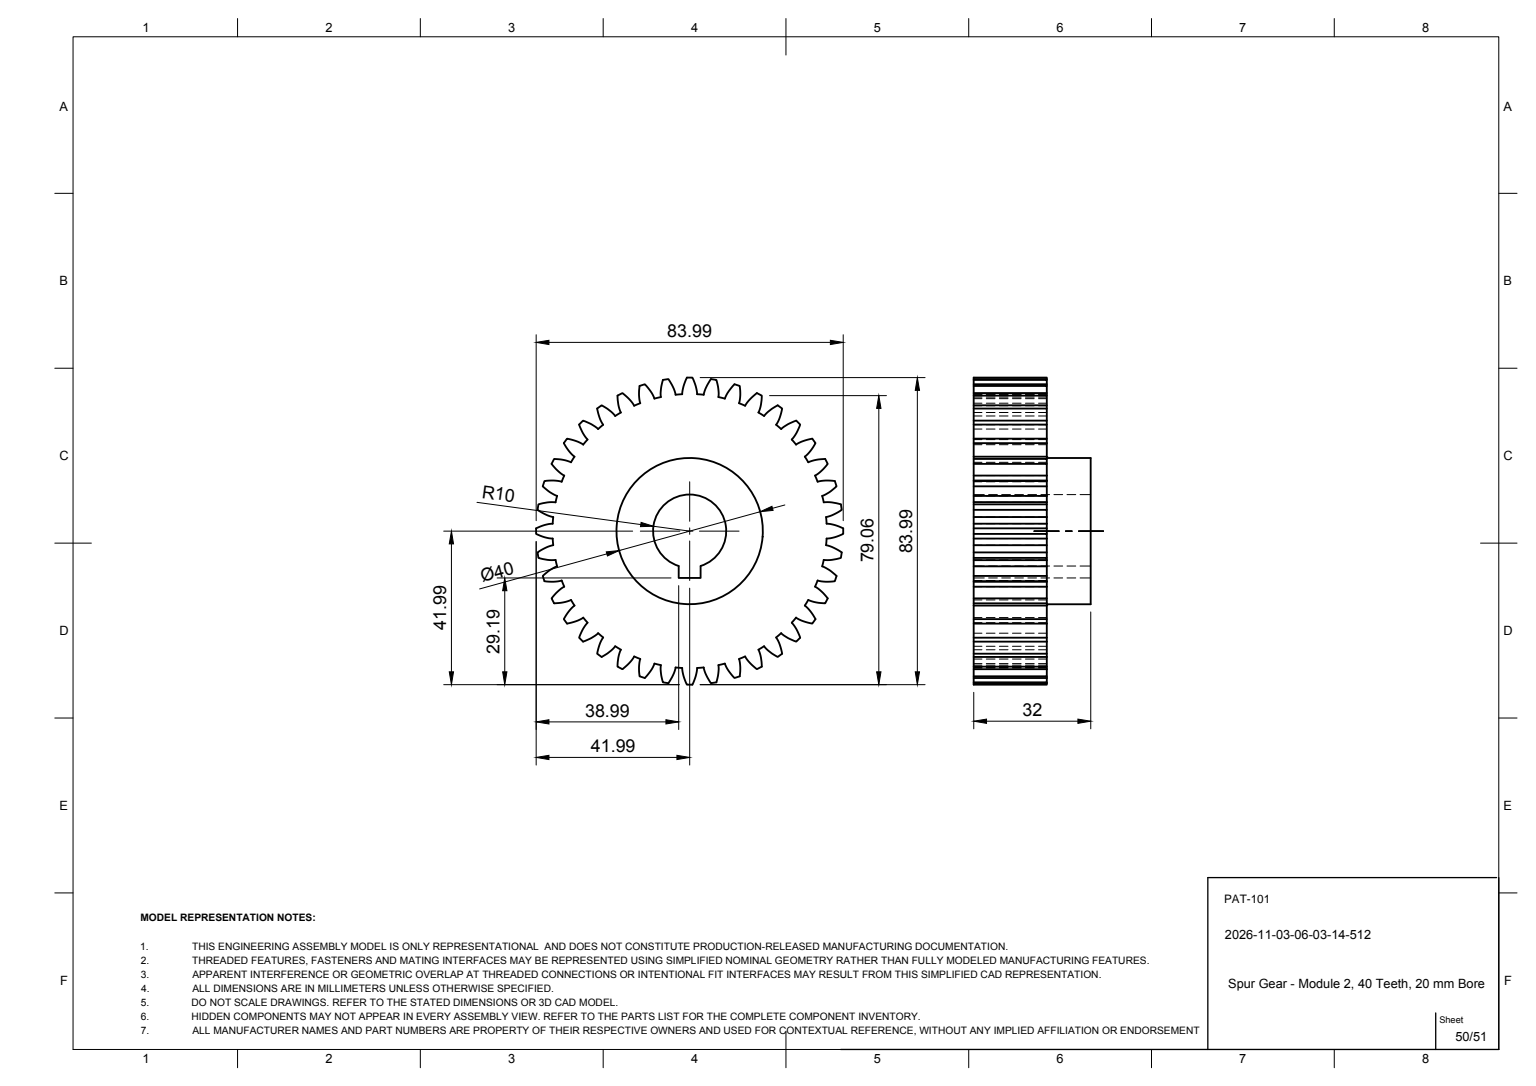
ISO-10303-21;
HEADER;
/* Generated by software containing ST-Developer
 * from STEP Tools, Inc. (www.steptools.com) 
 */

FILE_DESCRIPTION(
/* description */ ('Spur gear reduction stage 2-1 on bearing plates'),
/* implementation_level */ '2;1');

FILE_NAME(
/* name */ 'Spur Gear - Module 2, 40 Teeth, 20 mm Bore.step',
/* time_stamp */ '2026-10-28T03:22:07-07:00',
/* author */ (''),
/* organization */ (''),
/* preprocessor_version */ 'ST-DEVELOPER v20.2',
/* originating_system */ 'Autodesk Translation Framework v15.17.0.0',
/* authorisation */ '');

FILE_SCHEMA (('AUTOMOTIVE_DESIGN { 1 0 10303 214 3 1 1 }'));
ENDSEC;

DATA;
#10=MECHANICAL_DESIGN_GEOMETRIC_PRESENTATION_REPRESENTATION('',(#1002),#53909);
#51=(
BOUNDED_SURFACE()
B_SPLINE_SURFACE(5,1,((#35999,#36000),(#36001,#36002),(#36003,#36004),(#36005,
#36006),(#36007,#36008),(#36009,#36010),(#36011,#36012),(#36013,#36014),
(#36015,#36016),(#36017,#36018),(#36019,#36020),(#36021,#36022),(#36023,
#36024),(#36025,#36026),(#36027,#36028),(#36029,#36030),(#36031,#36032),
(#36033,#36034),(#36035,#36036),(#36037,#36038),(#36039,#36040),(#36041,
#36042),(#36043,#36044),(#36045,#36046),(#36047,#36048),(#36049,#36050),
(#36051,#36052),(#36053,#36054),(#36055,#36056),(#36057,#36058),(#36059,
#36060),(#36061,#36062),(#36063,#36064),(#36065,#36066),(#36067,#36068),
(#36069,#36070),(#36071,#36072),(#36073,#36074),(#36075,#36076),(#36077,
#36078),(#36079,#36080),(#36081,#36082),(#36083,#36084),(#36085,#36086),
(#36087,#36088),(#36089,#36090),(#36091,#36092),(#36093,#36094),(#36095,
#36096),(#36097,#36098),(#36099,#36100),(#36101,#36102),(#36103,#36104),
(#36105,#36106),(#36107,#36108),(#36109,#36110),(#36111,#36112),(#36113,
#36114),(#36115,#36116),(#36117,#36118),(#36119,#36120),(#36121,#36122),
(#36123,#36124),(#36125,#36126),(#36127,#36128),(#36129,#36130),(#36131,
#36132),(#36133,#36134),(#36135,#36136),(#36137,#36138)),.UNSPECIFIED.,
 .F.,.F.,.F.)
B_SPLINE_SURFACE_WITH_KNOTS((6,1,1,1,1,1,1,1,1,1,1,1,1,1,1,1,1,1,1,1,1,
1,1,1,1,1,1,1,1,1,1,1,1,1,1,1,1,1,1,1,1,1,1,1,1,1,1,1,1,1,1,1,1,1,1,1,1,
1,1,1,1,1,1,1,1,6),(2,2),(-1.,-0.984615384615383,-0.969230769230768,-0.953846153846152,
-0.938461538461537,-0.923076923076922,-0.907692307692306,-0.892307692307691,
-0.876923076923076,-0.86153846153846,-0.846153846153845,-0.83076923076923,
-0.815384615384614,-0.799999999999999,-0.784615384615384,-0.769230769230768,
-0.753846153846153,-0.738461538461538,-0.723076923076922,-0.707692307692307,
-0.692307692307692,-0.676923076923076,-0.661538461538461,-0.646153846153846,
-0.63076923076923,-0.615384615384615,-0.6,-0.584615384615384,-0.569230769230769,
-0.553846153846154,-0.538461538461538,-0.523076923076923,-0.507692307692308,
-0.492307692307692,-0.476923076923077,-0.461538461538462,-0.446153846153846,
-0.430769230769231,-0.415384615384615,-0.4,-0.384615384615385,-0.369230769230769,
-0.353846153846154,-0.338461538461538,-0.323076923076923,-0.307692307692308,
-0.292307692307692,-0.276923076923077,-0.261538461538462,-0.246153846153846,
-0.230769230769231,-0.215384615384615,-0.2,-0.184615384615385,-0.169230769230769,
-0.153846153846154,-0.138461538461538,-0.123076923076923,-0.107692307692308,
-0.0923076923076923,-0.0769230769230769,-0.0615384615384615,-0.0461538461538462,
-0.0307692307692308,-0.0153846153846154,0.),(-1.,1.),.UNSPECIFIED.)
GEOMETRIC_REPRESENTATION_ITEM()
RATIONAL_B_SPLINE_SURFACE(((1.,1.),(1.,1.),(1.,1.),(1.,1.),(1.,1.),(1.,
1.),(1.,1.),(1.,1.),(1.,1.),(1.,1.),(1.,1.),(1.,1.),(1.,1.),(1.,1.),(1.,
1.),(1.,1.),(1.,1.),(1.,1.),(1.,1.),(1.,1.),(1.,1.),(1.,1.),(1.,1.),(1.,
1.),(1.,1.),(1.,1.),(1.,1.),(1.,1.),(1.,1.),(1.,1.),(1.,1.),(1.,1.),(1.,
1.),(1.,1.),(1.,1.),(1.,1.),(1.,1.),(1.,1.),(1.,1.),(1.,1.),(1.,1.),(1.,
1.),(1.,1.),(1.,1.),(1.,1.),(1.,1.),(1.,1.),(1.,1.),(1.,1.),(1.,1.),(1.,
1.),(1.,1.),(1.,1.),(1.,1.),(1.,1.),(1.,1.),(1.,1.),(1.,1.),(1.,1.),(1.,
1.),(1.,1.),(1.,1.),(1.,1.),(1.,1.),(1.,1.),(1.,1.),(1.,1.),(1.,1.),(1.,
1.),(1.,1.)))
REPRESENTATION_ITEM('')
SURFACE()
);
#52=(
BOUNDED_SURFACE()
B_SPLINE_SURFACE(5,1,((#36218,#36219),(#36220,#36221),(#36222,#36223),(#36224,
#36225),(#36226,#36227),(#36228,#36229),(#36230,#36231),(#36232,#36233),
(#36234,#36235),(#36236,#36237),(#36238,#36239),(#36240,#36241),(#36242,
#36243),(#36244,#36245),(#36246,#36247),(#36248,#36249),(#36250,#36251),
(#36252,#36253),(#36254,#36255),(#36256,#36257),(#36258,#36259),(#36260,
#36261),(#36262,#36263),(#36264,#36265),(#36266,#36267),(#36268,#36269),
(#36270,#36271),(#36272,#36273),(#36274,#36275),(#36276,#36277),(#36278,
#36279),(#36280,#36281),(#36282,#36283),(#36284,#36285),(#36286,#36287),
(#36288,#36289),(#36290,#36291),(#36292,#36293),(#36294,#36295),(#36296,
#36297),(#36298,#36299),(#36300,#36301),(#36302,#36303),(#36304,#36305),
(#36306,#36307),(#36308,#36309),(#36310,#36311),(#36312,#36313),(#36314,
#36315),(#36316,#36317),(#36318,#36319),(#36320,#36321),(#36322,#36323),
(#36324,#36325),(#36326,#36327),(#36328,#36329),(#36330,#36331),(#36332,
#36333),(#36334,#36335),(#36336,#36337),(#36338,#36339),(#36340,#36341),
(#36342,#36343),(#36344,#36345),(#36346,#36347),(#36348,#36349),(#36350,
#36351),(#36352,#36353),(#36354,#36355),(#36356,#36357)),.UNSPECIFIED.,
 .F.,.F.,.F.)
B_SPLINE_SURFACE_WITH_KNOTS((6,1,1,1,1,1,1,1,1,1,1,1,1,1,1,1,1,1,1,1,1,
1,1,1,1,1,1,1,1,1,1,1,1,1,1,1,1,1,1,1,1,1,1,1,1,1,1,1,1,1,1,1,1,1,1,1,1,
1,1,1,1,1,1,1,1,6),(2,2),(-1.,-0.984615384615383,-0.969230769230768,-0.953846153846152,
-0.938461538461537,-0.923076923076922,-0.907692307692306,-0.892307692307691,
-0.876923076923076,-0.86153846153846,-0.846153846153845,-0.83076923076923,
-0.815384615384614,-0.799999999999999,-0.784615384615384,-0.769230769230768,
-0.753846153846153,-0.738461538461538,-0.723076923076922,-0.707692307692307,
-0.692307692307692,-0.676923076923076,-0.661538461538461,-0.646153846153846,
-0.63076923076923,-0.615384615384615,-0.6,-0.584615384615384,-0.569230769230769,
-0.553846153846154,-0.538461538461538,-0.523076923076923,-0.507692307692308,
-0.492307692307692,-0.476923076923077,-0.461538461538462,-0.446153846153846,
-0.430769230769231,-0.415384615384615,-0.4,-0.384615384615385,-0.369230769230769,
-0.353846153846154,-0.338461538461538,-0.323076923076923,-0.307692307692308,
-0.292307692307692,-0.276923076923077,-0.261538461538462,-0.246153846153846,
-0.230769230769231,-0.215384615384615,-0.2,-0.184615384615385,-0.169230769230769,
-0.153846153846154,-0.138461538461538,-0.123076923076923,-0.107692307692308,
-0.0923076923076923,-0.0769230769230769,-0.0615384615384615,-0.0461538461538462,
-0.0307692307692308,-0.0153846153846154,0.),(-1.,1.),.UNSPECIFIED.)
GEOMETRIC_REPRESENTATION_ITEM()
RATIONAL_B_SPLINE_SURFACE(((1.,1.),(1.,1.),(1.,1.),(1.,1.),(1.,1.),(1.,
1.),(1.,1.),(1.,1.),(1.,1.),(1.,1.),(1.,1.),(1.,1.),(1.,1.),(1.,1.),(1.,
1.),(1.,1.),(1.,1.),(1.,1.),(1.,1.),(1.,1.),(1.,1.),(1.,1.),(1.,1.),(1.,
1.),(1.,1.),(1.,1.),(1.,1.),(1.,1.),(1.,1.),(1.,1.),(1.,1.),(1.,1.),(1.,
1.),(1.,1.),(1.,1.),(1.,1.),(1.,1.),(1.,1.),(1.,1.),(1.,1.),(1.,1.),(1.,
1.),(1.,1.),(1.,1.),(1.,1.),(1.,1.),(1.,1.),(1.,1.),(1.,1.),(1.,1.),(1.,
1.),(1.,1.),(1.,1.),(1.,1.),(1.,1.),(1.,1.),(1.,1.),(1.,1.),(1.,1.),(1.,
1.),(1.,1.),(1.,1.),(1.,1.),(1.,1.),(1.,1.),(1.,1.),(1.,1.),(1.,1.),(1.,
1.),(1.,1.)))
REPRESENTATION_ITEM('')
SURFACE()
);
#53=(
BOUNDED_SURFACE()
B_SPLINE_SURFACE(5,1,((#36448,#36449),(#36450,#36451),(#36452,#36453),(#36454,
#36455),(#36456,#36457),(#36458,#36459),(#36460,#36461),(#36462,#36463),
(#36464,#36465),(#36466,#36467),(#36468,#36469),(#36470,#36471),(#36472,
#36473),(#36474,#36475),(#36476,#36477),(#36478,#36479),(#36480,#36481),
(#36482,#36483),(#36484,#36485),(#36486,#36487),(#36488,#36489),(#36490,
#36491),(#36492,#36493),(#36494,#36495),(#36496,#36497),(#36498,#36499),
(#36500,#36501),(#36502,#36503),(#36504,#36505),(#36506,#36507),(#36508,
#36509),(#36510,#36511),(#36512,#36513),(#36514,#36515),(#36516,#36517),
(#36518,#36519),(#36520,#36521),(#36522,#36523),(#36524,#36525),(#36526,
#36527),(#36528,#36529),(#36530,#36531),(#36532,#36533),(#36534,#36535),
(#36536,#36537),(#36538,#36539),(#36540,#36541),(#36542,#36543),(#36544,
#36545),(#36546,#36547),(#36548,#36549),(#36550,#36551),(#36552,#36553),
(#36554,#36555),(#36556,#36557),(#36558,#36559),(#36560,#36561),(#36562,
#36563),(#36564,#36565),(#36566,#36567),(#36568,#36569),(#36570,#36571),
(#36572,#36573),(#36574,#36575),(#36576,#36577),(#36578,#36579),(#36580,
#36581),(#36582,#36583),(#36584,#36585),(#36586,#36587)),.UNSPECIFIED.,
 .F.,.F.,.F.)
B_SPLINE_SURFACE_WITH_KNOTS((6,1,1,1,1,1,1,1,1,1,1,1,1,1,1,1,1,1,1,1,1,
1,1,1,1,1,1,1,1,1,1,1,1,1,1,1,1,1,1,1,1,1,1,1,1,1,1,1,1,1,1,1,1,1,1,1,1,
1,1,1,1,1,1,1,1,6),(2,2),(-1.,-0.984615384615383,-0.969230769230768,-0.953846153846152,
-0.938461538461537,-0.923076923076922,-0.907692307692306,-0.892307692307691,
-0.876923076923076,-0.86153846153846,-0.846153846153845,-0.83076923076923,
-0.815384615384614,-0.799999999999999,-0.784615384615384,-0.769230769230768,
-0.753846153846153,-0.738461538461538,-0.723076923076922,-0.707692307692307,
-0.692307692307692,-0.676923076923076,-0.661538461538461,-0.646153846153846,
-0.63076923076923,-0.615384615384615,-0.6,-0.584615384615384,-0.569230769230769,
-0.553846153846154,-0.538461538461538,-0.523076923076923,-0.507692307692308,
-0.492307692307692,-0.476923076923077,-0.461538461538462,-0.446153846153846,
-0.430769230769231,-0.415384615384615,-0.4,-0.384615384615385,-0.369230769230769,
-0.353846153846154,-0.338461538461538,-0.323076923076923,-0.307692307692308,
-0.292307692307692,-0.276923076923077,-0.261538461538462,-0.246153846153846,
-0.230769230769231,-0.215384615384615,-0.2,-0.184615384615385,-0.169230769230769,
-0.153846153846154,-0.138461538461538,-0.123076923076923,-0.107692307692308,
-0.0923076923076923,-0.0769230769230769,-0.0615384615384615,-0.0461538461538462,
-0.0307692307692308,-0.0153846153846154,0.),(-1.,1.),.UNSPECIFIED.)
GEOMETRIC_REPRESENTATION_ITEM()
RATIONAL_B_SPLINE_SURFACE(((1.,1.),(1.,1.),(1.,1.),(1.,1.),(1.,1.),(1.,
1.),(1.,1.),(1.,1.),(1.,1.),(1.,1.),(1.,1.),(1.,1.),(1.,1.),(1.,1.),(1.,
1.),(1.,1.),(1.,1.),(1.,1.),(1.,1.),(1.,1.),(1.,1.),(1.,1.),(1.,1.),(1.,
1.),(1.,1.),(1.,1.),(1.,1.),(1.,1.),(1.,1.),(1.,1.),(1.,1.),(1.,1.),(1.,
1.),(1.,1.),(1.,1.),(1.,1.),(1.,1.),(1.,1.),(1.,1.),(1.,1.),(1.,1.),(1.,
1.),(1.,1.),(1.,1.),(1.,1.),(1.,1.),(1.,1.),(1.,1.),(1.,1.),(1.,1.),(1.,
1.),(1.,1.),(1.,1.),(1.,1.),(1.,1.),(1.,1.),(1.,1.),(1.,1.),(1.,1.),(1.,
1.),(1.,1.),(1.,1.),(1.,1.),(1.,1.),(1.,1.),(1.,1.),(1.,1.),(1.,1.),(1.,
1.),(1.,1.)))
REPRESENTATION_ITEM('')
SURFACE()
);
#54=(
BOUNDED_SURFACE()
B_SPLINE_SURFACE(5,1,((#36660,#36661),(#36662,#36663),(#36664,#36665),(#36666,
#36667),(#36668,#36669),(#36670,#36671),(#36672,#36673),(#36674,#36675),
(#36676,#36677),(#36678,#36679),(#36680,#36681),(#36682,#36683),(#36684,
#36685),(#36686,#36687),(#36688,#36689),(#36690,#36691),(#36692,#36693),
(#36694,#36695),(#36696,#36697),(#36698,#36699),(#36700,#36701),(#36702,
#36703),(#36704,#36705),(#36706,#36707),(#36708,#36709),(#36710,#36711),
(#36712,#36713),(#36714,#36715),(#36716,#36717),(#36718,#36719),(#36720,
#36721),(#36722,#36723),(#36724,#36725),(#36726,#36727),(#36728,#36729),
(#36730,#36731),(#36732,#36733),(#36734,#36735),(#36736,#36737),(#36738,
#36739),(#36740,#36741),(#36742,#36743),(#36744,#36745),(#36746,#36747),
(#36748,#36749),(#36750,#36751),(#36752,#36753),(#36754,#36755),(#36756,
#36757),(#36758,#36759),(#36760,#36761),(#36762,#36763),(#36764,#36765),
(#36766,#36767),(#36768,#36769),(#36770,#36771),(#36772,#36773),(#36774,
#36775),(#36776,#36777),(#36778,#36779),(#36780,#36781),(#36782,#36783),
(#36784,#36785),(#36786,#36787),(#36788,#36789),(#36790,#36791),(#36792,
#36793),(#36794,#36795),(#36796,#36797),(#36798,#36799)),.UNSPECIFIED.,
 .F.,.F.,.F.)
B_SPLINE_SURFACE_WITH_KNOTS((6,1,1,1,1,1,1,1,1,1,1,1,1,1,1,1,1,1,1,1,1,
1,1,1,1,1,1,1,1,1,1,1,1,1,1,1,1,1,1,1,1,1,1,1,1,1,1,1,1,1,1,1,1,1,1,1,1,
1,1,1,1,1,1,1,1,6),(2,2),(-1.,-0.984615384615383,-0.969230769230768,-0.953846153846152,
-0.938461538461537,-0.923076923076922,-0.907692307692306,-0.892307692307691,
-0.876923076923076,-0.86153846153846,-0.846153846153845,-0.83076923076923,
-0.815384615384614,-0.799999999999999,-0.784615384615384,-0.769230769230768,
-0.753846153846153,-0.738461538461538,-0.723076923076922,-0.707692307692307,
-0.692307692307692,-0.676923076923076,-0.661538461538461,-0.646153846153846,
-0.63076923076923,-0.615384615384615,-0.6,-0.584615384615384,-0.569230769230769,
-0.553846153846154,-0.538461538461538,-0.523076923076923,-0.507692307692308,
-0.492307692307692,-0.476923076923077,-0.461538461538462,-0.446153846153846,
-0.430769230769231,-0.415384615384615,-0.4,-0.384615384615385,-0.369230769230769,
-0.353846153846154,-0.338461538461538,-0.323076923076923,-0.307692307692308,
-0.292307692307692,-0.276923076923077,-0.261538461538462,-0.246153846153846,
-0.230769230769231,-0.215384615384615,-0.2,-0.184615384615385,-0.169230769230769,
-0.153846153846154,-0.138461538461538,-0.123076923076923,-0.107692307692308,
-0.0923076923076923,-0.0769230769230769,-0.0615384615384615,-0.0461538461538462,
-0.0307692307692308,-0.0153846153846154,0.),(-1.,1.),.UNSPECIFIED.)
GEOMETRIC_REPRESENTATION_ITEM()
RATIONAL_B_SPLINE_SURFACE(((1.,1.),(1.,1.),(1.,1.),(1.,1.),(1.,1.),(1.,
1.),(1.,1.),(1.,1.),(1.,1.),(1.,1.),(1.,1.),(1.,1.),(1.,1.),(1.,1.),(1.,
1.),(1.,1.),(1.,1.),(1.,1.),(1.,1.),(1.,1.),(1.,1.),(1.,1.),(1.,1.),(1.,
1.),(1.,1.),(1.,1.),(1.,1.),(1.,1.),(1.,1.),(1.,1.),(1.,1.),(1.,1.),(1.,
1.),(1.,1.),(1.,1.),(1.,1.),(1.,1.),(1.,1.),(1.,1.),(1.,1.),(1.,1.),(1.,
1.),(1.,1.),(1.,1.),(1.,1.),(1.,1.),(1.,1.),(1.,1.),(1.,1.),(1.,1.),(1.,
1.),(1.,1.),(1.,1.),(1.,1.),(1.,1.),(1.,1.),(1.,1.),(1.,1.),(1.,1.),(1.,
1.),(1.,1.),(1.,1.),(1.,1.),(1.,1.),(1.,1.),(1.,1.),(1.,1.),(1.,1.),(1.,
1.),(1.,1.)))
REPRESENTATION_ITEM('')
SURFACE()
);
#55=(
BOUNDED_SURFACE()
B_SPLINE_SURFACE(5,1,((#36890,#36891),(#36892,#36893),(#36894,#36895),(#36896,
#36897),(#36898,#36899),(#36900,#36901),(#36902,#36903),(#36904,#36905),
(#36906,#36907),(#36908,#36909),(#36910,#36911),(#36912,#36913),(#36914,
#36915),(#36916,#36917),(#36918,#36919),(#36920,#36921),(#36922,#36923),
(#36924,#36925),(#36926,#36927),(#36928,#36929),(#36930,#36931),(#36932,
#36933),(#36934,#36935),(#36936,#36937),(#36938,#36939),(#36940,#36941),
(#36942,#36943),(#36944,#36945),(#36946,#36947),(#36948,#36949),(#36950,
#36951),(#36952,#36953),(#36954,#36955),(#36956,#36957),(#36958,#36959),
(#36960,#36961),(#36962,#36963),(#36964,#36965),(#36966,#36967),(#36968,
#36969),(#36970,#36971),(#36972,#36973),(#36974,#36975),(#36976,#36977),
(#36978,#36979),(#36980,#36981),(#36982,#36983),(#36984,#36985),(#36986,
#36987),(#36988,#36989),(#36990,#36991),(#36992,#36993),(#36994,#36995),
(#36996,#36997),(#36998,#36999),(#37000,#37001),(#37002,#37003),(#37004,
#37005),(#37006,#37007),(#37008,#37009),(#37010,#37011),(#37012,#37013),
(#37014,#37015),(#37016,#37017),(#37018,#37019),(#37020,#37021),(#37022,
#37023),(#37024,#37025),(#37026,#37027),(#37028,#37029)),.UNSPECIFIED.,
 .F.,.F.,.F.)
B_SPLINE_SURFACE_WITH_KNOTS((6,1,1,1,1,1,1,1,1,1,1,1,1,1,1,1,1,1,1,1,1,
1,1,1,1,1,1,1,1,1,1,1,1,1,1,1,1,1,1,1,1,1,1,1,1,1,1,1,1,1,1,1,1,1,1,1,1,
1,1,1,1,1,1,1,1,6),(2,2),(-1.,-0.984615384615383,-0.969230769230768,-0.953846153846152,
-0.938461538461537,-0.923076923076922,-0.907692307692306,-0.892307692307691,
-0.876923076923076,-0.86153846153846,-0.846153846153845,-0.83076923076923,
-0.815384615384614,-0.799999999999999,-0.784615384615384,-0.769230769230768,
-0.753846153846153,-0.738461538461538,-0.723076923076922,-0.707692307692307,
-0.692307692307692,-0.676923076923076,-0.661538461538461,-0.646153846153846,
-0.63076923076923,-0.615384615384615,-0.6,-0.584615384615384,-0.569230769230769,
-0.553846153846154,-0.538461538461538,-0.523076923076923,-0.507692307692308,
-0.492307692307692,-0.476923076923077,-0.461538461538462,-0.446153846153846,
-0.430769230769231,-0.415384615384615,-0.4,-0.384615384615385,-0.369230769230769,
-0.353846153846154,-0.338461538461538,-0.323076923076923,-0.307692307692308,
-0.292307692307692,-0.276923076923077,-0.261538461538462,-0.246153846153846,
-0.230769230769231,-0.215384615384615,-0.2,-0.184615384615385,-0.169230769230769,
-0.153846153846154,-0.138461538461538,-0.123076923076923,-0.107692307692308,
-0.0923076923076923,-0.0769230769230769,-0.0615384615384615,-0.0461538461538462,
-0.0307692307692308,-0.0153846153846154,0.),(-1.,1.),.UNSPECIFIED.)
GEOMETRIC_REPRESENTATION_ITEM()
RATIONAL_B_SPLINE_SURFACE(((1.,1.),(1.,1.),(1.,1.),(1.,1.),(1.,1.),(1.,
1.),(1.,1.),(1.,1.),(1.,1.),(1.,1.),(1.,1.),(1.,1.),(1.,1.),(1.,1.),(1.,
1.),(1.,1.),(1.,1.),(1.,1.),(1.,1.),(1.,1.),(1.,1.),(1.,1.),(1.,1.),(1.,
1.),(1.,1.),(1.,1.),(1.,1.),(1.,1.),(1.,1.),(1.,1.),(1.,1.),(1.,1.),(1.,
1.),(1.,1.),(1.,1.),(1.,1.),(1.,1.),(1.,1.),(1.,1.),(1.,1.),(1.,1.),(1.,
1.),(1.,1.),(1.,1.),(1.,1.),(1.,1.),(1.,1.),(1.,1.),(1.,1.),(1.,1.),(1.,
1.),(1.,1.),(1.,1.),(1.,1.),(1.,1.),(1.,1.),(1.,1.),(1.,1.),(1.,1.),(1.,
1.),(1.,1.),(1.,1.),(1.,1.),(1.,1.),(1.,1.),(1.,1.),(1.,1.),(1.,1.),(1.,
1.),(1.,1.)))
REPRESENTATION_ITEM('')
SURFACE()
);
#56=(
BOUNDED_SURFACE()
B_SPLINE_SURFACE(5,1,((#37102,#37103),(#37104,#37105),(#37106,#37107),(#37108,
#37109),(#37110,#37111),(#37112,#37113),(#37114,#37115),(#37116,#37117),
(#37118,#37119),(#37120,#37121),(#37122,#37123),(#37124,#37125),(#37126,
#37127),(#37128,#37129),(#37130,#37131),(#37132,#37133),(#37134,#37135),
(#37136,#37137),(#37138,#37139),(#37140,#37141),(#37142,#37143),(#37144,
#37145),(#37146,#37147),(#37148,#37149),(#37150,#37151),(#37152,#37153),
(#37154,#37155),(#37156,#37157),(#37158,#37159),(#37160,#37161),(#37162,
#37163),(#37164,#37165),(#37166,#37167),(#37168,#37169),(#37170,#37171),
(#37172,#37173),(#37174,#37175),(#37176,#37177),(#37178,#37179),(#37180,
#37181),(#37182,#37183),(#37184,#37185),(#37186,#37187),(#37188,#37189),
(#37190,#37191),(#37192,#37193),(#37194,#37195),(#37196,#37197),(#37198,
#37199),(#37200,#37201),(#37202,#37203),(#37204,#37205),(#37206,#37207),
(#37208,#37209),(#37210,#37211),(#37212,#37213),(#37214,#37215),(#37216,
#37217),(#37218,#37219),(#37220,#37221),(#37222,#37223),(#37224,#37225),
(#37226,#37227),(#37228,#37229),(#37230,#37231),(#37232,#37233),(#37234,
#37235),(#37236,#37237),(#37238,#37239),(#37240,#37241)),.UNSPECIFIED.,
 .F.,.F.,.F.)
B_SPLINE_SURFACE_WITH_KNOTS((6,1,1,1,1,1,1,1,1,1,1,1,1,1,1,1,1,1,1,1,1,
1,1,1,1,1,1,1,1,1,1,1,1,1,1,1,1,1,1,1,1,1,1,1,1,1,1,1,1,1,1,1,1,1,1,1,1,
1,1,1,1,1,1,1,1,6),(2,2),(-1.,-0.984615384615383,-0.969230769230768,-0.953846153846152,
-0.938461538461537,-0.923076923076922,-0.907692307692306,-0.892307692307691,
-0.876923076923076,-0.86153846153846,-0.846153846153845,-0.83076923076923,
-0.815384615384614,-0.799999999999999,-0.784615384615384,-0.769230769230768,
-0.753846153846153,-0.738461538461538,-0.723076923076922,-0.707692307692307,
-0.692307692307692,-0.676923076923076,-0.661538461538461,-0.646153846153846,
-0.63076923076923,-0.615384615384615,-0.6,-0.584615384615384,-0.569230769230769,
-0.553846153846154,-0.538461538461538,-0.523076923076923,-0.507692307692308,
-0.492307692307692,-0.476923076923077,-0.461538461538462,-0.446153846153846,
-0.430769230769231,-0.415384615384615,-0.4,-0.384615384615385,-0.369230769230769,
-0.353846153846154,-0.338461538461538,-0.323076923076923,-0.307692307692308,
-0.292307692307692,-0.276923076923077,-0.261538461538462,-0.246153846153846,
-0.230769230769231,-0.215384615384615,-0.2,-0.184615384615385,-0.169230769230769,
-0.153846153846154,-0.138461538461538,-0.123076923076923,-0.107692307692308,
-0.0923076923076923,-0.0769230769230769,-0.0615384615384615,-0.0461538461538462,
-0.0307692307692308,-0.0153846153846154,0.),(-1.,1.),.UNSPECIFIED.)
GEOMETRIC_REPRESENTATION_ITEM()
RATIONAL_B_SPLINE_SURFACE(((1.,1.),(1.,1.),(1.,1.),(1.,1.),(1.,1.),(1.,
1.),(1.,1.),(1.,1.),(1.,1.),(1.,1.),(1.,1.),(1.,1.),(1.,1.),(1.,1.),(1.,
1.),(1.,1.),(1.,1.),(1.,1.),(1.,1.),(1.,1.),(1.,1.),(1.,1.),(1.,1.),(1.,
1.),(1.,1.),(1.,1.),(1.,1.),(1.,1.),(1.,1.),(1.,1.),(1.,1.),(1.,1.),(1.,
1.),(1.,1.),(1.,1.),(1.,1.),(1.,1.),(1.,1.),(1.,1.),(1.,1.),(1.,1.),(1.,
1.),(1.,1.),(1.,1.),(1.,1.),(1.,1.),(1.,1.),(1.,1.),(1.,1.),(1.,1.),(1.,
1.),(1.,1.),(1.,1.),(1.,1.),(1.,1.),(1.,1.),(1.,1.),(1.,1.),(1.,1.),(1.,
1.),(1.,1.),(1.,1.),(1.,1.),(1.,1.),(1.,1.),(1.,1.),(1.,1.),(1.,1.),(1.,
1.),(1.,1.)))
REPRESENTATION_ITEM('')
SURFACE()
);
#57=(
BOUNDED_SURFACE()
B_SPLINE_SURFACE(5,1,((#37332,#37333),(#37334,#37335),(#37336,#37337),(#37338,
#37339),(#37340,#37341),(#37342,#37343),(#37344,#37345),(#37346,#37347),
(#37348,#37349),(#37350,#37351),(#37352,#37353),(#37354,#37355),(#37356,
#37357),(#37358,#37359),(#37360,#37361),(#37362,#37363),(#37364,#37365),
(#37366,#37367),(#37368,#37369),(#37370,#37371),(#37372,#37373),(#37374,
#37375),(#37376,#37377),(#37378,#37379),(#37380,#37381),(#37382,#37383),
(#37384,#37385),(#37386,#37387),(#37388,#37389),(#37390,#37391),(#37392,
#37393),(#37394,#37395),(#37396,#37397),(#37398,#37399),(#37400,#37401),
(#37402,#37403),(#37404,#37405),(#37406,#37407),(#37408,#37409),(#37410,
#37411),(#37412,#37413),(#37414,#37415),(#37416,#37417),(#37418,#37419),
(#37420,#37421),(#37422,#37423),(#37424,#37425),(#37426,#37427),(#37428,
#37429),(#37430,#37431),(#37432,#37433),(#37434,#37435),(#37436,#37437),
(#37438,#37439),(#37440,#37441),(#37442,#37443),(#37444,#37445),(#37446,
#37447),(#37448,#37449),(#37450,#37451),(#37452,#37453),(#37454,#37455),
(#37456,#37457),(#37458,#37459),(#37460,#37461),(#37462,#37463),(#37464,
#37465),(#37466,#37467),(#37468,#37469),(#37470,#37471)),.UNSPECIFIED.,
 .F.,.F.,.F.)
B_SPLINE_SURFACE_WITH_KNOTS((6,1,1,1,1,1,1,1,1,1,1,1,1,1,1,1,1,1,1,1,1,
1,1,1,1,1,1,1,1,1,1,1,1,1,1,1,1,1,1,1,1,1,1,1,1,1,1,1,1,1,1,1,1,1,1,1,1,
1,1,1,1,1,1,1,1,6),(2,2),(-1.,-0.984615384615383,-0.969230769230768,-0.953846153846152,
-0.938461538461537,-0.923076923076922,-0.907692307692306,-0.892307692307691,
-0.876923076923076,-0.86153846153846,-0.846153846153845,-0.83076923076923,
-0.815384615384614,-0.799999999999999,-0.784615384615384,-0.769230769230768,
-0.753846153846153,-0.738461538461538,-0.723076923076922,-0.707692307692307,
-0.692307692307692,-0.676923076923076,-0.661538461538461,-0.646153846153846,
-0.63076923076923,-0.615384615384615,-0.6,-0.584615384615384,-0.569230769230769,
-0.553846153846154,-0.538461538461538,-0.523076923076923,-0.507692307692308,
-0.492307692307692,-0.476923076923077,-0.461538461538462,-0.446153846153846,
-0.430769230769231,-0.415384615384615,-0.4,-0.384615384615385,-0.369230769230769,
-0.353846153846154,-0.338461538461538,-0.323076923076923,-0.307692307692308,
-0.292307692307692,-0.276923076923077,-0.261538461538462,-0.246153846153846,
-0.230769230769231,-0.215384615384615,-0.2,-0.184615384615385,-0.169230769230769,
-0.153846153846154,-0.138461538461538,-0.123076923076923,-0.107692307692308,
-0.0923076923076923,-0.0769230769230769,-0.0615384615384615,-0.0461538461538462,
-0.0307692307692308,-0.0153846153846154,0.),(-1.,1.),.UNSPECIFIED.)
GEOMETRIC_REPRESENTATION_ITEM()
RATIONAL_B_SPLINE_SURFACE(((1.,1.),(1.,1.),(1.,1.),(1.,1.),(1.,1.),(1.,
1.),(1.,1.),(1.,1.),(1.,1.),(1.,1.),(1.,1.),(1.,1.),(1.,1.),(1.,1.),(1.,
1.),(1.,1.),(1.,1.),(1.,1.),(1.,1.),(1.,1.),(1.,1.),(1.,1.),(1.,1.),(1.,
1.),(1.,1.),(1.,1.),(1.,1.),(1.,1.),(1.,1.),(1.,1.),(1.,1.),(1.,1.),(1.,
1.),(1.,1.),(1.,1.),(1.,1.),(1.,1.),(1.,1.),(1.,1.),(1.,1.),(1.,1.),(1.,
1.),(1.,1.),(1.,1.),(1.,1.),(1.,1.),(1.,1.),(1.,1.),(1.,1.),(1.,1.),(1.,
1.),(1.,1.),(1.,1.),(1.,1.),(1.,1.),(1.,1.),(1.,1.),(1.,1.),(1.,1.),(1.,
1.),(1.,1.),(1.,1.),(1.,1.),(1.,1.),(1.,1.),(1.,1.),(1.,1.),(1.,1.),(1.,
1.),(1.,1.)))
REPRESENTATION_ITEM('')
SURFACE()
);
#58=(
BOUNDED_SURFACE()
B_SPLINE_SURFACE(5,1,((#37544,#37545),(#37546,#37547),(#37548,#37549),(#37550,
#37551),(#37552,#37553),(#37554,#37555),(#37556,#37557),(#37558,#37559),
(#37560,#37561),(#37562,#37563),(#37564,#37565),(#37566,#37567),(#37568,
#37569),(#37570,#37571),(#37572,#37573),(#37574,#37575),(#37576,#37577),
(#37578,#37579),(#37580,#37581),(#37582,#37583),(#37584,#37585),(#37586,
#37587),(#37588,#37589),(#37590,#37591),(#37592,#37593),(#37594,#37595),
(#37596,#37597),(#37598,#37599),(#37600,#37601),(#37602,#37603),(#37604,
#37605),(#37606,#37607),(#37608,#37609),(#37610,#37611),(#37612,#37613),
(#37614,#37615),(#37616,#37617),(#37618,#37619),(#37620,#37621),(#37622,
#37623),(#37624,#37625),(#37626,#37627),(#37628,#37629),(#37630,#37631),
(#37632,#37633),(#37634,#37635),(#37636,#37637),(#37638,#37639),(#37640,
#37641),(#37642,#37643),(#37644,#37645),(#37646,#37647),(#37648,#37649),
(#37650,#37651),(#37652,#37653),(#37654,#37655),(#37656,#37657),(#37658,
#37659),(#37660,#37661),(#37662,#37663),(#37664,#37665),(#37666,#37667),
(#37668,#37669),(#37670,#37671),(#37672,#37673),(#37674,#37675),(#37676,
#37677),(#37678,#37679),(#37680,#37681),(#37682,#37683)),.UNSPECIFIED.,
 .F.,.F.,.F.)
B_SPLINE_SURFACE_WITH_KNOTS((6,1,1,1,1,1,1,1,1,1,1,1,1,1,1,1,1,1,1,1,1,
1,1,1,1,1,1,1,1,1,1,1,1,1,1,1,1,1,1,1,1,1,1,1,1,1,1,1,1,1,1,1,1,1,1,1,1,
1,1,1,1,1,1,1,1,6),(2,2),(-1.,-0.984615384615383,-0.969230769230768,-0.953846153846152,
-0.938461538461537,-0.923076923076922,-0.907692307692306,-0.892307692307691,
-0.876923076923076,-0.86153846153846,-0.846153846153845,-0.83076923076923,
-0.815384615384614,-0.799999999999999,-0.784615384615384,-0.769230769230768,
-0.753846153846153,-0.738461538461538,-0.723076923076922,-0.707692307692307,
-0.692307692307692,-0.676923076923076,-0.661538461538461,-0.646153846153846,
-0.63076923076923,-0.615384615384615,-0.6,-0.584615384615384,-0.569230769230769,
-0.553846153846154,-0.538461538461538,-0.523076923076923,-0.507692307692308,
-0.492307692307692,-0.476923076923077,-0.461538461538462,-0.446153846153846,
-0.430769230769231,-0.415384615384615,-0.4,-0.384615384615385,-0.369230769230769,
-0.353846153846154,-0.338461538461538,-0.323076923076923,-0.307692307692308,
-0.292307692307692,-0.276923076923077,-0.261538461538462,-0.246153846153846,
-0.230769230769231,-0.215384615384615,-0.2,-0.184615384615385,-0.169230769230769,
-0.153846153846154,-0.138461538461538,-0.123076923076923,-0.107692307692308,
-0.0923076923076923,-0.0769230769230769,-0.0615384615384615,-0.0461538461538462,
-0.0307692307692308,-0.0153846153846154,0.),(-1.,1.),.UNSPECIFIED.)
GEOMETRIC_REPRESENTATION_ITEM()
RATIONAL_B_SPLINE_SURFACE(((1.,1.),(1.,1.),(1.,1.),(1.,1.),(1.,1.),(1.,
1.),(1.,1.),(1.,1.),(1.,1.),(1.,1.),(1.,1.),(1.,1.),(1.,1.),(1.,1.),(1.,
1.),(1.,1.),(1.,1.),(1.,1.),(1.,1.),(1.,1.),(1.,1.),(1.,1.),(1.,1.),(1.,
1.),(1.,1.),(1.,1.),(1.,1.),(1.,1.),(1.,1.),(1.,1.),(1.,1.),(1.,1.),(1.,
1.),(1.,1.),(1.,1.),(1.,1.),(1.,1.),(1.,1.),(1.,1.),(1.,1.),(1.,1.),(1.,
1.),(1.,1.),(1.,1.),(1.,1.),(1.,1.),(1.,1.),(1.,1.),(1.,1.),(1.,1.),(1.,
1.),(1.,1.),(1.,1.),(1.,1.),(1.,1.),(1.,1.),(1.,1.),(1.,1.),(1.,1.),(1.,
1.),(1.,1.),(1.,1.),(1.,1.),(1.,1.),(1.,1.),(1.,1.),(1.,1.),(1.,1.),(1.,
1.),(1.,1.)))
REPRESENTATION_ITEM('')
SURFACE()
);
#59=(
BOUNDED_SURFACE()
B_SPLINE_SURFACE(5,1,((#37774,#37775),(#37776,#37777),(#37778,#37779),(#37780,
#37781),(#37782,#37783),(#37784,#37785),(#37786,#37787),(#37788,#37789),
(#37790,#37791),(#37792,#37793),(#37794,#37795),(#37796,#37797),(#37798,
#37799),(#37800,#37801),(#37802,#37803),(#37804,#37805),(#37806,#37807),
(#37808,#37809),(#37810,#37811),(#37812,#37813),(#37814,#37815),(#37816,
#37817),(#37818,#37819),(#37820,#37821),(#37822,#37823),(#37824,#37825),
(#37826,#37827),(#37828,#37829),(#37830,#37831),(#37832,#37833),(#37834,
#37835),(#37836,#37837),(#37838,#37839),(#37840,#37841),(#37842,#37843),
(#37844,#37845),(#37846,#37847),(#37848,#37849),(#37850,#37851),(#37852,
#37853),(#37854,#37855),(#37856,#37857),(#37858,#37859),(#37860,#37861),
(#37862,#37863),(#37864,#37865),(#37866,#37867),(#37868,#37869),(#37870,
#37871),(#37872,#37873),(#37874,#37875),(#37876,#37877),(#37878,#37879),
(#37880,#37881),(#37882,#37883),(#37884,#37885),(#37886,#37887),(#37888,
#37889),(#37890,#37891),(#37892,#37893),(#37894,#37895),(#37896,#37897),
(#37898,#37899),(#37900,#37901),(#37902,#37903),(#37904,#37905),(#37906,
#37907),(#37908,#37909),(#37910,#37911),(#37912,#37913)),.UNSPECIFIED.,
 .F.,.F.,.F.)
B_SPLINE_SURFACE_WITH_KNOTS((6,1,1,1,1,1,1,1,1,1,1,1,1,1,1,1,1,1,1,1,1,
1,1,1,1,1,1,1,1,1,1,1,1,1,1,1,1,1,1,1,1,1,1,1,1,1,1,1,1,1,1,1,1,1,1,1,1,
1,1,1,1,1,1,1,1,6),(2,2),(-1.,-0.984615384615383,-0.969230769230768,-0.953846153846152,
-0.938461538461537,-0.923076923076922,-0.907692307692306,-0.892307692307691,
-0.876923076923076,-0.86153846153846,-0.846153846153845,-0.83076923076923,
-0.815384615384614,-0.799999999999999,-0.784615384615384,-0.769230769230768,
-0.753846153846153,-0.738461538461538,-0.723076923076922,-0.707692307692307,
-0.692307692307692,-0.676923076923076,-0.661538461538461,-0.646153846153846,
-0.63076923076923,-0.615384615384615,-0.6,-0.584615384615384,-0.569230769230769,
-0.553846153846154,-0.538461538461538,-0.523076923076923,-0.507692307692308,
-0.492307692307692,-0.476923076923077,-0.461538461538462,-0.446153846153846,
-0.430769230769231,-0.415384615384615,-0.4,-0.384615384615385,-0.369230769230769,
-0.353846153846154,-0.338461538461538,-0.323076923076923,-0.307692307692308,
-0.292307692307692,-0.276923076923077,-0.261538461538462,-0.246153846153846,
-0.230769230769231,-0.215384615384615,-0.2,-0.184615384615385,-0.169230769230769,
-0.153846153846154,-0.138461538461538,-0.123076923076923,-0.107692307692308,
-0.0923076923076923,-0.0769230769230769,-0.0615384615384615,-0.0461538461538462,
-0.0307692307692308,-0.0153846153846154,0.),(-1.,1.),.UNSPECIFIED.)
GEOMETRIC_REPRESENTATION_ITEM()
RATIONAL_B_SPLINE_SURFACE(((1.,1.),(1.,1.),(1.,1.),(1.,1.),(1.,1.),(1.,
1.),(1.,1.),(1.,1.),(1.,1.),(1.,1.),(1.,1.),(1.,1.),(1.,1.),(1.,1.),(1.,
1.),(1.,1.),(1.,1.),(1.,1.),(1.,1.),(1.,1.),(1.,1.),(1.,1.),(1.,1.),(1.,
1.),(1.,1.),(1.,1.),(1.,1.),(1.,1.),(1.,1.),(1.,1.),(1.,1.),(1.,1.),(1.,
1.),(1.,1.),(1.,1.),(1.,1.),(1.,1.),(1.,1.),(1.,1.),(1.,1.),(1.,1.),(1.,
1.),(1.,1.),(1.,1.),(1.,1.),(1.,1.),(1.,1.),(1.,1.),(1.,1.),(1.,1.),(1.,
1.),(1.,1.),(1.,1.),(1.,1.),(1.,1.),(1.,1.),(1.,1.),(1.,1.),(1.,1.),(1.,
1.),(1.,1.),(1.,1.),(1.,1.),(1.,1.),(1.,1.),(1.,1.),(1.,1.),(1.,1.),(1.,
1.),(1.,1.)))
REPRESENTATION_ITEM('')
SURFACE()
);
#60=(
BOUNDED_SURFACE()
B_SPLINE_SURFACE(5,1,((#37986,#37987),(#37988,#37989),(#37990,#37991),(#37992,
#37993),(#37994,#37995),(#37996,#37997),(#37998,#37999),(#38000,#38001),
(#38002,#38003),(#38004,#38005),(#38006,#38007),(#38008,#38009),(#38010,
#38011),(#38012,#38013),(#38014,#38015),(#38016,#38017),(#38018,#38019),
(#38020,#38021),(#38022,#38023),(#38024,#38025),(#38026,#38027),(#38028,
#38029),(#38030,#38031),(#38032,#38033),(#38034,#38035),(#38036,#38037),
(#38038,#38039),(#38040,#38041),(#38042,#38043),(#38044,#38045),(#38046,
#38047),(#38048,#38049),(#38050,#38051),(#38052,#38053),(#38054,#38055),
(#38056,#38057),(#38058,#38059),(#38060,#38061),(#38062,#38063),(#38064,
#38065),(#38066,#38067),(#38068,#38069),(#38070,#38071),(#38072,#38073),
(#38074,#38075),(#38076,#38077),(#38078,#38079),(#38080,#38081),(#38082,
#38083),(#38084,#38085),(#38086,#38087),(#38088,#38089),(#38090,#38091),
(#38092,#38093),(#38094,#38095),(#38096,#38097),(#38098,#38099),(#38100,
#38101),(#38102,#38103),(#38104,#38105),(#38106,#38107),(#38108,#38109),
(#38110,#38111),(#38112,#38113),(#38114,#38115),(#38116,#38117),(#38118,
#38119),(#38120,#38121),(#38122,#38123),(#38124,#38125)),.UNSPECIFIED.,
 .F.,.F.,.F.)
B_SPLINE_SURFACE_WITH_KNOTS((6,1,1,1,1,1,1,1,1,1,1,1,1,1,1,1,1,1,1,1,1,
1,1,1,1,1,1,1,1,1,1,1,1,1,1,1,1,1,1,1,1,1,1,1,1,1,1,1,1,1,1,1,1,1,1,1,1,
1,1,1,1,1,1,1,1,6),(2,2),(-1.,-0.984615384615383,-0.969230769230768,-0.953846153846152,
-0.938461538461537,-0.923076923076922,-0.907692307692306,-0.892307692307691,
-0.876923076923076,-0.86153846153846,-0.846153846153845,-0.83076923076923,
-0.815384615384614,-0.799999999999999,-0.784615384615384,-0.769230769230768,
-0.753846153846153,-0.738461538461538,-0.723076923076922,-0.707692307692307,
-0.692307692307692,-0.676923076923076,-0.661538461538461,-0.646153846153846,
-0.63076923076923,-0.615384615384615,-0.6,-0.584615384615384,-0.569230769230769,
-0.553846153846154,-0.538461538461538,-0.523076923076923,-0.507692307692308,
-0.492307692307692,-0.476923076923077,-0.461538461538462,-0.446153846153846,
-0.430769230769231,-0.415384615384615,-0.4,-0.384615384615385,-0.369230769230769,
-0.353846153846154,-0.338461538461538,-0.323076923076923,-0.307692307692308,
-0.292307692307692,-0.276923076923077,-0.261538461538462,-0.246153846153846,
-0.230769230769231,-0.215384615384615,-0.2,-0.184615384615385,-0.169230769230769,
-0.153846153846154,-0.138461538461538,-0.123076923076923,-0.107692307692308,
-0.0923076923076923,-0.0769230769230769,-0.0615384615384615,-0.0461538461538462,
-0.0307692307692308,-0.0153846153846154,0.),(-1.,1.),.UNSPECIFIED.)
GEOMETRIC_REPRESENTATION_ITEM()
RATIONAL_B_SPLINE_SURFACE(((1.,1.),(1.,1.),(1.,1.),(1.,1.),(1.,1.),(1.,
1.),(1.,1.),(1.,1.),(1.,1.),(1.,1.),(1.,1.),(1.,1.),(1.,1.),(1.,1.),(1.,
1.),(1.,1.),(1.,1.),(1.,1.),(1.,1.),(1.,1.),(1.,1.),(1.,1.),(1.,1.),(1.,
1.),(1.,1.),(1.,1.),(1.,1.),(1.,1.),(1.,1.),(1.,1.),(1.,1.),(1.,1.),(1.,
1.),(1.,1.),(1.,1.),(1.,1.),(1.,1.),(1.,1.),(1.,1.),(1.,1.),(1.,1.),(1.,
1.),(1.,1.),(1.,1.),(1.,1.),(1.,1.),(1.,1.),(1.,1.),(1.,1.),(1.,1.),(1.,
1.),(1.,1.),(1.,1.),(1.,1.),(1.,1.),(1.,1.),(1.,1.),(1.,1.),(1.,1.),(1.,
1.),(1.,1.),(1.,1.),(1.,1.),(1.,1.),(1.,1.),(1.,1.),(1.,1.),(1.,1.),(1.,
1.),(1.,1.)))
REPRESENTATION_ITEM('')
SURFACE()
);
#61=(
BOUNDED_SURFACE()
B_SPLINE_SURFACE(5,1,((#38216,#38217),(#38218,#38219),(#38220,#38221),(#38222,
#38223),(#38224,#38225),(#38226,#38227),(#38228,#38229),(#38230,#38231),
(#38232,#38233),(#38234,#38235),(#38236,#38237),(#38238,#38239),(#38240,
#38241),(#38242,#38243),(#38244,#38245),(#38246,#38247),(#38248,#38249),
(#38250,#38251),(#38252,#38253),(#38254,#38255),(#38256,#38257),(#38258,
#38259),(#38260,#38261),(#38262,#38263),(#38264,#38265),(#38266,#38267),
(#38268,#38269),(#38270,#38271),(#38272,#38273),(#38274,#38275),(#38276,
#38277),(#38278,#38279),(#38280,#38281),(#38282,#38283),(#38284,#38285),
(#38286,#38287),(#38288,#38289),(#38290,#38291),(#38292,#38293),(#38294,
#38295),(#38296,#38297),(#38298,#38299),(#38300,#38301),(#38302,#38303),
(#38304,#38305),(#38306,#38307),(#38308,#38309),(#38310,#38311),(#38312,
#38313),(#38314,#38315),(#38316,#38317),(#38318,#38319),(#38320,#38321),
(#38322,#38323),(#38324,#38325),(#38326,#38327),(#38328,#38329),(#38330,
#38331),(#38332,#38333),(#38334,#38335),(#38336,#38337),(#38338,#38339),
(#38340,#38341),(#38342,#38343),(#38344,#38345),(#38346,#38347),(#38348,
#38349),(#38350,#38351),(#38352,#38353),(#38354,#38355)),.UNSPECIFIED.,
 .F.,.F.,.F.)
B_SPLINE_SURFACE_WITH_KNOTS((6,1,1,1,1,1,1,1,1,1,1,1,1,1,1,1,1,1,1,1,1,
1,1,1,1,1,1,1,1,1,1,1,1,1,1,1,1,1,1,1,1,1,1,1,1,1,1,1,1,1,1,1,1,1,1,1,1,
1,1,1,1,1,1,1,1,6),(2,2),(-1.,-0.984615384615383,-0.969230769230768,-0.953846153846152,
-0.938461538461537,-0.923076923076922,-0.907692307692306,-0.892307692307691,
-0.876923076923076,-0.86153846153846,-0.846153846153845,-0.83076923076923,
-0.815384615384614,-0.799999999999999,-0.784615384615384,-0.769230769230768,
-0.753846153846153,-0.738461538461538,-0.723076923076922,-0.707692307692307,
-0.692307692307692,-0.676923076923076,-0.661538461538461,-0.646153846153846,
-0.63076923076923,-0.615384615384615,-0.6,-0.584615384615384,-0.569230769230769,
-0.553846153846154,-0.538461538461538,-0.523076923076923,-0.507692307692308,
-0.492307692307692,-0.476923076923077,-0.461538461538462,-0.446153846153846,
-0.430769230769231,-0.415384615384615,-0.4,-0.384615384615385,-0.369230769230769,
-0.353846153846154,-0.338461538461538,-0.323076923076923,-0.307692307692308,
-0.292307692307692,-0.276923076923077,-0.261538461538462,-0.246153846153846,
-0.230769230769231,-0.215384615384615,-0.2,-0.184615384615385,-0.169230769230769,
-0.153846153846154,-0.138461538461538,-0.123076923076923,-0.107692307692308,
-0.0923076923076923,-0.0769230769230769,-0.0615384615384615,-0.0461538461538462,
-0.0307692307692308,-0.0153846153846154,0.),(-1.,1.),.UNSPECIFIED.)
GEOMETRIC_REPRESENTATION_ITEM()
RATIONAL_B_SPLINE_SURFACE(((1.,1.),(1.,1.),(1.,1.),(1.,1.),(1.,1.),(1.,
1.),(1.,1.),(1.,1.),(1.,1.),(1.,1.),(1.,1.),(1.,1.),(1.,1.),(1.,1.),(1.,
1.),(1.,1.),(1.,1.),(1.,1.),(1.,1.),(1.,1.),(1.,1.),(1.,1.),(1.,1.),(1.,
1.),(1.,1.),(1.,1.),(1.,1.),(1.,1.),(1.,1.),(1.,1.),(1.,1.),(1.,1.),(1.,
1.),(1.,1.),(1.,1.),(1.,1.),(1.,1.),(1.,1.),(1.,1.),(1.,1.),(1.,1.),(1.,
1.),(1.,1.),(1.,1.),(1.,1.),(1.,1.),(1.,1.),(1.,1.),(1.,1.),(1.,1.),(1.,
1.),(1.,1.),(1.,1.),(1.,1.),(1.,1.),(1.,1.),(1.,1.),(1.,1.),(1.,1.),(1.,
1.),(1.,1.),(1.,1.),(1.,1.),(1.,1.),(1.,1.),(1.,1.),(1.,1.),(1.,1.),(1.,
1.),(1.,1.)))
REPRESENTATION_ITEM('')
SURFACE()
);
#62=(
BOUNDED_SURFACE()
B_SPLINE_SURFACE(5,1,((#38428,#38429),(#38430,#38431),(#38432,#38433),(#38434,
#38435),(#38436,#38437),(#38438,#38439),(#38440,#38441),(#38442,#38443),
(#38444,#38445),(#38446,#38447),(#38448,#38449),(#38450,#38451),(#38452,
#38453),(#38454,#38455),(#38456,#38457),(#38458,#38459),(#38460,#38461),
(#38462,#38463),(#38464,#38465),(#38466,#38467),(#38468,#38469),(#38470,
#38471),(#38472,#38473),(#38474,#38475),(#38476,#38477),(#38478,#38479),
(#38480,#38481),(#38482,#38483),(#38484,#38485),(#38486,#38487),(#38488,
#38489),(#38490,#38491),(#38492,#38493),(#38494,#38495),(#38496,#38497),
(#38498,#38499),(#38500,#38501),(#38502,#38503),(#38504,#38505),(#38506,
#38507),(#38508,#38509),(#38510,#38511),(#38512,#38513),(#38514,#38515),
(#38516,#38517),(#38518,#38519),(#38520,#38521),(#38522,#38523),(#38524,
#38525),(#38526,#38527),(#38528,#38529),(#38530,#38531),(#38532,#38533),
(#38534,#38535),(#38536,#38537),(#38538,#38539),(#38540,#38541),(#38542,
#38543),(#38544,#38545),(#38546,#38547),(#38548,#38549),(#38550,#38551),
(#38552,#38553),(#38554,#38555),(#38556,#38557),(#38558,#38559),(#38560,
#38561),(#38562,#38563),(#38564,#38565),(#38566,#38567)),.UNSPECIFIED.,
 .F.,.F.,.F.)
B_SPLINE_SURFACE_WITH_KNOTS((6,1,1,1,1,1,1,1,1,1,1,1,1,1,1,1,1,1,1,1,1,
1,1,1,1,1,1,1,1,1,1,1,1,1,1,1,1,1,1,1,1,1,1,1,1,1,1,1,1,1,1,1,1,1,1,1,1,
1,1,1,1,1,1,1,1,6),(2,2),(-1.,-0.984615384615383,-0.969230769230768,-0.953846153846152,
-0.938461538461537,-0.923076923076922,-0.907692307692306,-0.892307692307691,
-0.876923076923076,-0.86153846153846,-0.846153846153845,-0.83076923076923,
-0.815384615384614,-0.799999999999999,-0.784615384615384,-0.769230769230768,
-0.753846153846153,-0.738461538461538,-0.723076923076922,-0.707692307692307,
-0.692307692307692,-0.676923076923076,-0.661538461538461,-0.646153846153846,
-0.63076923076923,-0.615384615384615,-0.6,-0.584615384615384,-0.569230769230769,
-0.553846153846154,-0.538461538461538,-0.523076923076923,-0.507692307692308,
-0.492307692307692,-0.476923076923077,-0.461538461538462,-0.446153846153846,
-0.430769230769231,-0.415384615384615,-0.4,-0.384615384615385,-0.369230769230769,
-0.353846153846154,-0.338461538461538,-0.323076923076923,-0.307692307692308,
-0.292307692307692,-0.276923076923077,-0.261538461538462,-0.246153846153846,
-0.230769230769231,-0.215384615384615,-0.2,-0.184615384615385,-0.169230769230769,
-0.153846153846154,-0.138461538461538,-0.123076923076923,-0.107692307692308,
-0.0923076923076923,-0.0769230769230769,-0.0615384615384615,-0.0461538461538462,
-0.0307692307692308,-0.0153846153846154,0.),(-1.,1.),.UNSPECIFIED.)
GEOMETRIC_REPRESENTATION_ITEM()
RATIONAL_B_SPLINE_SURFACE(((1.,1.),(1.,1.),(1.,1.),(1.,1.),(1.,1.),(1.,
1.),(1.,1.),(1.,1.),(1.,1.),(1.,1.),(1.,1.),(1.,1.),(1.,1.),(1.,1.),(1.,
1.),(1.,1.),(1.,1.),(1.,1.),(1.,1.),(1.,1.),(1.,1.),(1.,1.),(1.,1.),(1.,
1.),(1.,1.),(1.,1.),(1.,1.),(1.,1.),(1.,1.),(1.,1.),(1.,1.),(1.,1.),(1.,
1.),(1.,1.),(1.,1.),(1.,1.),(1.,1.),(1.,1.),(1.,1.),(1.,1.),(1.,1.),(1.,
1.),(1.,1.),(1.,1.),(1.,1.),(1.,1.),(1.,1.),(1.,1.),(1.,1.),(1.,1.),(1.,
1.),(1.,1.),(1.,1.),(1.,1.),(1.,1.),(1.,1.),(1.,1.),(1.,1.),(1.,1.),(1.,
1.),(1.,1.),(1.,1.),(1.,1.),(1.,1.),(1.,1.),(1.,1.),(1.,1.),(1.,1.),(1.,
1.),(1.,1.)))
REPRESENTATION_ITEM('')
SURFACE()
);
#63=(
BOUNDED_SURFACE()
B_SPLINE_SURFACE(5,1,((#38658,#38659),(#38660,#38661),(#38662,#38663),(#38664,
#38665),(#38666,#38667),(#38668,#38669),(#38670,#38671),(#38672,#38673),
(#38674,#38675),(#38676,#38677),(#38678,#38679),(#38680,#38681),(#38682,
#38683),(#38684,#38685),(#38686,#38687),(#38688,#38689),(#38690,#38691),
(#38692,#38693),(#38694,#38695),(#38696,#38697),(#38698,#38699),(#38700,
#38701),(#38702,#38703),(#38704,#38705),(#38706,#38707),(#38708,#38709),
(#38710,#38711),(#38712,#38713),(#38714,#38715),(#38716,#38717),(#38718,
#38719),(#38720,#38721),(#38722,#38723),(#38724,#38725),(#38726,#38727),
(#38728,#38729),(#38730,#38731),(#38732,#38733),(#38734,#38735),(#38736,
#38737),(#38738,#38739),(#38740,#38741),(#38742,#38743),(#38744,#38745),
(#38746,#38747),(#38748,#38749),(#38750,#38751),(#38752,#38753),(#38754,
#38755),(#38756,#38757),(#38758,#38759),(#38760,#38761),(#38762,#38763),
(#38764,#38765),(#38766,#38767),(#38768,#38769),(#38770,#38771),(#38772,
#38773),(#38774,#38775),(#38776,#38777),(#38778,#38779),(#38780,#38781),
(#38782,#38783),(#38784,#38785),(#38786,#38787),(#38788,#38789),(#38790,
#38791),(#38792,#38793),(#38794,#38795),(#38796,#38797)),.UNSPECIFIED.,
 .F.,.F.,.F.)
B_SPLINE_SURFACE_WITH_KNOTS((6,1,1,1,1,1,1,1,1,1,1,1,1,1,1,1,1,1,1,1,1,
1,1,1,1,1,1,1,1,1,1,1,1,1,1,1,1,1,1,1,1,1,1,1,1,1,1,1,1,1,1,1,1,1,1,1,1,
1,1,1,1,1,1,1,1,6),(2,2),(-1.,-0.984615384615383,-0.969230769230768,-0.953846153846152,
-0.938461538461537,-0.923076923076922,-0.907692307692306,-0.892307692307691,
-0.876923076923076,-0.86153846153846,-0.846153846153845,-0.83076923076923,
-0.815384615384614,-0.799999999999999,-0.784615384615384,-0.769230769230768,
-0.753846153846153,-0.738461538461538,-0.723076923076922,-0.707692307692307,
-0.692307692307692,-0.676923076923076,-0.661538461538461,-0.646153846153846,
-0.63076923076923,-0.615384615384615,-0.6,-0.584615384615384,-0.569230769230769,
-0.553846153846154,-0.538461538461538,-0.523076923076923,-0.507692307692308,
-0.492307692307692,-0.476923076923077,-0.461538461538462,-0.446153846153846,
-0.430769230769231,-0.415384615384615,-0.4,-0.384615384615385,-0.369230769230769,
-0.353846153846154,-0.338461538461538,-0.323076923076923,-0.307692307692308,
-0.292307692307692,-0.276923076923077,-0.261538461538462,-0.246153846153846,
-0.230769230769231,-0.215384615384615,-0.2,-0.184615384615385,-0.169230769230769,
-0.153846153846154,-0.138461538461538,-0.123076923076923,-0.107692307692308,
-0.0923076923076923,-0.0769230769230769,-0.0615384615384615,-0.0461538461538462,
-0.0307692307692308,-0.0153846153846154,0.),(-1.,1.),.UNSPECIFIED.)
GEOMETRIC_REPRESENTATION_ITEM()
RATIONAL_B_SPLINE_SURFACE(((1.,1.),(1.,1.),(1.,1.),(1.,1.),(1.,1.),(1.,
1.),(1.,1.),(1.,1.),(1.,1.),(1.,1.),(1.,1.),(1.,1.),(1.,1.),(1.,1.),(1.,
1.),(1.,1.),(1.,1.),(1.,1.),(1.,1.),(1.,1.),(1.,1.),(1.,1.),(1.,1.),(1.,
1.),(1.,1.),(1.,1.),(1.,1.),(1.,1.),(1.,1.),(1.,1.),(1.,1.),(1.,1.),(1.,
1.),(1.,1.),(1.,1.),(1.,1.),(1.,1.),(1.,1.),(1.,1.),(1.,1.),(1.,1.),(1.,
1.),(1.,1.),(1.,1.),(1.,1.),(1.,1.),(1.,1.),(1.,1.),(1.,1.),(1.,1.),(1.,
1.),(1.,1.),(1.,1.),(1.,1.),(1.,1.),(1.,1.),(1.,1.),(1.,1.),(1.,1.),(1.,
1.),(1.,1.),(1.,1.),(1.,1.),(1.,1.),(1.,1.),(1.,1.),(1.,1.),(1.,1.),(1.,
1.),(1.,1.)))
REPRESENTATION_ITEM('')
SURFACE()
);
#64=(
BOUNDED_SURFACE()
B_SPLINE_SURFACE(5,1,((#38870,#38871),(#38872,#38873),(#38874,#38875),(#38876,
#38877),(#38878,#38879),(#38880,#38881),(#38882,#38883),(#38884,#38885),
(#38886,#38887),(#38888,#38889),(#38890,#38891),(#38892,#38893),(#38894,
#38895),(#38896,#38897),(#38898,#38899),(#38900,#38901),(#38902,#38903),
(#38904,#38905),(#38906,#38907),(#38908,#38909),(#38910,#38911),(#38912,
#38913),(#38914,#38915),(#38916,#38917),(#38918,#38919),(#38920,#38921),
(#38922,#38923),(#38924,#38925),(#38926,#38927),(#38928,#38929),(#38930,
#38931),(#38932,#38933),(#38934,#38935),(#38936,#38937),(#38938,#38939),
(#38940,#38941),(#38942,#38943),(#38944,#38945),(#38946,#38947),(#38948,
#38949),(#38950,#38951),(#38952,#38953),(#38954,#38955),(#38956,#38957),
(#38958,#38959),(#38960,#38961),(#38962,#38963),(#38964,#38965),(#38966,
#38967),(#38968,#38969),(#38970,#38971),(#38972,#38973),(#38974,#38975),
(#38976,#38977),(#38978,#38979),(#38980,#38981),(#38982,#38983),(#38984,
#38985),(#38986,#38987),(#38988,#38989),(#38990,#38991),(#38992,#38993),
(#38994,#38995),(#38996,#38997),(#38998,#38999),(#39000,#39001),(#39002,
#39003),(#39004,#39005),(#39006,#39007),(#39008,#39009)),.UNSPECIFIED.,
 .F.,.F.,.F.)
B_SPLINE_SURFACE_WITH_KNOTS((6,1,1,1,1,1,1,1,1,1,1,1,1,1,1,1,1,1,1,1,1,
1,1,1,1,1,1,1,1,1,1,1,1,1,1,1,1,1,1,1,1,1,1,1,1,1,1,1,1,1,1,1,1,1,1,1,1,
1,1,1,1,1,1,1,1,6),(2,2),(-1.,-0.984615384615383,-0.969230769230768,-0.953846153846152,
-0.938461538461537,-0.923076923076922,-0.907692307692306,-0.892307692307691,
-0.876923076923076,-0.86153846153846,-0.846153846153845,-0.83076923076923,
-0.815384615384614,-0.799999999999999,-0.784615384615384,-0.769230769230768,
-0.753846153846153,-0.738461538461538,-0.723076923076922,-0.707692307692307,
-0.692307692307692,-0.676923076923076,-0.661538461538461,-0.646153846153846,
-0.63076923076923,-0.615384615384615,-0.6,-0.584615384615384,-0.569230769230769,
-0.553846153846154,-0.538461538461538,-0.523076923076923,-0.507692307692308,
-0.492307692307692,-0.476923076923077,-0.461538461538462,-0.446153846153846,
-0.430769230769231,-0.415384615384615,-0.4,-0.384615384615385,-0.369230769230769,
-0.353846153846154,-0.338461538461538,-0.323076923076923,-0.307692307692308,
-0.292307692307692,-0.276923076923077,-0.261538461538462,-0.246153846153846,
-0.230769230769231,-0.215384615384615,-0.2,-0.184615384615385,-0.169230769230769,
-0.153846153846154,-0.138461538461538,-0.123076923076923,-0.107692307692308,
-0.0923076923076923,-0.0769230769230769,-0.0615384615384615,-0.0461538461538462,
-0.0307692307692308,-0.0153846153846154,0.),(-1.,1.),.UNSPECIFIED.)
GEOMETRIC_REPRESENTATION_ITEM()
RATIONAL_B_SPLINE_SURFACE(((1.,1.),(1.,1.),(1.,1.),(1.,1.),(1.,1.),(1.,
1.),(1.,1.),(1.,1.),(1.,1.),(1.,1.),(1.,1.),(1.,1.),(1.,1.),(1.,1.),(1.,
1.),(1.,1.),(1.,1.),(1.,1.),(1.,1.),(1.,1.),(1.,1.),(1.,1.),(1.,1.),(1.,
1.),(1.,1.),(1.,1.),(1.,1.),(1.,1.),(1.,1.),(1.,1.),(1.,1.),(1.,1.),(1.,
1.),(1.,1.),(1.,1.),(1.,1.),(1.,1.),(1.,1.),(1.,1.),(1.,1.),(1.,1.),(1.,
1.),(1.,1.),(1.,1.),(1.,1.),(1.,1.),(1.,1.),(1.,1.),(1.,1.),(1.,1.),(1.,
1.),(1.,1.),(1.,1.),(1.,1.),(1.,1.),(1.,1.),(1.,1.),(1.,1.),(1.,1.),(1.,
1.),(1.,1.),(1.,1.),(1.,1.),(1.,1.),(1.,1.),(1.,1.),(1.,1.),(1.,1.),(1.,
1.),(1.,1.)))
REPRESENTATION_ITEM('')
SURFACE()
);
#65=(
BOUNDED_SURFACE()
B_SPLINE_SURFACE(5,1,((#39100,#39101),(#39102,#39103),(#39104,#39105),(#39106,
#39107),(#39108,#39109),(#39110,#39111),(#39112,#39113),(#39114,#39115),
(#39116,#39117),(#39118,#39119),(#39120,#39121),(#39122,#39123),(#39124,
#39125),(#39126,#39127),(#39128,#39129),(#39130,#39131),(#39132,#39133),
(#39134,#39135),(#39136,#39137),(#39138,#39139),(#39140,#39141),(#39142,
#39143),(#39144,#39145),(#39146,#39147),(#39148,#39149),(#39150,#39151),
(#39152,#39153),(#39154,#39155),(#39156,#39157),(#39158,#39159),(#39160,
#39161),(#39162,#39163),(#39164,#39165),(#39166,#39167),(#39168,#39169),
(#39170,#39171),(#39172,#39173),(#39174,#39175),(#39176,#39177),(#39178,
#39179),(#39180,#39181),(#39182,#39183),(#39184,#39185),(#39186,#39187),
(#39188,#39189),(#39190,#39191),(#39192,#39193),(#39194,#39195),(#39196,
#39197),(#39198,#39199),(#39200,#39201),(#39202,#39203),(#39204,#39205),
(#39206,#39207),(#39208,#39209),(#39210,#39211),(#39212,#39213),(#39214,
#39215),(#39216,#39217),(#39218,#39219),(#39220,#39221),(#39222,#39223),
(#39224,#39225),(#39226,#39227),(#39228,#39229),(#39230,#39231),(#39232,
#39233),(#39234,#39235),(#39236,#39237),(#39238,#39239)),.UNSPECIFIED.,
 .F.,.F.,.F.)
B_SPLINE_SURFACE_WITH_KNOTS((6,1,1,1,1,1,1,1,1,1,1,1,1,1,1,1,1,1,1,1,1,
1,1,1,1,1,1,1,1,1,1,1,1,1,1,1,1,1,1,1,1,1,1,1,1,1,1,1,1,1,1,1,1,1,1,1,1,
1,1,1,1,1,1,1,1,6),(2,2),(-1.,-0.984615384615383,-0.969230769230768,-0.953846153846152,
-0.938461538461537,-0.923076923076922,-0.907692307692306,-0.892307692307691,
-0.876923076923076,-0.86153846153846,-0.846153846153845,-0.83076923076923,
-0.815384615384614,-0.799999999999999,-0.784615384615384,-0.769230769230768,
-0.753846153846153,-0.738461538461538,-0.723076923076922,-0.707692307692307,
-0.692307692307692,-0.676923076923076,-0.661538461538461,-0.646153846153846,
-0.63076923076923,-0.615384615384615,-0.6,-0.584615384615384,-0.569230769230769,
-0.553846153846154,-0.538461538461538,-0.523076923076923,-0.507692307692308,
-0.492307692307692,-0.476923076923077,-0.461538461538462,-0.446153846153846,
-0.430769230769231,-0.415384615384615,-0.4,-0.384615384615385,-0.369230769230769,
-0.353846153846154,-0.338461538461538,-0.323076923076923,-0.307692307692308,
-0.292307692307692,-0.276923076923077,-0.261538461538462,-0.246153846153846,
-0.230769230769231,-0.215384615384615,-0.2,-0.184615384615385,-0.169230769230769,
-0.153846153846154,-0.138461538461538,-0.123076923076923,-0.107692307692308,
-0.0923076923076923,-0.0769230769230769,-0.0615384615384615,-0.0461538461538462,
-0.0307692307692308,-0.0153846153846154,0.),(-1.,1.),.UNSPECIFIED.)
GEOMETRIC_REPRESENTATION_ITEM()
RATIONAL_B_SPLINE_SURFACE(((1.,1.),(1.,1.),(1.,1.),(1.,1.),(1.,1.),(1.,
1.),(1.,1.),(1.,1.),(1.,1.),(1.,1.),(1.,1.),(1.,1.),(1.,1.),(1.,1.),(1.,
1.),(1.,1.),(1.,1.),(1.,1.),(1.,1.),(1.,1.),(1.,1.),(1.,1.),(1.,1.),(1.,
1.),(1.,1.),(1.,1.),(1.,1.),(1.,1.),(1.,1.),(1.,1.),(1.,1.),(1.,1.),(1.,
1.),(1.,1.),(1.,1.),(1.,1.),(1.,1.),(1.,1.),(1.,1.),(1.,1.),(1.,1.),(1.,
1.),(1.,1.),(1.,1.),(1.,1.),(1.,1.),(1.,1.),(1.,1.),(1.,1.),(1.,1.),(1.,
1.),(1.,1.),(1.,1.),(1.,1.),(1.,1.),(1.,1.),(1.,1.),(1.,1.),(1.,1.),(1.,
1.),(1.,1.),(1.,1.),(1.,1.),(1.,1.),(1.,1.),(1.,1.),(1.,1.),(1.,1.),(1.,
1.),(1.,1.)))
REPRESENTATION_ITEM('')
SURFACE()
);
#66=(
BOUNDED_SURFACE()
B_SPLINE_SURFACE(5,1,((#39312,#39313),(#39314,#39315),(#39316,#39317),(#39318,
#39319),(#39320,#39321),(#39322,#39323),(#39324,#39325),(#39326,#39327),
(#39328,#39329),(#39330,#39331),(#39332,#39333),(#39334,#39335),(#39336,
#39337),(#39338,#39339),(#39340,#39341),(#39342,#39343),(#39344,#39345),
(#39346,#39347),(#39348,#39349),(#39350,#39351),(#39352,#39353),(#39354,
#39355),(#39356,#39357),(#39358,#39359),(#39360,#39361),(#39362,#39363),
(#39364,#39365),(#39366,#39367),(#39368,#39369),(#39370,#39371),(#39372,
#39373),(#39374,#39375),(#39376,#39377),(#39378,#39379),(#39380,#39381),
(#39382,#39383),(#39384,#39385),(#39386,#39387),(#39388,#39389),(#39390,
#39391),(#39392,#39393),(#39394,#39395),(#39396,#39397),(#39398,#39399),
(#39400,#39401),(#39402,#39403),(#39404,#39405),(#39406,#39407),(#39408,
#39409),(#39410,#39411),(#39412,#39413),(#39414,#39415),(#39416,#39417),
(#39418,#39419),(#39420,#39421),(#39422,#39423),(#39424,#39425),(#39426,
#39427),(#39428,#39429),(#39430,#39431),(#39432,#39433),(#39434,#39435),
(#39436,#39437),(#39438,#39439),(#39440,#39441),(#39442,#39443),(#39444,
#39445),(#39446,#39447),(#39448,#39449),(#39450,#39451)),.UNSPECIFIED.,
 .F.,.F.,.F.)
B_SPLINE_SURFACE_WITH_KNOTS((6,1,1,1,1,1,1,1,1,1,1,1,1,1,1,1,1,1,1,1,1,
1,1,1,1,1,1,1,1,1,1,1,1,1,1,1,1,1,1,1,1,1,1,1,1,1,1,1,1,1,1,1,1,1,1,1,1,
1,1,1,1,1,1,1,1,6),(2,2),(-1.,-0.984615384615383,-0.969230769230768,-0.953846153846152,
-0.938461538461537,-0.923076923076922,-0.907692307692306,-0.892307692307691,
-0.876923076923076,-0.86153846153846,-0.846153846153845,-0.83076923076923,
-0.815384615384614,-0.799999999999999,-0.784615384615384,-0.769230769230768,
-0.753846153846153,-0.738461538461538,-0.723076923076922,-0.707692307692307,
-0.692307692307692,-0.676923076923076,-0.661538461538461,-0.646153846153846,
-0.63076923076923,-0.615384615384615,-0.6,-0.584615384615384,-0.569230769230769,
-0.553846153846154,-0.538461538461538,-0.523076923076923,-0.507692307692308,
-0.492307692307692,-0.476923076923077,-0.461538461538462,-0.446153846153846,
-0.430769230769231,-0.415384615384615,-0.4,-0.384615384615385,-0.369230769230769,
-0.353846153846154,-0.338461538461538,-0.323076923076923,-0.307692307692308,
-0.292307692307692,-0.276923076923077,-0.261538461538462,-0.246153846153846,
-0.230769230769231,-0.215384615384615,-0.2,-0.184615384615385,-0.169230769230769,
-0.153846153846154,-0.138461538461538,-0.123076923076923,-0.107692307692308,
-0.0923076923076923,-0.0769230769230769,-0.0615384615384615,-0.0461538461538462,
-0.0307692307692308,-0.0153846153846154,0.),(-1.,1.),.UNSPECIFIED.)
GEOMETRIC_REPRESENTATION_ITEM()
RATIONAL_B_SPLINE_SURFACE(((1.,1.),(1.,1.),(1.,1.),(1.,1.),(1.,1.),(1.,
1.),(1.,1.),(1.,1.),(1.,1.),(1.,1.),(1.,1.),(1.,1.),(1.,1.),(1.,1.),(1.,
1.),(1.,1.),(1.,1.),(1.,1.),(1.,1.),(1.,1.),(1.,1.),(1.,1.),(1.,1.),(1.,
1.),(1.,1.),(1.,1.),(1.,1.),(1.,1.),(1.,1.),(1.,1.),(1.,1.),(1.,1.),(1.,
1.),(1.,1.),(1.,1.),(1.,1.),(1.,1.),(1.,1.),(1.,1.),(1.,1.),(1.,1.),(1.,
1.),(1.,1.),(1.,1.),(1.,1.),(1.,1.),(1.,1.),(1.,1.),(1.,1.),(1.,1.),(1.,
1.),(1.,1.),(1.,1.),(1.,1.),(1.,1.),(1.,1.),(1.,1.),(1.,1.),(1.,1.),(1.,
1.),(1.,1.),(1.,1.),(1.,1.),(1.,1.),(1.,1.),(1.,1.),(1.,1.),(1.,1.),(1.,
1.),(1.,1.)))
REPRESENTATION_ITEM('')
SURFACE()
);
#67=(
BOUNDED_SURFACE()
B_SPLINE_SURFACE(5,1,((#39542,#39543),(#39544,#39545),(#39546,#39547),(#39548,
#39549),(#39550,#39551),(#39552,#39553),(#39554,#39555),(#39556,#39557),
(#39558,#39559),(#39560,#39561),(#39562,#39563),(#39564,#39565),(#39566,
#39567),(#39568,#39569),(#39570,#39571),(#39572,#39573),(#39574,#39575),
(#39576,#39577),(#39578,#39579),(#39580,#39581),(#39582,#39583),(#39584,
#39585),(#39586,#39587),(#39588,#39589),(#39590,#39591),(#39592,#39593),
(#39594,#39595),(#39596,#39597),(#39598,#39599),(#39600,#39601),(#39602,
#39603),(#39604,#39605),(#39606,#39607),(#39608,#39609),(#39610,#39611),
(#39612,#39613),(#39614,#39615),(#39616,#39617),(#39618,#39619),(#39620,
#39621),(#39622,#39623),(#39624,#39625),(#39626,#39627),(#39628,#39629),
(#39630,#39631),(#39632,#39633),(#39634,#39635),(#39636,#39637),(#39638,
#39639),(#39640,#39641),(#39642,#39643),(#39644,#39645),(#39646,#39647),
(#39648,#39649),(#39650,#39651),(#39652,#39653),(#39654,#39655),(#39656,
#39657),(#39658,#39659),(#39660,#39661),(#39662,#39663),(#39664,#39665),
(#39666,#39667),(#39668,#39669),(#39670,#39671),(#39672,#39673),(#39674,
#39675),(#39676,#39677),(#39678,#39679),(#39680,#39681)),.UNSPECIFIED.,
 .F.,.F.,.F.)
B_SPLINE_SURFACE_WITH_KNOTS((6,1,1,1,1,1,1,1,1,1,1,1,1,1,1,1,1,1,1,1,1,
1,1,1,1,1,1,1,1,1,1,1,1,1,1,1,1,1,1,1,1,1,1,1,1,1,1,1,1,1,1,1,1,1,1,1,1,
1,1,1,1,1,1,1,1,6),(2,2),(-1.,-0.984615384615383,-0.969230769230768,-0.953846153846152,
-0.938461538461537,-0.923076923076922,-0.907692307692306,-0.892307692307691,
-0.876923076923076,-0.86153846153846,-0.846153846153845,-0.83076923076923,
-0.815384615384614,-0.799999999999999,-0.784615384615384,-0.769230769230768,
-0.753846153846153,-0.738461538461538,-0.723076923076922,-0.707692307692307,
-0.692307692307692,-0.676923076923076,-0.661538461538461,-0.646153846153846,
-0.63076923076923,-0.615384615384615,-0.6,-0.584615384615384,-0.569230769230769,
-0.553846153846154,-0.538461538461538,-0.523076923076923,-0.507692307692308,
-0.492307692307692,-0.476923076923077,-0.461538461538462,-0.446153846153846,
-0.430769230769231,-0.415384615384615,-0.4,-0.384615384615385,-0.369230769230769,
-0.353846153846154,-0.338461538461538,-0.323076923076923,-0.307692307692308,
-0.292307692307692,-0.276923076923077,-0.261538461538462,-0.246153846153846,
-0.230769230769231,-0.215384615384615,-0.2,-0.184615384615385,-0.169230769230769,
-0.153846153846154,-0.138461538461538,-0.123076923076923,-0.107692307692308,
-0.0923076923076923,-0.0769230769230769,-0.0615384615384615,-0.0461538461538462,
-0.0307692307692308,-0.0153846153846154,0.),(-1.,1.),.UNSPECIFIED.)
GEOMETRIC_REPRESENTATION_ITEM()
RATIONAL_B_SPLINE_SURFACE(((1.,1.),(1.,1.),(1.,1.),(1.,1.),(1.,1.),(1.,
1.),(1.,1.),(1.,1.),(1.,1.),(1.,1.),(1.,1.),(1.,1.),(1.,1.),(1.,1.),(1.,
1.),(1.,1.),(1.,1.),(1.,1.),(1.,1.),(1.,1.),(1.,1.),(1.,1.),(1.,1.),(1.,
1.),(1.,1.),(1.,1.),(1.,1.),(1.,1.),(1.,1.),(1.,1.),(1.,1.),(1.,1.),(1.,
1.),(1.,1.),(1.,1.),(1.,1.),(1.,1.),(1.,1.),(1.,1.),(1.,1.),(1.,1.),(1.,
1.),(1.,1.),(1.,1.),(1.,1.),(1.,1.),(1.,1.),(1.,1.),(1.,1.),(1.,1.),(1.,
1.),(1.,1.),(1.,1.),(1.,1.),(1.,1.),(1.,1.),(1.,1.),(1.,1.),(1.,1.),(1.,
1.),(1.,1.),(1.,1.),(1.,1.),(1.,1.),(1.,1.),(1.,1.),(1.,1.),(1.,1.),(1.,
1.),(1.,1.)))
REPRESENTATION_ITEM('')
SURFACE()
);
#68=(
BOUNDED_SURFACE()
B_SPLINE_SURFACE(5,1,((#39754,#39755),(#39756,#39757),(#39758,#39759),(#39760,
#39761),(#39762,#39763),(#39764,#39765),(#39766,#39767),(#39768,#39769),
(#39770,#39771),(#39772,#39773),(#39774,#39775),(#39776,#39777),(#39778,
#39779),(#39780,#39781),(#39782,#39783),(#39784,#39785),(#39786,#39787),
(#39788,#39789),(#39790,#39791),(#39792,#39793),(#39794,#39795),(#39796,
#39797),(#39798,#39799),(#39800,#39801),(#39802,#39803),(#39804,#39805),
(#39806,#39807),(#39808,#39809),(#39810,#39811),(#39812,#39813),(#39814,
#39815),(#39816,#39817),(#39818,#39819),(#39820,#39821),(#39822,#39823),
(#39824,#39825),(#39826,#39827),(#39828,#39829),(#39830,#39831),(#39832,
#39833),(#39834,#39835),(#39836,#39837),(#39838,#39839),(#39840,#39841),
(#39842,#39843),(#39844,#39845),(#39846,#39847),(#39848,#39849),(#39850,
#39851),(#39852,#39853),(#39854,#39855),(#39856,#39857),(#39858,#39859),
(#39860,#39861),(#39862,#39863),(#39864,#39865),(#39866,#39867),(#39868,
#39869),(#39870,#39871),(#39872,#39873),(#39874,#39875),(#39876,#39877),
(#39878,#39879),(#39880,#39881),(#39882,#39883),(#39884,#39885),(#39886,
#39887),(#39888,#39889),(#39890,#39891),(#39892,#39893)),.UNSPECIFIED.,
 .F.,.F.,.F.)
B_SPLINE_SURFACE_WITH_KNOTS((6,1,1,1,1,1,1,1,1,1,1,1,1,1,1,1,1,1,1,1,1,
1,1,1,1,1,1,1,1,1,1,1,1,1,1,1,1,1,1,1,1,1,1,1,1,1,1,1,1,1,1,1,1,1,1,1,1,
1,1,1,1,1,1,1,1,6),(2,2),(-1.,-0.984615384615383,-0.969230769230768,-0.953846153846152,
-0.938461538461537,-0.923076923076922,-0.907692307692306,-0.892307692307691,
-0.876923076923076,-0.86153846153846,-0.846153846153845,-0.83076923076923,
-0.815384615384614,-0.799999999999999,-0.784615384615384,-0.769230769230768,
-0.753846153846153,-0.738461538461538,-0.723076923076922,-0.707692307692307,
-0.692307692307692,-0.676923076923076,-0.661538461538461,-0.646153846153846,
-0.63076923076923,-0.615384615384615,-0.6,-0.584615384615384,-0.569230769230769,
-0.553846153846154,-0.538461538461538,-0.523076923076923,-0.507692307692308,
-0.492307692307692,-0.476923076923077,-0.461538461538462,-0.446153846153846,
-0.430769230769231,-0.415384615384615,-0.4,-0.384615384615385,-0.369230769230769,
-0.353846153846154,-0.338461538461538,-0.323076923076923,-0.307692307692308,
-0.292307692307692,-0.276923076923077,-0.261538461538462,-0.246153846153846,
-0.230769230769231,-0.215384615384615,-0.2,-0.184615384615385,-0.169230769230769,
-0.153846153846154,-0.138461538461538,-0.123076923076923,-0.107692307692308,
-0.0923076923076923,-0.0769230769230769,-0.0615384615384615,-0.0461538461538462,
-0.0307692307692308,-0.0153846153846154,0.),(-1.,1.),.UNSPECIFIED.)
GEOMETRIC_REPRESENTATION_ITEM()
RATIONAL_B_SPLINE_SURFACE(((1.,1.),(1.,1.),(1.,1.),(1.,1.),(1.,1.),(1.,
1.),(1.,1.),(1.,1.),(1.,1.),(1.,1.),(1.,1.),(1.,1.),(1.,1.),(1.,1.),(1.,
1.),(1.,1.),(1.,1.),(1.,1.),(1.,1.),(1.,1.),(1.,1.),(1.,1.),(1.,1.),(1.,
1.),(1.,1.),(1.,1.),(1.,1.),(1.,1.),(1.,1.),(1.,1.),(1.,1.),(1.,1.),(1.,
1.),(1.,1.),(1.,1.),(1.,1.),(1.,1.),(1.,1.),(1.,1.),(1.,1.),(1.,1.),(1.,
1.),(1.,1.),(1.,1.),(1.,1.),(1.,1.),(1.,1.),(1.,1.),(1.,1.),(1.,1.),(1.,
1.),(1.,1.),(1.,1.),(1.,1.),(1.,1.),(1.,1.),(1.,1.),(1.,1.),(1.,1.),(1.,
1.),(1.,1.),(1.,1.),(1.,1.),(1.,1.),(1.,1.),(1.,1.),(1.,1.),(1.,1.),(1.,
1.),(1.,1.)))
REPRESENTATION_ITEM('')
SURFACE()
);
#69=(
BOUNDED_SURFACE()
B_SPLINE_SURFACE(5,1,((#39984,#39985),(#39986,#39987),(#39988,#39989),(#39990,
#39991),(#39992,#39993),(#39994,#39995),(#39996,#39997),(#39998,#39999),
(#40000,#40001),(#40002,#40003),(#40004,#40005),(#40006,#40007),(#40008,
#40009),(#40010,#40011),(#40012,#40013),(#40014,#40015),(#40016,#40017),
(#40018,#40019),(#40020,#40021),(#40022,#40023),(#40024,#40025),(#40026,
#40027),(#40028,#40029),(#40030,#40031),(#40032,#40033),(#40034,#40035),
(#40036,#40037),(#40038,#40039),(#40040,#40041),(#40042,#40043),(#40044,
#40045),(#40046,#40047),(#40048,#40049),(#40050,#40051),(#40052,#40053),
(#40054,#40055),(#40056,#40057),(#40058,#40059),(#40060,#40061),(#40062,
#40063),(#40064,#40065),(#40066,#40067),(#40068,#40069),(#40070,#40071),
(#40072,#40073),(#40074,#40075),(#40076,#40077),(#40078,#40079),(#40080,
#40081),(#40082,#40083),(#40084,#40085),(#40086,#40087),(#40088,#40089),
(#40090,#40091),(#40092,#40093),(#40094,#40095),(#40096,#40097),(#40098,
#40099),(#40100,#40101),(#40102,#40103),(#40104,#40105),(#40106,#40107),
(#40108,#40109),(#40110,#40111),(#40112,#40113),(#40114,#40115),(#40116,
#40117),(#40118,#40119),(#40120,#40121),(#40122,#40123)),.UNSPECIFIED.,
 .F.,.F.,.F.)
B_SPLINE_SURFACE_WITH_KNOTS((6,1,1,1,1,1,1,1,1,1,1,1,1,1,1,1,1,1,1,1,1,
1,1,1,1,1,1,1,1,1,1,1,1,1,1,1,1,1,1,1,1,1,1,1,1,1,1,1,1,1,1,1,1,1,1,1,1,
1,1,1,1,1,1,1,1,6),(2,2),(-1.,-0.984615384615383,-0.969230769230768,-0.953846153846152,
-0.938461538461537,-0.923076923076922,-0.907692307692306,-0.892307692307691,
-0.876923076923076,-0.86153846153846,-0.846153846153845,-0.83076923076923,
-0.815384615384614,-0.799999999999999,-0.784615384615384,-0.769230769230768,
-0.753846153846153,-0.738461538461538,-0.723076923076922,-0.707692307692307,
-0.692307692307692,-0.676923076923076,-0.661538461538461,-0.646153846153846,
-0.63076923076923,-0.615384615384615,-0.6,-0.584615384615384,-0.569230769230769,
-0.553846153846154,-0.538461538461538,-0.523076923076923,-0.507692307692308,
-0.492307692307692,-0.476923076923077,-0.461538461538462,-0.446153846153846,
-0.430769230769231,-0.415384615384615,-0.4,-0.384615384615385,-0.369230769230769,
-0.353846153846154,-0.338461538461538,-0.323076923076923,-0.307692307692308,
-0.292307692307692,-0.276923076923077,-0.261538461538462,-0.246153846153846,
-0.230769230769231,-0.215384615384615,-0.2,-0.184615384615385,-0.169230769230769,
-0.153846153846154,-0.138461538461538,-0.123076923076923,-0.107692307692308,
-0.0923076923076923,-0.0769230769230769,-0.0615384615384615,-0.0461538461538462,
-0.0307692307692308,-0.0153846153846154,0.),(-1.,1.),.UNSPECIFIED.)
GEOMETRIC_REPRESENTATION_ITEM()
RATIONAL_B_SPLINE_SURFACE(((1.,1.),(1.,1.),(1.,1.),(1.,1.),(1.,1.),(1.,
1.),(1.,1.),(1.,1.),(1.,1.),(1.,1.),(1.,1.),(1.,1.),(1.,1.),(1.,1.),(1.,
1.),(1.,1.),(1.,1.),(1.,1.),(1.,1.),(1.,1.),(1.,1.),(1.,1.),(1.,1.),(1.,
1.),(1.,1.),(1.,1.),(1.,1.),(1.,1.),(1.,1.),(1.,1.),(1.,1.),(1.,1.),(1.,
1.),(1.,1.),(1.,1.),(1.,1.),(1.,1.),(1.,1.),(1.,1.),(1.,1.),(1.,1.),(1.,
1.),(1.,1.),(1.,1.),(1.,1.),(1.,1.),(1.,1.),(1.,1.),(1.,1.),(1.,1.),(1.,
1.),(1.,1.),(1.,1.),(1.,1.),(1.,1.),(1.,1.),(1.,1.),(1.,1.),(1.,1.),(1.,
1.),(1.,1.),(1.,1.),(1.,1.),(1.,1.),(1.,1.),(1.,1.),(1.,1.),(1.,1.),(1.,
1.),(1.,1.)))
REPRESENTATION_ITEM('')
SURFACE()
);
#70=(
BOUNDED_SURFACE()
B_SPLINE_SURFACE(5,1,((#40196,#40197),(#40198,#40199),(#40200,#40201),(#40202,
#40203),(#40204,#40205),(#40206,#40207),(#40208,#40209),(#40210,#40211),
(#40212,#40213),(#40214,#40215),(#40216,#40217),(#40218,#40219),(#40220,
#40221),(#40222,#40223),(#40224,#40225),(#40226,#40227),(#40228,#40229),
(#40230,#40231),(#40232,#40233),(#40234,#40235),(#40236,#40237),(#40238,
#40239),(#40240,#40241),(#40242,#40243),(#40244,#40245),(#40246,#40247),
(#40248,#40249),(#40250,#40251),(#40252,#40253),(#40254,#40255),(#40256,
#40257),(#40258,#40259),(#40260,#40261),(#40262,#40263),(#40264,#40265),
(#40266,#40267),(#40268,#40269),(#40270,#40271),(#40272,#40273),(#40274,
#40275),(#40276,#40277),(#40278,#40279),(#40280,#40281),(#40282,#40283),
(#40284,#40285),(#40286,#40287),(#40288,#40289),(#40290,#40291),(#40292,
#40293),(#40294,#40295),(#40296,#40297),(#40298,#40299),(#40300,#40301),
(#40302,#40303),(#40304,#40305),(#40306,#40307),(#40308,#40309),(#40310,
#40311),(#40312,#40313),(#40314,#40315),(#40316,#40317),(#40318,#40319),
(#40320,#40321),(#40322,#40323),(#40324,#40325),(#40326,#40327),(#40328,
#40329),(#40330,#40331),(#40332,#40333),(#40334,#40335)),.UNSPECIFIED.,
 .F.,.F.,.F.)
B_SPLINE_SURFACE_WITH_KNOTS((6,1,1,1,1,1,1,1,1,1,1,1,1,1,1,1,1,1,1,1,1,
1,1,1,1,1,1,1,1,1,1,1,1,1,1,1,1,1,1,1,1,1,1,1,1,1,1,1,1,1,1,1,1,1,1,1,1,
1,1,1,1,1,1,1,1,6),(2,2),(-1.,-0.984615384615383,-0.969230769230768,-0.953846153846152,
-0.938461538461537,-0.923076923076922,-0.907692307692306,-0.892307692307691,
-0.876923076923076,-0.86153846153846,-0.846153846153845,-0.83076923076923,
-0.815384615384614,-0.799999999999999,-0.784615384615384,-0.769230769230768,
-0.753846153846153,-0.738461538461538,-0.723076923076922,-0.707692307692307,
-0.692307692307692,-0.676923076923076,-0.661538461538461,-0.646153846153846,
-0.63076923076923,-0.615384615384615,-0.6,-0.584615384615384,-0.569230769230769,
-0.553846153846154,-0.538461538461538,-0.523076923076923,-0.507692307692308,
-0.492307692307692,-0.476923076923077,-0.461538461538462,-0.446153846153846,
-0.430769230769231,-0.415384615384615,-0.4,-0.384615384615385,-0.369230769230769,
-0.353846153846154,-0.338461538461538,-0.323076923076923,-0.307692307692308,
-0.292307692307692,-0.276923076923077,-0.261538461538462,-0.246153846153846,
-0.230769230769231,-0.215384615384615,-0.2,-0.184615384615385,-0.169230769230769,
-0.153846153846154,-0.138461538461538,-0.123076923076923,-0.107692307692308,
-0.0923076923076923,-0.0769230769230769,-0.0615384615384615,-0.0461538461538462,
-0.0307692307692308,-0.0153846153846154,0.),(-1.,1.),.UNSPECIFIED.)
GEOMETRIC_REPRESENTATION_ITEM()
RATIONAL_B_SPLINE_SURFACE(((1.,1.),(1.,1.),(1.,1.),(1.,1.),(1.,1.),(1.,
1.),(1.,1.),(1.,1.),(1.,1.),(1.,1.),(1.,1.),(1.,1.),(1.,1.),(1.,1.),(1.,
1.),(1.,1.),(1.,1.),(1.,1.),(1.,1.),(1.,1.),(1.,1.),(1.,1.),(1.,1.),(1.,
1.),(1.,1.),(1.,1.),(1.,1.),(1.,1.),(1.,1.),(1.,1.),(1.,1.),(1.,1.),(1.,
1.),(1.,1.),(1.,1.),(1.,1.),(1.,1.),(1.,1.),(1.,1.),(1.,1.),(1.,1.),(1.,
1.),(1.,1.),(1.,1.),(1.,1.),(1.,1.),(1.,1.),(1.,1.),(1.,1.),(1.,1.),(1.,
1.),(1.,1.),(1.,1.),(1.,1.),(1.,1.),(1.,1.),(1.,1.),(1.,1.),(1.,1.),(1.,
1.),(1.,1.),(1.,1.),(1.,1.),(1.,1.),(1.,1.),(1.,1.),(1.,1.),(1.,1.),(1.,
1.),(1.,1.)))
REPRESENTATION_ITEM('')
SURFACE()
);
#71=(
BOUNDED_SURFACE()
B_SPLINE_SURFACE(5,1,((#40426,#40427),(#40428,#40429),(#40430,#40431),(#40432,
#40433),(#40434,#40435),(#40436,#40437),(#40438,#40439),(#40440,#40441),
(#40442,#40443),(#40444,#40445),(#40446,#40447),(#40448,#40449),(#40450,
#40451),(#40452,#40453),(#40454,#40455),(#40456,#40457),(#40458,#40459),
(#40460,#40461),(#40462,#40463),(#40464,#40465),(#40466,#40467),(#40468,
#40469),(#40470,#40471),(#40472,#40473),(#40474,#40475),(#40476,#40477),
(#40478,#40479),(#40480,#40481),(#40482,#40483),(#40484,#40485),(#40486,
#40487),(#40488,#40489),(#40490,#40491),(#40492,#40493),(#40494,#40495),
(#40496,#40497),(#40498,#40499),(#40500,#40501),(#40502,#40503),(#40504,
#40505),(#40506,#40507),(#40508,#40509),(#40510,#40511),(#40512,#40513),
(#40514,#40515),(#40516,#40517),(#40518,#40519),(#40520,#40521),(#40522,
#40523),(#40524,#40525),(#40526,#40527),(#40528,#40529),(#40530,#40531),
(#40532,#40533),(#40534,#40535),(#40536,#40537),(#40538,#40539),(#40540,
#40541),(#40542,#40543),(#40544,#40545),(#40546,#40547),(#40548,#40549),
(#40550,#40551),(#40552,#40553),(#40554,#40555),(#40556,#40557),(#40558,
#40559),(#40560,#40561),(#40562,#40563),(#40564,#40565)),.UNSPECIFIED.,
 .F.,.F.,.F.)
B_SPLINE_SURFACE_WITH_KNOTS((6,1,1,1,1,1,1,1,1,1,1,1,1,1,1,1,1,1,1,1,1,
1,1,1,1,1,1,1,1,1,1,1,1,1,1,1,1,1,1,1,1,1,1,1,1,1,1,1,1,1,1,1,1,1,1,1,1,
1,1,1,1,1,1,1,1,6),(2,2),(-1.,-0.984615384615383,-0.969230769230768,-0.953846153846152,
-0.938461538461537,-0.923076923076922,-0.907692307692306,-0.892307692307691,
-0.876923076923076,-0.86153846153846,-0.846153846153845,-0.83076923076923,
-0.815384615384614,-0.799999999999999,-0.784615384615384,-0.769230769230768,
-0.753846153846153,-0.738461538461538,-0.723076923076922,-0.707692307692307,
-0.692307692307692,-0.676923076923076,-0.661538461538461,-0.646153846153846,
-0.63076923076923,-0.615384615384615,-0.6,-0.584615384615384,-0.569230769230769,
-0.553846153846154,-0.538461538461538,-0.523076923076923,-0.507692307692308,
-0.492307692307692,-0.476923076923077,-0.461538461538462,-0.446153846153846,
-0.430769230769231,-0.415384615384615,-0.4,-0.384615384615385,-0.369230769230769,
-0.353846153846154,-0.338461538461538,-0.323076923076923,-0.307692307692308,
-0.292307692307692,-0.276923076923077,-0.261538461538462,-0.246153846153846,
-0.230769230769231,-0.215384615384615,-0.2,-0.184615384615385,-0.169230769230769,
-0.153846153846154,-0.138461538461538,-0.123076923076923,-0.107692307692308,
-0.0923076923076923,-0.0769230769230769,-0.0615384615384615,-0.0461538461538462,
-0.0307692307692308,-0.0153846153846154,0.),(-1.,1.),.UNSPECIFIED.)
GEOMETRIC_REPRESENTATION_ITEM()
RATIONAL_B_SPLINE_SURFACE(((1.,1.),(1.,1.),(1.,1.),(1.,1.),(1.,1.),(1.,
1.),(1.,1.),(1.,1.),(1.,1.),(1.,1.),(1.,1.),(1.,1.),(1.,1.),(1.,1.),(1.,
1.),(1.,1.),(1.,1.),(1.,1.),(1.,1.),(1.,1.),(1.,1.),(1.,1.),(1.,1.),(1.,
1.),(1.,1.),(1.,1.),(1.,1.),(1.,1.),(1.,1.),(1.,1.),(1.,1.),(1.,1.),(1.,
1.),(1.,1.),(1.,1.),(1.,1.),(1.,1.),(1.,1.),(1.,1.),(1.,1.),(1.,1.),(1.,
1.),(1.,1.),(1.,1.),(1.,1.),(1.,1.),(1.,1.),(1.,1.),(1.,1.),(1.,1.),(1.,
1.),(1.,1.),(1.,1.),(1.,1.),(1.,1.),(1.,1.),(1.,1.),(1.,1.),(1.,1.),(1.,
1.),(1.,1.),(1.,1.),(1.,1.),(1.,1.),(1.,1.),(1.,1.),(1.,1.),(1.,1.),(1.,
1.),(1.,1.)))
REPRESENTATION_ITEM('')
SURFACE()
);
#72=(
BOUNDED_SURFACE()
B_SPLINE_SURFACE(5,1,((#40638,#40639),(#40640,#40641),(#40642,#40643),(#40644,
#40645),(#40646,#40647),(#40648,#40649),(#40650,#40651),(#40652,#40653),
(#40654,#40655),(#40656,#40657),(#40658,#40659),(#40660,#40661),(#40662,
#40663),(#40664,#40665),(#40666,#40667),(#40668,#40669),(#40670,#40671),
(#40672,#40673),(#40674,#40675),(#40676,#40677),(#40678,#40679),(#40680,
#40681),(#40682,#40683),(#40684,#40685),(#40686,#40687),(#40688,#40689),
(#40690,#40691),(#40692,#40693),(#40694,#40695),(#40696,#40697),(#40698,
#40699),(#40700,#40701),(#40702,#40703),(#40704,#40705),(#40706,#40707),
(#40708,#40709),(#40710,#40711),(#40712,#40713),(#40714,#40715),(#40716,
#40717),(#40718,#40719),(#40720,#40721),(#40722,#40723),(#40724,#40725),
(#40726,#40727),(#40728,#40729),(#40730,#40731),(#40732,#40733),(#40734,
#40735),(#40736,#40737),(#40738,#40739),(#40740,#40741),(#40742,#40743),
(#40744,#40745),(#40746,#40747),(#40748,#40749),(#40750,#40751),(#40752,
#40753),(#40754,#40755),(#40756,#40757),(#40758,#40759),(#40760,#40761),
(#40762,#40763),(#40764,#40765),(#40766,#40767),(#40768,#40769),(#40770,
#40771),(#40772,#40773),(#40774,#40775),(#40776,#40777)),.UNSPECIFIED.,
 .F.,.F.,.F.)
B_SPLINE_SURFACE_WITH_KNOTS((6,1,1,1,1,1,1,1,1,1,1,1,1,1,1,1,1,1,1,1,1,
1,1,1,1,1,1,1,1,1,1,1,1,1,1,1,1,1,1,1,1,1,1,1,1,1,1,1,1,1,1,1,1,1,1,1,1,
1,1,1,1,1,1,1,1,6),(2,2),(-1.,-0.984615384615383,-0.969230769230768,-0.953846153846152,
-0.938461538461537,-0.923076923076922,-0.907692307692306,-0.892307692307691,
-0.876923076923076,-0.86153846153846,-0.846153846153845,-0.83076923076923,
-0.815384615384614,-0.799999999999999,-0.784615384615384,-0.769230769230768,
-0.753846153846153,-0.738461538461538,-0.723076923076922,-0.707692307692307,
-0.692307692307692,-0.676923076923076,-0.661538461538461,-0.646153846153846,
-0.63076923076923,-0.615384615384615,-0.6,-0.584615384615384,-0.569230769230769,
-0.553846153846154,-0.538461538461538,-0.523076923076923,-0.507692307692308,
-0.492307692307692,-0.476923076923077,-0.461538461538462,-0.446153846153846,
-0.430769230769231,-0.415384615384615,-0.4,-0.384615384615385,-0.369230769230769,
-0.353846153846154,-0.338461538461538,-0.323076923076923,-0.307692307692308,
-0.292307692307692,-0.276923076923077,-0.261538461538462,-0.246153846153846,
-0.230769230769231,-0.215384615384615,-0.2,-0.184615384615385,-0.169230769230769,
-0.153846153846154,-0.138461538461538,-0.123076923076923,-0.107692307692308,
-0.0923076923076923,-0.0769230769230769,-0.0615384615384615,-0.0461538461538462,
-0.0307692307692308,-0.0153846153846154,0.),(-1.,1.),.UNSPECIFIED.)
GEOMETRIC_REPRESENTATION_ITEM()
RATIONAL_B_SPLINE_SURFACE(((1.,1.),(1.,1.),(1.,1.),(1.,1.),(1.,1.),(1.,
1.),(1.,1.),(1.,1.),(1.,1.),(1.,1.),(1.,1.),(1.,1.),(1.,1.),(1.,1.),(1.,
1.),(1.,1.),(1.,1.),(1.,1.),(1.,1.),(1.,1.),(1.,1.),(1.,1.),(1.,1.),(1.,
1.),(1.,1.),(1.,1.),(1.,1.),(1.,1.),(1.,1.),(1.,1.),(1.,1.),(1.,1.),(1.,
1.),(1.,1.),(1.,1.),(1.,1.),(1.,1.),(1.,1.),(1.,1.),(1.,1.),(1.,1.),(1.,
1.),(1.,1.),(1.,1.),(1.,1.),(1.,1.),(1.,1.),(1.,1.),(1.,1.),(1.,1.),(1.,
1.),(1.,1.),(1.,1.),(1.,1.),(1.,1.),(1.,1.),(1.,1.),(1.,1.),(1.,1.),(1.,
1.),(1.,1.),(1.,1.),(1.,1.),(1.,1.),(1.,1.),(1.,1.),(1.,1.),(1.,1.),(1.,
1.),(1.,1.)))
REPRESENTATION_ITEM('')
SURFACE()
);
#73=(
BOUNDED_SURFACE()
B_SPLINE_SURFACE(5,1,((#40868,#40869),(#40870,#40871),(#40872,#40873),(#40874,
#40875),(#40876,#40877),(#40878,#40879),(#40880,#40881),(#40882,#40883),
(#40884,#40885),(#40886,#40887),(#40888,#40889),(#40890,#40891),(#40892,
#40893),(#40894,#40895),(#40896,#40897),(#40898,#40899),(#40900,#40901),
(#40902,#40903),(#40904,#40905),(#40906,#40907),(#40908,#40909),(#40910,
#40911),(#40912,#40913),(#40914,#40915),(#40916,#40917),(#40918,#40919),
(#40920,#40921),(#40922,#40923),(#40924,#40925),(#40926,#40927),(#40928,
#40929),(#40930,#40931),(#40932,#40933),(#40934,#40935),(#40936,#40937),
(#40938,#40939),(#40940,#40941),(#40942,#40943),(#40944,#40945),(#40946,
#40947),(#40948,#40949),(#40950,#40951),(#40952,#40953),(#40954,#40955),
(#40956,#40957),(#40958,#40959),(#40960,#40961),(#40962,#40963),(#40964,
#40965),(#40966,#40967),(#40968,#40969),(#40970,#40971),(#40972,#40973),
(#40974,#40975),(#40976,#40977),(#40978,#40979),(#40980,#40981),(#40982,
#40983),(#40984,#40985),(#40986,#40987),(#40988,#40989),(#40990,#40991),
(#40992,#40993),(#40994,#40995),(#40996,#40997),(#40998,#40999),(#41000,
#41001),(#41002,#41003),(#41004,#41005),(#41006,#41007)),.UNSPECIFIED.,
 .F.,.F.,.F.)
B_SPLINE_SURFACE_WITH_KNOTS((6,1,1,1,1,1,1,1,1,1,1,1,1,1,1,1,1,1,1,1,1,
1,1,1,1,1,1,1,1,1,1,1,1,1,1,1,1,1,1,1,1,1,1,1,1,1,1,1,1,1,1,1,1,1,1,1,1,
1,1,1,1,1,1,1,1,6),(2,2),(-1.,-0.984615384615383,-0.969230769230768,-0.953846153846152,
-0.938461538461537,-0.923076923076922,-0.907692307692306,-0.892307692307691,
-0.876923076923076,-0.86153846153846,-0.846153846153845,-0.83076923076923,
-0.815384615384614,-0.799999999999999,-0.784615384615384,-0.769230769230768,
-0.753846153846153,-0.738461538461538,-0.723076923076922,-0.707692307692307,
-0.692307692307692,-0.676923076923076,-0.661538461538461,-0.646153846153846,
-0.63076923076923,-0.615384615384615,-0.6,-0.584615384615384,-0.569230769230769,
-0.553846153846154,-0.538461538461538,-0.523076923076923,-0.507692307692308,
-0.492307692307692,-0.476923076923077,-0.461538461538462,-0.446153846153846,
-0.430769230769231,-0.415384615384615,-0.4,-0.384615384615385,-0.369230769230769,
-0.353846153846154,-0.338461538461538,-0.323076923076923,-0.307692307692308,
-0.292307692307692,-0.276923076923077,-0.261538461538462,-0.246153846153846,
-0.230769230769231,-0.215384615384615,-0.2,-0.184615384615385,-0.169230769230769,
-0.153846153846154,-0.138461538461538,-0.123076923076923,-0.107692307692308,
-0.0923076923076923,-0.0769230769230769,-0.0615384615384615,-0.0461538461538462,
-0.0307692307692308,-0.0153846153846154,0.),(-1.,1.),.UNSPECIFIED.)
GEOMETRIC_REPRESENTATION_ITEM()
RATIONAL_B_SPLINE_SURFACE(((1.,1.),(1.,1.),(1.,1.),(1.,1.),(1.,1.),(1.,
1.),(1.,1.),(1.,1.),(1.,1.),(1.,1.),(1.,1.),(1.,1.),(1.,1.),(1.,1.),(1.,
1.),(1.,1.),(1.,1.),(1.,1.),(1.,1.),(1.,1.),(1.,1.),(1.,1.),(1.,1.),(1.,
1.),(1.,1.),(1.,1.),(1.,1.),(1.,1.),(1.,1.),(1.,1.),(1.,1.),(1.,1.),(1.,
1.),(1.,1.),(1.,1.),(1.,1.),(1.,1.),(1.,1.),(1.,1.),(1.,1.),(1.,1.),(1.,
1.),(1.,1.),(1.,1.),(1.,1.),(1.,1.),(1.,1.),(1.,1.),(1.,1.),(1.,1.),(1.,
1.),(1.,1.),(1.,1.),(1.,1.),(1.,1.),(1.,1.),(1.,1.),(1.,1.),(1.,1.),(1.,
1.),(1.,1.),(1.,1.),(1.,1.),(1.,1.),(1.,1.),(1.,1.),(1.,1.),(1.,1.),(1.,
1.),(1.,1.)))
REPRESENTATION_ITEM('')
SURFACE()
);
#74=(
BOUNDED_SURFACE()
B_SPLINE_SURFACE(5,1,((#41080,#41081),(#41082,#41083),(#41084,#41085),(#41086,
#41087),(#41088,#41089),(#41090,#41091),(#41092,#41093),(#41094,#41095),
(#41096,#41097),(#41098,#41099),(#41100,#41101),(#41102,#41103),(#41104,
#41105),(#41106,#41107),(#41108,#41109),(#41110,#41111),(#41112,#41113),
(#41114,#41115),(#41116,#41117),(#41118,#41119),(#41120,#41121),(#41122,
#41123),(#41124,#41125),(#41126,#41127),(#41128,#41129),(#41130,#41131),
(#41132,#41133),(#41134,#41135),(#41136,#41137),(#41138,#41139),(#41140,
#41141),(#41142,#41143),(#41144,#41145),(#41146,#41147),(#41148,#41149),
(#41150,#41151),(#41152,#41153),(#41154,#41155),(#41156,#41157),(#41158,
#41159),(#41160,#41161),(#41162,#41163),(#41164,#41165),(#41166,#41167),
(#41168,#41169),(#41170,#41171),(#41172,#41173),(#41174,#41175),(#41176,
#41177),(#41178,#41179),(#41180,#41181),(#41182,#41183),(#41184,#41185),
(#41186,#41187),(#41188,#41189),(#41190,#41191),(#41192,#41193),(#41194,
#41195),(#41196,#41197),(#41198,#41199),(#41200,#41201),(#41202,#41203),
(#41204,#41205),(#41206,#41207),(#41208,#41209),(#41210,#41211),(#41212,
#41213),(#41214,#41215),(#41216,#41217),(#41218,#41219)),.UNSPECIFIED.,
 .F.,.F.,.F.)
B_SPLINE_SURFACE_WITH_KNOTS((6,1,1,1,1,1,1,1,1,1,1,1,1,1,1,1,1,1,1,1,1,
1,1,1,1,1,1,1,1,1,1,1,1,1,1,1,1,1,1,1,1,1,1,1,1,1,1,1,1,1,1,1,1,1,1,1,1,
1,1,1,1,1,1,1,1,6),(2,2),(-1.,-0.984615384615383,-0.969230769230768,-0.953846153846152,
-0.938461538461537,-0.923076923076922,-0.907692307692306,-0.892307692307691,
-0.876923076923076,-0.86153846153846,-0.846153846153845,-0.83076923076923,
-0.815384615384614,-0.799999999999999,-0.784615384615384,-0.769230769230768,
-0.753846153846153,-0.738461538461538,-0.723076923076922,-0.707692307692307,
-0.692307692307692,-0.676923076923076,-0.661538461538461,-0.646153846153846,
-0.63076923076923,-0.615384615384615,-0.6,-0.584615384615384,-0.569230769230769,
-0.553846153846154,-0.538461538461538,-0.523076923076923,-0.507692307692308,
-0.492307692307692,-0.476923076923077,-0.461538461538462,-0.446153846153846,
-0.430769230769231,-0.415384615384615,-0.4,-0.384615384615385,-0.369230769230769,
-0.353846153846154,-0.338461538461538,-0.323076923076923,-0.307692307692308,
-0.292307692307692,-0.276923076923077,-0.261538461538462,-0.246153846153846,
-0.230769230769231,-0.215384615384615,-0.2,-0.184615384615385,-0.169230769230769,
-0.153846153846154,-0.138461538461538,-0.123076923076923,-0.107692307692308,
-0.0923076923076923,-0.0769230769230769,-0.0615384615384615,-0.0461538461538462,
-0.0307692307692308,-0.0153846153846154,0.),(-1.,1.),.UNSPECIFIED.)
GEOMETRIC_REPRESENTATION_ITEM()
RATIONAL_B_SPLINE_SURFACE(((1.,1.),(1.,1.),(1.,1.),(1.,1.),(1.,1.),(1.,
1.),(1.,1.),(1.,1.),(1.,1.),(1.,1.),(1.,1.),(1.,1.),(1.,1.),(1.,1.),(1.,
1.),(1.,1.),(1.,1.),(1.,1.),(1.,1.),(1.,1.),(1.,1.),(1.,1.),(1.,1.),(1.,
1.),(1.,1.),(1.,1.),(1.,1.),(1.,1.),(1.,1.),(1.,1.),(1.,1.),(1.,1.),(1.,
1.),(1.,1.),(1.,1.),(1.,1.),(1.,1.),(1.,1.),(1.,1.),(1.,1.),(1.,1.),(1.,
1.),(1.,1.),(1.,1.),(1.,1.),(1.,1.),(1.,1.),(1.,1.),(1.,1.),(1.,1.),(1.,
1.),(1.,1.),(1.,1.),(1.,1.),(1.,1.),(1.,1.),(1.,1.),(1.,1.),(1.,1.),(1.,
1.),(1.,1.),(1.,1.),(1.,1.),(1.,1.),(1.,1.),(1.,1.),(1.,1.),(1.,1.),(1.,
1.),(1.,1.)))
REPRESENTATION_ITEM('')
SURFACE()
);
#75=(
BOUNDED_SURFACE()
B_SPLINE_SURFACE(5,1,((#41310,#41311),(#41312,#41313),(#41314,#41315),(#41316,
#41317),(#41318,#41319),(#41320,#41321),(#41322,#41323),(#41324,#41325),
(#41326,#41327),(#41328,#41329),(#41330,#41331),(#41332,#41333),(#41334,
#41335),(#41336,#41337),(#41338,#41339),(#41340,#41341),(#41342,#41343),
(#41344,#41345),(#41346,#41347),(#41348,#41349),(#41350,#41351),(#41352,
#41353),(#41354,#41355),(#41356,#41357),(#41358,#41359),(#41360,#41361),
(#41362,#41363),(#41364,#41365),(#41366,#41367),(#41368,#41369),(#41370,
#41371),(#41372,#41373),(#41374,#41375),(#41376,#41377),(#41378,#41379),
(#41380,#41381),(#41382,#41383),(#41384,#41385),(#41386,#41387),(#41388,
#41389),(#41390,#41391),(#41392,#41393),(#41394,#41395),(#41396,#41397),
(#41398,#41399),(#41400,#41401),(#41402,#41403),(#41404,#41405),(#41406,
#41407),(#41408,#41409),(#41410,#41411),(#41412,#41413),(#41414,#41415),
(#41416,#41417),(#41418,#41419),(#41420,#41421),(#41422,#41423),(#41424,
#41425),(#41426,#41427),(#41428,#41429),(#41430,#41431),(#41432,#41433),
(#41434,#41435),(#41436,#41437),(#41438,#41439),(#41440,#41441),(#41442,
#41443),(#41444,#41445),(#41446,#41447),(#41448,#41449)),.UNSPECIFIED.,
 .F.,.F.,.F.)
B_SPLINE_SURFACE_WITH_KNOTS((6,1,1,1,1,1,1,1,1,1,1,1,1,1,1,1,1,1,1,1,1,
1,1,1,1,1,1,1,1,1,1,1,1,1,1,1,1,1,1,1,1,1,1,1,1,1,1,1,1,1,1,1,1,1,1,1,1,
1,1,1,1,1,1,1,1,6),(2,2),(-1.,-0.984615384615383,-0.969230769230768,-0.953846153846152,
-0.938461538461537,-0.923076923076922,-0.907692307692306,-0.892307692307691,
-0.876923076923076,-0.86153846153846,-0.846153846153845,-0.83076923076923,
-0.815384615384614,-0.799999999999999,-0.784615384615384,-0.769230769230768,
-0.753846153846153,-0.738461538461538,-0.723076923076922,-0.707692307692307,
-0.692307692307692,-0.676923076923076,-0.661538461538461,-0.646153846153846,
-0.63076923076923,-0.615384615384615,-0.6,-0.584615384615384,-0.569230769230769,
-0.553846153846154,-0.538461538461538,-0.523076923076923,-0.507692307692308,
-0.492307692307692,-0.476923076923077,-0.461538461538462,-0.446153846153846,
-0.430769230769231,-0.415384615384615,-0.4,-0.384615384615385,-0.369230769230769,
-0.353846153846154,-0.338461538461538,-0.323076923076923,-0.307692307692308,
-0.292307692307692,-0.276923076923077,-0.261538461538462,-0.246153846153846,
-0.230769230769231,-0.215384615384615,-0.2,-0.184615384615385,-0.169230769230769,
-0.153846153846154,-0.138461538461538,-0.123076923076923,-0.107692307692308,
-0.0923076923076923,-0.0769230769230769,-0.0615384615384615,-0.0461538461538462,
-0.0307692307692308,-0.0153846153846154,0.),(-1.,1.),.UNSPECIFIED.)
GEOMETRIC_REPRESENTATION_ITEM()
RATIONAL_B_SPLINE_SURFACE(((1.,1.),(1.,1.),(1.,1.),(1.,1.),(1.,1.),(1.,
1.),(1.,1.),(1.,1.),(1.,1.),(1.,1.),(1.,1.),(1.,1.),(1.,1.),(1.,1.),(1.,
1.),(1.,1.),(1.,1.),(1.,1.),(1.,1.),(1.,1.),(1.,1.),(1.,1.),(1.,1.),(1.,
1.),(1.,1.),(1.,1.),(1.,1.),(1.,1.),(1.,1.),(1.,1.),(1.,1.),(1.,1.),(1.,
1.),(1.,1.),(1.,1.),(1.,1.),(1.,1.),(1.,1.),(1.,1.),(1.,1.),(1.,1.),(1.,
1.),(1.,1.),(1.,1.),(1.,1.),(1.,1.),(1.,1.),(1.,1.),(1.,1.),(1.,1.),(1.,
1.),(1.,1.),(1.,1.),(1.,1.),(1.,1.),(1.,1.),(1.,1.),(1.,1.),(1.,1.),(1.,
1.),(1.,1.),(1.,1.),(1.,1.),(1.,1.),(1.,1.),(1.,1.),(1.,1.),(1.,1.),(1.,
1.),(1.,1.)))
REPRESENTATION_ITEM('')
SURFACE()
);
#76=(
BOUNDED_SURFACE()
B_SPLINE_SURFACE(5,1,((#41522,#41523),(#41524,#41525),(#41526,#41527),(#41528,
#41529),(#41530,#41531),(#41532,#41533),(#41534,#41535),(#41536,#41537),
(#41538,#41539),(#41540,#41541),(#41542,#41543),(#41544,#41545),(#41546,
#41547),(#41548,#41549),(#41550,#41551),(#41552,#41553),(#41554,#41555),
(#41556,#41557),(#41558,#41559),(#41560,#41561),(#41562,#41563),(#41564,
#41565),(#41566,#41567),(#41568,#41569),(#41570,#41571),(#41572,#41573),
(#41574,#41575),(#41576,#41577),(#41578,#41579),(#41580,#41581),(#41582,
#41583),(#41584,#41585),(#41586,#41587),(#41588,#41589),(#41590,#41591),
(#41592,#41593),(#41594,#41595),(#41596,#41597),(#41598,#41599),(#41600,
#41601),(#41602,#41603),(#41604,#41605),(#41606,#41607),(#41608,#41609),
(#41610,#41611),(#41612,#41613),(#41614,#41615),(#41616,#41617),(#41618,
#41619),(#41620,#41621),(#41622,#41623),(#41624,#41625),(#41626,#41627),
(#41628,#41629),(#41630,#41631),(#41632,#41633),(#41634,#41635),(#41636,
#41637),(#41638,#41639),(#41640,#41641),(#41642,#41643),(#41644,#41645),
(#41646,#41647),(#41648,#41649),(#41650,#41651),(#41652,#41653),(#41654,
#41655),(#41656,#41657),(#41658,#41659),(#41660,#41661)),.UNSPECIFIED.,
 .F.,.F.,.F.)
B_SPLINE_SURFACE_WITH_KNOTS((6,1,1,1,1,1,1,1,1,1,1,1,1,1,1,1,1,1,1,1,1,
1,1,1,1,1,1,1,1,1,1,1,1,1,1,1,1,1,1,1,1,1,1,1,1,1,1,1,1,1,1,1,1,1,1,1,1,
1,1,1,1,1,1,1,1,6),(2,2),(-1.,-0.984615384615383,-0.969230769230768,-0.953846153846152,
-0.938461538461537,-0.923076923076922,-0.907692307692306,-0.892307692307691,
-0.876923076923076,-0.86153846153846,-0.846153846153845,-0.83076923076923,
-0.815384615384614,-0.799999999999999,-0.784615384615384,-0.769230769230768,
-0.753846153846153,-0.738461538461538,-0.723076923076922,-0.707692307692307,
-0.692307692307692,-0.676923076923076,-0.661538461538461,-0.646153846153846,
-0.63076923076923,-0.615384615384615,-0.6,-0.584615384615384,-0.569230769230769,
-0.553846153846154,-0.538461538461538,-0.523076923076923,-0.507692307692308,
-0.492307692307692,-0.476923076923077,-0.461538461538462,-0.446153846153846,
-0.430769230769231,-0.415384615384615,-0.4,-0.384615384615385,-0.369230769230769,
-0.353846153846154,-0.338461538461538,-0.323076923076923,-0.307692307692308,
-0.292307692307692,-0.276923076923077,-0.261538461538462,-0.246153846153846,
-0.230769230769231,-0.215384615384615,-0.2,-0.184615384615385,-0.169230769230769,
-0.153846153846154,-0.138461538461538,-0.123076923076923,-0.107692307692308,
-0.0923076923076923,-0.0769230769230769,-0.0615384615384615,-0.0461538461538462,
-0.0307692307692308,-0.0153846153846154,0.),(-1.,1.),.UNSPECIFIED.)
GEOMETRIC_REPRESENTATION_ITEM()
RATIONAL_B_SPLINE_SURFACE(((1.,1.),(1.,1.),(1.,1.),(1.,1.),(1.,1.),(1.,
1.),(1.,1.),(1.,1.),(1.,1.),(1.,1.),(1.,1.),(1.,1.),(1.,1.),(1.,1.),(1.,
1.),(1.,1.),(1.,1.),(1.,1.),(1.,1.),(1.,1.),(1.,1.),(1.,1.),(1.,1.),(1.,
1.),(1.,1.),(1.,1.),(1.,1.),(1.,1.),(1.,1.),(1.,1.),(1.,1.),(1.,1.),(1.,
1.),(1.,1.),(1.,1.),(1.,1.),(1.,1.),(1.,1.),(1.,1.),(1.,1.),(1.,1.),(1.,
1.),(1.,1.),(1.,1.),(1.,1.),(1.,1.),(1.,1.),(1.,1.),(1.,1.),(1.,1.),(1.,
1.),(1.,1.),(1.,1.),(1.,1.),(1.,1.),(1.,1.),(1.,1.),(1.,1.),(1.,1.),(1.,
1.),(1.,1.),(1.,1.),(1.,1.),(1.,1.),(1.,1.),(1.,1.),(1.,1.),(1.,1.),(1.,
1.),(1.,1.)))
REPRESENTATION_ITEM('')
SURFACE()
);
#77=(
BOUNDED_SURFACE()
B_SPLINE_SURFACE(5,1,((#41752,#41753),(#41754,#41755),(#41756,#41757),(#41758,
#41759),(#41760,#41761),(#41762,#41763),(#41764,#41765),(#41766,#41767),
(#41768,#41769),(#41770,#41771),(#41772,#41773),(#41774,#41775),(#41776,
#41777),(#41778,#41779),(#41780,#41781),(#41782,#41783),(#41784,#41785),
(#41786,#41787),(#41788,#41789),(#41790,#41791),(#41792,#41793),(#41794,
#41795),(#41796,#41797),(#41798,#41799),(#41800,#41801),(#41802,#41803),
(#41804,#41805),(#41806,#41807),(#41808,#41809),(#41810,#41811),(#41812,
#41813),(#41814,#41815),(#41816,#41817),(#41818,#41819),(#41820,#41821),
(#41822,#41823),(#41824,#41825),(#41826,#41827),(#41828,#41829),(#41830,
#41831),(#41832,#41833),(#41834,#41835),(#41836,#41837),(#41838,#41839),
(#41840,#41841),(#41842,#41843),(#41844,#41845),(#41846,#41847),(#41848,
#41849),(#41850,#41851),(#41852,#41853),(#41854,#41855),(#41856,#41857),
(#41858,#41859),(#41860,#41861),(#41862,#41863),(#41864,#41865),(#41866,
#41867),(#41868,#41869),(#41870,#41871),(#41872,#41873),(#41874,#41875),
(#41876,#41877),(#41878,#41879),(#41880,#41881),(#41882,#41883),(#41884,
#41885),(#41886,#41887),(#41888,#41889),(#41890,#41891)),.UNSPECIFIED.,
 .F.,.F.,.F.)
B_SPLINE_SURFACE_WITH_KNOTS((6,1,1,1,1,1,1,1,1,1,1,1,1,1,1,1,1,1,1,1,1,
1,1,1,1,1,1,1,1,1,1,1,1,1,1,1,1,1,1,1,1,1,1,1,1,1,1,1,1,1,1,1,1,1,1,1,1,
1,1,1,1,1,1,1,1,6),(2,2),(-1.,-0.984615384615383,-0.969230769230768,-0.953846153846152,
-0.938461538461537,-0.923076923076922,-0.907692307692306,-0.892307692307691,
-0.876923076923076,-0.86153846153846,-0.846153846153845,-0.83076923076923,
-0.815384615384614,-0.799999999999999,-0.784615384615384,-0.769230769230768,
-0.753846153846153,-0.738461538461538,-0.723076923076922,-0.707692307692307,
-0.692307692307692,-0.676923076923076,-0.661538461538461,-0.646153846153846,
-0.63076923076923,-0.615384615384615,-0.6,-0.584615384615384,-0.569230769230769,
-0.553846153846154,-0.538461538461538,-0.523076923076923,-0.507692307692308,
-0.492307692307692,-0.476923076923077,-0.461538461538462,-0.446153846153846,
-0.430769230769231,-0.415384615384615,-0.4,-0.384615384615385,-0.369230769230769,
-0.353846153846154,-0.338461538461538,-0.323076923076923,-0.307692307692308,
-0.292307692307692,-0.276923076923077,-0.261538461538462,-0.246153846153846,
-0.230769230769231,-0.215384615384615,-0.2,-0.184615384615385,-0.169230769230769,
-0.153846153846154,-0.138461538461538,-0.123076923076923,-0.107692307692308,
-0.0923076923076923,-0.0769230769230769,-0.0615384615384615,-0.0461538461538462,
-0.0307692307692308,-0.0153846153846154,0.),(-1.,1.),.UNSPECIFIED.)
GEOMETRIC_REPRESENTATION_ITEM()
RATIONAL_B_SPLINE_SURFACE(((1.,1.),(1.,1.),(1.,1.),(1.,1.),(1.,1.),(1.,
1.),(1.,1.),(1.,1.),(1.,1.),(1.,1.),(1.,1.),(1.,1.),(1.,1.),(1.,1.),(1.,
1.),(1.,1.),(1.,1.),(1.,1.),(1.,1.),(1.,1.),(1.,1.),(1.,1.),(1.,1.),(1.,
1.),(1.,1.),(1.,1.),(1.,1.),(1.,1.),(1.,1.),(1.,1.),(1.,1.),(1.,1.),(1.,
1.),(1.,1.),(1.,1.),(1.,1.),(1.,1.),(1.,1.),(1.,1.),(1.,1.),(1.,1.),(1.,
1.),(1.,1.),(1.,1.),(1.,1.),(1.,1.),(1.,1.),(1.,1.),(1.,1.),(1.,1.),(1.,
1.),(1.,1.),(1.,1.),(1.,1.),(1.,1.),(1.,1.),(1.,1.),(1.,1.),(1.,1.),(1.,
1.),(1.,1.),(1.,1.),(1.,1.),(1.,1.),(1.,1.),(1.,1.),(1.,1.),(1.,1.),(1.,
1.),(1.,1.)))
REPRESENTATION_ITEM('')
SURFACE()
);
#78=(
BOUNDED_SURFACE()
B_SPLINE_SURFACE(5,1,((#41964,#41965),(#41966,#41967),(#41968,#41969),(#41970,
#41971),(#41972,#41973),(#41974,#41975),(#41976,#41977),(#41978,#41979),
(#41980,#41981),(#41982,#41983),(#41984,#41985),(#41986,#41987),(#41988,
#41989),(#41990,#41991),(#41992,#41993),(#41994,#41995),(#41996,#41997),
(#41998,#41999),(#42000,#42001),(#42002,#42003),(#42004,#42005),(#42006,
#42007),(#42008,#42009),(#42010,#42011),(#42012,#42013),(#42014,#42015),
(#42016,#42017),(#42018,#42019),(#42020,#42021),(#42022,#42023),(#42024,
#42025),(#42026,#42027),(#42028,#42029),(#42030,#42031),(#42032,#42033),
(#42034,#42035),(#42036,#42037),(#42038,#42039),(#42040,#42041),(#42042,
#42043),(#42044,#42045),(#42046,#42047),(#42048,#42049),(#42050,#42051),
(#42052,#42053),(#42054,#42055),(#42056,#42057),(#42058,#42059),(#42060,
#42061),(#42062,#42063),(#42064,#42065),(#42066,#42067),(#42068,#42069),
(#42070,#42071),(#42072,#42073),(#42074,#42075),(#42076,#42077),(#42078,
#42079),(#42080,#42081),(#42082,#42083),(#42084,#42085),(#42086,#42087),
(#42088,#42089),(#42090,#42091),(#42092,#42093),(#42094,#42095),(#42096,
#42097),(#42098,#42099),(#42100,#42101),(#42102,#42103)),.UNSPECIFIED.,
 .F.,.F.,.F.)
B_SPLINE_SURFACE_WITH_KNOTS((6,1,1,1,1,1,1,1,1,1,1,1,1,1,1,1,1,1,1,1,1,
1,1,1,1,1,1,1,1,1,1,1,1,1,1,1,1,1,1,1,1,1,1,1,1,1,1,1,1,1,1,1,1,1,1,1,1,
1,1,1,1,1,1,1,1,6),(2,2),(-1.,-0.984615384615383,-0.969230769230768,-0.953846153846152,
-0.938461538461537,-0.923076923076922,-0.907692307692306,-0.892307692307691,
-0.876923076923076,-0.86153846153846,-0.846153846153845,-0.83076923076923,
-0.815384615384614,-0.799999999999999,-0.784615384615384,-0.769230769230768,
-0.753846153846153,-0.738461538461538,-0.723076923076922,-0.707692307692307,
-0.692307692307692,-0.676923076923076,-0.661538461538461,-0.646153846153846,
-0.63076923076923,-0.615384615384615,-0.6,-0.584615384615384,-0.569230769230769,
-0.553846153846154,-0.538461538461538,-0.523076923076923,-0.507692307692308,
-0.492307692307692,-0.476923076923077,-0.461538461538462,-0.446153846153846,
-0.430769230769231,-0.415384615384615,-0.4,-0.384615384615385,-0.369230769230769,
-0.353846153846154,-0.338461538461538,-0.323076923076923,-0.307692307692308,
-0.292307692307692,-0.276923076923077,-0.261538461538462,-0.246153846153846,
-0.230769230769231,-0.215384615384615,-0.2,-0.184615384615385,-0.169230769230769,
-0.153846153846154,-0.138461538461538,-0.123076923076923,-0.107692307692308,
-0.0923076923076923,-0.0769230769230769,-0.0615384615384615,-0.0461538461538462,
-0.0307692307692308,-0.0153846153846154,0.),(-1.,1.),.UNSPECIFIED.)
GEOMETRIC_REPRESENTATION_ITEM()
RATIONAL_B_SPLINE_SURFACE(((1.,1.),(1.,1.),(1.,1.),(1.,1.),(1.,1.),(1.,
1.),(1.,1.),(1.,1.),(1.,1.),(1.,1.),(1.,1.),(1.,1.),(1.,1.),(1.,1.),(1.,
1.),(1.,1.),(1.,1.),(1.,1.),(1.,1.),(1.,1.),(1.,1.),(1.,1.),(1.,1.),(1.,
1.),(1.,1.),(1.,1.),(1.,1.),(1.,1.),(1.,1.),(1.,1.),(1.,1.),(1.,1.),(1.,
1.),(1.,1.),(1.,1.),(1.,1.),(1.,1.),(1.,1.),(1.,1.),(1.,1.),(1.,1.),(1.,
1.),(1.,1.),(1.,1.),(1.,1.),(1.,1.),(1.,1.),(1.,1.),(1.,1.),(1.,1.),(1.,
1.),(1.,1.),(1.,1.),(1.,1.),(1.,1.),(1.,1.),(1.,1.),(1.,1.),(1.,1.),(1.,
1.),(1.,1.),(1.,1.),(1.,1.),(1.,1.),(1.,1.),(1.,1.),(1.,1.),(1.,1.),(1.,
1.),(1.,1.)))
REPRESENTATION_ITEM('')
SURFACE()
);
#79=(
BOUNDED_SURFACE()
B_SPLINE_SURFACE(5,1,((#42194,#42195),(#42196,#42197),(#42198,#42199),(#42200,
#42201),(#42202,#42203),(#42204,#42205),(#42206,#42207),(#42208,#42209),
(#42210,#42211),(#42212,#42213),(#42214,#42215),(#42216,#42217),(#42218,
#42219),(#42220,#42221),(#42222,#42223),(#42224,#42225),(#42226,#42227),
(#42228,#42229),(#42230,#42231),(#42232,#42233),(#42234,#42235),(#42236,
#42237),(#42238,#42239),(#42240,#42241),(#42242,#42243),(#42244,#42245),
(#42246,#42247),(#42248,#42249),(#42250,#42251),(#42252,#42253),(#42254,
#42255),(#42256,#42257),(#42258,#42259),(#42260,#42261),(#42262,#42263),
(#42264,#42265),(#42266,#42267),(#42268,#42269),(#42270,#42271),(#42272,
#42273),(#42274,#42275),(#42276,#42277),(#42278,#42279),(#42280,#42281),
(#42282,#42283),(#42284,#42285),(#42286,#42287),(#42288,#42289),(#42290,
#42291),(#42292,#42293),(#42294,#42295),(#42296,#42297),(#42298,#42299),
(#42300,#42301),(#42302,#42303),(#42304,#42305),(#42306,#42307),(#42308,
#42309),(#42310,#42311),(#42312,#42313),(#42314,#42315),(#42316,#42317),
(#42318,#42319),(#42320,#42321),(#42322,#42323),(#42324,#42325),(#42326,
#42327),(#42328,#42329),(#42330,#42331),(#42332,#42333)),.UNSPECIFIED.,
 .F.,.F.,.F.)
B_SPLINE_SURFACE_WITH_KNOTS((6,1,1,1,1,1,1,1,1,1,1,1,1,1,1,1,1,1,1,1,1,
1,1,1,1,1,1,1,1,1,1,1,1,1,1,1,1,1,1,1,1,1,1,1,1,1,1,1,1,1,1,1,1,1,1,1,1,
1,1,1,1,1,1,1,1,6),(2,2),(-1.,-0.984615384615383,-0.969230769230768,-0.953846153846152,
-0.938461538461537,-0.923076923076922,-0.907692307692306,-0.892307692307691,
-0.876923076923076,-0.86153846153846,-0.846153846153845,-0.83076923076923,
-0.815384615384614,-0.799999999999999,-0.784615384615384,-0.769230769230768,
-0.753846153846153,-0.738461538461538,-0.723076923076922,-0.707692307692307,
-0.692307692307692,-0.676923076923076,-0.661538461538461,-0.646153846153846,
-0.63076923076923,-0.615384615384615,-0.6,-0.584615384615384,-0.569230769230769,
-0.553846153846154,-0.538461538461538,-0.523076923076923,-0.507692307692308,
-0.492307692307692,-0.476923076923077,-0.461538461538462,-0.446153846153846,
-0.430769230769231,-0.415384615384615,-0.4,-0.384615384615385,-0.369230769230769,
-0.353846153846154,-0.338461538461538,-0.323076923076923,-0.307692307692308,
-0.292307692307692,-0.276923076923077,-0.261538461538462,-0.246153846153846,
-0.230769230769231,-0.215384615384615,-0.2,-0.184615384615385,-0.169230769230769,
-0.153846153846154,-0.138461538461538,-0.123076923076923,-0.107692307692308,
-0.0923076923076923,-0.0769230769230769,-0.0615384615384615,-0.0461538461538462,
-0.0307692307692308,-0.0153846153846154,0.),(-1.,1.),.UNSPECIFIED.)
GEOMETRIC_REPRESENTATION_ITEM()
RATIONAL_B_SPLINE_SURFACE(((1.,1.),(1.,1.),(1.,1.),(1.,1.),(1.,1.),(1.,
1.),(1.,1.),(1.,1.),(1.,1.),(1.,1.),(1.,1.),(1.,1.),(1.,1.),(1.,1.),(1.,
1.),(1.,1.),(1.,1.),(1.,1.),(1.,1.),(1.,1.),(1.,1.),(1.,1.),(1.,1.),(1.,
1.),(1.,1.),(1.,1.),(1.,1.),(1.,1.),(1.,1.),(1.,1.),(1.,1.),(1.,1.),(1.,
1.),(1.,1.),(1.,1.),(1.,1.),(1.,1.),(1.,1.),(1.,1.),(1.,1.),(1.,1.),(1.,
1.),(1.,1.),(1.,1.),(1.,1.),(1.,1.),(1.,1.),(1.,1.),(1.,1.),(1.,1.),(1.,
1.),(1.,1.),(1.,1.),(1.,1.),(1.,1.),(1.,1.),(1.,1.),(1.,1.),(1.,1.),(1.,
1.),(1.,1.),(1.,1.),(1.,1.),(1.,1.),(1.,1.),(1.,1.),(1.,1.),(1.,1.),(1.,
1.),(1.,1.)))
REPRESENTATION_ITEM('')
SURFACE()
);
#80=(
BOUNDED_SURFACE()
B_SPLINE_SURFACE(5,1,((#42406,#42407),(#42408,#42409),(#42410,#42411),(#42412,
#42413),(#42414,#42415),(#42416,#42417),(#42418,#42419),(#42420,#42421),
(#42422,#42423),(#42424,#42425),(#42426,#42427),(#42428,#42429),(#42430,
#42431),(#42432,#42433),(#42434,#42435),(#42436,#42437),(#42438,#42439),
(#42440,#42441),(#42442,#42443),(#42444,#42445),(#42446,#42447),(#42448,
#42449),(#42450,#42451),(#42452,#42453),(#42454,#42455),(#42456,#42457),
(#42458,#42459),(#42460,#42461),(#42462,#42463),(#42464,#42465),(#42466,
#42467),(#42468,#42469),(#42470,#42471),(#42472,#42473),(#42474,#42475),
(#42476,#42477),(#42478,#42479),(#42480,#42481),(#42482,#42483),(#42484,
#42485),(#42486,#42487),(#42488,#42489),(#42490,#42491),(#42492,#42493),
(#42494,#42495),(#42496,#42497),(#42498,#42499),(#42500,#42501),(#42502,
#42503),(#42504,#42505),(#42506,#42507),(#42508,#42509),(#42510,#42511),
(#42512,#42513),(#42514,#42515),(#42516,#42517),(#42518,#42519),(#42520,
#42521),(#42522,#42523),(#42524,#42525),(#42526,#42527),(#42528,#42529),
(#42530,#42531),(#42532,#42533),(#42534,#42535),(#42536,#42537),(#42538,
#42539),(#42540,#42541),(#42542,#42543),(#42544,#42545)),.UNSPECIFIED.,
 .F.,.F.,.F.)
B_SPLINE_SURFACE_WITH_KNOTS((6,1,1,1,1,1,1,1,1,1,1,1,1,1,1,1,1,1,1,1,1,
1,1,1,1,1,1,1,1,1,1,1,1,1,1,1,1,1,1,1,1,1,1,1,1,1,1,1,1,1,1,1,1,1,1,1,1,
1,1,1,1,1,1,1,1,6),(2,2),(-1.,-0.984615384615383,-0.969230769230768,-0.953846153846152,
-0.938461538461537,-0.923076923076922,-0.907692307692306,-0.892307692307691,
-0.876923076923076,-0.86153846153846,-0.846153846153845,-0.83076923076923,
-0.815384615384614,-0.799999999999999,-0.784615384615384,-0.769230769230768,
-0.753846153846153,-0.738461538461538,-0.723076923076922,-0.707692307692307,
-0.692307692307692,-0.676923076923076,-0.661538461538461,-0.646153846153846,
-0.63076923076923,-0.615384615384615,-0.6,-0.584615384615384,-0.569230769230769,
-0.553846153846154,-0.538461538461538,-0.523076923076923,-0.507692307692308,
-0.492307692307692,-0.476923076923077,-0.461538461538462,-0.446153846153846,
-0.430769230769231,-0.415384615384615,-0.4,-0.384615384615385,-0.369230769230769,
-0.353846153846154,-0.338461538461538,-0.323076923076923,-0.307692307692308,
-0.292307692307692,-0.276923076923077,-0.261538461538462,-0.246153846153846,
-0.230769230769231,-0.215384615384615,-0.2,-0.184615384615385,-0.169230769230769,
-0.153846153846154,-0.138461538461538,-0.123076923076923,-0.107692307692308,
-0.0923076923076923,-0.0769230769230769,-0.0615384615384615,-0.0461538461538462,
-0.0307692307692308,-0.0153846153846154,0.),(-1.,1.),.UNSPECIFIED.)
GEOMETRIC_REPRESENTATION_ITEM()
RATIONAL_B_SPLINE_SURFACE(((1.,1.),(1.,1.),(1.,1.),(1.,1.),(1.,1.),(1.,
1.),(1.,1.),(1.,1.),(1.,1.),(1.,1.),(1.,1.),(1.,1.),(1.,1.),(1.,1.),(1.,
1.),(1.,1.),(1.,1.),(1.,1.),(1.,1.),(1.,1.),(1.,1.),(1.,1.),(1.,1.),(1.,
1.),(1.,1.),(1.,1.),(1.,1.),(1.,1.),(1.,1.),(1.,1.),(1.,1.),(1.,1.),(1.,
1.),(1.,1.),(1.,1.),(1.,1.),(1.,1.),(1.,1.),(1.,1.),(1.,1.),(1.,1.),(1.,
1.),(1.,1.),(1.,1.),(1.,1.),(1.,1.),(1.,1.),(1.,1.),(1.,1.),(1.,1.),(1.,
1.),(1.,1.),(1.,1.),(1.,1.),(1.,1.),(1.,1.),(1.,1.),(1.,1.),(1.,1.),(1.,
1.),(1.,1.),(1.,1.),(1.,1.),(1.,1.),(1.,1.),(1.,1.),(1.,1.),(1.,1.),(1.,
1.),(1.,1.)))
REPRESENTATION_ITEM('')
SURFACE()
);
#81=(
BOUNDED_SURFACE()
B_SPLINE_SURFACE(5,1,((#42636,#42637),(#42638,#42639),(#42640,#42641),(#42642,
#42643),(#42644,#42645),(#42646,#42647),(#42648,#42649),(#42650,#42651),
(#42652,#42653),(#42654,#42655),(#42656,#42657),(#42658,#42659),(#42660,
#42661),(#42662,#42663),(#42664,#42665),(#42666,#42667),(#42668,#42669),
(#42670,#42671),(#42672,#42673),(#42674,#42675),(#42676,#42677),(#42678,
#42679),(#42680,#42681),(#42682,#42683),(#42684,#42685),(#42686,#42687),
(#42688,#42689),(#42690,#42691),(#42692,#42693),(#42694,#42695),(#42696,
#42697),(#42698,#42699),(#42700,#42701),(#42702,#42703),(#42704,#42705),
(#42706,#42707),(#42708,#42709),(#42710,#42711),(#42712,#42713),(#42714,
#42715),(#42716,#42717),(#42718,#42719),(#42720,#42721),(#42722,#42723),
(#42724,#42725),(#42726,#42727),(#42728,#42729),(#42730,#42731),(#42732,
#42733),(#42734,#42735),(#42736,#42737),(#42738,#42739),(#42740,#42741),
(#42742,#42743),(#42744,#42745),(#42746,#42747),(#42748,#42749),(#42750,
#42751),(#42752,#42753),(#42754,#42755),(#42756,#42757),(#42758,#42759),
(#42760,#42761),(#42762,#42763),(#42764,#42765),(#42766,#42767),(#42768,
#42769),(#42770,#42771),(#42772,#42773),(#42774,#42775)),.UNSPECIFIED.,
 .F.,.F.,.F.)
B_SPLINE_SURFACE_WITH_KNOTS((6,1,1,1,1,1,1,1,1,1,1,1,1,1,1,1,1,1,1,1,1,
1,1,1,1,1,1,1,1,1,1,1,1,1,1,1,1,1,1,1,1,1,1,1,1,1,1,1,1,1,1,1,1,1,1,1,1,
1,1,1,1,1,1,1,1,6),(2,2),(-1.,-0.984615384615383,-0.969230769230768,-0.953846153846152,
-0.938461538461537,-0.923076923076922,-0.907692307692306,-0.892307692307691,
-0.876923076923076,-0.86153846153846,-0.846153846153845,-0.83076923076923,
-0.815384615384614,-0.799999999999999,-0.784615384615384,-0.769230769230768,
-0.753846153846153,-0.738461538461538,-0.723076923076922,-0.707692307692307,
-0.692307692307692,-0.676923076923076,-0.661538461538461,-0.646153846153846,
-0.63076923076923,-0.615384615384615,-0.6,-0.584615384615384,-0.569230769230769,
-0.553846153846154,-0.538461538461538,-0.523076923076923,-0.507692307692308,
-0.492307692307692,-0.476923076923077,-0.461538461538462,-0.446153846153846,
-0.430769230769231,-0.415384615384615,-0.4,-0.384615384615385,-0.369230769230769,
-0.353846153846154,-0.338461538461538,-0.323076923076923,-0.307692307692308,
-0.292307692307692,-0.276923076923077,-0.261538461538462,-0.246153846153846,
-0.230769230769231,-0.215384615384615,-0.2,-0.184615384615385,-0.169230769230769,
-0.153846153846154,-0.138461538461538,-0.123076923076923,-0.107692307692308,
-0.0923076923076923,-0.0769230769230769,-0.0615384615384615,-0.0461538461538462,
-0.0307692307692308,-0.0153846153846154,0.),(-1.,1.),.UNSPECIFIED.)
GEOMETRIC_REPRESENTATION_ITEM()
RATIONAL_B_SPLINE_SURFACE(((1.,1.),(1.,1.),(1.,1.),(1.,1.),(1.,1.),(1.,
1.),(1.,1.),(1.,1.),(1.,1.),(1.,1.),(1.,1.),(1.,1.),(1.,1.),(1.,1.),(1.,
1.),(1.,1.),(1.,1.),(1.,1.),(1.,1.),(1.,1.),(1.,1.),(1.,1.),(1.,1.),(1.,
1.),(1.,1.),(1.,1.),(1.,1.),(1.,1.),(1.,1.),(1.,1.),(1.,1.),(1.,1.),(1.,
1.),(1.,1.),(1.,1.),(1.,1.),(1.,1.),(1.,1.),(1.,1.),(1.,1.),(1.,1.),(1.,
1.),(1.,1.),(1.,1.),(1.,1.),(1.,1.),(1.,1.),(1.,1.),(1.,1.),(1.,1.),(1.,
1.),(1.,1.),(1.,1.),(1.,1.),(1.,1.),(1.,1.),(1.,1.),(1.,1.),(1.,1.),(1.,
1.),(1.,1.),(1.,1.),(1.,1.),(1.,1.),(1.,1.),(1.,1.),(1.,1.),(1.,1.),(1.,
1.),(1.,1.)))
REPRESENTATION_ITEM('')
SURFACE()
);
#82=(
BOUNDED_SURFACE()
B_SPLINE_SURFACE(5,1,((#42848,#42849),(#42850,#42851),(#42852,#42853),(#42854,
#42855),(#42856,#42857),(#42858,#42859),(#42860,#42861),(#42862,#42863),
(#42864,#42865),(#42866,#42867),(#42868,#42869),(#42870,#42871),(#42872,
#42873),(#42874,#42875),(#42876,#42877),(#42878,#42879),(#42880,#42881),
(#42882,#42883),(#42884,#42885),(#42886,#42887),(#42888,#42889),(#42890,
#42891),(#42892,#42893),(#42894,#42895),(#42896,#42897),(#42898,#42899),
(#42900,#42901),(#42902,#42903),(#42904,#42905),(#42906,#42907),(#42908,
#42909),(#42910,#42911),(#42912,#42913),(#42914,#42915),(#42916,#42917),
(#42918,#42919),(#42920,#42921),(#42922,#42923),(#42924,#42925),(#42926,
#42927),(#42928,#42929),(#42930,#42931),(#42932,#42933),(#42934,#42935),
(#42936,#42937),(#42938,#42939),(#42940,#42941),(#42942,#42943),(#42944,
#42945),(#42946,#42947),(#42948,#42949),(#42950,#42951),(#42952,#42953),
(#42954,#42955),(#42956,#42957),(#42958,#42959),(#42960,#42961),(#42962,
#42963),(#42964,#42965),(#42966,#42967),(#42968,#42969),(#42970,#42971),
(#42972,#42973),(#42974,#42975),(#42976,#42977),(#42978,#42979),(#42980,
#42981),(#42982,#42983),(#42984,#42985),(#42986,#42987)),.UNSPECIFIED.,
 .F.,.F.,.F.)
B_SPLINE_SURFACE_WITH_KNOTS((6,1,1,1,1,1,1,1,1,1,1,1,1,1,1,1,1,1,1,1,1,
1,1,1,1,1,1,1,1,1,1,1,1,1,1,1,1,1,1,1,1,1,1,1,1,1,1,1,1,1,1,1,1,1,1,1,1,
1,1,1,1,1,1,1,1,6),(2,2),(-1.,-0.984615384615383,-0.969230769230768,-0.953846153846152,
-0.938461538461537,-0.923076923076922,-0.907692307692306,-0.892307692307691,
-0.876923076923076,-0.86153846153846,-0.846153846153845,-0.83076923076923,
-0.815384615384614,-0.799999999999999,-0.784615384615384,-0.769230769230768,
-0.753846153846153,-0.738461538461538,-0.723076923076922,-0.707692307692307,
-0.692307692307692,-0.676923076923076,-0.661538461538461,-0.646153846153846,
-0.63076923076923,-0.615384615384615,-0.6,-0.584615384615384,-0.569230769230769,
-0.553846153846154,-0.538461538461538,-0.523076923076923,-0.507692307692308,
-0.492307692307692,-0.476923076923077,-0.461538461538462,-0.446153846153846,
-0.430769230769231,-0.415384615384615,-0.4,-0.384615384615385,-0.369230769230769,
-0.353846153846154,-0.338461538461538,-0.323076923076923,-0.307692307692308,
-0.292307692307692,-0.276923076923077,-0.261538461538462,-0.246153846153846,
-0.230769230769231,-0.215384615384615,-0.2,-0.184615384615385,-0.169230769230769,
-0.153846153846154,-0.138461538461538,-0.123076923076923,-0.107692307692308,
-0.0923076923076923,-0.0769230769230769,-0.0615384615384615,-0.0461538461538462,
-0.0307692307692308,-0.0153846153846154,0.),(-1.,1.),.UNSPECIFIED.)
GEOMETRIC_REPRESENTATION_ITEM()
RATIONAL_B_SPLINE_SURFACE(((1.,1.),(1.,1.),(1.,1.),(1.,1.),(1.,1.),(1.,
1.),(1.,1.),(1.,1.),(1.,1.),(1.,1.),(1.,1.),(1.,1.),(1.,1.),(1.,1.),(1.,
1.),(1.,1.),(1.,1.),(1.,1.),(1.,1.),(1.,1.),(1.,1.),(1.,1.),(1.,1.),(1.,
1.),(1.,1.),(1.,1.),(1.,1.),(1.,1.),(1.,1.),(1.,1.),(1.,1.),(1.,1.),(1.,
1.),(1.,1.),(1.,1.),(1.,1.),(1.,1.),(1.,1.),(1.,1.),(1.,1.),(1.,1.),(1.,
1.),(1.,1.),(1.,1.),(1.,1.),(1.,1.),(1.,1.),(1.,1.),(1.,1.),(1.,1.),(1.,
1.),(1.,1.),(1.,1.),(1.,1.),(1.,1.),(1.,1.),(1.,1.),(1.,1.),(1.,1.),(1.,
1.),(1.,1.),(1.,1.),(1.,1.),(1.,1.),(1.,1.),(1.,1.),(1.,1.),(1.,1.),(1.,
1.),(1.,1.)))
REPRESENTATION_ITEM('')
SURFACE()
);
#83=(
BOUNDED_SURFACE()
B_SPLINE_SURFACE(5,1,((#43078,#43079),(#43080,#43081),(#43082,#43083),(#43084,
#43085),(#43086,#43087),(#43088,#43089),(#43090,#43091),(#43092,#43093),
(#43094,#43095),(#43096,#43097),(#43098,#43099),(#43100,#43101),(#43102,
#43103),(#43104,#43105),(#43106,#43107),(#43108,#43109),(#43110,#43111),
(#43112,#43113),(#43114,#43115),(#43116,#43117),(#43118,#43119),(#43120,
#43121),(#43122,#43123),(#43124,#43125),(#43126,#43127),(#43128,#43129),
(#43130,#43131),(#43132,#43133),(#43134,#43135),(#43136,#43137),(#43138,
#43139),(#43140,#43141),(#43142,#43143),(#43144,#43145),(#43146,#43147),
(#43148,#43149),(#43150,#43151),(#43152,#43153),(#43154,#43155),(#43156,
#43157),(#43158,#43159),(#43160,#43161),(#43162,#43163),(#43164,#43165),
(#43166,#43167),(#43168,#43169),(#43170,#43171),(#43172,#43173),(#43174,
#43175),(#43176,#43177),(#43178,#43179),(#43180,#43181),(#43182,#43183),
(#43184,#43185),(#43186,#43187),(#43188,#43189),(#43190,#43191),(#43192,
#43193),(#43194,#43195),(#43196,#43197),(#43198,#43199),(#43200,#43201),
(#43202,#43203),(#43204,#43205),(#43206,#43207),(#43208,#43209),(#43210,
#43211),(#43212,#43213),(#43214,#43215),(#43216,#43217)),.UNSPECIFIED.,
 .F.,.F.,.F.)
B_SPLINE_SURFACE_WITH_KNOTS((6,1,1,1,1,1,1,1,1,1,1,1,1,1,1,1,1,1,1,1,1,
1,1,1,1,1,1,1,1,1,1,1,1,1,1,1,1,1,1,1,1,1,1,1,1,1,1,1,1,1,1,1,1,1,1,1,1,
1,1,1,1,1,1,1,1,6),(2,2),(-1.,-0.984615384615383,-0.969230769230768,-0.953846153846152,
-0.938461538461537,-0.923076923076922,-0.907692307692306,-0.892307692307691,
-0.876923076923076,-0.86153846153846,-0.846153846153845,-0.83076923076923,
-0.815384615384614,-0.799999999999999,-0.784615384615384,-0.769230769230768,
-0.753846153846153,-0.738461538461538,-0.723076923076922,-0.707692307692307,
-0.692307692307692,-0.676923076923076,-0.661538461538461,-0.646153846153846,
-0.63076923076923,-0.615384615384615,-0.6,-0.584615384615384,-0.569230769230769,
-0.553846153846154,-0.538461538461538,-0.523076923076923,-0.507692307692308,
-0.492307692307692,-0.476923076923077,-0.461538461538462,-0.446153846153846,
-0.430769230769231,-0.415384615384615,-0.4,-0.384615384615385,-0.369230769230769,
-0.353846153846154,-0.338461538461538,-0.323076923076923,-0.307692307692308,
-0.292307692307692,-0.276923076923077,-0.261538461538462,-0.246153846153846,
-0.230769230769231,-0.215384615384615,-0.2,-0.184615384615385,-0.169230769230769,
-0.153846153846154,-0.138461538461538,-0.123076923076923,-0.107692307692308,
-0.0923076923076923,-0.0769230769230769,-0.0615384615384615,-0.0461538461538462,
-0.0307692307692308,-0.0153846153846154,0.),(-1.,1.),.UNSPECIFIED.)
GEOMETRIC_REPRESENTATION_ITEM()
RATIONAL_B_SPLINE_SURFACE(((1.,1.),(1.,1.),(1.,1.),(1.,1.),(1.,1.),(1.,
1.),(1.,1.),(1.,1.),(1.,1.),(1.,1.),(1.,1.),(1.,1.),(1.,1.),(1.,1.),(1.,
1.),(1.,1.),(1.,1.),(1.,1.),(1.,1.),(1.,1.),(1.,1.),(1.,1.),(1.,1.),(1.,
1.),(1.,1.),(1.,1.),(1.,1.),(1.,1.),(1.,1.),(1.,1.),(1.,1.),(1.,1.),(1.,
1.),(1.,1.),(1.,1.),(1.,1.),(1.,1.),(1.,1.),(1.,1.),(1.,1.),(1.,1.),(1.,
1.),(1.,1.),(1.,1.),(1.,1.),(1.,1.),(1.,1.),(1.,1.),(1.,1.),(1.,1.),(1.,
1.),(1.,1.),(1.,1.),(1.,1.),(1.,1.),(1.,1.),(1.,1.),(1.,1.),(1.,1.),(1.,
1.),(1.,1.),(1.,1.),(1.,1.),(1.,1.),(1.,1.),(1.,1.),(1.,1.),(1.,1.),(1.,
1.),(1.,1.)))
REPRESENTATION_ITEM('')
SURFACE()
);
#84=(
BOUNDED_SURFACE()
B_SPLINE_SURFACE(5,1,((#43290,#43291),(#43292,#43293),(#43294,#43295),(#43296,
#43297),(#43298,#43299),(#43300,#43301),(#43302,#43303),(#43304,#43305),
(#43306,#43307),(#43308,#43309),(#43310,#43311),(#43312,#43313),(#43314,
#43315),(#43316,#43317),(#43318,#43319),(#43320,#43321),(#43322,#43323),
(#43324,#43325),(#43326,#43327),(#43328,#43329),(#43330,#43331),(#43332,
#43333),(#43334,#43335),(#43336,#43337),(#43338,#43339),(#43340,#43341),
(#43342,#43343),(#43344,#43345),(#43346,#43347),(#43348,#43349),(#43350,
#43351),(#43352,#43353),(#43354,#43355),(#43356,#43357),(#43358,#43359),
(#43360,#43361),(#43362,#43363),(#43364,#43365),(#43366,#43367),(#43368,
#43369),(#43370,#43371),(#43372,#43373),(#43374,#43375),(#43376,#43377),
(#43378,#43379),(#43380,#43381),(#43382,#43383),(#43384,#43385),(#43386,
#43387),(#43388,#43389),(#43390,#43391),(#43392,#43393),(#43394,#43395),
(#43396,#43397),(#43398,#43399),(#43400,#43401),(#43402,#43403),(#43404,
#43405),(#43406,#43407),(#43408,#43409),(#43410,#43411),(#43412,#43413),
(#43414,#43415),(#43416,#43417),(#43418,#43419),(#43420,#43421),(#43422,
#43423),(#43424,#43425),(#43426,#43427),(#43428,#43429)),.UNSPECIFIED.,
 .F.,.F.,.F.)
B_SPLINE_SURFACE_WITH_KNOTS((6,1,1,1,1,1,1,1,1,1,1,1,1,1,1,1,1,1,1,1,1,
1,1,1,1,1,1,1,1,1,1,1,1,1,1,1,1,1,1,1,1,1,1,1,1,1,1,1,1,1,1,1,1,1,1,1,1,
1,1,1,1,1,1,1,1,6),(2,2),(-1.,-0.984615384615383,-0.969230769230768,-0.953846153846152,
-0.938461538461537,-0.923076923076922,-0.907692307692306,-0.892307692307691,
-0.876923076923076,-0.86153846153846,-0.846153846153845,-0.83076923076923,
-0.815384615384614,-0.799999999999999,-0.784615384615384,-0.769230769230768,
-0.753846153846153,-0.738461538461538,-0.723076923076922,-0.707692307692307,
-0.692307692307692,-0.676923076923076,-0.661538461538461,-0.646153846153846,
-0.63076923076923,-0.615384615384615,-0.6,-0.584615384615384,-0.569230769230769,
-0.553846153846154,-0.538461538461538,-0.523076923076923,-0.507692307692308,
-0.492307692307692,-0.476923076923077,-0.461538461538462,-0.446153846153846,
-0.430769230769231,-0.415384615384615,-0.4,-0.384615384615385,-0.369230769230769,
-0.353846153846154,-0.338461538461538,-0.323076923076923,-0.307692307692308,
-0.292307692307692,-0.276923076923077,-0.261538461538462,-0.246153846153846,
-0.230769230769231,-0.215384615384615,-0.2,-0.184615384615385,-0.169230769230769,
-0.153846153846154,-0.138461538461538,-0.123076923076923,-0.107692307692308,
-0.0923076923076923,-0.0769230769230769,-0.0615384615384615,-0.0461538461538462,
-0.0307692307692308,-0.0153846153846154,0.),(-1.,1.),.UNSPECIFIED.)
GEOMETRIC_REPRESENTATION_ITEM()
RATIONAL_B_SPLINE_SURFACE(((1.,1.),(1.,1.),(1.,1.),(1.,1.),(1.,1.),(1.,
1.),(1.,1.),(1.,1.),(1.,1.),(1.,1.),(1.,1.),(1.,1.),(1.,1.),(1.,1.),(1.,
1.),(1.,1.),(1.,1.),(1.,1.),(1.,1.),(1.,1.),(1.,1.),(1.,1.),(1.,1.),(1.,
1.),(1.,1.),(1.,1.),(1.,1.),(1.,1.),(1.,1.),(1.,1.),(1.,1.),(1.,1.),(1.,
1.),(1.,1.),(1.,1.),(1.,1.),(1.,1.),(1.,1.),(1.,1.),(1.,1.),(1.,1.),(1.,
1.),(1.,1.),(1.,1.),(1.,1.),(1.,1.),(1.,1.),(1.,1.),(1.,1.),(1.,1.),(1.,
1.),(1.,1.),(1.,1.),(1.,1.),(1.,1.),(1.,1.),(1.,1.),(1.,1.),(1.,1.),(1.,
1.),(1.,1.),(1.,1.),(1.,1.),(1.,1.),(1.,1.),(1.,1.),(1.,1.),(1.,1.),(1.,
1.),(1.,1.)))
REPRESENTATION_ITEM('')
SURFACE()
);
#85=(
BOUNDED_SURFACE()
B_SPLINE_SURFACE(5,1,((#43520,#43521),(#43522,#43523),(#43524,#43525),(#43526,
#43527),(#43528,#43529),(#43530,#43531),(#43532,#43533),(#43534,#43535),
(#43536,#43537),(#43538,#43539),(#43540,#43541),(#43542,#43543),(#43544,
#43545),(#43546,#43547),(#43548,#43549),(#43550,#43551),(#43552,#43553),
(#43554,#43555),(#43556,#43557),(#43558,#43559),(#43560,#43561),(#43562,
#43563),(#43564,#43565),(#43566,#43567),(#43568,#43569),(#43570,#43571),
(#43572,#43573),(#43574,#43575),(#43576,#43577),(#43578,#43579),(#43580,
#43581),(#43582,#43583),(#43584,#43585),(#43586,#43587),(#43588,#43589),
(#43590,#43591),(#43592,#43593),(#43594,#43595),(#43596,#43597),(#43598,
#43599),(#43600,#43601),(#43602,#43603),(#43604,#43605),(#43606,#43607),
(#43608,#43609),(#43610,#43611),(#43612,#43613),(#43614,#43615),(#43616,
#43617),(#43618,#43619),(#43620,#43621),(#43622,#43623),(#43624,#43625),
(#43626,#43627),(#43628,#43629),(#43630,#43631),(#43632,#43633),(#43634,
#43635),(#43636,#43637),(#43638,#43639),(#43640,#43641),(#43642,#43643),
(#43644,#43645),(#43646,#43647),(#43648,#43649),(#43650,#43651),(#43652,
#43653),(#43654,#43655),(#43656,#43657),(#43658,#43659)),.UNSPECIFIED.,
 .F.,.F.,.F.)
B_SPLINE_SURFACE_WITH_KNOTS((6,1,1,1,1,1,1,1,1,1,1,1,1,1,1,1,1,1,1,1,1,
1,1,1,1,1,1,1,1,1,1,1,1,1,1,1,1,1,1,1,1,1,1,1,1,1,1,1,1,1,1,1,1,1,1,1,1,
1,1,1,1,1,1,1,1,6),(2,2),(-1.,-0.984615384615383,-0.969230769230768,-0.953846153846152,
-0.938461538461537,-0.923076923076922,-0.907692307692306,-0.892307692307691,
-0.876923076923076,-0.86153846153846,-0.846153846153845,-0.83076923076923,
-0.815384615384614,-0.799999999999999,-0.784615384615384,-0.769230769230768,
-0.753846153846153,-0.738461538461538,-0.723076923076922,-0.707692307692307,
-0.692307692307692,-0.676923076923076,-0.661538461538461,-0.646153846153846,
-0.63076923076923,-0.615384615384615,-0.6,-0.584615384615384,-0.569230769230769,
-0.553846153846154,-0.538461538461538,-0.523076923076923,-0.507692307692308,
-0.492307692307692,-0.476923076923077,-0.461538461538462,-0.446153846153846,
-0.430769230769231,-0.415384615384615,-0.4,-0.384615384615385,-0.369230769230769,
-0.353846153846154,-0.338461538461538,-0.323076923076923,-0.307692307692308,
-0.292307692307692,-0.276923076923077,-0.261538461538462,-0.246153846153846,
-0.230769230769231,-0.215384615384615,-0.2,-0.184615384615385,-0.169230769230769,
-0.153846153846154,-0.138461538461538,-0.123076923076923,-0.107692307692308,
-0.0923076923076923,-0.0769230769230769,-0.0615384615384615,-0.0461538461538462,
-0.0307692307692308,-0.0153846153846154,0.),(-1.,1.),.UNSPECIFIED.)
GEOMETRIC_REPRESENTATION_ITEM()
RATIONAL_B_SPLINE_SURFACE(((1.,1.),(1.,1.),(1.,1.),(1.,1.),(1.,1.),(1.,
1.),(1.,1.),(1.,1.),(1.,1.),(1.,1.),(1.,1.),(1.,1.),(1.,1.),(1.,1.),(1.,
1.),(1.,1.),(1.,1.),(1.,1.),(1.,1.),(1.,1.),(1.,1.),(1.,1.),(1.,1.),(1.,
1.),(1.,1.),(1.,1.),(1.,1.),(1.,1.),(1.,1.),(1.,1.),(1.,1.),(1.,1.),(1.,
1.),(1.,1.),(1.,1.),(1.,1.),(1.,1.),(1.,1.),(1.,1.),(1.,1.),(1.,1.),(1.,
1.),(1.,1.),(1.,1.),(1.,1.),(1.,1.),(1.,1.),(1.,1.),(1.,1.),(1.,1.),(1.,
1.),(1.,1.),(1.,1.),(1.,1.),(1.,1.),(1.,1.),(1.,1.),(1.,1.),(1.,1.),(1.,
1.),(1.,1.),(1.,1.),(1.,1.),(1.,1.),(1.,1.),(1.,1.),(1.,1.),(1.,1.),(1.,
1.),(1.,1.)))
REPRESENTATION_ITEM('')
SURFACE()
);
#86=(
BOUNDED_SURFACE()
B_SPLINE_SURFACE(5,1,((#43732,#43733),(#43734,#43735),(#43736,#43737),(#43738,
#43739),(#43740,#43741),(#43742,#43743),(#43744,#43745),(#43746,#43747),
(#43748,#43749),(#43750,#43751),(#43752,#43753),(#43754,#43755),(#43756,
#43757),(#43758,#43759),(#43760,#43761),(#43762,#43763),(#43764,#43765),
(#43766,#43767),(#43768,#43769),(#43770,#43771),(#43772,#43773),(#43774,
#43775),(#43776,#43777),(#43778,#43779),(#43780,#43781),(#43782,#43783),
(#43784,#43785),(#43786,#43787),(#43788,#43789),(#43790,#43791),(#43792,
#43793),(#43794,#43795),(#43796,#43797),(#43798,#43799),(#43800,#43801),
(#43802,#43803),(#43804,#43805),(#43806,#43807),(#43808,#43809),(#43810,
#43811),(#43812,#43813),(#43814,#43815),(#43816,#43817),(#43818,#43819),
(#43820,#43821),(#43822,#43823),(#43824,#43825),(#43826,#43827),(#43828,
#43829),(#43830,#43831),(#43832,#43833),(#43834,#43835),(#43836,#43837),
(#43838,#43839),(#43840,#43841),(#43842,#43843),(#43844,#43845),(#43846,
#43847),(#43848,#43849),(#43850,#43851),(#43852,#43853),(#43854,#43855),
(#43856,#43857),(#43858,#43859),(#43860,#43861),(#43862,#43863),(#43864,
#43865),(#43866,#43867),(#43868,#43869),(#43870,#43871)),.UNSPECIFIED.,
 .F.,.F.,.F.)
B_SPLINE_SURFACE_WITH_KNOTS((6,1,1,1,1,1,1,1,1,1,1,1,1,1,1,1,1,1,1,1,1,
1,1,1,1,1,1,1,1,1,1,1,1,1,1,1,1,1,1,1,1,1,1,1,1,1,1,1,1,1,1,1,1,1,1,1,1,
1,1,1,1,1,1,1,1,6),(2,2),(-1.,-0.984615384615383,-0.969230769230768,-0.953846153846152,
-0.938461538461537,-0.923076923076922,-0.907692307692306,-0.892307692307691,
-0.876923076923076,-0.86153846153846,-0.846153846153845,-0.83076923076923,
-0.815384615384614,-0.799999999999999,-0.784615384615384,-0.769230769230768,
-0.753846153846153,-0.738461538461538,-0.723076923076922,-0.707692307692307,
-0.692307692307692,-0.676923076923076,-0.661538461538461,-0.646153846153846,
-0.63076923076923,-0.615384615384615,-0.6,-0.584615384615384,-0.569230769230769,
-0.553846153846154,-0.538461538461538,-0.523076923076923,-0.507692307692308,
-0.492307692307692,-0.476923076923077,-0.461538461538462,-0.446153846153846,
-0.430769230769231,-0.415384615384615,-0.4,-0.384615384615385,-0.369230769230769,
-0.353846153846154,-0.338461538461538,-0.323076923076923,-0.307692307692308,
-0.292307692307692,-0.276923076923077,-0.261538461538462,-0.246153846153846,
-0.230769230769231,-0.215384615384615,-0.2,-0.184615384615385,-0.169230769230769,
-0.153846153846154,-0.138461538461538,-0.123076923076923,-0.107692307692308,
-0.0923076923076923,-0.0769230769230769,-0.0615384615384615,-0.0461538461538462,
-0.0307692307692308,-0.0153846153846154,0.),(-1.,1.),.UNSPECIFIED.)
GEOMETRIC_REPRESENTATION_ITEM()
RATIONAL_B_SPLINE_SURFACE(((1.,1.),(1.,1.),(1.,1.),(1.,1.),(1.,1.),(1.,
1.),(1.,1.),(1.,1.),(1.,1.),(1.,1.),(1.,1.),(1.,1.),(1.,1.),(1.,1.),(1.,
1.),(1.,1.),(1.,1.),(1.,1.),(1.,1.),(1.,1.),(1.,1.),(1.,1.),(1.,1.),(1.,
1.),(1.,1.),(1.,1.),(1.,1.),(1.,1.),(1.,1.),(1.,1.),(1.,1.),(1.,1.),(1.,
1.),(1.,1.),(1.,1.),(1.,1.),(1.,1.),(1.,1.),(1.,1.),(1.,1.),(1.,1.),(1.,
1.),(1.,1.),(1.,1.),(1.,1.),(1.,1.),(1.,1.),(1.,1.),(1.,1.),(1.,1.),(1.,
1.),(1.,1.),(1.,1.),(1.,1.),(1.,1.),(1.,1.),(1.,1.),(1.,1.),(1.,1.),(1.,
1.),(1.,1.),(1.,1.),(1.,1.),(1.,1.),(1.,1.),(1.,1.),(1.,1.),(1.,1.),(1.,
1.),(1.,1.)))
REPRESENTATION_ITEM('')
SURFACE()
);
#87=(
BOUNDED_SURFACE()
B_SPLINE_SURFACE(5,1,((#43962,#43963),(#43964,#43965),(#43966,#43967),(#43968,
#43969),(#43970,#43971),(#43972,#43973),(#43974,#43975),(#43976,#43977),
(#43978,#43979),(#43980,#43981),(#43982,#43983),(#43984,#43985),(#43986,
#43987),(#43988,#43989),(#43990,#43991),(#43992,#43993),(#43994,#43995),
(#43996,#43997),(#43998,#43999),(#44000,#44001),(#44002,#44003),(#44004,
#44005),(#44006,#44007),(#44008,#44009),(#44010,#44011),(#44012,#44013),
(#44014,#44015),(#44016,#44017),(#44018,#44019),(#44020,#44021),(#44022,
#44023),(#44024,#44025),(#44026,#44027),(#44028,#44029),(#44030,#44031),
(#44032,#44033),(#44034,#44035),(#44036,#44037),(#44038,#44039),(#44040,
#44041),(#44042,#44043),(#44044,#44045),(#44046,#44047),(#44048,#44049),
(#44050,#44051),(#44052,#44053),(#44054,#44055),(#44056,#44057),(#44058,
#44059),(#44060,#44061),(#44062,#44063),(#44064,#44065),(#44066,#44067),
(#44068,#44069),(#44070,#44071),(#44072,#44073),(#44074,#44075),(#44076,
#44077),(#44078,#44079),(#44080,#44081),(#44082,#44083),(#44084,#44085),
(#44086,#44087),(#44088,#44089),(#44090,#44091),(#44092,#44093),(#44094,
#44095),(#44096,#44097),(#44098,#44099),(#44100,#44101)),.UNSPECIFIED.,
 .F.,.F.,.F.)
B_SPLINE_SURFACE_WITH_KNOTS((6,1,1,1,1,1,1,1,1,1,1,1,1,1,1,1,1,1,1,1,1,
1,1,1,1,1,1,1,1,1,1,1,1,1,1,1,1,1,1,1,1,1,1,1,1,1,1,1,1,1,1,1,1,1,1,1,1,
1,1,1,1,1,1,1,1,6),(2,2),(-1.,-0.984615384615383,-0.969230769230768,-0.953846153846152,
-0.938461538461537,-0.923076923076922,-0.907692307692306,-0.892307692307691,
-0.876923076923076,-0.86153846153846,-0.846153846153845,-0.83076923076923,
-0.815384615384614,-0.799999999999999,-0.784615384615384,-0.769230769230768,
-0.753846153846153,-0.738461538461538,-0.723076923076922,-0.707692307692307,
-0.692307692307692,-0.676923076923076,-0.661538461538461,-0.646153846153846,
-0.63076923076923,-0.615384615384615,-0.6,-0.584615384615384,-0.569230769230769,
-0.553846153846154,-0.538461538461538,-0.523076923076923,-0.507692307692308,
-0.492307692307692,-0.476923076923077,-0.461538461538462,-0.446153846153846,
-0.430769230769231,-0.415384615384615,-0.4,-0.384615384615385,-0.369230769230769,
-0.353846153846154,-0.338461538461538,-0.323076923076923,-0.307692307692308,
-0.292307692307692,-0.276923076923077,-0.261538461538462,-0.246153846153846,
-0.230769230769231,-0.215384615384615,-0.2,-0.184615384615385,-0.169230769230769,
-0.153846153846154,-0.138461538461538,-0.123076923076923,-0.107692307692308,
-0.0923076923076923,-0.0769230769230769,-0.0615384615384615,-0.0461538461538462,
-0.0307692307692308,-0.0153846153846154,0.),(-1.,1.),.UNSPECIFIED.)
GEOMETRIC_REPRESENTATION_ITEM()
RATIONAL_B_SPLINE_SURFACE(((1.,1.),(1.,1.),(1.,1.),(1.,1.),(1.,1.),(1.,
1.),(1.,1.),(1.,1.),(1.,1.),(1.,1.),(1.,1.),(1.,1.),(1.,1.),(1.,1.),(1.,
1.),(1.,1.),(1.,1.),(1.,1.),(1.,1.),(1.,1.),(1.,1.),(1.,1.),(1.,1.),(1.,
1.),(1.,1.),(1.,1.),(1.,1.),(1.,1.),(1.,1.),(1.,1.),(1.,1.),(1.,1.),(1.,
1.),(1.,1.),(1.,1.),(1.,1.),(1.,1.),(1.,1.),(1.,1.),(1.,1.),(1.,1.),(1.,
1.),(1.,1.),(1.,1.),(1.,1.),(1.,1.),(1.,1.),(1.,1.),(1.,1.),(1.,1.),(1.,
1.),(1.,1.),(1.,1.),(1.,1.),(1.,1.),(1.,1.),(1.,1.),(1.,1.),(1.,1.),(1.,
1.),(1.,1.),(1.,1.),(1.,1.),(1.,1.),(1.,1.),(1.,1.),(1.,1.),(1.,1.),(1.,
1.),(1.,1.)))
REPRESENTATION_ITEM('')
SURFACE()
);
#88=(
BOUNDED_SURFACE()
B_SPLINE_SURFACE(5,1,((#44174,#44175),(#44176,#44177),(#44178,#44179),(#44180,
#44181),(#44182,#44183),(#44184,#44185),(#44186,#44187),(#44188,#44189),
(#44190,#44191),(#44192,#44193),(#44194,#44195),(#44196,#44197),(#44198,
#44199),(#44200,#44201),(#44202,#44203),(#44204,#44205),(#44206,#44207),
(#44208,#44209),(#44210,#44211),(#44212,#44213),(#44214,#44215),(#44216,
#44217),(#44218,#44219),(#44220,#44221),(#44222,#44223),(#44224,#44225),
(#44226,#44227),(#44228,#44229),(#44230,#44231),(#44232,#44233),(#44234,
#44235),(#44236,#44237),(#44238,#44239),(#44240,#44241),(#44242,#44243),
(#44244,#44245),(#44246,#44247),(#44248,#44249),(#44250,#44251),(#44252,
#44253),(#44254,#44255),(#44256,#44257),(#44258,#44259),(#44260,#44261),
(#44262,#44263),(#44264,#44265),(#44266,#44267),(#44268,#44269),(#44270,
#44271),(#44272,#44273),(#44274,#44275),(#44276,#44277),(#44278,#44279),
(#44280,#44281),(#44282,#44283),(#44284,#44285),(#44286,#44287),(#44288,
#44289),(#44290,#44291),(#44292,#44293),(#44294,#44295),(#44296,#44297),
(#44298,#44299),(#44300,#44301),(#44302,#44303),(#44304,#44305),(#44306,
#44307),(#44308,#44309),(#44310,#44311),(#44312,#44313)),.UNSPECIFIED.,
 .F.,.F.,.F.)
B_SPLINE_SURFACE_WITH_KNOTS((6,1,1,1,1,1,1,1,1,1,1,1,1,1,1,1,1,1,1,1,1,
1,1,1,1,1,1,1,1,1,1,1,1,1,1,1,1,1,1,1,1,1,1,1,1,1,1,1,1,1,1,1,1,1,1,1,1,
1,1,1,1,1,1,1,1,6),(2,2),(-1.,-0.984615384615383,-0.969230769230768,-0.953846153846152,
-0.938461538461537,-0.923076923076922,-0.907692307692306,-0.892307692307691,
-0.876923076923076,-0.86153846153846,-0.846153846153845,-0.83076923076923,
-0.815384615384614,-0.799999999999999,-0.784615384615384,-0.769230769230768,
-0.753846153846153,-0.738461538461538,-0.723076923076922,-0.707692307692307,
-0.692307692307692,-0.676923076923076,-0.661538461538461,-0.646153846153846,
-0.63076923076923,-0.615384615384615,-0.6,-0.584615384615384,-0.569230769230769,
-0.553846153846154,-0.538461538461538,-0.523076923076923,-0.507692307692308,
-0.492307692307692,-0.476923076923077,-0.461538461538462,-0.446153846153846,
-0.430769230769231,-0.415384615384615,-0.4,-0.384615384615385,-0.369230769230769,
-0.353846153846154,-0.338461538461538,-0.323076923076923,-0.307692307692308,
-0.292307692307692,-0.276923076923077,-0.261538461538462,-0.246153846153846,
-0.230769230769231,-0.215384615384615,-0.2,-0.184615384615385,-0.169230769230769,
-0.153846153846154,-0.138461538461538,-0.123076923076923,-0.107692307692308,
-0.0923076923076923,-0.0769230769230769,-0.0615384615384615,-0.0461538461538462,
-0.0307692307692308,-0.0153846153846154,0.),(-1.,1.),.UNSPECIFIED.)
GEOMETRIC_REPRESENTATION_ITEM()
RATIONAL_B_SPLINE_SURFACE(((1.,1.),(1.,1.),(1.,1.),(1.,1.),(1.,1.),(1.,
1.),(1.,1.),(1.,1.),(1.,1.),(1.,1.),(1.,1.),(1.,1.),(1.,1.),(1.,1.),(1.,
1.),(1.,1.),(1.,1.),(1.,1.),(1.,1.),(1.,1.),(1.,1.),(1.,1.),(1.,1.),(1.,
1.),(1.,1.),(1.,1.),(1.,1.),(1.,1.),(1.,1.),(1.,1.),(1.,1.),(1.,1.),(1.,
1.),(1.,1.),(1.,1.),(1.,1.),(1.,1.),(1.,1.),(1.,1.),(1.,1.),(1.,1.),(1.,
1.),(1.,1.),(1.,1.),(1.,1.),(1.,1.),(1.,1.),(1.,1.),(1.,1.),(1.,1.),(1.,
1.),(1.,1.),(1.,1.),(1.,1.),(1.,1.),(1.,1.),(1.,1.),(1.,1.),(1.,1.),(1.,
1.),(1.,1.),(1.,1.),(1.,1.),(1.,1.),(1.,1.),(1.,1.),(1.,1.),(1.,1.),(1.,
1.),(1.,1.)))
REPRESENTATION_ITEM('')
SURFACE()
);
#89=(
BOUNDED_SURFACE()
B_SPLINE_SURFACE(5,1,((#44404,#44405),(#44406,#44407),(#44408,#44409),(#44410,
#44411),(#44412,#44413),(#44414,#44415),(#44416,#44417),(#44418,#44419),
(#44420,#44421),(#44422,#44423),(#44424,#44425),(#44426,#44427),(#44428,
#44429),(#44430,#44431),(#44432,#44433),(#44434,#44435),(#44436,#44437),
(#44438,#44439),(#44440,#44441),(#44442,#44443),(#44444,#44445),(#44446,
#44447),(#44448,#44449),(#44450,#44451),(#44452,#44453),(#44454,#44455),
(#44456,#44457),(#44458,#44459),(#44460,#44461),(#44462,#44463),(#44464,
#44465),(#44466,#44467),(#44468,#44469),(#44470,#44471),(#44472,#44473),
(#44474,#44475),(#44476,#44477),(#44478,#44479),(#44480,#44481),(#44482,
#44483),(#44484,#44485),(#44486,#44487),(#44488,#44489),(#44490,#44491),
(#44492,#44493),(#44494,#44495),(#44496,#44497),(#44498,#44499),(#44500,
#44501),(#44502,#44503),(#44504,#44505),(#44506,#44507),(#44508,#44509),
(#44510,#44511),(#44512,#44513),(#44514,#44515),(#44516,#44517),(#44518,
#44519),(#44520,#44521),(#44522,#44523),(#44524,#44525),(#44526,#44527),
(#44528,#44529),(#44530,#44531),(#44532,#44533),(#44534,#44535),(#44536,
#44537),(#44538,#44539),(#44540,#44541),(#44542,#44543)),.UNSPECIFIED.,
 .F.,.F.,.F.)
B_SPLINE_SURFACE_WITH_KNOTS((6,1,1,1,1,1,1,1,1,1,1,1,1,1,1,1,1,1,1,1,1,
1,1,1,1,1,1,1,1,1,1,1,1,1,1,1,1,1,1,1,1,1,1,1,1,1,1,1,1,1,1,1,1,1,1,1,1,
1,1,1,1,1,1,1,1,6),(2,2),(-1.,-0.984615384615383,-0.969230769230768,-0.953846153846152,
-0.938461538461537,-0.923076923076922,-0.907692307692306,-0.892307692307691,
-0.876923076923076,-0.86153846153846,-0.846153846153845,-0.83076923076923,
-0.815384615384614,-0.799999999999999,-0.784615384615384,-0.769230769230768,
-0.753846153846153,-0.738461538461538,-0.723076923076922,-0.707692307692307,
-0.692307692307692,-0.676923076923076,-0.661538461538461,-0.646153846153846,
-0.63076923076923,-0.615384615384615,-0.6,-0.584615384615384,-0.569230769230769,
-0.553846153846154,-0.538461538461538,-0.523076923076923,-0.507692307692308,
-0.492307692307692,-0.476923076923077,-0.461538461538462,-0.446153846153846,
-0.430769230769231,-0.415384615384615,-0.4,-0.384615384615385,-0.369230769230769,
-0.353846153846154,-0.338461538461538,-0.323076923076923,-0.307692307692308,
-0.292307692307692,-0.276923076923077,-0.261538461538462,-0.246153846153846,
-0.230769230769231,-0.215384615384615,-0.2,-0.184615384615385,-0.169230769230769,
-0.153846153846154,-0.138461538461538,-0.123076923076923,-0.107692307692308,
-0.0923076923076923,-0.0769230769230769,-0.0615384615384615,-0.0461538461538462,
-0.0307692307692308,-0.0153846153846154,0.),(-1.,1.),.UNSPECIFIED.)
GEOMETRIC_REPRESENTATION_ITEM()
RATIONAL_B_SPLINE_SURFACE(((1.,1.),(1.,1.),(1.,1.),(1.,1.),(1.,1.),(1.,
1.),(1.,1.),(1.,1.),(1.,1.),(1.,1.),(1.,1.),(1.,1.),(1.,1.),(1.,1.),(1.,
1.),(1.,1.),(1.,1.),(1.,1.),(1.,1.),(1.,1.),(1.,1.),(1.,1.),(1.,1.),(1.,
1.),(1.,1.),(1.,1.),(1.,1.),(1.,1.),(1.,1.),(1.,1.),(1.,1.),(1.,1.),(1.,
1.),(1.,1.),(1.,1.),(1.,1.),(1.,1.),(1.,1.),(1.,1.),(1.,1.),(1.,1.),(1.,
1.),(1.,1.),(1.,1.),(1.,1.),(1.,1.),(1.,1.),(1.,1.),(1.,1.),(1.,1.),(1.,
1.),(1.,1.),(1.,1.),(1.,1.),(1.,1.),(1.,1.),(1.,1.),(1.,1.),(1.,1.),(1.,
1.),(1.,1.),(1.,1.),(1.,1.),(1.,1.),(1.,1.),(1.,1.),(1.,1.),(1.,1.),(1.,
1.),(1.,1.)))
REPRESENTATION_ITEM('')
SURFACE()
);
#90=(
BOUNDED_SURFACE()
B_SPLINE_SURFACE(5,1,((#44616,#44617),(#44618,#44619),(#44620,#44621),(#44622,
#44623),(#44624,#44625),(#44626,#44627),(#44628,#44629),(#44630,#44631),
(#44632,#44633),(#44634,#44635),(#44636,#44637),(#44638,#44639),(#44640,
#44641),(#44642,#44643),(#44644,#44645),(#44646,#44647),(#44648,#44649),
(#44650,#44651),(#44652,#44653),(#44654,#44655),(#44656,#44657),(#44658,
#44659),(#44660,#44661),(#44662,#44663),(#44664,#44665),(#44666,#44667),
(#44668,#44669),(#44670,#44671),(#44672,#44673),(#44674,#44675),(#44676,
#44677),(#44678,#44679),(#44680,#44681),(#44682,#44683),(#44684,#44685),
(#44686,#44687),(#44688,#44689),(#44690,#44691),(#44692,#44693),(#44694,
#44695),(#44696,#44697),(#44698,#44699),(#44700,#44701),(#44702,#44703),
(#44704,#44705),(#44706,#44707),(#44708,#44709),(#44710,#44711),(#44712,
#44713),(#44714,#44715),(#44716,#44717),(#44718,#44719),(#44720,#44721),
(#44722,#44723),(#44724,#44725),(#44726,#44727),(#44728,#44729),(#44730,
#44731),(#44732,#44733),(#44734,#44735),(#44736,#44737),(#44738,#44739),
(#44740,#44741),(#44742,#44743),(#44744,#44745),(#44746,#44747),(#44748,
#44749),(#44750,#44751),(#44752,#44753),(#44754,#44755)),.UNSPECIFIED.,
 .F.,.F.,.F.)
B_SPLINE_SURFACE_WITH_KNOTS((6,1,1,1,1,1,1,1,1,1,1,1,1,1,1,1,1,1,1,1,1,
1,1,1,1,1,1,1,1,1,1,1,1,1,1,1,1,1,1,1,1,1,1,1,1,1,1,1,1,1,1,1,1,1,1,1,1,
1,1,1,1,1,1,1,1,6),(2,2),(-1.,-0.984615384615383,-0.969230769230768,-0.953846153846152,
-0.938461538461537,-0.923076923076922,-0.907692307692306,-0.892307692307691,
-0.876923076923076,-0.86153846153846,-0.846153846153845,-0.83076923076923,
-0.815384615384614,-0.799999999999999,-0.784615384615384,-0.769230769230768,
-0.753846153846153,-0.738461538461538,-0.723076923076922,-0.707692307692307,
-0.692307692307692,-0.676923076923076,-0.661538461538461,-0.646153846153846,
-0.63076923076923,-0.615384615384615,-0.6,-0.584615384615384,-0.569230769230769,
-0.553846153846154,-0.538461538461538,-0.523076923076923,-0.507692307692308,
-0.492307692307692,-0.476923076923077,-0.461538461538462,-0.446153846153846,
-0.430769230769231,-0.415384615384615,-0.4,-0.384615384615385,-0.369230769230769,
-0.353846153846154,-0.338461538461538,-0.323076923076923,-0.307692307692308,
-0.292307692307692,-0.276923076923077,-0.261538461538462,-0.246153846153846,
-0.230769230769231,-0.215384615384615,-0.2,-0.184615384615385,-0.169230769230769,
-0.153846153846154,-0.138461538461538,-0.123076923076923,-0.107692307692308,
-0.0923076923076923,-0.0769230769230769,-0.0615384615384615,-0.0461538461538462,
-0.0307692307692308,-0.0153846153846154,0.),(-1.,1.),.UNSPECIFIED.)
GEOMETRIC_REPRESENTATION_ITEM()
RATIONAL_B_SPLINE_SURFACE(((1.,1.),(1.,1.),(1.,1.),(1.,1.),(1.,1.),(1.,
1.),(1.,1.),(1.,1.),(1.,1.),(1.,1.),(1.,1.),(1.,1.),(1.,1.),(1.,1.),(1.,
1.),(1.,1.),(1.,1.),(1.,1.),(1.,1.),(1.,1.),(1.,1.),(1.,1.),(1.,1.),(1.,
1.),(1.,1.),(1.,1.),(1.,1.),(1.,1.),(1.,1.),(1.,1.),(1.,1.),(1.,1.),(1.,
1.),(1.,1.),(1.,1.),(1.,1.),(1.,1.),(1.,1.),(1.,1.),(1.,1.),(1.,1.),(1.,
1.),(1.,1.),(1.,1.),(1.,1.),(1.,1.),(1.,1.),(1.,1.),(1.,1.),(1.,1.),(1.,
1.),(1.,1.),(1.,1.),(1.,1.),(1.,1.),(1.,1.),(1.,1.),(1.,1.),(1.,1.),(1.,
1.),(1.,1.),(1.,1.),(1.,1.),(1.,1.),(1.,1.),(1.,1.),(1.,1.),(1.,1.),(1.,
1.),(1.,1.)))
REPRESENTATION_ITEM('')
SURFACE()
);
#91=(
BOUNDED_SURFACE()
B_SPLINE_SURFACE(5,1,((#44846,#44847),(#44848,#44849),(#44850,#44851),(#44852,
#44853),(#44854,#44855),(#44856,#44857),(#44858,#44859),(#44860,#44861),
(#44862,#44863),(#44864,#44865),(#44866,#44867),(#44868,#44869),(#44870,
#44871),(#44872,#44873),(#44874,#44875),(#44876,#44877),(#44878,#44879),
(#44880,#44881),(#44882,#44883),(#44884,#44885),(#44886,#44887),(#44888,
#44889),(#44890,#44891),(#44892,#44893),(#44894,#44895),(#44896,#44897),
(#44898,#44899),(#44900,#44901),(#44902,#44903),(#44904,#44905),(#44906,
#44907),(#44908,#44909),(#44910,#44911),(#44912,#44913),(#44914,#44915),
(#44916,#44917),(#44918,#44919),(#44920,#44921),(#44922,#44923),(#44924,
#44925),(#44926,#44927),(#44928,#44929),(#44930,#44931),(#44932,#44933),
(#44934,#44935),(#44936,#44937),(#44938,#44939),(#44940,#44941),(#44942,
#44943),(#44944,#44945),(#44946,#44947),(#44948,#44949),(#44950,#44951),
(#44952,#44953),(#44954,#44955),(#44956,#44957),(#44958,#44959),(#44960,
#44961),(#44962,#44963),(#44964,#44965),(#44966,#44967),(#44968,#44969),
(#44970,#44971),(#44972,#44973),(#44974,#44975),(#44976,#44977),(#44978,
#44979),(#44980,#44981),(#44982,#44983),(#44984,#44985)),.UNSPECIFIED.,
 .F.,.F.,.F.)
B_SPLINE_SURFACE_WITH_KNOTS((6,1,1,1,1,1,1,1,1,1,1,1,1,1,1,1,1,1,1,1,1,
1,1,1,1,1,1,1,1,1,1,1,1,1,1,1,1,1,1,1,1,1,1,1,1,1,1,1,1,1,1,1,1,1,1,1,1,
1,1,1,1,1,1,1,1,6),(2,2),(-1.,-0.984615384615383,-0.969230769230768,-0.953846153846152,
-0.938461538461537,-0.923076923076922,-0.907692307692306,-0.892307692307691,
-0.876923076923076,-0.86153846153846,-0.846153846153845,-0.83076923076923,
-0.815384615384614,-0.799999999999999,-0.784615384615384,-0.769230769230768,
-0.753846153846153,-0.738461538461538,-0.723076923076922,-0.707692307692307,
-0.692307692307692,-0.676923076923076,-0.661538461538461,-0.646153846153846,
-0.63076923076923,-0.615384615384615,-0.6,-0.584615384615384,-0.569230769230769,
-0.553846153846154,-0.538461538461538,-0.523076923076923,-0.507692307692308,
-0.492307692307692,-0.476923076923077,-0.461538461538462,-0.446153846153846,
-0.430769230769231,-0.415384615384615,-0.4,-0.384615384615385,-0.369230769230769,
-0.353846153846154,-0.338461538461538,-0.323076923076923,-0.307692307692308,
-0.292307692307692,-0.276923076923077,-0.261538461538462,-0.246153846153846,
-0.230769230769231,-0.215384615384615,-0.2,-0.184615384615385,-0.169230769230769,
-0.153846153846154,-0.138461538461538,-0.123076923076923,-0.107692307692308,
-0.0923076923076923,-0.0769230769230769,-0.0615384615384615,-0.0461538461538462,
-0.0307692307692308,-0.0153846153846154,0.),(-1.,1.),.UNSPECIFIED.)
GEOMETRIC_REPRESENTATION_ITEM()
RATIONAL_B_SPLINE_SURFACE(((1.,1.),(1.,1.),(1.,1.),(1.,1.),(1.,1.),(1.,
1.),(1.,1.),(1.,1.),(1.,1.),(1.,1.),(1.,1.),(1.,1.),(1.,1.),(1.,1.),(1.,
1.),(1.,1.),(1.,1.),(1.,1.),(1.,1.),(1.,1.),(1.,1.),(1.,1.),(1.,1.),(1.,
1.),(1.,1.),(1.,1.),(1.,1.),(1.,1.),(1.,1.),(1.,1.),(1.,1.),(1.,1.),(1.,
1.),(1.,1.),(1.,1.),(1.,1.),(1.,1.),(1.,1.),(1.,1.),(1.,1.),(1.,1.),(1.,
1.),(1.,1.),(1.,1.),(1.,1.),(1.,1.),(1.,1.),(1.,1.),(1.,1.),(1.,1.),(1.,
1.),(1.,1.),(1.,1.),(1.,1.),(1.,1.),(1.,1.),(1.,1.),(1.,1.),(1.,1.),(1.,
1.),(1.,1.),(1.,1.),(1.,1.),(1.,1.),(1.,1.),(1.,1.),(1.,1.),(1.,1.),(1.,
1.),(1.,1.)))
REPRESENTATION_ITEM('')
SURFACE()
);
#92=(
BOUNDED_SURFACE()
B_SPLINE_SURFACE(5,1,((#45058,#45059),(#45060,#45061),(#45062,#45063),(#45064,
#45065),(#45066,#45067),(#45068,#45069),(#45070,#45071),(#45072,#45073),
(#45074,#45075),(#45076,#45077),(#45078,#45079),(#45080,#45081),(#45082,
#45083),(#45084,#45085),(#45086,#45087),(#45088,#45089),(#45090,#45091),
(#45092,#45093),(#45094,#45095),(#45096,#45097),(#45098,#45099),(#45100,
#45101),(#45102,#45103),(#45104,#45105),(#45106,#45107),(#45108,#45109),
(#45110,#45111),(#45112,#45113),(#45114,#45115),(#45116,#45117),(#45118,
#45119),(#45120,#45121),(#45122,#45123),(#45124,#45125),(#45126,#45127),
(#45128,#45129),(#45130,#45131),(#45132,#45133),(#45134,#45135),(#45136,
#45137),(#45138,#45139),(#45140,#45141),(#45142,#45143),(#45144,#45145),
(#45146,#45147),(#45148,#45149),(#45150,#45151),(#45152,#45153),(#45154,
#45155),(#45156,#45157),(#45158,#45159),(#45160,#45161),(#45162,#45163),
(#45164,#45165),(#45166,#45167),(#45168,#45169),(#45170,#45171),(#45172,
#45173),(#45174,#45175),(#45176,#45177),(#45178,#45179),(#45180,#45181),
(#45182,#45183),(#45184,#45185),(#45186,#45187),(#45188,#45189),(#45190,
#45191),(#45192,#45193),(#45194,#45195),(#45196,#45197)),.UNSPECIFIED.,
 .F.,.F.,.F.)
B_SPLINE_SURFACE_WITH_KNOTS((6,1,1,1,1,1,1,1,1,1,1,1,1,1,1,1,1,1,1,1,1,
1,1,1,1,1,1,1,1,1,1,1,1,1,1,1,1,1,1,1,1,1,1,1,1,1,1,1,1,1,1,1,1,1,1,1,1,
1,1,1,1,1,1,1,1,6),(2,2),(-1.,-0.984615384615383,-0.969230769230768,-0.953846153846152,
-0.938461538461537,-0.923076923076922,-0.907692307692306,-0.892307692307691,
-0.876923076923076,-0.86153846153846,-0.846153846153845,-0.83076923076923,
-0.815384615384614,-0.799999999999999,-0.784615384615384,-0.769230769230768,
-0.753846153846153,-0.738461538461538,-0.723076923076922,-0.707692307692307,
-0.692307692307692,-0.676923076923076,-0.661538461538461,-0.646153846153846,
-0.63076923076923,-0.615384615384615,-0.6,-0.584615384615384,-0.569230769230769,
-0.553846153846154,-0.538461538461538,-0.523076923076923,-0.507692307692308,
-0.492307692307692,-0.476923076923077,-0.461538461538462,-0.446153846153846,
-0.430769230769231,-0.415384615384615,-0.4,-0.384615384615385,-0.369230769230769,
-0.353846153846154,-0.338461538461538,-0.323076923076923,-0.307692307692308,
-0.292307692307692,-0.276923076923077,-0.261538461538462,-0.246153846153846,
-0.230769230769231,-0.215384615384615,-0.2,-0.184615384615385,-0.169230769230769,
-0.153846153846154,-0.138461538461538,-0.123076923076923,-0.107692307692308,
-0.0923076923076923,-0.0769230769230769,-0.0615384615384615,-0.0461538461538462,
-0.0307692307692308,-0.0153846153846154,0.),(-1.,1.),.UNSPECIFIED.)
GEOMETRIC_REPRESENTATION_ITEM()
RATIONAL_B_SPLINE_SURFACE(((1.,1.),(1.,1.),(1.,1.),(1.,1.),(1.,1.),(1.,
1.),(1.,1.),(1.,1.),(1.,1.),(1.,1.),(1.,1.),(1.,1.),(1.,1.),(1.,1.),(1.,
1.),(1.,1.),(1.,1.),(1.,1.),(1.,1.),(1.,1.),(1.,1.),(1.,1.),(1.,1.),(1.,
1.),(1.,1.),(1.,1.),(1.,1.),(1.,1.),(1.,1.),(1.,1.),(1.,1.),(1.,1.),(1.,
1.),(1.,1.),(1.,1.),(1.,1.),(1.,1.),(1.,1.),(1.,1.),(1.,1.),(1.,1.),(1.,
1.),(1.,1.),(1.,1.),(1.,1.),(1.,1.),(1.,1.),(1.,1.),(1.,1.),(1.,1.),(1.,
1.),(1.,1.),(1.,1.),(1.,1.),(1.,1.),(1.,1.),(1.,1.),(1.,1.),(1.,1.),(1.,
1.),(1.,1.),(1.,1.),(1.,1.),(1.,1.),(1.,1.),(1.,1.),(1.,1.),(1.,1.),(1.,
1.),(1.,1.)))
REPRESENTATION_ITEM('')
SURFACE()
);
#93=(
BOUNDED_SURFACE()
B_SPLINE_SURFACE(5,1,((#45288,#45289),(#45290,#45291),(#45292,#45293),(#45294,
#45295),(#45296,#45297),(#45298,#45299),(#45300,#45301),(#45302,#45303),
(#45304,#45305),(#45306,#45307),(#45308,#45309),(#45310,#45311),(#45312,
#45313),(#45314,#45315),(#45316,#45317),(#45318,#45319),(#45320,#45321),
(#45322,#45323),(#45324,#45325),(#45326,#45327),(#45328,#45329),(#45330,
#45331),(#45332,#45333),(#45334,#45335),(#45336,#45337),(#45338,#45339),
(#45340,#45341),(#45342,#45343),(#45344,#45345),(#45346,#45347),(#45348,
#45349),(#45350,#45351),(#45352,#45353),(#45354,#45355),(#45356,#45357),
(#45358,#45359),(#45360,#45361),(#45362,#45363),(#45364,#45365),(#45366,
#45367),(#45368,#45369),(#45370,#45371),(#45372,#45373),(#45374,#45375),
(#45376,#45377),(#45378,#45379),(#45380,#45381),(#45382,#45383),(#45384,
#45385),(#45386,#45387),(#45388,#45389),(#45390,#45391),(#45392,#45393),
(#45394,#45395),(#45396,#45397),(#45398,#45399),(#45400,#45401),(#45402,
#45403),(#45404,#45405),(#45406,#45407),(#45408,#45409),(#45410,#45411),
(#45412,#45413),(#45414,#45415),(#45416,#45417),(#45418,#45419),(#45420,
#45421),(#45422,#45423),(#45424,#45425),(#45426,#45427)),.UNSPECIFIED.,
 .F.,.F.,.F.)
B_SPLINE_SURFACE_WITH_KNOTS((6,1,1,1,1,1,1,1,1,1,1,1,1,1,1,1,1,1,1,1,1,
1,1,1,1,1,1,1,1,1,1,1,1,1,1,1,1,1,1,1,1,1,1,1,1,1,1,1,1,1,1,1,1,1,1,1,1,
1,1,1,1,1,1,1,1,6),(2,2),(-1.,-0.984615384615383,-0.969230769230768,-0.953846153846152,
-0.938461538461537,-0.923076923076922,-0.907692307692306,-0.892307692307691,
-0.876923076923076,-0.86153846153846,-0.846153846153845,-0.83076923076923,
-0.815384615384614,-0.799999999999999,-0.784615384615384,-0.769230769230768,
-0.753846153846153,-0.738461538461538,-0.723076923076922,-0.707692307692307,
-0.692307692307692,-0.676923076923076,-0.661538461538461,-0.646153846153846,
-0.63076923076923,-0.615384615384615,-0.6,-0.584615384615384,-0.569230769230769,
-0.553846153846154,-0.538461538461538,-0.523076923076923,-0.507692307692308,
-0.492307692307692,-0.476923076923077,-0.461538461538462,-0.446153846153846,
-0.430769230769231,-0.415384615384615,-0.4,-0.384615384615385,-0.369230769230769,
-0.353846153846154,-0.338461538461538,-0.323076923076923,-0.307692307692308,
-0.292307692307692,-0.276923076923077,-0.261538461538462,-0.246153846153846,
-0.230769230769231,-0.215384615384615,-0.2,-0.184615384615385,-0.169230769230769,
-0.153846153846154,-0.138461538461538,-0.123076923076923,-0.107692307692308,
-0.0923076923076923,-0.0769230769230769,-0.0615384615384615,-0.0461538461538462,
-0.0307692307692308,-0.0153846153846154,0.),(-1.,1.),.UNSPECIFIED.)
GEOMETRIC_REPRESENTATION_ITEM()
RATIONAL_B_SPLINE_SURFACE(((1.,1.),(1.,1.),(1.,1.),(1.,1.),(1.,1.),(1.,
1.),(1.,1.),(1.,1.),(1.,1.),(1.,1.),(1.,1.),(1.,1.),(1.,1.),(1.,1.),(1.,
1.),(1.,1.),(1.,1.),(1.,1.),(1.,1.),(1.,1.),(1.,1.),(1.,1.),(1.,1.),(1.,
1.),(1.,1.),(1.,1.),(1.,1.),(1.,1.),(1.,1.),(1.,1.),(1.,1.),(1.,1.),(1.,
1.),(1.,1.),(1.,1.),(1.,1.),(1.,1.),(1.,1.),(1.,1.),(1.,1.),(1.,1.),(1.,
1.),(1.,1.),(1.,1.),(1.,1.),(1.,1.),(1.,1.),(1.,1.),(1.,1.),(1.,1.),(1.,
1.),(1.,1.),(1.,1.),(1.,1.),(1.,1.),(1.,1.),(1.,1.),(1.,1.),(1.,1.),(1.,
1.),(1.,1.),(1.,1.),(1.,1.),(1.,1.),(1.,1.),(1.,1.),(1.,1.),(1.,1.),(1.,
1.),(1.,1.)))
REPRESENTATION_ITEM('')
SURFACE()
);
#94=(
BOUNDED_SURFACE()
B_SPLINE_SURFACE(5,1,((#45500,#45501),(#45502,#45503),(#45504,#45505),(#45506,
#45507),(#45508,#45509),(#45510,#45511),(#45512,#45513),(#45514,#45515),
(#45516,#45517),(#45518,#45519),(#45520,#45521),(#45522,#45523),(#45524,
#45525),(#45526,#45527),(#45528,#45529),(#45530,#45531),(#45532,#45533),
(#45534,#45535),(#45536,#45537),(#45538,#45539),(#45540,#45541),(#45542,
#45543),(#45544,#45545),(#45546,#45547),(#45548,#45549),(#45550,#45551),
(#45552,#45553),(#45554,#45555),(#45556,#45557),(#45558,#45559),(#45560,
#45561),(#45562,#45563),(#45564,#45565),(#45566,#45567),(#45568,#45569),
(#45570,#45571),(#45572,#45573),(#45574,#45575),(#45576,#45577),(#45578,
#45579),(#45580,#45581),(#45582,#45583),(#45584,#45585),(#45586,#45587),
(#45588,#45589),(#45590,#45591),(#45592,#45593),(#45594,#45595),(#45596,
#45597),(#45598,#45599),(#45600,#45601),(#45602,#45603),(#45604,#45605),
(#45606,#45607),(#45608,#45609),(#45610,#45611),(#45612,#45613),(#45614,
#45615),(#45616,#45617),(#45618,#45619),(#45620,#45621),(#45622,#45623),
(#45624,#45625),(#45626,#45627),(#45628,#45629),(#45630,#45631),(#45632,
#45633),(#45634,#45635),(#45636,#45637),(#45638,#45639)),.UNSPECIFIED.,
 .F.,.F.,.F.)
B_SPLINE_SURFACE_WITH_KNOTS((6,1,1,1,1,1,1,1,1,1,1,1,1,1,1,1,1,1,1,1,1,
1,1,1,1,1,1,1,1,1,1,1,1,1,1,1,1,1,1,1,1,1,1,1,1,1,1,1,1,1,1,1,1,1,1,1,1,
1,1,1,1,1,1,1,1,6),(2,2),(-1.,-0.984615384615383,-0.969230769230768,-0.953846153846152,
-0.938461538461537,-0.923076923076922,-0.907692307692306,-0.892307692307691,
-0.876923076923076,-0.86153846153846,-0.846153846153845,-0.83076923076923,
-0.815384615384614,-0.799999999999999,-0.784615384615384,-0.769230769230768,
-0.753846153846153,-0.738461538461538,-0.723076923076922,-0.707692307692307,
-0.692307692307692,-0.676923076923076,-0.661538461538461,-0.646153846153846,
-0.63076923076923,-0.615384615384615,-0.6,-0.584615384615384,-0.569230769230769,
-0.553846153846154,-0.538461538461538,-0.523076923076923,-0.507692307692308,
-0.492307692307692,-0.476923076923077,-0.461538461538462,-0.446153846153846,
-0.430769230769231,-0.415384615384615,-0.4,-0.384615384615385,-0.369230769230769,
-0.353846153846154,-0.338461538461538,-0.323076923076923,-0.307692307692308,
-0.292307692307692,-0.276923076923077,-0.261538461538462,-0.246153846153846,
-0.230769230769231,-0.215384615384615,-0.2,-0.184615384615385,-0.169230769230769,
-0.153846153846154,-0.138461538461538,-0.123076923076923,-0.107692307692308,
-0.0923076923076923,-0.0769230769230769,-0.0615384615384615,-0.0461538461538462,
-0.0307692307692308,-0.0153846153846154,0.),(-1.,1.),.UNSPECIFIED.)
GEOMETRIC_REPRESENTATION_ITEM()
RATIONAL_B_SPLINE_SURFACE(((1.,1.),(1.,1.),(1.,1.),(1.,1.),(1.,1.),(1.,
1.),(1.,1.),(1.,1.),(1.,1.),(1.,1.),(1.,1.),(1.,1.),(1.,1.),(1.,1.),(1.,
1.),(1.,1.),(1.,1.),(1.,1.),(1.,1.),(1.,1.),(1.,1.),(1.,1.),(1.,1.),(1.,
1.),(1.,1.),(1.,1.),(1.,1.),(1.,1.),(1.,1.),(1.,1.),(1.,1.),(1.,1.),(1.,
1.),(1.,1.),(1.,1.),(1.,1.),(1.,1.),(1.,1.),(1.,1.),(1.,1.),(1.,1.),(1.,
1.),(1.,1.),(1.,1.),(1.,1.),(1.,1.),(1.,1.),(1.,1.),(1.,1.),(1.,1.),(1.,
1.),(1.,1.),(1.,1.),(1.,1.),(1.,1.),(1.,1.),(1.,1.),(1.,1.),(1.,1.),(1.,
1.),(1.,1.),(1.,1.),(1.,1.),(1.,1.),(1.,1.),(1.,1.),(1.,1.),(1.,1.),(1.,
1.),(1.,1.)))
REPRESENTATION_ITEM('')
SURFACE()
);
#95=(
BOUNDED_SURFACE()
B_SPLINE_SURFACE(5,1,((#45730,#45731),(#45732,#45733),(#45734,#45735),(#45736,
#45737),(#45738,#45739),(#45740,#45741),(#45742,#45743),(#45744,#45745),
(#45746,#45747),(#45748,#45749),(#45750,#45751),(#45752,#45753),(#45754,
#45755),(#45756,#45757),(#45758,#45759),(#45760,#45761),(#45762,#45763),
(#45764,#45765),(#45766,#45767),(#45768,#45769),(#45770,#45771),(#45772,
#45773),(#45774,#45775),(#45776,#45777),(#45778,#45779),(#45780,#45781),
(#45782,#45783),(#45784,#45785),(#45786,#45787),(#45788,#45789),(#45790,
#45791),(#45792,#45793),(#45794,#45795),(#45796,#45797),(#45798,#45799),
(#45800,#45801),(#45802,#45803),(#45804,#45805),(#45806,#45807),(#45808,
#45809),(#45810,#45811),(#45812,#45813),(#45814,#45815),(#45816,#45817),
(#45818,#45819),(#45820,#45821),(#45822,#45823),(#45824,#45825),(#45826,
#45827),(#45828,#45829),(#45830,#45831),(#45832,#45833),(#45834,#45835),
(#45836,#45837),(#45838,#45839),(#45840,#45841),(#45842,#45843),(#45844,
#45845),(#45846,#45847),(#45848,#45849),(#45850,#45851),(#45852,#45853),
(#45854,#45855),(#45856,#45857),(#45858,#45859),(#45860,#45861),(#45862,
#45863),(#45864,#45865),(#45866,#45867),(#45868,#45869)),.UNSPECIFIED.,
 .F.,.F.,.F.)
B_SPLINE_SURFACE_WITH_KNOTS((6,1,1,1,1,1,1,1,1,1,1,1,1,1,1,1,1,1,1,1,1,
1,1,1,1,1,1,1,1,1,1,1,1,1,1,1,1,1,1,1,1,1,1,1,1,1,1,1,1,1,1,1,1,1,1,1,1,
1,1,1,1,1,1,1,1,6),(2,2),(-1.,-0.984615384615383,-0.969230769230768,-0.953846153846152,
-0.938461538461537,-0.923076923076922,-0.907692307692306,-0.892307692307691,
-0.876923076923076,-0.86153846153846,-0.846153846153845,-0.83076923076923,
-0.815384615384614,-0.799999999999999,-0.784615384615384,-0.769230769230768,
-0.753846153846153,-0.738461538461538,-0.723076923076922,-0.707692307692307,
-0.692307692307692,-0.676923076923076,-0.661538461538461,-0.646153846153846,
-0.63076923076923,-0.615384615384615,-0.6,-0.584615384615384,-0.569230769230769,
-0.553846153846154,-0.538461538461538,-0.523076923076923,-0.507692307692308,
-0.492307692307692,-0.476923076923077,-0.461538461538462,-0.446153846153846,
-0.430769230769231,-0.415384615384615,-0.4,-0.384615384615385,-0.369230769230769,
-0.353846153846154,-0.338461538461538,-0.323076923076923,-0.307692307692308,
-0.292307692307692,-0.276923076923077,-0.261538461538462,-0.246153846153846,
-0.230769230769231,-0.215384615384615,-0.2,-0.184615384615385,-0.169230769230769,
-0.153846153846154,-0.138461538461538,-0.123076923076923,-0.107692307692308,
-0.0923076923076923,-0.0769230769230769,-0.0615384615384615,-0.0461538461538462,
-0.0307692307692308,-0.0153846153846154,0.),(-1.,1.),.UNSPECIFIED.)
GEOMETRIC_REPRESENTATION_ITEM()
RATIONAL_B_SPLINE_SURFACE(((1.,1.),(1.,1.),(1.,1.),(1.,1.),(1.,1.),(1.,
1.),(1.,1.),(1.,1.),(1.,1.),(1.,1.),(1.,1.),(1.,1.),(1.,1.),(1.,1.),(1.,
1.),(1.,1.),(1.,1.),(1.,1.),(1.,1.),(1.,1.),(1.,1.),(1.,1.),(1.,1.),(1.,
1.),(1.,1.),(1.,1.),(1.,1.),(1.,1.),(1.,1.),(1.,1.),(1.,1.),(1.,1.),(1.,
1.),(1.,1.),(1.,1.),(1.,1.),(1.,1.),(1.,1.),(1.,1.),(1.,1.),(1.,1.),(1.,
1.),(1.,1.),(1.,1.),(1.,1.),(1.,1.),(1.,1.),(1.,1.),(1.,1.),(1.,1.),(1.,
1.),(1.,1.),(1.,1.),(1.,1.),(1.,1.),(1.,1.),(1.,1.),(1.,1.),(1.,1.),(1.,
1.),(1.,1.),(1.,1.),(1.,1.),(1.,1.),(1.,1.),(1.,1.),(1.,1.),(1.,1.),(1.,
1.),(1.,1.)))
REPRESENTATION_ITEM('')
SURFACE()
);
#96=(
BOUNDED_SURFACE()
B_SPLINE_SURFACE(5,1,((#45942,#45943),(#45944,#45945),(#45946,#45947),(#45948,
#45949),(#45950,#45951),(#45952,#45953),(#45954,#45955),(#45956,#45957),
(#45958,#45959),(#45960,#45961),(#45962,#45963),(#45964,#45965),(#45966,
#45967),(#45968,#45969),(#45970,#45971),(#45972,#45973),(#45974,#45975),
(#45976,#45977),(#45978,#45979),(#45980,#45981),(#45982,#45983),(#45984,
#45985),(#45986,#45987),(#45988,#45989),(#45990,#45991),(#45992,#45993),
(#45994,#45995),(#45996,#45997),(#45998,#45999),(#46000,#46001),(#46002,
#46003),(#46004,#46005),(#46006,#46007),(#46008,#46009),(#46010,#46011),
(#46012,#46013),(#46014,#46015),(#46016,#46017),(#46018,#46019),(#46020,
#46021),(#46022,#46023),(#46024,#46025),(#46026,#46027),(#46028,#46029),
(#46030,#46031),(#46032,#46033),(#46034,#46035),(#46036,#46037),(#46038,
#46039),(#46040,#46041),(#46042,#46043),(#46044,#46045),(#46046,#46047),
(#46048,#46049),(#46050,#46051),(#46052,#46053),(#46054,#46055),(#46056,
#46057),(#46058,#46059),(#46060,#46061),(#46062,#46063),(#46064,#46065),
(#46066,#46067),(#46068,#46069),(#46070,#46071),(#46072,#46073),(#46074,
#46075),(#46076,#46077),(#46078,#46079),(#46080,#46081)),.UNSPECIFIED.,
 .F.,.F.,.F.)
B_SPLINE_SURFACE_WITH_KNOTS((6,1,1,1,1,1,1,1,1,1,1,1,1,1,1,1,1,1,1,1,1,
1,1,1,1,1,1,1,1,1,1,1,1,1,1,1,1,1,1,1,1,1,1,1,1,1,1,1,1,1,1,1,1,1,1,1,1,
1,1,1,1,1,1,1,1,6),(2,2),(-1.,-0.984615384615383,-0.969230769230768,-0.953846153846152,
-0.938461538461537,-0.923076923076922,-0.907692307692306,-0.892307692307691,
-0.876923076923076,-0.86153846153846,-0.846153846153845,-0.83076923076923,
-0.815384615384614,-0.799999999999999,-0.784615384615384,-0.769230769230768,
-0.753846153846153,-0.738461538461538,-0.723076923076922,-0.707692307692307,
-0.692307692307692,-0.676923076923076,-0.661538461538461,-0.646153846153846,
-0.63076923076923,-0.615384615384615,-0.6,-0.584615384615384,-0.569230769230769,
-0.553846153846154,-0.538461538461538,-0.523076923076923,-0.507692307692308,
-0.492307692307692,-0.476923076923077,-0.461538461538462,-0.446153846153846,
-0.430769230769231,-0.415384615384615,-0.4,-0.384615384615385,-0.369230769230769,
-0.353846153846154,-0.338461538461538,-0.323076923076923,-0.307692307692308,
-0.292307692307692,-0.276923076923077,-0.261538461538462,-0.246153846153846,
-0.230769230769231,-0.215384615384615,-0.2,-0.184615384615385,-0.169230769230769,
-0.153846153846154,-0.138461538461538,-0.123076923076923,-0.107692307692308,
-0.0923076923076923,-0.0769230769230769,-0.0615384615384615,-0.0461538461538462,
-0.0307692307692308,-0.0153846153846154,0.),(-1.,1.),.UNSPECIFIED.)
GEOMETRIC_REPRESENTATION_ITEM()
RATIONAL_B_SPLINE_SURFACE(((1.,1.),(1.,1.),(1.,1.),(1.,1.),(1.,1.),(1.,
1.),(1.,1.),(1.,1.),(1.,1.),(1.,1.),(1.,1.),(1.,1.),(1.,1.),(1.,1.),(1.,
1.),(1.,1.),(1.,1.),(1.,1.),(1.,1.),(1.,1.),(1.,1.),(1.,1.),(1.,1.),(1.,
1.),(1.,1.),(1.,1.),(1.,1.),(1.,1.),(1.,1.),(1.,1.),(1.,1.),(1.,1.),(1.,
1.),(1.,1.),(1.,1.),(1.,1.),(1.,1.),(1.,1.),(1.,1.),(1.,1.),(1.,1.),(1.,
1.),(1.,1.),(1.,1.),(1.,1.),(1.,1.),(1.,1.),(1.,1.),(1.,1.),(1.,1.),(1.,
1.),(1.,1.),(1.,1.),(1.,1.),(1.,1.),(1.,1.),(1.,1.),(1.,1.),(1.,1.),(1.,
1.),(1.,1.),(1.,1.),(1.,1.),(1.,1.),(1.,1.),(1.,1.),(1.,1.),(1.,1.),(1.,
1.),(1.,1.)))
REPRESENTATION_ITEM('')
SURFACE()
);
#97=(
BOUNDED_SURFACE()
B_SPLINE_SURFACE(5,1,((#46172,#46173),(#46174,#46175),(#46176,#46177),(#46178,
#46179),(#46180,#46181),(#46182,#46183),(#46184,#46185),(#46186,#46187),
(#46188,#46189),(#46190,#46191),(#46192,#46193),(#46194,#46195),(#46196,
#46197),(#46198,#46199),(#46200,#46201),(#46202,#46203),(#46204,#46205),
(#46206,#46207),(#46208,#46209),(#46210,#46211),(#46212,#46213),(#46214,
#46215),(#46216,#46217),(#46218,#46219),(#46220,#46221),(#46222,#46223),
(#46224,#46225),(#46226,#46227),(#46228,#46229),(#46230,#46231),(#46232,
#46233),(#46234,#46235),(#46236,#46237),(#46238,#46239),(#46240,#46241),
(#46242,#46243),(#46244,#46245),(#46246,#46247),(#46248,#46249),(#46250,
#46251),(#46252,#46253),(#46254,#46255),(#46256,#46257),(#46258,#46259),
(#46260,#46261),(#46262,#46263),(#46264,#46265),(#46266,#46267),(#46268,
#46269),(#46270,#46271),(#46272,#46273),(#46274,#46275),(#46276,#46277),
(#46278,#46279),(#46280,#46281),(#46282,#46283),(#46284,#46285),(#46286,
#46287),(#46288,#46289),(#46290,#46291),(#46292,#46293),(#46294,#46295),
(#46296,#46297),(#46298,#46299),(#46300,#46301),(#46302,#46303),(#46304,
#46305),(#46306,#46307),(#46308,#46309),(#46310,#46311)),.UNSPECIFIED.,
 .F.,.F.,.F.)
B_SPLINE_SURFACE_WITH_KNOTS((6,1,1,1,1,1,1,1,1,1,1,1,1,1,1,1,1,1,1,1,1,
1,1,1,1,1,1,1,1,1,1,1,1,1,1,1,1,1,1,1,1,1,1,1,1,1,1,1,1,1,1,1,1,1,1,1,1,
1,1,1,1,1,1,1,1,6),(2,2),(-1.,-0.984615384615383,-0.969230769230768,-0.953846153846152,
-0.938461538461537,-0.923076923076922,-0.907692307692306,-0.892307692307691,
-0.876923076923076,-0.86153846153846,-0.846153846153845,-0.83076923076923,
-0.815384615384614,-0.799999999999999,-0.784615384615384,-0.769230769230768,
-0.753846153846153,-0.738461538461538,-0.723076923076922,-0.707692307692307,
-0.692307692307692,-0.676923076923076,-0.661538461538461,-0.646153846153846,
-0.63076923076923,-0.615384615384615,-0.6,-0.584615384615384,-0.569230769230769,
-0.553846153846154,-0.538461538461538,-0.523076923076923,-0.507692307692308,
-0.492307692307692,-0.476923076923077,-0.461538461538462,-0.446153846153846,
-0.430769230769231,-0.415384615384615,-0.4,-0.384615384615385,-0.369230769230769,
-0.353846153846154,-0.338461538461538,-0.323076923076923,-0.307692307692308,
-0.292307692307692,-0.276923076923077,-0.261538461538462,-0.246153846153846,
-0.230769230769231,-0.215384615384615,-0.2,-0.184615384615385,-0.169230769230769,
-0.153846153846154,-0.138461538461538,-0.123076923076923,-0.107692307692308,
-0.0923076923076923,-0.0769230769230769,-0.0615384615384615,-0.0461538461538462,
-0.0307692307692308,-0.0153846153846154,0.),(-1.,1.),.UNSPECIFIED.)
GEOMETRIC_REPRESENTATION_ITEM()
RATIONAL_B_SPLINE_SURFACE(((1.,1.),(1.,1.),(1.,1.),(1.,1.),(1.,1.),(1.,
1.),(1.,1.),(1.,1.),(1.,1.),(1.,1.),(1.,1.),(1.,1.),(1.,1.),(1.,1.),(1.,
1.),(1.,1.),(1.,1.),(1.,1.),(1.,1.),(1.,1.),(1.,1.),(1.,1.),(1.,1.),(1.,
1.),(1.,1.),(1.,1.),(1.,1.),(1.,1.),(1.,1.),(1.,1.),(1.,1.),(1.,1.),(1.,
1.),(1.,1.),(1.,1.),(1.,1.),(1.,1.),(1.,1.),(1.,1.),(1.,1.),(1.,1.),(1.,
1.),(1.,1.),(1.,1.),(1.,1.),(1.,1.),(1.,1.),(1.,1.),(1.,1.),(1.,1.),(1.,
1.),(1.,1.),(1.,1.),(1.,1.),(1.,1.),(1.,1.),(1.,1.),(1.,1.),(1.,1.),(1.,
1.),(1.,1.),(1.,1.),(1.,1.),(1.,1.),(1.,1.),(1.,1.),(1.,1.),(1.,1.),(1.,
1.),(1.,1.)))
REPRESENTATION_ITEM('')
SURFACE()
);
#98=(
BOUNDED_SURFACE()
B_SPLINE_SURFACE(5,1,((#46384,#46385),(#46386,#46387),(#46388,#46389),(#46390,
#46391),(#46392,#46393),(#46394,#46395),(#46396,#46397),(#46398,#46399),
(#46400,#46401),(#46402,#46403),(#46404,#46405),(#46406,#46407),(#46408,
#46409),(#46410,#46411),(#46412,#46413),(#46414,#46415),(#46416,#46417),
(#46418,#46419),(#46420,#46421),(#46422,#46423),(#46424,#46425),(#46426,
#46427),(#46428,#46429),(#46430,#46431),(#46432,#46433),(#46434,#46435),
(#46436,#46437),(#46438,#46439),(#46440,#46441),(#46442,#46443),(#46444,
#46445),(#46446,#46447),(#46448,#46449),(#46450,#46451),(#46452,#46453),
(#46454,#46455),(#46456,#46457),(#46458,#46459),(#46460,#46461),(#46462,
#46463),(#46464,#46465),(#46466,#46467),(#46468,#46469),(#46470,#46471),
(#46472,#46473),(#46474,#46475),(#46476,#46477),(#46478,#46479),(#46480,
#46481),(#46482,#46483),(#46484,#46485),(#46486,#46487),(#46488,#46489),
(#46490,#46491),(#46492,#46493),(#46494,#46495),(#46496,#46497),(#46498,
#46499),(#46500,#46501),(#46502,#46503),(#46504,#46505),(#46506,#46507),
(#46508,#46509),(#46510,#46511),(#46512,#46513),(#46514,#46515),(#46516,
#46517),(#46518,#46519),(#46520,#46521),(#46522,#46523)),.UNSPECIFIED.,
 .F.,.F.,.F.)
B_SPLINE_SURFACE_WITH_KNOTS((6,1,1,1,1,1,1,1,1,1,1,1,1,1,1,1,1,1,1,1,1,
1,1,1,1,1,1,1,1,1,1,1,1,1,1,1,1,1,1,1,1,1,1,1,1,1,1,1,1,1,1,1,1,1,1,1,1,
1,1,1,1,1,1,1,1,6),(2,2),(-1.,-0.984615384615383,-0.969230769230768,-0.953846153846152,
-0.938461538461537,-0.923076923076922,-0.907692307692306,-0.892307692307691,
-0.876923076923076,-0.86153846153846,-0.846153846153845,-0.83076923076923,
-0.815384615384614,-0.799999999999999,-0.784615384615384,-0.769230769230768,
-0.753846153846153,-0.738461538461538,-0.723076923076922,-0.707692307692307,
-0.692307692307692,-0.676923076923076,-0.661538461538461,-0.646153846153846,
-0.63076923076923,-0.615384615384615,-0.6,-0.584615384615384,-0.569230769230769,
-0.553846153846154,-0.538461538461538,-0.523076923076923,-0.507692307692308,
-0.492307692307692,-0.476923076923077,-0.461538461538462,-0.446153846153846,
-0.430769230769231,-0.415384615384615,-0.4,-0.384615384615385,-0.369230769230769,
-0.353846153846154,-0.338461538461538,-0.323076923076923,-0.307692307692308,
-0.292307692307692,-0.276923076923077,-0.261538461538462,-0.246153846153846,
-0.230769230769231,-0.215384615384615,-0.2,-0.184615384615385,-0.169230769230769,
-0.153846153846154,-0.138461538461538,-0.123076923076923,-0.107692307692308,
-0.0923076923076923,-0.0769230769230769,-0.0615384615384615,-0.0461538461538462,
-0.0307692307692308,-0.0153846153846154,0.),(-1.,1.),.UNSPECIFIED.)
GEOMETRIC_REPRESENTATION_ITEM()
RATIONAL_B_SPLINE_SURFACE(((1.,1.),(1.,1.),(1.,1.),(1.,1.),(1.,1.),(1.,
1.),(1.,1.),(1.,1.),(1.,1.),(1.,1.),(1.,1.),(1.,1.),(1.,1.),(1.,1.),(1.,
1.),(1.,1.),(1.,1.),(1.,1.),(1.,1.),(1.,1.),(1.,1.),(1.,1.),(1.,1.),(1.,
1.),(1.,1.),(1.,1.),(1.,1.),(1.,1.),(1.,1.),(1.,1.),(1.,1.),(1.,1.),(1.,
1.),(1.,1.),(1.,1.),(1.,1.),(1.,1.),(1.,1.),(1.,1.),(1.,1.),(1.,1.),(1.,
1.),(1.,1.),(1.,1.),(1.,1.),(1.,1.),(1.,1.),(1.,1.),(1.,1.),(1.,1.),(1.,
1.),(1.,1.),(1.,1.),(1.,1.),(1.,1.),(1.,1.),(1.,1.),(1.,1.),(1.,1.),(1.,
1.),(1.,1.),(1.,1.),(1.,1.),(1.,1.),(1.,1.),(1.,1.),(1.,1.),(1.,1.),(1.,
1.),(1.,1.)))
REPRESENTATION_ITEM('')
SURFACE()
);
#99=(
BOUNDED_SURFACE()
B_SPLINE_SURFACE(5,1,((#46614,#46615),(#46616,#46617),(#46618,#46619),(#46620,
#46621),(#46622,#46623),(#46624,#46625),(#46626,#46627),(#46628,#46629),
(#46630,#46631),(#46632,#46633),(#46634,#46635),(#46636,#46637),(#46638,
#46639),(#46640,#46641),(#46642,#46643),(#46644,#46645),(#46646,#46647),
(#46648,#46649),(#46650,#46651),(#46652,#46653),(#46654,#46655),(#46656,
#46657),(#46658,#46659),(#46660,#46661),(#46662,#46663),(#46664,#46665),
(#46666,#46667),(#46668,#46669),(#46670,#46671),(#46672,#46673),(#46674,
#46675),(#46676,#46677),(#46678,#46679),(#46680,#46681),(#46682,#46683),
(#46684,#46685),(#46686,#46687),(#46688,#46689),(#46690,#46691),(#46692,
#46693),(#46694,#46695),(#46696,#46697),(#46698,#46699),(#46700,#46701),
(#46702,#46703),(#46704,#46705),(#46706,#46707),(#46708,#46709),(#46710,
#46711),(#46712,#46713),(#46714,#46715),(#46716,#46717),(#46718,#46719),
(#46720,#46721),(#46722,#46723),(#46724,#46725),(#46726,#46727),(#46728,
#46729),(#46730,#46731),(#46732,#46733),(#46734,#46735),(#46736,#46737),
(#46738,#46739),(#46740,#46741),(#46742,#46743),(#46744,#46745),(#46746,
#46747),(#46748,#46749),(#46750,#46751),(#46752,#46753)),.UNSPECIFIED.,
 .F.,.F.,.F.)
B_SPLINE_SURFACE_WITH_KNOTS((6,1,1,1,1,1,1,1,1,1,1,1,1,1,1,1,1,1,1,1,1,
1,1,1,1,1,1,1,1,1,1,1,1,1,1,1,1,1,1,1,1,1,1,1,1,1,1,1,1,1,1,1,1,1,1,1,1,
1,1,1,1,1,1,1,1,6),(2,2),(-1.,-0.984615384615383,-0.969230769230768,-0.953846153846152,
-0.938461538461537,-0.923076923076922,-0.907692307692306,-0.892307692307691,
-0.876923076923076,-0.86153846153846,-0.846153846153845,-0.83076923076923,
-0.815384615384614,-0.799999999999999,-0.784615384615384,-0.769230769230768,
-0.753846153846153,-0.738461538461538,-0.723076923076922,-0.707692307692307,
-0.692307692307692,-0.676923076923076,-0.661538461538461,-0.646153846153846,
-0.63076923076923,-0.615384615384615,-0.6,-0.584615384615384,-0.569230769230769,
-0.553846153846154,-0.538461538461538,-0.523076923076923,-0.507692307692308,
-0.492307692307692,-0.476923076923077,-0.461538461538462,-0.446153846153846,
-0.430769230769231,-0.415384615384615,-0.4,-0.384615384615385,-0.369230769230769,
-0.353846153846154,-0.338461538461538,-0.323076923076923,-0.307692307692308,
-0.292307692307692,-0.276923076923077,-0.261538461538462,-0.246153846153846,
-0.230769230769231,-0.215384615384615,-0.2,-0.184615384615385,-0.169230769230769,
-0.153846153846154,-0.138461538461538,-0.123076923076923,-0.107692307692308,
-0.0923076923076923,-0.0769230769230769,-0.0615384615384615,-0.0461538461538462,
-0.0307692307692308,-0.0153846153846154,0.),(-1.,1.),.UNSPECIFIED.)
GEOMETRIC_REPRESENTATION_ITEM()
RATIONAL_B_SPLINE_SURFACE(((1.,1.),(1.,1.),(1.,1.),(1.,1.),(1.,1.),(1.,
1.),(1.,1.),(1.,1.),(1.,1.),(1.,1.),(1.,1.),(1.,1.),(1.,1.),(1.,1.),(1.,
1.),(1.,1.),(1.,1.),(1.,1.),(1.,1.),(1.,1.),(1.,1.),(1.,1.),(1.,1.),(1.,
1.),(1.,1.),(1.,1.),(1.,1.),(1.,1.),(1.,1.),(1.,1.),(1.,1.),(1.,1.),(1.,
1.),(1.,1.),(1.,1.),(1.,1.),(1.,1.),(1.,1.),(1.,1.),(1.,1.),(1.,1.),(1.,
1.),(1.,1.),(1.,1.),(1.,1.),(1.,1.),(1.,1.),(1.,1.),(1.,1.),(1.,1.),(1.,
1.),(1.,1.),(1.,1.),(1.,1.),(1.,1.),(1.,1.),(1.,1.),(1.,1.),(1.,1.),(1.,
1.),(1.,1.),(1.,1.),(1.,1.),(1.,1.),(1.,1.),(1.,1.),(1.,1.),(1.,1.),(1.,
1.),(1.,1.)))
REPRESENTATION_ITEM('')
SURFACE()
);
#100=(
BOUNDED_SURFACE()
B_SPLINE_SURFACE(5,1,((#46826,#46827),(#46828,#46829),(#46830,#46831),(#46832,
#46833),(#46834,#46835),(#46836,#46837),(#46838,#46839),(#46840,#46841),
(#46842,#46843),(#46844,#46845),(#46846,#46847),(#46848,#46849),(#46850,
#46851),(#46852,#46853),(#46854,#46855),(#46856,#46857),(#46858,#46859),
(#46860,#46861),(#46862,#46863),(#46864,#46865),(#46866,#46867),(#46868,
#46869),(#46870,#46871),(#46872,#46873),(#46874,#46875),(#46876,#46877),
(#46878,#46879),(#46880,#46881),(#46882,#46883),(#46884,#46885),(#46886,
#46887),(#46888,#46889),(#46890,#46891),(#46892,#46893),(#46894,#46895),
(#46896,#46897),(#46898,#46899),(#46900,#46901),(#46902,#46903),(#46904,
#46905),(#46906,#46907),(#46908,#46909),(#46910,#46911),(#46912,#46913),
(#46914,#46915),(#46916,#46917),(#46918,#46919),(#46920,#46921),(#46922,
#46923),(#46924,#46925),(#46926,#46927),(#46928,#46929),(#46930,#46931),
(#46932,#46933),(#46934,#46935),(#46936,#46937),(#46938,#46939),(#46940,
#46941),(#46942,#46943),(#46944,#46945),(#46946,#46947),(#46948,#46949),
(#46950,#46951),(#46952,#46953),(#46954,#46955),(#46956,#46957),(#46958,
#46959),(#46960,#46961),(#46962,#46963),(#46964,#46965)),.UNSPECIFIED.,
 .F.,.F.,.F.)
B_SPLINE_SURFACE_WITH_KNOTS((6,1,1,1,1,1,1,1,1,1,1,1,1,1,1,1,1,1,1,1,1,
1,1,1,1,1,1,1,1,1,1,1,1,1,1,1,1,1,1,1,1,1,1,1,1,1,1,1,1,1,1,1,1,1,1,1,1,
1,1,1,1,1,1,1,1,6),(2,2),(-1.,-0.984615384615383,-0.969230769230768,-0.953846153846152,
-0.938461538461537,-0.923076923076922,-0.907692307692306,-0.892307692307691,
-0.876923076923076,-0.86153846153846,-0.846153846153845,-0.83076923076923,
-0.815384615384614,-0.799999999999999,-0.784615384615384,-0.769230769230768,
-0.753846153846153,-0.738461538461538,-0.723076923076922,-0.707692307692307,
-0.692307692307692,-0.676923076923076,-0.661538461538461,-0.646153846153846,
-0.63076923076923,-0.615384615384615,-0.6,-0.584615384615384,-0.569230769230769,
-0.553846153846154,-0.538461538461538,-0.523076923076923,-0.507692307692308,
-0.492307692307692,-0.476923076923077,-0.461538461538462,-0.446153846153846,
-0.430769230769231,-0.415384615384615,-0.4,-0.384615384615385,-0.369230769230769,
-0.353846153846154,-0.338461538461538,-0.323076923076923,-0.307692307692308,
-0.292307692307692,-0.276923076923077,-0.261538461538462,-0.246153846153846,
-0.230769230769231,-0.215384615384615,-0.2,-0.184615384615385,-0.169230769230769,
-0.153846153846154,-0.138461538461538,-0.123076923076923,-0.107692307692308,
-0.0923076923076923,-0.0769230769230769,-0.0615384615384615,-0.0461538461538462,
-0.0307692307692308,-0.0153846153846154,0.),(-1.,1.),.UNSPECIFIED.)
GEOMETRIC_REPRESENTATION_ITEM()
RATIONAL_B_SPLINE_SURFACE(((1.,1.),(1.,1.),(1.,1.),(1.,1.),(1.,1.),(1.,
1.),(1.,1.),(1.,1.),(1.,1.),(1.,1.),(1.,1.),(1.,1.),(1.,1.),(1.,1.),(1.,
1.),(1.,1.),(1.,1.),(1.,1.),(1.,1.),(1.,1.),(1.,1.),(1.,1.),(1.,1.),(1.,
1.),(1.,1.),(1.,1.),(1.,1.),(1.,1.),(1.,1.),(1.,1.),(1.,1.),(1.,1.),(1.,
1.),(1.,1.),(1.,1.),(1.,1.),(1.,1.),(1.,1.),(1.,1.),(1.,1.),(1.,1.),(1.,
1.),(1.,1.),(1.,1.),(1.,1.),(1.,1.),(1.,1.),(1.,1.),(1.,1.),(1.,1.),(1.,
1.),(1.,1.),(1.,1.),(1.,1.),(1.,1.),(1.,1.),(1.,1.),(1.,1.),(1.,1.),(1.,
1.),(1.,1.),(1.,1.),(1.,1.),(1.,1.),(1.,1.),(1.,1.),(1.,1.),(1.,1.),(1.,
1.),(1.,1.)))
REPRESENTATION_ITEM('')
SURFACE()
);
#101=(
BOUNDED_SURFACE()
B_SPLINE_SURFACE(5,1,((#47056,#47057),(#47058,#47059),(#47060,#47061),(#47062,
#47063),(#47064,#47065),(#47066,#47067),(#47068,#47069),(#47070,#47071),
(#47072,#47073),(#47074,#47075),(#47076,#47077),(#47078,#47079),(#47080,
#47081),(#47082,#47083),(#47084,#47085),(#47086,#47087),(#47088,#47089),
(#47090,#47091),(#47092,#47093),(#47094,#47095),(#47096,#47097),(#47098,
#47099),(#47100,#47101),(#47102,#47103),(#47104,#47105),(#47106,#47107),
(#47108,#47109),(#47110,#47111),(#47112,#47113),(#47114,#47115),(#47116,
#47117),(#47118,#47119),(#47120,#47121),(#47122,#47123),(#47124,#47125),
(#47126,#47127),(#47128,#47129),(#47130,#47131),(#47132,#47133),(#47134,
#47135),(#47136,#47137),(#47138,#47139),(#47140,#47141),(#47142,#47143),
(#47144,#47145),(#47146,#47147),(#47148,#47149),(#47150,#47151),(#47152,
#47153),(#47154,#47155),(#47156,#47157),(#47158,#47159),(#47160,#47161),
(#47162,#47163),(#47164,#47165),(#47166,#47167),(#47168,#47169),(#47170,
#47171),(#47172,#47173),(#47174,#47175),(#47176,#47177),(#47178,#47179),
(#47180,#47181),(#47182,#47183),(#47184,#47185),(#47186,#47187),(#47188,
#47189),(#47190,#47191),(#47192,#47193),(#47194,#47195)),.UNSPECIFIED.,
 .F.,.F.,.F.)
B_SPLINE_SURFACE_WITH_KNOTS((6,1,1,1,1,1,1,1,1,1,1,1,1,1,1,1,1,1,1,1,1,
1,1,1,1,1,1,1,1,1,1,1,1,1,1,1,1,1,1,1,1,1,1,1,1,1,1,1,1,1,1,1,1,1,1,1,1,
1,1,1,1,1,1,1,1,6),(2,2),(-1.,-0.984615384615383,-0.969230769230768,-0.953846153846152,
-0.938461538461537,-0.923076923076922,-0.907692307692306,-0.892307692307691,
-0.876923076923076,-0.86153846153846,-0.846153846153845,-0.83076923076923,
-0.815384615384614,-0.799999999999999,-0.784615384615384,-0.769230769230768,
-0.753846153846153,-0.738461538461538,-0.723076923076922,-0.707692307692307,
-0.692307692307692,-0.676923076923076,-0.661538461538461,-0.646153846153846,
-0.63076923076923,-0.615384615384615,-0.6,-0.584615384615384,-0.569230769230769,
-0.553846153846154,-0.538461538461538,-0.523076923076923,-0.507692307692308,
-0.492307692307692,-0.476923076923077,-0.461538461538462,-0.446153846153846,
-0.430769230769231,-0.415384615384615,-0.4,-0.384615384615385,-0.369230769230769,
-0.353846153846154,-0.338461538461538,-0.323076923076923,-0.307692307692308,
-0.292307692307692,-0.276923076923077,-0.261538461538462,-0.246153846153846,
-0.230769230769231,-0.215384615384615,-0.2,-0.184615384615385,-0.169230769230769,
-0.153846153846154,-0.138461538461538,-0.123076923076923,-0.107692307692308,
-0.0923076923076923,-0.0769230769230769,-0.0615384615384615,-0.0461538461538462,
-0.0307692307692308,-0.0153846153846154,0.),(-1.,1.),.UNSPECIFIED.)
GEOMETRIC_REPRESENTATION_ITEM()
RATIONAL_B_SPLINE_SURFACE(((1.,1.),(1.,1.),(1.,1.),(1.,1.),(1.,1.),(1.,
1.),(1.,1.),(1.,1.),(1.,1.),(1.,1.),(1.,1.),(1.,1.),(1.,1.),(1.,1.),(1.,
1.),(1.,1.),(1.,1.),(1.,1.),(1.,1.),(1.,1.),(1.,1.),(1.,1.),(1.,1.),(1.,
1.),(1.,1.),(1.,1.),(1.,1.),(1.,1.),(1.,1.),(1.,1.),(1.,1.),(1.,1.),(1.,
1.),(1.,1.),(1.,1.),(1.,1.),(1.,1.),(1.,1.),(1.,1.),(1.,1.),(1.,1.),(1.,
1.),(1.,1.),(1.,1.),(1.,1.),(1.,1.),(1.,1.),(1.,1.),(1.,1.),(1.,1.),(1.,
1.),(1.,1.),(1.,1.),(1.,1.),(1.,1.),(1.,1.),(1.,1.),(1.,1.),(1.,1.),(1.,
1.),(1.,1.),(1.,1.),(1.,1.),(1.,1.),(1.,1.),(1.,1.),(1.,1.),(1.,1.),(1.,
1.),(1.,1.)))
REPRESENTATION_ITEM('')
SURFACE()
);
#102=(
BOUNDED_SURFACE()
B_SPLINE_SURFACE(5,1,((#47268,#47269),(#47270,#47271),(#47272,#47273),(#47274,
#47275),(#47276,#47277),(#47278,#47279),(#47280,#47281),(#47282,#47283),
(#47284,#47285),(#47286,#47287),(#47288,#47289),(#47290,#47291),(#47292,
#47293),(#47294,#47295),(#47296,#47297),(#47298,#47299),(#47300,#47301),
(#47302,#47303),(#47304,#47305),(#47306,#47307),(#47308,#47309),(#47310,
#47311),(#47312,#47313),(#47314,#47315),(#47316,#47317),(#47318,#47319),
(#47320,#47321),(#47322,#47323),(#47324,#47325),(#47326,#47327),(#47328,
#47329),(#47330,#47331),(#47332,#47333),(#47334,#47335),(#47336,#47337),
(#47338,#47339),(#47340,#47341),(#47342,#47343),(#47344,#47345),(#47346,
#47347),(#47348,#47349),(#47350,#47351),(#47352,#47353),(#47354,#47355),
(#47356,#47357),(#47358,#47359),(#47360,#47361),(#47362,#47363),(#47364,
#47365),(#47366,#47367),(#47368,#47369),(#47370,#47371),(#47372,#47373),
(#47374,#47375),(#47376,#47377),(#47378,#47379),(#47380,#47381),(#47382,
#47383),(#47384,#47385),(#47386,#47387),(#47388,#47389),(#47390,#47391),
(#47392,#47393),(#47394,#47395),(#47396,#47397),(#47398,#47399),(#47400,
#47401),(#47402,#47403),(#47404,#47405),(#47406,#47407)),.UNSPECIFIED.,
 .F.,.F.,.F.)
B_SPLINE_SURFACE_WITH_KNOTS((6,1,1,1,1,1,1,1,1,1,1,1,1,1,1,1,1,1,1,1,1,
1,1,1,1,1,1,1,1,1,1,1,1,1,1,1,1,1,1,1,1,1,1,1,1,1,1,1,1,1,1,1,1,1,1,1,1,
1,1,1,1,1,1,1,1,6),(2,2),(-1.,-0.984615384615383,-0.969230769230768,-0.953846153846152,
-0.938461538461537,-0.923076923076922,-0.907692307692306,-0.892307692307691,
-0.876923076923076,-0.86153846153846,-0.846153846153845,-0.83076923076923,
-0.815384615384614,-0.799999999999999,-0.784615384615384,-0.769230769230768,
-0.753846153846153,-0.738461538461538,-0.723076923076922,-0.707692307692307,
-0.692307692307692,-0.676923076923076,-0.661538461538461,-0.646153846153846,
-0.63076923076923,-0.615384615384615,-0.6,-0.584615384615384,-0.569230769230769,
-0.553846153846154,-0.538461538461538,-0.523076923076923,-0.507692307692308,
-0.492307692307692,-0.476923076923077,-0.461538461538462,-0.446153846153846,
-0.430769230769231,-0.415384615384615,-0.4,-0.384615384615385,-0.369230769230769,
-0.353846153846154,-0.338461538461538,-0.323076923076923,-0.307692307692308,
-0.292307692307692,-0.276923076923077,-0.261538461538462,-0.246153846153846,
-0.230769230769231,-0.215384615384615,-0.2,-0.184615384615385,-0.169230769230769,
-0.153846153846154,-0.138461538461538,-0.123076923076923,-0.107692307692308,
-0.0923076923076923,-0.0769230769230769,-0.0615384615384615,-0.0461538461538462,
-0.0307692307692308,-0.0153846153846154,0.),(-1.,1.),.UNSPECIFIED.)
GEOMETRIC_REPRESENTATION_ITEM()
RATIONAL_B_SPLINE_SURFACE(((1.,1.),(1.,1.),(1.,1.),(1.,1.),(1.,1.),(1.,
1.),(1.,1.),(1.,1.),(1.,1.),(1.,1.),(1.,1.),(1.,1.),(1.,1.),(1.,1.),(1.,
1.),(1.,1.),(1.,1.),(1.,1.),(1.,1.),(1.,1.),(1.,1.),(1.,1.),(1.,1.),(1.,
1.),(1.,1.),(1.,1.),(1.,1.),(1.,1.),(1.,1.),(1.,1.),(1.,1.),(1.,1.),(1.,
1.),(1.,1.),(1.,1.),(1.,1.),(1.,1.),(1.,1.),(1.,1.),(1.,1.),(1.,1.),(1.,
1.),(1.,1.),(1.,1.),(1.,1.),(1.,1.),(1.,1.),(1.,1.),(1.,1.),(1.,1.),(1.,
1.),(1.,1.),(1.,1.),(1.,1.),(1.,1.),(1.,1.),(1.,1.),(1.,1.),(1.,1.),(1.,
1.),(1.,1.),(1.,1.),(1.,1.),(1.,1.),(1.,1.),(1.,1.),(1.,1.),(1.,1.),(1.,
1.),(1.,1.)))
REPRESENTATION_ITEM('')
SURFACE()
);
#103=(
BOUNDED_SURFACE()
B_SPLINE_SURFACE(5,1,((#47498,#47499),(#47500,#47501),(#47502,#47503),(#47504,
#47505),(#47506,#47507),(#47508,#47509),(#47510,#47511),(#47512,#47513),
(#47514,#47515),(#47516,#47517),(#47518,#47519),(#47520,#47521),(#47522,
#47523),(#47524,#47525),(#47526,#47527),(#47528,#47529),(#47530,#47531),
(#47532,#47533),(#47534,#47535),(#47536,#47537),(#47538,#47539),(#47540,
#47541),(#47542,#47543),(#47544,#47545),(#47546,#47547),(#47548,#47549),
(#47550,#47551),(#47552,#47553),(#47554,#47555),(#47556,#47557),(#47558,
#47559),(#47560,#47561),(#47562,#47563),(#47564,#47565),(#47566,#47567),
(#47568,#47569),(#47570,#47571),(#47572,#47573),(#47574,#47575),(#47576,
#47577),(#47578,#47579),(#47580,#47581),(#47582,#47583),(#47584,#47585),
(#47586,#47587),(#47588,#47589),(#47590,#47591),(#47592,#47593),(#47594,
#47595),(#47596,#47597),(#47598,#47599),(#47600,#47601),(#47602,#47603),
(#47604,#47605),(#47606,#47607),(#47608,#47609),(#47610,#47611),(#47612,
#47613),(#47614,#47615),(#47616,#47617),(#47618,#47619),(#47620,#47621),
(#47622,#47623),(#47624,#47625),(#47626,#47627),(#47628,#47629),(#47630,
#47631),(#47632,#47633),(#47634,#47635),(#47636,#47637)),.UNSPECIFIED.,
 .F.,.F.,.F.)
B_SPLINE_SURFACE_WITH_KNOTS((6,1,1,1,1,1,1,1,1,1,1,1,1,1,1,1,1,1,1,1,1,
1,1,1,1,1,1,1,1,1,1,1,1,1,1,1,1,1,1,1,1,1,1,1,1,1,1,1,1,1,1,1,1,1,1,1,1,
1,1,1,1,1,1,1,1,6),(2,2),(-1.,-0.984615384615383,-0.969230769230768,-0.953846153846152,
-0.938461538461537,-0.923076923076922,-0.907692307692306,-0.892307692307691,
-0.876923076923076,-0.86153846153846,-0.846153846153845,-0.83076923076923,
-0.815384615384614,-0.799999999999999,-0.784615384615384,-0.769230769230768,
-0.753846153846153,-0.738461538461538,-0.723076923076922,-0.707692307692307,
-0.692307692307692,-0.676923076923076,-0.661538461538461,-0.646153846153846,
-0.63076923076923,-0.615384615384615,-0.6,-0.584615384615384,-0.569230769230769,
-0.553846153846154,-0.538461538461538,-0.523076923076923,-0.507692307692308,
-0.492307692307692,-0.476923076923077,-0.461538461538462,-0.446153846153846,
-0.430769230769231,-0.415384615384615,-0.4,-0.384615384615385,-0.369230769230769,
-0.353846153846154,-0.338461538461538,-0.323076923076923,-0.307692307692308,
-0.292307692307692,-0.276923076923077,-0.261538461538462,-0.246153846153846,
-0.230769230769231,-0.215384615384615,-0.2,-0.184615384615385,-0.169230769230769,
-0.153846153846154,-0.138461538461538,-0.123076923076923,-0.107692307692308,
-0.0923076923076923,-0.0769230769230769,-0.0615384615384615,-0.0461538461538462,
-0.0307692307692308,-0.0153846153846154,0.),(-1.,1.),.UNSPECIFIED.)
GEOMETRIC_REPRESENTATION_ITEM()
RATIONAL_B_SPLINE_SURFACE(((1.,1.),(1.,1.),(1.,1.),(1.,1.),(1.,1.),(1.,
1.),(1.,1.),(1.,1.),(1.,1.),(1.,1.),(1.,1.),(1.,1.),(1.,1.),(1.,1.),(1.,
1.),(1.,1.),(1.,1.),(1.,1.),(1.,1.),(1.,1.),(1.,1.),(1.,1.),(1.,1.),(1.,
1.),(1.,1.),(1.,1.),(1.,1.),(1.,1.),(1.,1.),(1.,1.),(1.,1.),(1.,1.),(1.,
1.),(1.,1.),(1.,1.),(1.,1.),(1.,1.),(1.,1.),(1.,1.),(1.,1.),(1.,1.),(1.,
1.),(1.,1.),(1.,1.),(1.,1.),(1.,1.),(1.,1.),(1.,1.),(1.,1.),(1.,1.),(1.,
1.),(1.,1.),(1.,1.),(1.,1.),(1.,1.),(1.,1.),(1.,1.),(1.,1.),(1.,1.),(1.,
1.),(1.,1.),(1.,1.),(1.,1.),(1.,1.),(1.,1.),(1.,1.),(1.,1.),(1.,1.),(1.,
1.),(1.,1.)))
REPRESENTATION_ITEM('')
SURFACE()
);
#104=(
BOUNDED_SURFACE()
B_SPLINE_SURFACE(5,1,((#47710,#47711),(#47712,#47713),(#47714,#47715),(#47716,
#47717),(#47718,#47719),(#47720,#47721),(#47722,#47723),(#47724,#47725),
(#47726,#47727),(#47728,#47729),(#47730,#47731),(#47732,#47733),(#47734,
#47735),(#47736,#47737),(#47738,#47739),(#47740,#47741),(#47742,#47743),
(#47744,#47745),(#47746,#47747),(#47748,#47749),(#47750,#47751),(#47752,
#47753),(#47754,#47755),(#47756,#47757),(#47758,#47759),(#47760,#47761),
(#47762,#47763),(#47764,#47765),(#47766,#47767),(#47768,#47769),(#47770,
#47771),(#47772,#47773),(#47774,#47775),(#47776,#47777),(#47778,#47779),
(#47780,#47781),(#47782,#47783),(#47784,#47785),(#47786,#47787),(#47788,
#47789),(#47790,#47791),(#47792,#47793),(#47794,#47795),(#47796,#47797),
(#47798,#47799),(#47800,#47801),(#47802,#47803),(#47804,#47805),(#47806,
#47807),(#47808,#47809),(#47810,#47811),(#47812,#47813),(#47814,#47815),
(#47816,#47817),(#47818,#47819),(#47820,#47821),(#47822,#47823),(#47824,
#47825),(#47826,#47827),(#47828,#47829),(#47830,#47831),(#47832,#47833),
(#47834,#47835),(#47836,#47837),(#47838,#47839),(#47840,#47841),(#47842,
#47843),(#47844,#47845),(#47846,#47847),(#47848,#47849)),.UNSPECIFIED.,
 .F.,.F.,.F.)
B_SPLINE_SURFACE_WITH_KNOTS((6,1,1,1,1,1,1,1,1,1,1,1,1,1,1,1,1,1,1,1,1,
1,1,1,1,1,1,1,1,1,1,1,1,1,1,1,1,1,1,1,1,1,1,1,1,1,1,1,1,1,1,1,1,1,1,1,1,
1,1,1,1,1,1,1,1,6),(2,2),(-1.,-0.984615384615383,-0.969230769230768,-0.953846153846152,
-0.938461538461537,-0.923076923076922,-0.907692307692306,-0.892307692307691,
-0.876923076923076,-0.86153846153846,-0.846153846153845,-0.83076923076923,
-0.815384615384614,-0.799999999999999,-0.784615384615384,-0.769230769230768,
-0.753846153846153,-0.738461538461538,-0.723076923076922,-0.707692307692307,
-0.692307692307692,-0.676923076923076,-0.661538461538461,-0.646153846153846,
-0.63076923076923,-0.615384615384615,-0.6,-0.584615384615384,-0.569230769230769,
-0.553846153846154,-0.538461538461538,-0.523076923076923,-0.507692307692308,
-0.492307692307692,-0.476923076923077,-0.461538461538462,-0.446153846153846,
-0.430769230769231,-0.415384615384615,-0.4,-0.384615384615385,-0.369230769230769,
-0.353846153846154,-0.338461538461538,-0.323076923076923,-0.307692307692308,
-0.292307692307692,-0.276923076923077,-0.261538461538462,-0.246153846153846,
-0.230769230769231,-0.215384615384615,-0.2,-0.184615384615385,-0.169230769230769,
-0.153846153846154,-0.138461538461538,-0.123076923076923,-0.107692307692308,
-0.0923076923076923,-0.0769230769230769,-0.0615384615384615,-0.0461538461538462,
-0.0307692307692308,-0.0153846153846154,0.),(-1.,1.),.UNSPECIFIED.)
GEOMETRIC_REPRESENTATION_ITEM()
RATIONAL_B_SPLINE_SURFACE(((1.,1.),(1.,1.),(1.,1.),(1.,1.),(1.,1.),(1.,
1.),(1.,1.),(1.,1.),(1.,1.),(1.,1.),(1.,1.),(1.,1.),(1.,1.),(1.,1.),(1.,
1.),(1.,1.),(1.,1.),(1.,1.),(1.,1.),(1.,1.),(1.,1.),(1.,1.),(1.,1.),(1.,
1.),(1.,1.),(1.,1.),(1.,1.),(1.,1.),(1.,1.),(1.,1.),(1.,1.),(1.,1.),(1.,
1.),(1.,1.),(1.,1.),(1.,1.),(1.,1.),(1.,1.),(1.,1.),(1.,1.),(1.,1.),(1.,
1.),(1.,1.),(1.,1.),(1.,1.),(1.,1.),(1.,1.),(1.,1.),(1.,1.),(1.,1.),(1.,
1.),(1.,1.),(1.,1.),(1.,1.),(1.,1.),(1.,1.),(1.,1.),(1.,1.),(1.,1.),(1.,
1.),(1.,1.),(1.,1.),(1.,1.),(1.,1.),(1.,1.),(1.,1.),(1.,1.),(1.,1.),(1.,
1.),(1.,1.)))
REPRESENTATION_ITEM('')
SURFACE()
);
#105=(
BOUNDED_SURFACE()
B_SPLINE_SURFACE(5,1,((#47940,#47941),(#47942,#47943),(#47944,#47945),(#47946,
#47947),(#47948,#47949),(#47950,#47951),(#47952,#47953),(#47954,#47955),
(#47956,#47957),(#47958,#47959),(#47960,#47961),(#47962,#47963),(#47964,
#47965),(#47966,#47967),(#47968,#47969),(#47970,#47971),(#47972,#47973),
(#47974,#47975),(#47976,#47977),(#47978,#47979),(#47980,#47981),(#47982,
#47983),(#47984,#47985),(#47986,#47987),(#47988,#47989),(#47990,#47991),
(#47992,#47993),(#47994,#47995),(#47996,#47997),(#47998,#47999),(#48000,
#48001),(#48002,#48003),(#48004,#48005),(#48006,#48007),(#48008,#48009),
(#48010,#48011),(#48012,#48013),(#48014,#48015),(#48016,#48017),(#48018,
#48019),(#48020,#48021),(#48022,#48023),(#48024,#48025),(#48026,#48027),
(#48028,#48029),(#48030,#48031),(#48032,#48033),(#48034,#48035),(#48036,
#48037),(#48038,#48039),(#48040,#48041),(#48042,#48043),(#48044,#48045),
(#48046,#48047),(#48048,#48049),(#48050,#48051),(#48052,#48053),(#48054,
#48055),(#48056,#48057),(#48058,#48059),(#48060,#48061),(#48062,#48063),
(#48064,#48065),(#48066,#48067),(#48068,#48069),(#48070,#48071),(#48072,
#48073),(#48074,#48075),(#48076,#48077),(#48078,#48079)),.UNSPECIFIED.,
 .F.,.F.,.F.)
B_SPLINE_SURFACE_WITH_KNOTS((6,1,1,1,1,1,1,1,1,1,1,1,1,1,1,1,1,1,1,1,1,
1,1,1,1,1,1,1,1,1,1,1,1,1,1,1,1,1,1,1,1,1,1,1,1,1,1,1,1,1,1,1,1,1,1,1,1,
1,1,1,1,1,1,1,1,6),(2,2),(-1.,-0.984615384615383,-0.969230769230768,-0.953846153846152,
-0.938461538461537,-0.923076923076922,-0.907692307692306,-0.892307692307691,
-0.876923076923076,-0.86153846153846,-0.846153846153845,-0.83076923076923,
-0.815384615384614,-0.799999999999999,-0.784615384615384,-0.769230769230768,
-0.753846153846153,-0.738461538461538,-0.723076923076922,-0.707692307692307,
-0.692307692307692,-0.676923076923076,-0.661538461538461,-0.646153846153846,
-0.63076923076923,-0.615384615384615,-0.6,-0.584615384615384,-0.569230769230769,
-0.553846153846154,-0.538461538461538,-0.523076923076923,-0.507692307692308,
-0.492307692307692,-0.476923076923077,-0.461538461538462,-0.446153846153846,
-0.430769230769231,-0.415384615384615,-0.4,-0.384615384615385,-0.369230769230769,
-0.353846153846154,-0.338461538461538,-0.323076923076923,-0.307692307692308,
-0.292307692307692,-0.276923076923077,-0.261538461538462,-0.246153846153846,
-0.230769230769231,-0.215384615384615,-0.2,-0.184615384615385,-0.169230769230769,
-0.153846153846154,-0.138461538461538,-0.123076923076923,-0.107692307692308,
-0.0923076923076923,-0.0769230769230769,-0.0615384615384615,-0.0461538461538462,
-0.0307692307692308,-0.0153846153846154,0.),(-1.,1.),.UNSPECIFIED.)
GEOMETRIC_REPRESENTATION_ITEM()
RATIONAL_B_SPLINE_SURFACE(((1.,1.),(1.,1.),(1.,1.),(1.,1.),(1.,1.),(1.,
1.),(1.,1.),(1.,1.),(1.,1.),(1.,1.),(1.,1.),(1.,1.),(1.,1.),(1.,1.),(1.,
1.),(1.,1.),(1.,1.),(1.,1.),(1.,1.),(1.,1.),(1.,1.),(1.,1.),(1.,1.),(1.,
1.),(1.,1.),(1.,1.),(1.,1.),(1.,1.),(1.,1.),(1.,1.),(1.,1.),(1.,1.),(1.,
1.),(1.,1.),(1.,1.),(1.,1.),(1.,1.),(1.,1.),(1.,1.),(1.,1.),(1.,1.),(1.,
1.),(1.,1.),(1.,1.),(1.,1.),(1.,1.),(1.,1.),(1.,1.),(1.,1.),(1.,1.),(1.,
1.),(1.,1.),(1.,1.),(1.,1.),(1.,1.),(1.,1.),(1.,1.),(1.,1.),(1.,1.),(1.,
1.),(1.,1.),(1.,1.),(1.,1.),(1.,1.),(1.,1.),(1.,1.),(1.,1.),(1.,1.),(1.,
1.),(1.,1.)))
REPRESENTATION_ITEM('')
SURFACE()
);
#106=(
BOUNDED_SURFACE()
B_SPLINE_SURFACE(5,1,((#48152,#48153),(#48154,#48155),(#48156,#48157),(#48158,
#48159),(#48160,#48161),(#48162,#48163),(#48164,#48165),(#48166,#48167),
(#48168,#48169),(#48170,#48171),(#48172,#48173),(#48174,#48175),(#48176,
#48177),(#48178,#48179),(#48180,#48181),(#48182,#48183),(#48184,#48185),
(#48186,#48187),(#48188,#48189),(#48190,#48191),(#48192,#48193),(#48194,
#48195),(#48196,#48197),(#48198,#48199),(#48200,#48201),(#48202,#48203),
(#48204,#48205),(#48206,#48207),(#48208,#48209),(#48210,#48211),(#48212,
#48213),(#48214,#48215),(#48216,#48217),(#48218,#48219),(#48220,#48221),
(#48222,#48223),(#48224,#48225),(#48226,#48227),(#48228,#48229),(#48230,
#48231),(#48232,#48233),(#48234,#48235),(#48236,#48237),(#48238,#48239),
(#48240,#48241),(#48242,#48243),(#48244,#48245),(#48246,#48247),(#48248,
#48249),(#48250,#48251),(#48252,#48253),(#48254,#48255),(#48256,#48257),
(#48258,#48259),(#48260,#48261),(#48262,#48263),(#48264,#48265),(#48266,
#48267),(#48268,#48269),(#48270,#48271),(#48272,#48273),(#48274,#48275),
(#48276,#48277),(#48278,#48279),(#48280,#48281),(#48282,#48283),(#48284,
#48285),(#48286,#48287),(#48288,#48289),(#48290,#48291)),.UNSPECIFIED.,
 .F.,.F.,.F.)
B_SPLINE_SURFACE_WITH_KNOTS((6,1,1,1,1,1,1,1,1,1,1,1,1,1,1,1,1,1,1,1,1,
1,1,1,1,1,1,1,1,1,1,1,1,1,1,1,1,1,1,1,1,1,1,1,1,1,1,1,1,1,1,1,1,1,1,1,1,
1,1,1,1,1,1,1,1,6),(2,2),(-1.,-0.984615384615383,-0.969230769230768,-0.953846153846152,
-0.938461538461537,-0.923076923076922,-0.907692307692306,-0.892307692307691,
-0.876923076923076,-0.86153846153846,-0.846153846153845,-0.83076923076923,
-0.815384615384614,-0.799999999999999,-0.784615384615384,-0.769230769230768,
-0.753846153846153,-0.738461538461538,-0.723076923076922,-0.707692307692307,
-0.692307692307692,-0.676923076923076,-0.661538461538461,-0.646153846153846,
-0.63076923076923,-0.615384615384615,-0.6,-0.584615384615384,-0.569230769230769,
-0.553846153846154,-0.538461538461538,-0.523076923076923,-0.507692307692308,
-0.492307692307692,-0.476923076923077,-0.461538461538462,-0.446153846153846,
-0.430769230769231,-0.415384615384615,-0.4,-0.384615384615385,-0.369230769230769,
-0.353846153846154,-0.338461538461538,-0.323076923076923,-0.307692307692308,
-0.292307692307692,-0.276923076923077,-0.261538461538462,-0.246153846153846,
-0.230769230769231,-0.215384615384615,-0.2,-0.184615384615385,-0.169230769230769,
-0.153846153846154,-0.138461538461538,-0.123076923076923,-0.107692307692308,
-0.0923076923076923,-0.0769230769230769,-0.0615384615384615,-0.0461538461538462,
-0.0307692307692308,-0.0153846153846154,0.),(-1.,1.),.UNSPECIFIED.)
GEOMETRIC_REPRESENTATION_ITEM()
RATIONAL_B_SPLINE_SURFACE(((1.,1.),(1.,1.),(1.,1.),(1.,1.),(1.,1.),(1.,
1.),(1.,1.),(1.,1.),(1.,1.),(1.,1.),(1.,1.),(1.,1.),(1.,1.),(1.,1.),(1.,
1.),(1.,1.),(1.,1.),(1.,1.),(1.,1.),(1.,1.),(1.,1.),(1.,1.),(1.,1.),(1.,
1.),(1.,1.),(1.,1.),(1.,1.),(1.,1.),(1.,1.),(1.,1.),(1.,1.),(1.,1.),(1.,
1.),(1.,1.),(1.,1.),(1.,1.),(1.,1.),(1.,1.),(1.,1.),(1.,1.),(1.,1.),(1.,
1.),(1.,1.),(1.,1.),(1.,1.),(1.,1.),(1.,1.),(1.,1.),(1.,1.),(1.,1.),(1.,
1.),(1.,1.),(1.,1.),(1.,1.),(1.,1.),(1.,1.),(1.,1.),(1.,1.),(1.,1.),(1.,
1.),(1.,1.),(1.,1.),(1.,1.),(1.,1.),(1.,1.),(1.,1.),(1.,1.),(1.,1.),(1.,
1.),(1.,1.)))
REPRESENTATION_ITEM('')
SURFACE()
);
#107=(
BOUNDED_SURFACE()
B_SPLINE_SURFACE(5,1,((#48382,#48383),(#48384,#48385),(#48386,#48387),(#48388,
#48389),(#48390,#48391),(#48392,#48393),(#48394,#48395),(#48396,#48397),
(#48398,#48399),(#48400,#48401),(#48402,#48403),(#48404,#48405),(#48406,
#48407),(#48408,#48409),(#48410,#48411),(#48412,#48413),(#48414,#48415),
(#48416,#48417),(#48418,#48419),(#48420,#48421),(#48422,#48423),(#48424,
#48425),(#48426,#48427),(#48428,#48429),(#48430,#48431),(#48432,#48433),
(#48434,#48435),(#48436,#48437),(#48438,#48439),(#48440,#48441),(#48442,
#48443),(#48444,#48445),(#48446,#48447),(#48448,#48449),(#48450,#48451),
(#48452,#48453),(#48454,#48455),(#48456,#48457),(#48458,#48459),(#48460,
#48461),(#48462,#48463),(#48464,#48465),(#48466,#48467),(#48468,#48469),
(#48470,#48471),(#48472,#48473),(#48474,#48475),(#48476,#48477),(#48478,
#48479),(#48480,#48481),(#48482,#48483),(#48484,#48485),(#48486,#48487),
(#48488,#48489),(#48490,#48491),(#48492,#48493),(#48494,#48495),(#48496,
#48497),(#48498,#48499),(#48500,#48501),(#48502,#48503),(#48504,#48505),
(#48506,#48507),(#48508,#48509),(#48510,#48511),(#48512,#48513),(#48514,
#48515),(#48516,#48517),(#48518,#48519),(#48520,#48521)),.UNSPECIFIED.,
 .F.,.F.,.F.)
B_SPLINE_SURFACE_WITH_KNOTS((6,1,1,1,1,1,1,1,1,1,1,1,1,1,1,1,1,1,1,1,1,
1,1,1,1,1,1,1,1,1,1,1,1,1,1,1,1,1,1,1,1,1,1,1,1,1,1,1,1,1,1,1,1,1,1,1,1,
1,1,1,1,1,1,1,1,6),(2,2),(-1.,-0.984615384615383,-0.969230769230768,-0.953846153846152,
-0.938461538461537,-0.923076923076922,-0.907692307692306,-0.892307692307691,
-0.876923076923076,-0.86153846153846,-0.846153846153845,-0.83076923076923,
-0.815384615384614,-0.799999999999999,-0.784615384615384,-0.769230769230768,
-0.753846153846153,-0.738461538461538,-0.723076923076922,-0.707692307692307,
-0.692307692307692,-0.676923076923076,-0.661538461538461,-0.646153846153846,
-0.63076923076923,-0.615384615384615,-0.6,-0.584615384615384,-0.569230769230769,
-0.553846153846154,-0.538461538461538,-0.523076923076923,-0.507692307692308,
-0.492307692307692,-0.476923076923077,-0.461538461538462,-0.446153846153846,
-0.430769230769231,-0.415384615384615,-0.4,-0.384615384615385,-0.369230769230769,
-0.353846153846154,-0.338461538461538,-0.323076923076923,-0.307692307692308,
-0.292307692307692,-0.276923076923077,-0.261538461538462,-0.246153846153846,
-0.230769230769231,-0.215384615384615,-0.2,-0.184615384615385,-0.169230769230769,
-0.153846153846154,-0.138461538461538,-0.123076923076923,-0.107692307692308,
-0.0923076923076923,-0.0769230769230769,-0.0615384615384615,-0.0461538461538462,
-0.0307692307692308,-0.0153846153846154,0.),(-1.,1.),.UNSPECIFIED.)
GEOMETRIC_REPRESENTATION_ITEM()
RATIONAL_B_SPLINE_SURFACE(((1.,1.),(1.,1.),(1.,1.),(1.,1.),(1.,1.),(1.,
1.),(1.,1.),(1.,1.),(1.,1.),(1.,1.),(1.,1.),(1.,1.),(1.,1.),(1.,1.),(1.,
1.),(1.,1.),(1.,1.),(1.,1.),(1.,1.),(1.,1.),(1.,1.),(1.,1.),(1.,1.),(1.,
1.),(1.,1.),(1.,1.),(1.,1.),(1.,1.),(1.,1.),(1.,1.),(1.,1.),(1.,1.),(1.,
1.),(1.,1.),(1.,1.),(1.,1.),(1.,1.),(1.,1.),(1.,1.),(1.,1.),(1.,1.),(1.,
1.),(1.,1.),(1.,1.),(1.,1.),(1.,1.),(1.,1.),(1.,1.),(1.,1.),(1.,1.),(1.,
1.),(1.,1.),(1.,1.),(1.,1.),(1.,1.),(1.,1.),(1.,1.),(1.,1.),(1.,1.),(1.,
1.),(1.,1.),(1.,1.),(1.,1.),(1.,1.),(1.,1.),(1.,1.),(1.,1.),(1.,1.),(1.,
1.),(1.,1.)))
REPRESENTATION_ITEM('')
SURFACE()
);
#108=(
BOUNDED_SURFACE()
B_SPLINE_SURFACE(5,1,((#48594,#48595),(#48596,#48597),(#48598,#48599),(#48600,
#48601),(#48602,#48603),(#48604,#48605),(#48606,#48607),(#48608,#48609),
(#48610,#48611),(#48612,#48613),(#48614,#48615),(#48616,#48617),(#48618,
#48619),(#48620,#48621),(#48622,#48623),(#48624,#48625),(#48626,#48627),
(#48628,#48629),(#48630,#48631),(#48632,#48633),(#48634,#48635),(#48636,
#48637),(#48638,#48639),(#48640,#48641),(#48642,#48643),(#48644,#48645),
(#48646,#48647),(#48648,#48649),(#48650,#48651),(#48652,#48653),(#48654,
#48655),(#48656,#48657),(#48658,#48659),(#48660,#48661),(#48662,#48663),
(#48664,#48665),(#48666,#48667),(#48668,#48669),(#48670,#48671),(#48672,
#48673),(#48674,#48675),(#48676,#48677),(#48678,#48679),(#48680,#48681),
(#48682,#48683),(#48684,#48685),(#48686,#48687),(#48688,#48689),(#48690,
#48691),(#48692,#48693),(#48694,#48695),(#48696,#48697),(#48698,#48699),
(#48700,#48701),(#48702,#48703),(#48704,#48705),(#48706,#48707),(#48708,
#48709),(#48710,#48711),(#48712,#48713),(#48714,#48715),(#48716,#48717),
(#48718,#48719),(#48720,#48721),(#48722,#48723),(#48724,#48725),(#48726,
#48727),(#48728,#48729),(#48730,#48731),(#48732,#48733)),.UNSPECIFIED.,
 .F.,.F.,.F.)
B_SPLINE_SURFACE_WITH_KNOTS((6,1,1,1,1,1,1,1,1,1,1,1,1,1,1,1,1,1,1,1,1,
1,1,1,1,1,1,1,1,1,1,1,1,1,1,1,1,1,1,1,1,1,1,1,1,1,1,1,1,1,1,1,1,1,1,1,1,
1,1,1,1,1,1,1,1,6),(2,2),(-1.,-0.984615384615383,-0.969230769230768,-0.953846153846152,
-0.938461538461537,-0.923076923076922,-0.907692307692306,-0.892307692307691,
-0.876923076923076,-0.86153846153846,-0.846153846153845,-0.83076923076923,
-0.815384615384614,-0.799999999999999,-0.784615384615384,-0.769230769230768,
-0.753846153846153,-0.738461538461538,-0.723076923076922,-0.707692307692307,
-0.692307692307692,-0.676923076923076,-0.661538461538461,-0.646153846153846,
-0.63076923076923,-0.615384615384615,-0.6,-0.584615384615384,-0.569230769230769,
-0.553846153846154,-0.538461538461538,-0.523076923076923,-0.507692307692308,
-0.492307692307692,-0.476923076923077,-0.461538461538462,-0.446153846153846,
-0.430769230769231,-0.415384615384615,-0.4,-0.384615384615385,-0.369230769230769,
-0.353846153846154,-0.338461538461538,-0.323076923076923,-0.307692307692308,
-0.292307692307692,-0.276923076923077,-0.261538461538462,-0.246153846153846,
-0.230769230769231,-0.215384615384615,-0.2,-0.184615384615385,-0.169230769230769,
-0.153846153846154,-0.138461538461538,-0.123076923076923,-0.107692307692308,
-0.0923076923076923,-0.0769230769230769,-0.0615384615384615,-0.0461538461538462,
-0.0307692307692308,-0.0153846153846154,0.),(-1.,1.),.UNSPECIFIED.)
GEOMETRIC_REPRESENTATION_ITEM()
RATIONAL_B_SPLINE_SURFACE(((1.,1.),(1.,1.),(1.,1.),(1.,1.),(1.,1.),(1.,
1.),(1.,1.),(1.,1.),(1.,1.),(1.,1.),(1.,1.),(1.,1.),(1.,1.),(1.,1.),(1.,
1.),(1.,1.),(1.,1.),(1.,1.),(1.,1.),(1.,1.),(1.,1.),(1.,1.),(1.,1.),(1.,
1.),(1.,1.),(1.,1.),(1.,1.),(1.,1.),(1.,1.),(1.,1.),(1.,1.),(1.,1.),(1.,
1.),(1.,1.),(1.,1.),(1.,1.),(1.,1.),(1.,1.),(1.,1.),(1.,1.),(1.,1.),(1.,
1.),(1.,1.),(1.,1.),(1.,1.),(1.,1.),(1.,1.),(1.,1.),(1.,1.),(1.,1.),(1.,
1.),(1.,1.),(1.,1.),(1.,1.),(1.,1.),(1.,1.),(1.,1.),(1.,1.),(1.,1.),(1.,
1.),(1.,1.),(1.,1.),(1.,1.),(1.,1.),(1.,1.),(1.,1.),(1.,1.),(1.,1.),(1.,
1.),(1.,1.)))
REPRESENTATION_ITEM('')
SURFACE()
);
#109=(
BOUNDED_SURFACE()
B_SPLINE_SURFACE(5,1,((#48824,#48825),(#48826,#48827),(#48828,#48829),(#48830,
#48831),(#48832,#48833),(#48834,#48835),(#48836,#48837),(#48838,#48839),
(#48840,#48841),(#48842,#48843),(#48844,#48845),(#48846,#48847),(#48848,
#48849),(#48850,#48851),(#48852,#48853),(#48854,#48855),(#48856,#48857),
(#48858,#48859),(#48860,#48861),(#48862,#48863),(#48864,#48865),(#48866,
#48867),(#48868,#48869),(#48870,#48871),(#48872,#48873),(#48874,#48875),
(#48876,#48877),(#48878,#48879),(#48880,#48881),(#48882,#48883),(#48884,
#48885),(#48886,#48887),(#48888,#48889),(#48890,#48891),(#48892,#48893),
(#48894,#48895),(#48896,#48897),(#48898,#48899),(#48900,#48901),(#48902,
#48903),(#48904,#48905),(#48906,#48907),(#48908,#48909),(#48910,#48911),
(#48912,#48913),(#48914,#48915),(#48916,#48917),(#48918,#48919),(#48920,
#48921),(#48922,#48923),(#48924,#48925),(#48926,#48927),(#48928,#48929),
(#48930,#48931),(#48932,#48933),(#48934,#48935),(#48936,#48937),(#48938,
#48939),(#48940,#48941),(#48942,#48943),(#48944,#48945),(#48946,#48947),
(#48948,#48949),(#48950,#48951),(#48952,#48953),(#48954,#48955),(#48956,
#48957),(#48958,#48959),(#48960,#48961),(#48962,#48963)),.UNSPECIFIED.,
 .F.,.F.,.F.)
B_SPLINE_SURFACE_WITH_KNOTS((6,1,1,1,1,1,1,1,1,1,1,1,1,1,1,1,1,1,1,1,1,
1,1,1,1,1,1,1,1,1,1,1,1,1,1,1,1,1,1,1,1,1,1,1,1,1,1,1,1,1,1,1,1,1,1,1,1,
1,1,1,1,1,1,1,1,6),(2,2),(-1.,-0.984615384615383,-0.969230769230768,-0.953846153846152,
-0.938461538461537,-0.923076923076922,-0.907692307692306,-0.892307692307691,
-0.876923076923076,-0.86153846153846,-0.846153846153845,-0.83076923076923,
-0.815384615384614,-0.799999999999999,-0.784615384615384,-0.769230769230768,
-0.753846153846153,-0.738461538461538,-0.723076923076922,-0.707692307692307,
-0.692307692307692,-0.676923076923076,-0.661538461538461,-0.646153846153846,
-0.63076923076923,-0.615384615384615,-0.6,-0.584615384615384,-0.569230769230769,
-0.553846153846154,-0.538461538461538,-0.523076923076923,-0.507692307692308,
-0.492307692307692,-0.476923076923077,-0.461538461538462,-0.446153846153846,
-0.430769230769231,-0.415384615384615,-0.4,-0.384615384615385,-0.369230769230769,
-0.353846153846154,-0.338461538461538,-0.323076923076923,-0.307692307692308,
-0.292307692307692,-0.276923076923077,-0.261538461538462,-0.246153846153846,
-0.230769230769231,-0.215384615384615,-0.2,-0.184615384615385,-0.169230769230769,
-0.153846153846154,-0.138461538461538,-0.123076923076923,-0.107692307692308,
-0.0923076923076923,-0.0769230769230769,-0.0615384615384615,-0.0461538461538462,
-0.0307692307692308,-0.0153846153846154,0.),(-1.,1.),.UNSPECIFIED.)
GEOMETRIC_REPRESENTATION_ITEM()
RATIONAL_B_SPLINE_SURFACE(((1.,1.),(1.,1.),(1.,1.),(1.,1.),(1.,1.),(1.,
1.),(1.,1.),(1.,1.),(1.,1.),(1.,1.),(1.,1.),(1.,1.),(1.,1.),(1.,1.),(1.,
1.),(1.,1.),(1.,1.),(1.,1.),(1.,1.),(1.,1.),(1.,1.),(1.,1.),(1.,1.),(1.,
1.),(1.,1.),(1.,1.),(1.,1.),(1.,1.),(1.,1.),(1.,1.),(1.,1.),(1.,1.),(1.,
1.),(1.,1.),(1.,1.),(1.,1.),(1.,1.),(1.,1.),(1.,1.),(1.,1.),(1.,1.),(1.,
1.),(1.,1.),(1.,1.),(1.,1.),(1.,1.),(1.,1.),(1.,1.),(1.,1.),(1.,1.),(1.,
1.),(1.,1.),(1.,1.),(1.,1.),(1.,1.),(1.,1.),(1.,1.),(1.,1.),(1.,1.),(1.,
1.),(1.,1.),(1.,1.),(1.,1.),(1.,1.),(1.,1.),(1.,1.),(1.,1.),(1.,1.),(1.,
1.),(1.,1.)))
REPRESENTATION_ITEM('')
SURFACE()
);
#110=(
BOUNDED_SURFACE()
B_SPLINE_SURFACE(5,1,((#49036,#49037),(#49038,#49039),(#49040,#49041),(#49042,
#49043),(#49044,#49045),(#49046,#49047),(#49048,#49049),(#49050,#49051),
(#49052,#49053),(#49054,#49055),(#49056,#49057),(#49058,#49059),(#49060,
#49061),(#49062,#49063),(#49064,#49065),(#49066,#49067),(#49068,#49069),
(#49070,#49071),(#49072,#49073),(#49074,#49075),(#49076,#49077),(#49078,
#49079),(#49080,#49081),(#49082,#49083),(#49084,#49085),(#49086,#49087),
(#49088,#49089),(#49090,#49091),(#49092,#49093),(#49094,#49095),(#49096,
#49097),(#49098,#49099),(#49100,#49101),(#49102,#49103),(#49104,#49105),
(#49106,#49107),(#49108,#49109),(#49110,#49111),(#49112,#49113),(#49114,
#49115),(#49116,#49117),(#49118,#49119),(#49120,#49121),(#49122,#49123),
(#49124,#49125),(#49126,#49127),(#49128,#49129),(#49130,#49131),(#49132,
#49133),(#49134,#49135),(#49136,#49137),(#49138,#49139),(#49140,#49141),
(#49142,#49143),(#49144,#49145),(#49146,#49147),(#49148,#49149),(#49150,
#49151),(#49152,#49153),(#49154,#49155),(#49156,#49157),(#49158,#49159),
(#49160,#49161),(#49162,#49163),(#49164,#49165),(#49166,#49167),(#49168,
#49169),(#49170,#49171),(#49172,#49173),(#49174,#49175)),.UNSPECIFIED.,
 .F.,.F.,.F.)
B_SPLINE_SURFACE_WITH_KNOTS((6,1,1,1,1,1,1,1,1,1,1,1,1,1,1,1,1,1,1,1,1,
1,1,1,1,1,1,1,1,1,1,1,1,1,1,1,1,1,1,1,1,1,1,1,1,1,1,1,1,1,1,1,1,1,1,1,1,
1,1,1,1,1,1,1,1,6),(2,2),(-1.,-0.984615384615383,-0.969230769230768,-0.953846153846152,
-0.938461538461537,-0.923076923076922,-0.907692307692306,-0.892307692307691,
-0.876923076923076,-0.86153846153846,-0.846153846153845,-0.83076923076923,
-0.815384615384614,-0.799999999999999,-0.784615384615384,-0.769230769230768,
-0.753846153846153,-0.738461538461538,-0.723076923076922,-0.707692307692307,
-0.692307692307692,-0.676923076923076,-0.661538461538461,-0.646153846153846,
-0.63076923076923,-0.615384615384615,-0.6,-0.584615384615384,-0.569230769230769,
-0.553846153846154,-0.538461538461538,-0.523076923076923,-0.507692307692308,
-0.492307692307692,-0.476923076923077,-0.461538461538462,-0.446153846153846,
-0.430769230769231,-0.415384615384615,-0.4,-0.384615384615385,-0.369230769230769,
-0.353846153846154,-0.338461538461538,-0.323076923076923,-0.307692307692308,
-0.292307692307692,-0.276923076923077,-0.261538461538462,-0.246153846153846,
-0.230769230769231,-0.215384615384615,-0.2,-0.184615384615385,-0.169230769230769,
-0.153846153846154,-0.138461538461538,-0.123076923076923,-0.107692307692308,
-0.0923076923076923,-0.0769230769230769,-0.0615384615384615,-0.0461538461538462,
-0.0307692307692308,-0.0153846153846154,0.),(-1.,1.),.UNSPECIFIED.)
GEOMETRIC_REPRESENTATION_ITEM()
RATIONAL_B_SPLINE_SURFACE(((1.,1.),(1.,1.),(1.,1.),(1.,1.),(1.,1.),(1.,
1.),(1.,1.),(1.,1.),(1.,1.),(1.,1.),(1.,1.),(1.,1.),(1.,1.),(1.,1.),(1.,
1.),(1.,1.),(1.,1.),(1.,1.),(1.,1.),(1.,1.),(1.,1.),(1.,1.),(1.,1.),(1.,
1.),(1.,1.),(1.,1.),(1.,1.),(1.,1.),(1.,1.),(1.,1.),(1.,1.),(1.,1.),(1.,
1.),(1.,1.),(1.,1.),(1.,1.),(1.,1.),(1.,1.),(1.,1.),(1.,1.),(1.,1.),(1.,
1.),(1.,1.),(1.,1.),(1.,1.),(1.,1.),(1.,1.),(1.,1.),(1.,1.),(1.,1.),(1.,
1.),(1.,1.),(1.,1.),(1.,1.),(1.,1.),(1.,1.),(1.,1.),(1.,1.),(1.,1.),(1.,
1.),(1.,1.),(1.,1.),(1.,1.),(1.,1.),(1.,1.),(1.,1.),(1.,1.),(1.,1.),(1.,
1.),(1.,1.)))
REPRESENTATION_ITEM('')
SURFACE()
);
#111=(
BOUNDED_SURFACE()
B_SPLINE_SURFACE(5,1,((#49266,#49267),(#49268,#49269),(#49270,#49271),(#49272,
#49273),(#49274,#49275),(#49276,#49277),(#49278,#49279),(#49280,#49281),
(#49282,#49283),(#49284,#49285),(#49286,#49287),(#49288,#49289),(#49290,
#49291),(#49292,#49293),(#49294,#49295),(#49296,#49297),(#49298,#49299),
(#49300,#49301),(#49302,#49303),(#49304,#49305),(#49306,#49307),(#49308,
#49309),(#49310,#49311),(#49312,#49313),(#49314,#49315),(#49316,#49317),
(#49318,#49319),(#49320,#49321),(#49322,#49323),(#49324,#49325),(#49326,
#49327),(#49328,#49329),(#49330,#49331),(#49332,#49333),(#49334,#49335),
(#49336,#49337),(#49338,#49339),(#49340,#49341),(#49342,#49343),(#49344,
#49345),(#49346,#49347),(#49348,#49349),(#49350,#49351),(#49352,#49353),
(#49354,#49355),(#49356,#49357),(#49358,#49359),(#49360,#49361),(#49362,
#49363),(#49364,#49365),(#49366,#49367),(#49368,#49369),(#49370,#49371),
(#49372,#49373),(#49374,#49375),(#49376,#49377),(#49378,#49379),(#49380,
#49381),(#49382,#49383),(#49384,#49385),(#49386,#49387),(#49388,#49389),
(#49390,#49391),(#49392,#49393),(#49394,#49395),(#49396,#49397),(#49398,
#49399),(#49400,#49401),(#49402,#49403),(#49404,#49405)),.UNSPECIFIED.,
 .F.,.F.,.F.)
B_SPLINE_SURFACE_WITH_KNOTS((6,1,1,1,1,1,1,1,1,1,1,1,1,1,1,1,1,1,1,1,1,
1,1,1,1,1,1,1,1,1,1,1,1,1,1,1,1,1,1,1,1,1,1,1,1,1,1,1,1,1,1,1,1,1,1,1,1,
1,1,1,1,1,1,1,1,6),(2,2),(-1.,-0.984615384615383,-0.969230769230768,-0.953846153846152,
-0.938461538461537,-0.923076923076922,-0.907692307692306,-0.892307692307691,
-0.876923076923076,-0.86153846153846,-0.846153846153845,-0.83076923076923,
-0.815384615384614,-0.799999999999999,-0.784615384615384,-0.769230769230768,
-0.753846153846153,-0.738461538461538,-0.723076923076922,-0.707692307692307,
-0.692307692307692,-0.676923076923076,-0.661538461538461,-0.646153846153846,
-0.63076923076923,-0.615384615384615,-0.6,-0.584615384615384,-0.569230769230769,
-0.553846153846154,-0.538461538461538,-0.523076923076923,-0.507692307692308,
-0.492307692307692,-0.476923076923077,-0.461538461538462,-0.446153846153846,
-0.430769230769231,-0.415384615384615,-0.4,-0.384615384615385,-0.369230769230769,
-0.353846153846154,-0.338461538461538,-0.323076923076923,-0.307692307692308,
-0.292307692307692,-0.276923076923077,-0.261538461538462,-0.246153846153846,
-0.230769230769231,-0.215384615384615,-0.2,-0.184615384615385,-0.169230769230769,
-0.153846153846154,-0.138461538461538,-0.123076923076923,-0.107692307692308,
-0.0923076923076923,-0.0769230769230769,-0.0615384615384615,-0.0461538461538462,
-0.0307692307692308,-0.0153846153846154,0.),(-1.,1.),.UNSPECIFIED.)
GEOMETRIC_REPRESENTATION_ITEM()
RATIONAL_B_SPLINE_SURFACE(((1.,1.),(1.,1.),(1.,1.),(1.,1.),(1.,1.),(1.,
1.),(1.,1.),(1.,1.),(1.,1.),(1.,1.),(1.,1.),(1.,1.),(1.,1.),(1.,1.),(1.,
1.),(1.,1.),(1.,1.),(1.,1.),(1.,1.),(1.,1.),(1.,1.),(1.,1.),(1.,1.),(1.,
1.),(1.,1.),(1.,1.),(1.,1.),(1.,1.),(1.,1.),(1.,1.),(1.,1.),(1.,1.),(1.,
1.),(1.,1.),(1.,1.),(1.,1.),(1.,1.),(1.,1.),(1.,1.),(1.,1.),(1.,1.),(1.,
1.),(1.,1.),(1.,1.),(1.,1.),(1.,1.),(1.,1.),(1.,1.),(1.,1.),(1.,1.),(1.,
1.),(1.,1.),(1.,1.),(1.,1.),(1.,1.),(1.,1.),(1.,1.),(1.,1.),(1.,1.),(1.,
1.),(1.,1.),(1.,1.),(1.,1.),(1.,1.),(1.,1.),(1.,1.),(1.,1.),(1.,1.),(1.,
1.),(1.,1.)))
REPRESENTATION_ITEM('')
SURFACE()
);
#112=(
BOUNDED_SURFACE()
B_SPLINE_SURFACE(5,1,((#49478,#49479),(#49480,#49481),(#49482,#49483),(#49484,
#49485),(#49486,#49487),(#49488,#49489),(#49490,#49491),(#49492,#49493),
(#49494,#49495),(#49496,#49497),(#49498,#49499),(#49500,#49501),(#49502,
#49503),(#49504,#49505),(#49506,#49507),(#49508,#49509),(#49510,#49511),
(#49512,#49513),(#49514,#49515),(#49516,#49517),(#49518,#49519),(#49520,
#49521),(#49522,#49523),(#49524,#49525),(#49526,#49527),(#49528,#49529),
(#49530,#49531),(#49532,#49533),(#49534,#49535),(#49536,#49537),(#49538,
#49539),(#49540,#49541),(#49542,#49543),(#49544,#49545),(#49546,#49547),
(#49548,#49549),(#49550,#49551),(#49552,#49553),(#49554,#49555),(#49556,
#49557),(#49558,#49559),(#49560,#49561),(#49562,#49563),(#49564,#49565),
(#49566,#49567),(#49568,#49569),(#49570,#49571),(#49572,#49573),(#49574,
#49575),(#49576,#49577),(#49578,#49579),(#49580,#49581),(#49582,#49583),
(#49584,#49585),(#49586,#49587),(#49588,#49589),(#49590,#49591),(#49592,
#49593),(#49594,#49595),(#49596,#49597),(#49598,#49599),(#49600,#49601),
(#49602,#49603),(#49604,#49605),(#49606,#49607),(#49608,#49609),(#49610,
#49611),(#49612,#49613),(#49614,#49615),(#49616,#49617)),.UNSPECIFIED.,
 .F.,.F.,.F.)
B_SPLINE_SURFACE_WITH_KNOTS((6,1,1,1,1,1,1,1,1,1,1,1,1,1,1,1,1,1,1,1,1,
1,1,1,1,1,1,1,1,1,1,1,1,1,1,1,1,1,1,1,1,1,1,1,1,1,1,1,1,1,1,1,1,1,1,1,1,
1,1,1,1,1,1,1,1,6),(2,2),(-1.,-0.984615384615383,-0.969230769230768,-0.953846153846152,
-0.938461538461537,-0.923076923076922,-0.907692307692306,-0.892307692307691,
-0.876923076923076,-0.86153846153846,-0.846153846153845,-0.83076923076923,
-0.815384615384614,-0.799999999999999,-0.784615384615384,-0.769230769230768,
-0.753846153846153,-0.738461538461538,-0.723076923076922,-0.707692307692307,
-0.692307692307692,-0.676923076923076,-0.661538461538461,-0.646153846153846,
-0.63076923076923,-0.615384615384615,-0.6,-0.584615384615384,-0.569230769230769,
-0.553846153846154,-0.538461538461538,-0.523076923076923,-0.507692307692308,
-0.492307692307692,-0.476923076923077,-0.461538461538462,-0.446153846153846,
-0.430769230769231,-0.415384615384615,-0.4,-0.384615384615385,-0.369230769230769,
-0.353846153846154,-0.338461538461538,-0.323076923076923,-0.307692307692308,
-0.292307692307692,-0.276923076923077,-0.261538461538462,-0.246153846153846,
-0.230769230769231,-0.215384615384615,-0.2,-0.184615384615385,-0.169230769230769,
-0.153846153846154,-0.138461538461538,-0.123076923076923,-0.107692307692308,
-0.0923076923076923,-0.0769230769230769,-0.0615384615384615,-0.0461538461538462,
-0.0307692307692308,-0.0153846153846154,0.),(-1.,1.),.UNSPECIFIED.)
GEOMETRIC_REPRESENTATION_ITEM()
RATIONAL_B_SPLINE_SURFACE(((1.,1.),(1.,1.),(1.,1.),(1.,1.),(1.,1.),(1.,
1.),(1.,1.),(1.,1.),(1.,1.),(1.,1.),(1.,1.),(1.,1.),(1.,1.),(1.,1.),(1.,
1.),(1.,1.),(1.,1.),(1.,1.),(1.,1.),(1.,1.),(1.,1.),(1.,1.),(1.,1.),(1.,
1.),(1.,1.),(1.,1.),(1.,1.),(1.,1.),(1.,1.),(1.,1.),(1.,1.),(1.,1.),(1.,
1.),(1.,1.),(1.,1.),(1.,1.),(1.,1.),(1.,1.),(1.,1.),(1.,1.),(1.,1.),(1.,
1.),(1.,1.),(1.,1.),(1.,1.),(1.,1.),(1.,1.),(1.,1.),(1.,1.),(1.,1.),(1.,
1.),(1.,1.),(1.,1.),(1.,1.),(1.,1.),(1.,1.),(1.,1.),(1.,1.),(1.,1.),(1.,
1.),(1.,1.),(1.,1.),(1.,1.),(1.,1.),(1.,1.),(1.,1.),(1.,1.),(1.,1.),(1.,
1.),(1.,1.)))
REPRESENTATION_ITEM('')
SURFACE()
);
#113=(
BOUNDED_SURFACE()
B_SPLINE_SURFACE(5,1,((#49708,#49709),(#49710,#49711),(#49712,#49713),(#49714,
#49715),(#49716,#49717),(#49718,#49719),(#49720,#49721),(#49722,#49723),
(#49724,#49725),(#49726,#49727),(#49728,#49729),(#49730,#49731),(#49732,
#49733),(#49734,#49735),(#49736,#49737),(#49738,#49739),(#49740,#49741),
(#49742,#49743),(#49744,#49745),(#49746,#49747),(#49748,#49749),(#49750,
#49751),(#49752,#49753),(#49754,#49755),(#49756,#49757),(#49758,#49759),
(#49760,#49761),(#49762,#49763),(#49764,#49765),(#49766,#49767),(#49768,
#49769),(#49770,#49771),(#49772,#49773),(#49774,#49775),(#49776,#49777),
(#49778,#49779),(#49780,#49781),(#49782,#49783),(#49784,#49785),(#49786,
#49787),(#49788,#49789),(#49790,#49791),(#49792,#49793),(#49794,#49795),
(#49796,#49797),(#49798,#49799),(#49800,#49801),(#49802,#49803),(#49804,
#49805),(#49806,#49807),(#49808,#49809),(#49810,#49811),(#49812,#49813),
(#49814,#49815),(#49816,#49817),(#49818,#49819),(#49820,#49821),(#49822,
#49823),(#49824,#49825),(#49826,#49827),(#49828,#49829),(#49830,#49831),
(#49832,#49833),(#49834,#49835),(#49836,#49837),(#49838,#49839),(#49840,
#49841),(#49842,#49843),(#49844,#49845),(#49846,#49847)),.UNSPECIFIED.,
 .F.,.F.,.F.)
B_SPLINE_SURFACE_WITH_KNOTS((6,1,1,1,1,1,1,1,1,1,1,1,1,1,1,1,1,1,1,1,1,
1,1,1,1,1,1,1,1,1,1,1,1,1,1,1,1,1,1,1,1,1,1,1,1,1,1,1,1,1,1,1,1,1,1,1,1,
1,1,1,1,1,1,1,1,6),(2,2),(-1.,-0.984615384615383,-0.969230769230768,-0.953846153846152,
-0.938461538461537,-0.923076923076922,-0.907692307692306,-0.892307692307691,
-0.876923076923076,-0.86153846153846,-0.846153846153845,-0.83076923076923,
-0.815384615384614,-0.799999999999999,-0.784615384615384,-0.769230769230768,
-0.753846153846153,-0.738461538461538,-0.723076923076922,-0.707692307692307,
-0.692307692307692,-0.676923076923076,-0.661538461538461,-0.646153846153846,
-0.63076923076923,-0.615384615384615,-0.6,-0.584615384615384,-0.569230769230769,
-0.553846153846154,-0.538461538461538,-0.523076923076923,-0.507692307692308,
-0.492307692307692,-0.476923076923077,-0.461538461538462,-0.446153846153846,
-0.430769230769231,-0.415384615384615,-0.4,-0.384615384615385,-0.369230769230769,
-0.353846153846154,-0.338461538461538,-0.323076923076923,-0.307692307692308,
-0.292307692307692,-0.276923076923077,-0.261538461538462,-0.246153846153846,
-0.230769230769231,-0.215384615384615,-0.2,-0.184615384615385,-0.169230769230769,
-0.153846153846154,-0.138461538461538,-0.123076923076923,-0.107692307692308,
-0.0923076923076923,-0.0769230769230769,-0.0615384615384615,-0.0461538461538462,
-0.0307692307692308,-0.0153846153846154,0.),(-1.,1.),.UNSPECIFIED.)
GEOMETRIC_REPRESENTATION_ITEM()
RATIONAL_B_SPLINE_SURFACE(((1.,1.),(1.,1.),(1.,1.),(1.,1.),(1.,1.),(1.,
1.),(1.,1.),(1.,1.),(1.,1.),(1.,1.),(1.,1.),(1.,1.),(1.,1.),(1.,1.),(1.,
1.),(1.,1.),(1.,1.),(1.,1.),(1.,1.),(1.,1.),(1.,1.),(1.,1.),(1.,1.),(1.,
1.),(1.,1.),(1.,1.),(1.,1.),(1.,1.),(1.,1.),(1.,1.),(1.,1.),(1.,1.),(1.,
1.),(1.,1.),(1.,1.),(1.,1.),(1.,1.),(1.,1.),(1.,1.),(1.,1.),(1.,1.),(1.,
1.),(1.,1.),(1.,1.),(1.,1.),(1.,1.),(1.,1.),(1.,1.),(1.,1.),(1.,1.),(1.,
1.),(1.,1.),(1.,1.),(1.,1.),(1.,1.),(1.,1.),(1.,1.),(1.,1.),(1.,1.),(1.,
1.),(1.,1.),(1.,1.),(1.,1.),(1.,1.),(1.,1.),(1.,1.),(1.,1.),(1.,1.),(1.,
1.),(1.,1.)))
REPRESENTATION_ITEM('')
SURFACE()
);
#114=(
BOUNDED_SURFACE()
B_SPLINE_SURFACE(5,1,((#49920,#49921),(#49922,#49923),(#49924,#49925),(#49926,
#49927),(#49928,#49929),(#49930,#49931),(#49932,#49933),(#49934,#49935),
(#49936,#49937),(#49938,#49939),(#49940,#49941),(#49942,#49943),(#49944,
#49945),(#49946,#49947),(#49948,#49949),(#49950,#49951),(#49952,#49953),
(#49954,#49955),(#49956,#49957),(#49958,#49959),(#49960,#49961),(#49962,
#49963),(#49964,#49965),(#49966,#49967),(#49968,#49969),(#49970,#49971),
(#49972,#49973),(#49974,#49975),(#49976,#49977),(#49978,#49979),(#49980,
#49981),(#49982,#49983),(#49984,#49985),(#49986,#49987),(#49988,#49989),
(#49990,#49991),(#49992,#49993),(#49994,#49995),(#49996,#49997),(#49998,
#49999),(#50000,#50001),(#50002,#50003),(#50004,#50005),(#50006,#50007),
(#50008,#50009),(#50010,#50011),(#50012,#50013),(#50014,#50015),(#50016,
#50017),(#50018,#50019),(#50020,#50021),(#50022,#50023),(#50024,#50025),
(#50026,#50027),(#50028,#50029),(#50030,#50031),(#50032,#50033),(#50034,
#50035),(#50036,#50037),(#50038,#50039),(#50040,#50041),(#50042,#50043),
(#50044,#50045),(#50046,#50047),(#50048,#50049),(#50050,#50051),(#50052,
#50053),(#50054,#50055),(#50056,#50057),(#50058,#50059)),.UNSPECIFIED.,
 .F.,.F.,.F.)
B_SPLINE_SURFACE_WITH_KNOTS((6,1,1,1,1,1,1,1,1,1,1,1,1,1,1,1,1,1,1,1,1,
1,1,1,1,1,1,1,1,1,1,1,1,1,1,1,1,1,1,1,1,1,1,1,1,1,1,1,1,1,1,1,1,1,1,1,1,
1,1,1,1,1,1,1,1,6),(2,2),(-1.,-0.984615384615383,-0.969230769230768,-0.953846153846152,
-0.938461538461537,-0.923076923076922,-0.907692307692306,-0.892307692307691,
-0.876923076923076,-0.86153846153846,-0.846153846153845,-0.83076923076923,
-0.815384615384614,-0.799999999999999,-0.784615384615384,-0.769230769230768,
-0.753846153846153,-0.738461538461538,-0.723076923076922,-0.707692307692307,
-0.692307692307692,-0.676923076923076,-0.661538461538461,-0.646153846153846,
-0.63076923076923,-0.615384615384615,-0.6,-0.584615384615384,-0.569230769230769,
-0.553846153846154,-0.538461538461538,-0.523076923076923,-0.507692307692308,
-0.492307692307692,-0.476923076923077,-0.461538461538462,-0.446153846153846,
-0.430769230769231,-0.415384615384615,-0.4,-0.384615384615385,-0.369230769230769,
-0.353846153846154,-0.338461538461538,-0.323076923076923,-0.307692307692308,
-0.292307692307692,-0.276923076923077,-0.261538461538462,-0.246153846153846,
-0.230769230769231,-0.215384615384615,-0.2,-0.184615384615385,-0.169230769230769,
-0.153846153846154,-0.138461538461538,-0.123076923076923,-0.107692307692308,
-0.0923076923076923,-0.0769230769230769,-0.0615384615384615,-0.0461538461538462,
-0.0307692307692308,-0.0153846153846154,0.),(-1.,1.),.UNSPECIFIED.)
GEOMETRIC_REPRESENTATION_ITEM()
RATIONAL_B_SPLINE_SURFACE(((1.,1.),(1.,1.),(1.,1.),(1.,1.),(1.,1.),(1.,
1.),(1.,1.),(1.,1.),(1.,1.),(1.,1.),(1.,1.),(1.,1.),(1.,1.),(1.,1.),(1.,
1.),(1.,1.),(1.,1.),(1.,1.),(1.,1.),(1.,1.),(1.,1.),(1.,1.),(1.,1.),(1.,
1.),(1.,1.),(1.,1.),(1.,1.),(1.,1.),(1.,1.),(1.,1.),(1.,1.),(1.,1.),(1.,
1.),(1.,1.),(1.,1.),(1.,1.),(1.,1.),(1.,1.),(1.,1.),(1.,1.),(1.,1.),(1.,
1.),(1.,1.),(1.,1.),(1.,1.),(1.,1.),(1.,1.),(1.,1.),(1.,1.),(1.,1.),(1.,
1.),(1.,1.),(1.,1.),(1.,1.),(1.,1.),(1.,1.),(1.,1.),(1.,1.),(1.,1.),(1.,
1.),(1.,1.),(1.,1.),(1.,1.),(1.,1.),(1.,1.),(1.,1.),(1.,1.),(1.,1.),(1.,
1.),(1.,1.)))
REPRESENTATION_ITEM('')
SURFACE()
);
#115=(
BOUNDED_SURFACE()
B_SPLINE_SURFACE(5,1,((#50150,#50151),(#50152,#50153),(#50154,#50155),(#50156,
#50157),(#50158,#50159),(#50160,#50161),(#50162,#50163),(#50164,#50165),
(#50166,#50167),(#50168,#50169),(#50170,#50171),(#50172,#50173),(#50174,
#50175),(#50176,#50177),(#50178,#50179),(#50180,#50181),(#50182,#50183),
(#50184,#50185),(#50186,#50187),(#50188,#50189),(#50190,#50191),(#50192,
#50193),(#50194,#50195),(#50196,#50197),(#50198,#50199),(#50200,#50201),
(#50202,#50203),(#50204,#50205),(#50206,#50207),(#50208,#50209),(#50210,
#50211),(#50212,#50213),(#50214,#50215),(#50216,#50217),(#50218,#50219),
(#50220,#50221),(#50222,#50223),(#50224,#50225),(#50226,#50227),(#50228,
#50229),(#50230,#50231),(#50232,#50233),(#50234,#50235),(#50236,#50237),
(#50238,#50239),(#50240,#50241),(#50242,#50243),(#50244,#50245),(#50246,
#50247),(#50248,#50249),(#50250,#50251),(#50252,#50253),(#50254,#50255),
(#50256,#50257),(#50258,#50259),(#50260,#50261),(#50262,#50263),(#50264,
#50265),(#50266,#50267),(#50268,#50269),(#50270,#50271),(#50272,#50273),
(#50274,#50275),(#50276,#50277),(#50278,#50279),(#50280,#50281),(#50282,
#50283),(#50284,#50285),(#50286,#50287),(#50288,#50289)),.UNSPECIFIED.,
 .F.,.F.,.F.)
B_SPLINE_SURFACE_WITH_KNOTS((6,1,1,1,1,1,1,1,1,1,1,1,1,1,1,1,1,1,1,1,1,
1,1,1,1,1,1,1,1,1,1,1,1,1,1,1,1,1,1,1,1,1,1,1,1,1,1,1,1,1,1,1,1,1,1,1,1,
1,1,1,1,1,1,1,1,6),(2,2),(-1.,-0.984615384615383,-0.969230769230768,-0.953846153846152,
-0.938461538461537,-0.923076923076922,-0.907692307692306,-0.892307692307691,
-0.876923076923076,-0.86153846153846,-0.846153846153845,-0.83076923076923,
-0.815384615384614,-0.799999999999999,-0.784615384615384,-0.769230769230768,
-0.753846153846153,-0.738461538461538,-0.723076923076922,-0.707692307692307,
-0.692307692307692,-0.676923076923076,-0.661538461538461,-0.646153846153846,
-0.63076923076923,-0.615384615384615,-0.6,-0.584615384615384,-0.569230769230769,
-0.553846153846154,-0.538461538461538,-0.523076923076923,-0.507692307692308,
-0.492307692307692,-0.476923076923077,-0.461538461538462,-0.446153846153846,
-0.430769230769231,-0.415384615384615,-0.4,-0.384615384615385,-0.369230769230769,
-0.353846153846154,-0.338461538461538,-0.323076923076923,-0.307692307692308,
-0.292307692307692,-0.276923076923077,-0.261538461538462,-0.246153846153846,
-0.230769230769231,-0.215384615384615,-0.2,-0.184615384615385,-0.169230769230769,
-0.153846153846154,-0.138461538461538,-0.123076923076923,-0.107692307692308,
-0.0923076923076923,-0.0769230769230769,-0.0615384615384615,-0.0461538461538462,
-0.0307692307692308,-0.0153846153846154,0.),(-1.,1.),.UNSPECIFIED.)
GEOMETRIC_REPRESENTATION_ITEM()
RATIONAL_B_SPLINE_SURFACE(((1.,1.),(1.,1.),(1.,1.),(1.,1.),(1.,1.),(1.,
1.),(1.,1.),(1.,1.),(1.,1.),(1.,1.),(1.,1.),(1.,1.),(1.,1.),(1.,1.),(1.,
1.),(1.,1.),(1.,1.),(1.,1.),(1.,1.),(1.,1.),(1.,1.),(1.,1.),(1.,1.),(1.,
1.),(1.,1.),(1.,1.),(1.,1.),(1.,1.),(1.,1.),(1.,1.),(1.,1.),(1.,1.),(1.,
1.),(1.,1.),(1.,1.),(1.,1.),(1.,1.),(1.,1.),(1.,1.),(1.,1.),(1.,1.),(1.,
1.),(1.,1.),(1.,1.),(1.,1.),(1.,1.),(1.,1.),(1.,1.),(1.,1.),(1.,1.),(1.,
1.),(1.,1.),(1.,1.),(1.,1.),(1.,1.),(1.,1.),(1.,1.),(1.,1.),(1.,1.),(1.,
1.),(1.,1.),(1.,1.),(1.,1.),(1.,1.),(1.,1.),(1.,1.),(1.,1.),(1.,1.),(1.,
1.),(1.,1.)))
REPRESENTATION_ITEM('')
SURFACE()
);
#116=(
BOUNDED_SURFACE()
B_SPLINE_SURFACE(5,1,((#50362,#50363),(#50364,#50365),(#50366,#50367),(#50368,
#50369),(#50370,#50371),(#50372,#50373),(#50374,#50375),(#50376,#50377),
(#50378,#50379),(#50380,#50381),(#50382,#50383),(#50384,#50385),(#50386,
#50387),(#50388,#50389),(#50390,#50391),(#50392,#50393),(#50394,#50395),
(#50396,#50397),(#50398,#50399),(#50400,#50401),(#50402,#50403),(#50404,
#50405),(#50406,#50407),(#50408,#50409),(#50410,#50411),(#50412,#50413),
(#50414,#50415),(#50416,#50417),(#50418,#50419),(#50420,#50421),(#50422,
#50423),(#50424,#50425),(#50426,#50427),(#50428,#50429),(#50430,#50431),
(#50432,#50433),(#50434,#50435),(#50436,#50437),(#50438,#50439),(#50440,
#50441),(#50442,#50443),(#50444,#50445),(#50446,#50447),(#50448,#50449),
(#50450,#50451),(#50452,#50453),(#50454,#50455),(#50456,#50457),(#50458,
#50459),(#50460,#50461),(#50462,#50463),(#50464,#50465),(#50466,#50467),
(#50468,#50469),(#50470,#50471),(#50472,#50473),(#50474,#50475),(#50476,
#50477),(#50478,#50479),(#50480,#50481),(#50482,#50483),(#50484,#50485),
(#50486,#50487),(#50488,#50489),(#50490,#50491),(#50492,#50493),(#50494,
#50495),(#50496,#50497),(#50498,#50499),(#50500,#50501)),.UNSPECIFIED.,
 .F.,.F.,.F.)
B_SPLINE_SURFACE_WITH_KNOTS((6,1,1,1,1,1,1,1,1,1,1,1,1,1,1,1,1,1,1,1,1,
1,1,1,1,1,1,1,1,1,1,1,1,1,1,1,1,1,1,1,1,1,1,1,1,1,1,1,1,1,1,1,1,1,1,1,1,
1,1,1,1,1,1,1,1,6),(2,2),(-1.,-0.984615384615383,-0.969230769230768,-0.953846153846152,
-0.938461538461537,-0.923076923076922,-0.907692307692306,-0.892307692307691,
-0.876923076923076,-0.86153846153846,-0.846153846153845,-0.83076923076923,
-0.815384615384614,-0.799999999999999,-0.784615384615384,-0.769230769230768,
-0.753846153846153,-0.738461538461538,-0.723076923076922,-0.707692307692307,
-0.692307692307692,-0.676923076923076,-0.661538461538461,-0.646153846153846,
-0.63076923076923,-0.615384615384615,-0.6,-0.584615384615384,-0.569230769230769,
-0.553846153846154,-0.538461538461538,-0.523076923076923,-0.507692307692308,
-0.492307692307692,-0.476923076923077,-0.461538461538462,-0.446153846153846,
-0.430769230769231,-0.415384615384615,-0.4,-0.384615384615385,-0.369230769230769,
-0.353846153846154,-0.338461538461538,-0.323076923076923,-0.307692307692308,
-0.292307692307692,-0.276923076923077,-0.261538461538462,-0.246153846153846,
-0.230769230769231,-0.215384615384615,-0.2,-0.184615384615385,-0.169230769230769,
-0.153846153846154,-0.138461538461538,-0.123076923076923,-0.107692307692308,
-0.0923076923076923,-0.0769230769230769,-0.0615384615384615,-0.0461538461538462,
-0.0307692307692308,-0.0153846153846154,0.),(-1.,1.),.UNSPECIFIED.)
GEOMETRIC_REPRESENTATION_ITEM()
RATIONAL_B_SPLINE_SURFACE(((1.,1.),(1.,1.),(1.,1.),(1.,1.),(1.,1.),(1.,
1.),(1.,1.),(1.,1.),(1.,1.),(1.,1.),(1.,1.),(1.,1.),(1.,1.),(1.,1.),(1.,
1.),(1.,1.),(1.,1.),(1.,1.),(1.,1.),(1.,1.),(1.,1.),(1.,1.),(1.,1.),(1.,
1.),(1.,1.),(1.,1.),(1.,1.),(1.,1.),(1.,1.),(1.,1.),(1.,1.),(1.,1.),(1.,
1.),(1.,1.),(1.,1.),(1.,1.),(1.,1.),(1.,1.),(1.,1.),(1.,1.),(1.,1.),(1.,
1.),(1.,1.),(1.,1.),(1.,1.),(1.,1.),(1.,1.),(1.,1.),(1.,1.),(1.,1.),(1.,
1.),(1.,1.),(1.,1.),(1.,1.),(1.,1.),(1.,1.),(1.,1.),(1.,1.),(1.,1.),(1.,
1.),(1.,1.),(1.,1.),(1.,1.),(1.,1.),(1.,1.),(1.,1.),(1.,1.),(1.,1.),(1.,
1.),(1.,1.)))
REPRESENTATION_ITEM('')
SURFACE()
);
#117=(
BOUNDED_SURFACE()
B_SPLINE_SURFACE(5,1,((#50592,#50593),(#50594,#50595),(#50596,#50597),(#50598,
#50599),(#50600,#50601),(#50602,#50603),(#50604,#50605),(#50606,#50607),
(#50608,#50609),(#50610,#50611),(#50612,#50613),(#50614,#50615),(#50616,
#50617),(#50618,#50619),(#50620,#50621),(#50622,#50623),(#50624,#50625),
(#50626,#50627),(#50628,#50629),(#50630,#50631),(#50632,#50633),(#50634,
#50635),(#50636,#50637),(#50638,#50639),(#50640,#50641),(#50642,#50643),
(#50644,#50645),(#50646,#50647),(#50648,#50649),(#50650,#50651),(#50652,
#50653),(#50654,#50655),(#50656,#50657),(#50658,#50659),(#50660,#50661),
(#50662,#50663),(#50664,#50665),(#50666,#50667),(#50668,#50669),(#50670,
#50671),(#50672,#50673),(#50674,#50675),(#50676,#50677),(#50678,#50679),
(#50680,#50681),(#50682,#50683),(#50684,#50685),(#50686,#50687),(#50688,
#50689),(#50690,#50691),(#50692,#50693),(#50694,#50695),(#50696,#50697),
(#50698,#50699),(#50700,#50701),(#50702,#50703),(#50704,#50705),(#50706,
#50707),(#50708,#50709),(#50710,#50711),(#50712,#50713),(#50714,#50715),
(#50716,#50717),(#50718,#50719),(#50720,#50721),(#50722,#50723),(#50724,
#50725),(#50726,#50727),(#50728,#50729),(#50730,#50731)),.UNSPECIFIED.,
 .F.,.F.,.F.)
B_SPLINE_SURFACE_WITH_KNOTS((6,1,1,1,1,1,1,1,1,1,1,1,1,1,1,1,1,1,1,1,1,
1,1,1,1,1,1,1,1,1,1,1,1,1,1,1,1,1,1,1,1,1,1,1,1,1,1,1,1,1,1,1,1,1,1,1,1,
1,1,1,1,1,1,1,1,6),(2,2),(-1.,-0.984615384615383,-0.969230769230768,-0.953846153846152,
-0.938461538461537,-0.923076923076922,-0.907692307692306,-0.892307692307691,
-0.876923076923076,-0.86153846153846,-0.846153846153845,-0.83076923076923,
-0.815384615384614,-0.799999999999999,-0.784615384615384,-0.769230769230768,
-0.753846153846153,-0.738461538461538,-0.723076923076922,-0.707692307692307,
-0.692307692307692,-0.676923076923076,-0.661538461538461,-0.646153846153846,
-0.63076923076923,-0.615384615384615,-0.6,-0.584615384615384,-0.569230769230769,
-0.553846153846154,-0.538461538461538,-0.523076923076923,-0.507692307692308,
-0.492307692307692,-0.476923076923077,-0.461538461538462,-0.446153846153846,
-0.430769230769231,-0.415384615384615,-0.4,-0.384615384615385,-0.369230769230769,
-0.353846153846154,-0.338461538461538,-0.323076923076923,-0.307692307692308,
-0.292307692307692,-0.276923076923077,-0.261538461538462,-0.246153846153846,
-0.230769230769231,-0.215384615384615,-0.2,-0.184615384615385,-0.169230769230769,
-0.153846153846154,-0.138461538461538,-0.123076923076923,-0.107692307692308,
-0.0923076923076923,-0.0769230769230769,-0.0615384615384615,-0.0461538461538462,
-0.0307692307692308,-0.0153846153846154,0.),(-1.,1.),.UNSPECIFIED.)
GEOMETRIC_REPRESENTATION_ITEM()
RATIONAL_B_SPLINE_SURFACE(((1.,1.),(1.,1.),(1.,1.),(1.,1.),(1.,1.),(1.,
1.),(1.,1.),(1.,1.),(1.,1.),(1.,1.),(1.,1.),(1.,1.),(1.,1.),(1.,1.),(1.,
1.),(1.,1.),(1.,1.),(1.,1.),(1.,1.),(1.,1.),(1.,1.),(1.,1.),(1.,1.),(1.,
1.),(1.,1.),(1.,1.),(1.,1.),(1.,1.),(1.,1.),(1.,1.),(1.,1.),(1.,1.),(1.,
1.),(1.,1.),(1.,1.),(1.,1.),(1.,1.),(1.,1.),(1.,1.),(1.,1.),(1.,1.),(1.,
1.),(1.,1.),(1.,1.),(1.,1.),(1.,1.),(1.,1.),(1.,1.),(1.,1.),(1.,1.),(1.,
1.),(1.,1.),(1.,1.),(1.,1.),(1.,1.),(1.,1.),(1.,1.),(1.,1.),(1.,1.),(1.,
1.),(1.,1.),(1.,1.),(1.,1.),(1.,1.),(1.,1.),(1.,1.),(1.,1.),(1.,1.),(1.,
1.),(1.,1.)))
REPRESENTATION_ITEM('')
SURFACE()
);
#118=(
BOUNDED_SURFACE()
B_SPLINE_SURFACE(5,1,((#50804,#50805),(#50806,#50807),(#50808,#50809),(#50810,
#50811),(#50812,#50813),(#50814,#50815),(#50816,#50817),(#50818,#50819),
(#50820,#50821),(#50822,#50823),(#50824,#50825),(#50826,#50827),(#50828,
#50829),(#50830,#50831),(#50832,#50833),(#50834,#50835),(#50836,#50837),
(#50838,#50839),(#50840,#50841),(#50842,#50843),(#50844,#50845),(#50846,
#50847),(#50848,#50849),(#50850,#50851),(#50852,#50853),(#50854,#50855),
(#50856,#50857),(#50858,#50859),(#50860,#50861),(#50862,#50863),(#50864,
#50865),(#50866,#50867),(#50868,#50869),(#50870,#50871),(#50872,#50873),
(#50874,#50875),(#50876,#50877),(#50878,#50879),(#50880,#50881),(#50882,
#50883),(#50884,#50885),(#50886,#50887),(#50888,#50889),(#50890,#50891),
(#50892,#50893),(#50894,#50895),(#50896,#50897),(#50898,#50899),(#50900,
#50901),(#50902,#50903),(#50904,#50905),(#50906,#50907),(#50908,#50909),
(#50910,#50911),(#50912,#50913),(#50914,#50915),(#50916,#50917),(#50918,
#50919),(#50920,#50921),(#50922,#50923),(#50924,#50925),(#50926,#50927),
(#50928,#50929),(#50930,#50931),(#50932,#50933),(#50934,#50935),(#50936,
#50937),(#50938,#50939),(#50940,#50941),(#50942,#50943)),.UNSPECIFIED.,
 .F.,.F.,.F.)
B_SPLINE_SURFACE_WITH_KNOTS((6,1,1,1,1,1,1,1,1,1,1,1,1,1,1,1,1,1,1,1,1,
1,1,1,1,1,1,1,1,1,1,1,1,1,1,1,1,1,1,1,1,1,1,1,1,1,1,1,1,1,1,1,1,1,1,1,1,
1,1,1,1,1,1,1,1,6),(2,2),(-1.,-0.984615384615383,-0.969230769230768,-0.953846153846152,
-0.938461538461537,-0.923076923076922,-0.907692307692306,-0.892307692307691,
-0.876923076923076,-0.86153846153846,-0.846153846153845,-0.83076923076923,
-0.815384615384614,-0.799999999999999,-0.784615384615384,-0.769230769230768,
-0.753846153846153,-0.738461538461538,-0.723076923076922,-0.707692307692307,
-0.692307692307692,-0.676923076923076,-0.661538461538461,-0.646153846153846,
-0.63076923076923,-0.615384615384615,-0.6,-0.584615384615384,-0.569230769230769,
-0.553846153846154,-0.538461538461538,-0.523076923076923,-0.507692307692308,
-0.492307692307692,-0.476923076923077,-0.461538461538462,-0.446153846153846,
-0.430769230769231,-0.415384615384615,-0.4,-0.384615384615385,-0.369230769230769,
-0.353846153846154,-0.338461538461538,-0.323076923076923,-0.307692307692308,
-0.292307692307692,-0.276923076923077,-0.261538461538462,-0.246153846153846,
-0.230769230769231,-0.215384615384615,-0.2,-0.184615384615385,-0.169230769230769,
-0.153846153846154,-0.138461538461538,-0.123076923076923,-0.107692307692308,
-0.0923076923076923,-0.0769230769230769,-0.0615384615384615,-0.0461538461538462,
-0.0307692307692308,-0.0153846153846154,0.),(-1.,1.),.UNSPECIFIED.)
GEOMETRIC_REPRESENTATION_ITEM()
RATIONAL_B_SPLINE_SURFACE(((1.,1.),(1.,1.),(1.,1.),(1.,1.),(1.,1.),(1.,
1.),(1.,1.),(1.,1.),(1.,1.),(1.,1.),(1.,1.),(1.,1.),(1.,1.),(1.,1.),(1.,
1.),(1.,1.),(1.,1.),(1.,1.),(1.,1.),(1.,1.),(1.,1.),(1.,1.),(1.,1.),(1.,
1.),(1.,1.),(1.,1.),(1.,1.),(1.,1.),(1.,1.),(1.,1.),(1.,1.),(1.,1.),(1.,
1.),(1.,1.),(1.,1.),(1.,1.),(1.,1.),(1.,1.),(1.,1.),(1.,1.),(1.,1.),(1.,
1.),(1.,1.),(1.,1.),(1.,1.),(1.,1.),(1.,1.),(1.,1.),(1.,1.),(1.,1.),(1.,
1.),(1.,1.),(1.,1.),(1.,1.),(1.,1.),(1.,1.),(1.,1.),(1.,1.),(1.,1.),(1.,
1.),(1.,1.),(1.,1.),(1.,1.),(1.,1.),(1.,1.),(1.,1.),(1.,1.),(1.,1.),(1.,
1.),(1.,1.)))
REPRESENTATION_ITEM('')
SURFACE()
);
#119=(
BOUNDED_SURFACE()
B_SPLINE_SURFACE(5,1,((#51034,#51035),(#51036,#51037),(#51038,#51039),(#51040,
#51041),(#51042,#51043),(#51044,#51045),(#51046,#51047),(#51048,#51049),
(#51050,#51051),(#51052,#51053),(#51054,#51055),(#51056,#51057),(#51058,
#51059),(#51060,#51061),(#51062,#51063),(#51064,#51065),(#51066,#51067),
(#51068,#51069),(#51070,#51071),(#51072,#51073),(#51074,#51075),(#51076,
#51077),(#51078,#51079),(#51080,#51081),(#51082,#51083),(#51084,#51085),
(#51086,#51087),(#51088,#51089),(#51090,#51091),(#51092,#51093),(#51094,
#51095),(#51096,#51097),(#51098,#51099),(#51100,#51101),(#51102,#51103),
(#51104,#51105),(#51106,#51107),(#51108,#51109),(#51110,#51111),(#51112,
#51113),(#51114,#51115),(#51116,#51117),(#51118,#51119),(#51120,#51121),
(#51122,#51123),(#51124,#51125),(#51126,#51127),(#51128,#51129),(#51130,
#51131),(#51132,#51133),(#51134,#51135),(#51136,#51137),(#51138,#51139),
(#51140,#51141),(#51142,#51143),(#51144,#51145),(#51146,#51147),(#51148,
#51149),(#51150,#51151),(#51152,#51153),(#51154,#51155),(#51156,#51157),
(#51158,#51159),(#51160,#51161),(#51162,#51163),(#51164,#51165),(#51166,
#51167),(#51168,#51169),(#51170,#51171),(#51172,#51173)),.UNSPECIFIED.,
 .F.,.F.,.F.)
B_SPLINE_SURFACE_WITH_KNOTS((6,1,1,1,1,1,1,1,1,1,1,1,1,1,1,1,1,1,1,1,1,
1,1,1,1,1,1,1,1,1,1,1,1,1,1,1,1,1,1,1,1,1,1,1,1,1,1,1,1,1,1,1,1,1,1,1,1,
1,1,1,1,1,1,1,1,6),(2,2),(-1.,-0.984615384615383,-0.969230769230768,-0.953846153846152,
-0.938461538461537,-0.923076923076922,-0.907692307692306,-0.892307692307691,
-0.876923076923076,-0.86153846153846,-0.846153846153845,-0.83076923076923,
-0.815384615384614,-0.799999999999999,-0.784615384615384,-0.769230769230768,
-0.753846153846153,-0.738461538461538,-0.723076923076922,-0.707692307692307,
-0.692307692307692,-0.676923076923076,-0.661538461538461,-0.646153846153846,
-0.63076923076923,-0.615384615384615,-0.6,-0.584615384615384,-0.569230769230769,
-0.553846153846154,-0.538461538461538,-0.523076923076923,-0.507692307692308,
-0.492307692307692,-0.476923076923077,-0.461538461538462,-0.446153846153846,
-0.430769230769231,-0.415384615384615,-0.4,-0.384615384615385,-0.369230769230769,
-0.353846153846154,-0.338461538461538,-0.323076923076923,-0.307692307692308,
-0.292307692307692,-0.276923076923077,-0.261538461538462,-0.246153846153846,
-0.230769230769231,-0.215384615384615,-0.2,-0.184615384615385,-0.169230769230769,
-0.153846153846154,-0.138461538461538,-0.123076923076923,-0.107692307692308,
-0.0923076923076923,-0.0769230769230769,-0.0615384615384615,-0.0461538461538462,
-0.0307692307692308,-0.0153846153846154,0.),(-1.,1.),.UNSPECIFIED.)
GEOMETRIC_REPRESENTATION_ITEM()
RATIONAL_B_SPLINE_SURFACE(((1.,1.),(1.,1.),(1.,1.),(1.,1.),(1.,1.),(1.,
1.),(1.,1.),(1.,1.),(1.,1.),(1.,1.),(1.,1.),(1.,1.),(1.,1.),(1.,1.),(1.,
1.),(1.,1.),(1.,1.),(1.,1.),(1.,1.),(1.,1.),(1.,1.),(1.,1.),(1.,1.),(1.,
1.),(1.,1.),(1.,1.),(1.,1.),(1.,1.),(1.,1.),(1.,1.),(1.,1.),(1.,1.),(1.,
1.),(1.,1.),(1.,1.),(1.,1.),(1.,1.),(1.,1.),(1.,1.),(1.,1.),(1.,1.),(1.,
1.),(1.,1.),(1.,1.),(1.,1.),(1.,1.),(1.,1.),(1.,1.),(1.,1.),(1.,1.),(1.,
1.),(1.,1.),(1.,1.),(1.,1.),(1.,1.),(1.,1.),(1.,1.),(1.,1.),(1.,1.),(1.,
1.),(1.,1.),(1.,1.),(1.,1.),(1.,1.),(1.,1.),(1.,1.),(1.,1.),(1.,1.),(1.,
1.),(1.,1.)))
REPRESENTATION_ITEM('')
SURFACE()
);
#120=(
BOUNDED_SURFACE()
B_SPLINE_SURFACE(5,1,((#51246,#51247),(#51248,#51249),(#51250,#51251),(#51252,
#51253),(#51254,#51255),(#51256,#51257),(#51258,#51259),(#51260,#51261),
(#51262,#51263),(#51264,#51265),(#51266,#51267),(#51268,#51269),(#51270,
#51271),(#51272,#51273),(#51274,#51275),(#51276,#51277),(#51278,#51279),
(#51280,#51281),(#51282,#51283),(#51284,#51285),(#51286,#51287),(#51288,
#51289),(#51290,#51291),(#51292,#51293),(#51294,#51295),(#51296,#51297),
(#51298,#51299),(#51300,#51301),(#51302,#51303),(#51304,#51305),(#51306,
#51307),(#51308,#51309),(#51310,#51311),(#51312,#51313),(#51314,#51315),
(#51316,#51317),(#51318,#51319),(#51320,#51321),(#51322,#51323),(#51324,
#51325),(#51326,#51327),(#51328,#51329),(#51330,#51331),(#51332,#51333),
(#51334,#51335),(#51336,#51337),(#51338,#51339),(#51340,#51341),(#51342,
#51343),(#51344,#51345),(#51346,#51347),(#51348,#51349),(#51350,#51351),
(#51352,#51353),(#51354,#51355),(#51356,#51357),(#51358,#51359),(#51360,
#51361),(#51362,#51363),(#51364,#51365),(#51366,#51367),(#51368,#51369),
(#51370,#51371),(#51372,#51373),(#51374,#51375),(#51376,#51377),(#51378,
#51379),(#51380,#51381),(#51382,#51383),(#51384,#51385)),.UNSPECIFIED.,
 .F.,.F.,.F.)
B_SPLINE_SURFACE_WITH_KNOTS((6,1,1,1,1,1,1,1,1,1,1,1,1,1,1,1,1,1,1,1,1,
1,1,1,1,1,1,1,1,1,1,1,1,1,1,1,1,1,1,1,1,1,1,1,1,1,1,1,1,1,1,1,1,1,1,1,1,
1,1,1,1,1,1,1,1,6),(2,2),(-1.,-0.984615384615383,-0.969230769230768,-0.953846153846152,
-0.938461538461537,-0.923076923076922,-0.907692307692306,-0.892307692307691,
-0.876923076923076,-0.86153846153846,-0.846153846153845,-0.83076923076923,
-0.815384615384614,-0.799999999999999,-0.784615384615384,-0.769230769230768,
-0.753846153846153,-0.738461538461538,-0.723076923076922,-0.707692307692307,
-0.692307692307692,-0.676923076923076,-0.661538461538461,-0.646153846153846,
-0.63076923076923,-0.615384615384615,-0.6,-0.584615384615384,-0.569230769230769,
-0.553846153846154,-0.538461538461538,-0.523076923076923,-0.507692307692308,
-0.492307692307692,-0.476923076923077,-0.461538461538462,-0.446153846153846,
-0.430769230769231,-0.415384615384615,-0.4,-0.384615384615385,-0.369230769230769,
-0.353846153846154,-0.338461538461538,-0.323076923076923,-0.307692307692308,
-0.292307692307692,-0.276923076923077,-0.261538461538462,-0.246153846153846,
-0.230769230769231,-0.215384615384615,-0.2,-0.184615384615385,-0.169230769230769,
-0.153846153846154,-0.138461538461538,-0.123076923076923,-0.107692307692308,
-0.0923076923076923,-0.0769230769230769,-0.0615384615384615,-0.0461538461538462,
-0.0307692307692308,-0.0153846153846154,0.),(-1.,1.),.UNSPECIFIED.)
GEOMETRIC_REPRESENTATION_ITEM()
RATIONAL_B_SPLINE_SURFACE(((1.,1.),(1.,1.),(1.,1.),(1.,1.),(1.,1.),(1.,
1.),(1.,1.),(1.,1.),(1.,1.),(1.,1.),(1.,1.),(1.,1.),(1.,1.),(1.,1.),(1.,
1.),(1.,1.),(1.,1.),(1.,1.),(1.,1.),(1.,1.),(1.,1.),(1.,1.),(1.,1.),(1.,
1.),(1.,1.),(1.,1.),(1.,1.),(1.,1.),(1.,1.),(1.,1.),(1.,1.),(1.,1.),(1.,
1.),(1.,1.),(1.,1.),(1.,1.),(1.,1.),(1.,1.),(1.,1.),(1.,1.),(1.,1.),(1.,
1.),(1.,1.),(1.,1.),(1.,1.),(1.,1.),(1.,1.),(1.,1.),(1.,1.),(1.,1.),(1.,
1.),(1.,1.),(1.,1.),(1.,1.),(1.,1.),(1.,1.),(1.,1.),(1.,1.),(1.,1.),(1.,
1.),(1.,1.),(1.,1.),(1.,1.),(1.,1.),(1.,1.),(1.,1.),(1.,1.),(1.,1.),(1.,
1.),(1.,1.)))
REPRESENTATION_ITEM('')
SURFACE()
);
#121=(
BOUNDED_SURFACE()
B_SPLINE_SURFACE(5,1,((#51476,#51477),(#51478,#51479),(#51480,#51481),(#51482,
#51483),(#51484,#51485),(#51486,#51487),(#51488,#51489),(#51490,#51491),
(#51492,#51493),(#51494,#51495),(#51496,#51497),(#51498,#51499),(#51500,
#51501),(#51502,#51503),(#51504,#51505),(#51506,#51507),(#51508,#51509),
(#51510,#51511),(#51512,#51513),(#51514,#51515),(#51516,#51517),(#51518,
#51519),(#51520,#51521),(#51522,#51523),(#51524,#51525),(#51526,#51527),
(#51528,#51529),(#51530,#51531),(#51532,#51533),(#51534,#51535),(#51536,
#51537),(#51538,#51539),(#51540,#51541),(#51542,#51543),(#51544,#51545),
(#51546,#51547),(#51548,#51549),(#51550,#51551),(#51552,#51553),(#51554,
#51555),(#51556,#51557),(#51558,#51559),(#51560,#51561),(#51562,#51563),
(#51564,#51565),(#51566,#51567),(#51568,#51569),(#51570,#51571),(#51572,
#51573),(#51574,#51575),(#51576,#51577),(#51578,#51579),(#51580,#51581),
(#51582,#51583),(#51584,#51585),(#51586,#51587),(#51588,#51589),(#51590,
#51591),(#51592,#51593),(#51594,#51595),(#51596,#51597),(#51598,#51599),
(#51600,#51601),(#51602,#51603),(#51604,#51605),(#51606,#51607),(#51608,
#51609),(#51610,#51611),(#51612,#51613),(#51614,#51615)),.UNSPECIFIED.,
 .F.,.F.,.F.)
B_SPLINE_SURFACE_WITH_KNOTS((6,1,1,1,1,1,1,1,1,1,1,1,1,1,1,1,1,1,1,1,1,
1,1,1,1,1,1,1,1,1,1,1,1,1,1,1,1,1,1,1,1,1,1,1,1,1,1,1,1,1,1,1,1,1,1,1,1,
1,1,1,1,1,1,1,1,6),(2,2),(-1.,-0.984615384615383,-0.969230769230768,-0.953846153846152,
-0.938461538461537,-0.923076923076922,-0.907692307692306,-0.892307692307691,
-0.876923076923076,-0.86153846153846,-0.846153846153845,-0.83076923076923,
-0.815384615384614,-0.799999999999999,-0.784615384615384,-0.769230769230768,
-0.753846153846153,-0.738461538461538,-0.723076923076922,-0.707692307692307,
-0.692307692307692,-0.676923076923076,-0.661538461538461,-0.646153846153846,
-0.63076923076923,-0.615384615384615,-0.6,-0.584615384615384,-0.569230769230769,
-0.553846153846154,-0.538461538461538,-0.523076923076923,-0.507692307692308,
-0.492307692307692,-0.476923076923077,-0.461538461538462,-0.446153846153846,
-0.430769230769231,-0.415384615384615,-0.4,-0.384615384615385,-0.369230769230769,
-0.353846153846154,-0.338461538461538,-0.323076923076923,-0.307692307692308,
-0.292307692307692,-0.276923076923077,-0.261538461538462,-0.246153846153846,
-0.230769230769231,-0.215384615384615,-0.2,-0.184615384615385,-0.169230769230769,
-0.153846153846154,-0.138461538461538,-0.123076923076923,-0.107692307692308,
-0.0923076923076923,-0.0769230769230769,-0.0615384615384615,-0.0461538461538462,
-0.0307692307692308,-0.0153846153846154,0.),(-1.,1.),.UNSPECIFIED.)
GEOMETRIC_REPRESENTATION_ITEM()
RATIONAL_B_SPLINE_SURFACE(((1.,1.),(1.,1.),(1.,1.),(1.,1.),(1.,1.),(1.,
1.),(1.,1.),(1.,1.),(1.,1.),(1.,1.),(1.,1.),(1.,1.),(1.,1.),(1.,1.),(1.,
1.),(1.,1.),(1.,1.),(1.,1.),(1.,1.),(1.,1.),(1.,1.),(1.,1.),(1.,1.),(1.,
1.),(1.,1.),(1.,1.),(1.,1.),(1.,1.),(1.,1.),(1.,1.),(1.,1.),(1.,1.),(1.,
1.),(1.,1.),(1.,1.),(1.,1.),(1.,1.),(1.,1.),(1.,1.),(1.,1.),(1.,1.),(1.,
1.),(1.,1.),(1.,1.),(1.,1.),(1.,1.),(1.,1.),(1.,1.),(1.,1.),(1.,1.),(1.,
1.),(1.,1.),(1.,1.),(1.,1.),(1.,1.),(1.,1.),(1.,1.),(1.,1.),(1.,1.),(1.,
1.),(1.,1.),(1.,1.),(1.,1.),(1.,1.),(1.,1.),(1.,1.),(1.,1.),(1.,1.),(1.,
1.),(1.,1.)))
REPRESENTATION_ITEM('')
SURFACE()
);
#122=(
BOUNDED_SURFACE()
B_SPLINE_SURFACE(5,1,((#51688,#51689),(#51690,#51691),(#51692,#51693),(#51694,
#51695),(#51696,#51697),(#51698,#51699),(#51700,#51701),(#51702,#51703),
(#51704,#51705),(#51706,#51707),(#51708,#51709),(#51710,#51711),(#51712,
#51713),(#51714,#51715),(#51716,#51717),(#51718,#51719),(#51720,#51721),
(#51722,#51723),(#51724,#51725),(#51726,#51727),(#51728,#51729),(#51730,
#51731),(#51732,#51733),(#51734,#51735),(#51736,#51737),(#51738,#51739),
(#51740,#51741),(#51742,#51743),(#51744,#51745),(#51746,#51747),(#51748,
#51749),(#51750,#51751),(#51752,#51753),(#51754,#51755),(#51756,#51757),
(#51758,#51759),(#51760,#51761),(#51762,#51763),(#51764,#51765),(#51766,
#51767),(#51768,#51769),(#51770,#51771),(#51772,#51773),(#51774,#51775),
(#51776,#51777),(#51778,#51779),(#51780,#51781),(#51782,#51783),(#51784,
#51785),(#51786,#51787),(#51788,#51789),(#51790,#51791),(#51792,#51793),
(#51794,#51795),(#51796,#51797),(#51798,#51799),(#51800,#51801),(#51802,
#51803),(#51804,#51805),(#51806,#51807),(#51808,#51809),(#51810,#51811),
(#51812,#51813),(#51814,#51815),(#51816,#51817),(#51818,#51819),(#51820,
#51821),(#51822,#51823),(#51824,#51825),(#51826,#51827)),.UNSPECIFIED.,
 .F.,.F.,.F.)
B_SPLINE_SURFACE_WITH_KNOTS((6,1,1,1,1,1,1,1,1,1,1,1,1,1,1,1,1,1,1,1,1,
1,1,1,1,1,1,1,1,1,1,1,1,1,1,1,1,1,1,1,1,1,1,1,1,1,1,1,1,1,1,1,1,1,1,1,1,
1,1,1,1,1,1,1,1,6),(2,2),(-1.,-0.984615384615383,-0.969230769230768,-0.953846153846152,
-0.938461538461537,-0.923076923076922,-0.907692307692306,-0.892307692307691,
-0.876923076923076,-0.86153846153846,-0.846153846153845,-0.83076923076923,
-0.815384615384614,-0.799999999999999,-0.784615384615384,-0.769230769230768,
-0.753846153846153,-0.738461538461538,-0.723076923076922,-0.707692307692307,
-0.692307692307692,-0.676923076923076,-0.661538461538461,-0.646153846153846,
-0.63076923076923,-0.615384615384615,-0.6,-0.584615384615384,-0.569230769230769,
-0.553846153846154,-0.538461538461538,-0.523076923076923,-0.507692307692308,
-0.492307692307692,-0.476923076923077,-0.461538461538462,-0.446153846153846,
-0.430769230769231,-0.415384615384615,-0.4,-0.384615384615385,-0.369230769230769,
-0.353846153846154,-0.338461538461538,-0.323076923076923,-0.307692307692308,
-0.292307692307692,-0.276923076923077,-0.261538461538462,-0.246153846153846,
-0.230769230769231,-0.215384615384615,-0.2,-0.184615384615385,-0.169230769230769,
-0.153846153846154,-0.138461538461538,-0.123076923076923,-0.107692307692308,
-0.0923076923076923,-0.0769230769230769,-0.0615384615384615,-0.0461538461538462,
-0.0307692307692308,-0.0153846153846154,0.),(-1.,1.),.UNSPECIFIED.)
GEOMETRIC_REPRESENTATION_ITEM()
RATIONAL_B_SPLINE_SURFACE(((1.,1.),(1.,1.),(1.,1.),(1.,1.),(1.,1.),(1.,
1.),(1.,1.),(1.,1.),(1.,1.),(1.,1.),(1.,1.),(1.,1.),(1.,1.),(1.,1.),(1.,
1.),(1.,1.),(1.,1.),(1.,1.),(1.,1.),(1.,1.),(1.,1.),(1.,1.),(1.,1.),(1.,
1.),(1.,1.),(1.,1.),(1.,1.),(1.,1.),(1.,1.),(1.,1.),(1.,1.),(1.,1.),(1.,
1.),(1.,1.),(1.,1.),(1.,1.),(1.,1.),(1.,1.),(1.,1.),(1.,1.),(1.,1.),(1.,
1.),(1.,1.),(1.,1.),(1.,1.),(1.,1.),(1.,1.),(1.,1.),(1.,1.),(1.,1.),(1.,
1.),(1.,1.),(1.,1.),(1.,1.),(1.,1.),(1.,1.),(1.,1.),(1.,1.),(1.,1.),(1.,
1.),(1.,1.),(1.,1.),(1.,1.),(1.,1.),(1.,1.),(1.,1.),(1.,1.),(1.,1.),(1.,
1.),(1.,1.)))
REPRESENTATION_ITEM('')
SURFACE()
);
#123=(
BOUNDED_SURFACE()
B_SPLINE_SURFACE(5,1,((#51918,#51919),(#51920,#51921),(#51922,#51923),(#51924,
#51925),(#51926,#51927),(#51928,#51929),(#51930,#51931),(#51932,#51933),
(#51934,#51935),(#51936,#51937),(#51938,#51939),(#51940,#51941),(#51942,
#51943),(#51944,#51945),(#51946,#51947),(#51948,#51949),(#51950,#51951),
(#51952,#51953),(#51954,#51955),(#51956,#51957),(#51958,#51959),(#51960,
#51961),(#51962,#51963),(#51964,#51965),(#51966,#51967),(#51968,#51969),
(#51970,#51971),(#51972,#51973),(#51974,#51975),(#51976,#51977),(#51978,
#51979),(#51980,#51981),(#51982,#51983),(#51984,#51985),(#51986,#51987),
(#51988,#51989),(#51990,#51991),(#51992,#51993),(#51994,#51995),(#51996,
#51997),(#51998,#51999),(#52000,#52001),(#52002,#52003),(#52004,#52005),
(#52006,#52007),(#52008,#52009),(#52010,#52011),(#52012,#52013),(#52014,
#52015),(#52016,#52017),(#52018,#52019),(#52020,#52021),(#52022,#52023),
(#52024,#52025),(#52026,#52027),(#52028,#52029),(#52030,#52031),(#52032,
#52033),(#52034,#52035),(#52036,#52037),(#52038,#52039),(#52040,#52041),
(#52042,#52043),(#52044,#52045),(#52046,#52047),(#52048,#52049),(#52050,
#52051),(#52052,#52053),(#52054,#52055),(#52056,#52057)),.UNSPECIFIED.,
 .F.,.F.,.F.)
B_SPLINE_SURFACE_WITH_KNOTS((6,1,1,1,1,1,1,1,1,1,1,1,1,1,1,1,1,1,1,1,1,
1,1,1,1,1,1,1,1,1,1,1,1,1,1,1,1,1,1,1,1,1,1,1,1,1,1,1,1,1,1,1,1,1,1,1,1,
1,1,1,1,1,1,1,1,6),(2,2),(-1.,-0.984615384615383,-0.969230769230768,-0.953846153846152,
-0.938461538461537,-0.923076923076922,-0.907692307692306,-0.892307692307691,
-0.876923076923076,-0.86153846153846,-0.846153846153845,-0.83076923076923,
-0.815384615384614,-0.799999999999999,-0.784615384615384,-0.769230769230768,
-0.753846153846153,-0.738461538461538,-0.723076923076922,-0.707692307692307,
-0.692307692307692,-0.676923076923076,-0.661538461538461,-0.646153846153846,
-0.63076923076923,-0.615384615384615,-0.6,-0.584615384615384,-0.569230769230769,
-0.553846153846154,-0.538461538461538,-0.523076923076923,-0.507692307692308,
-0.492307692307692,-0.476923076923077,-0.461538461538462,-0.446153846153846,
-0.430769230769231,-0.415384615384615,-0.4,-0.384615384615385,-0.369230769230769,
-0.353846153846154,-0.338461538461538,-0.323076923076923,-0.307692307692308,
-0.292307692307692,-0.276923076923077,-0.261538461538462,-0.246153846153846,
-0.230769230769231,-0.215384615384615,-0.2,-0.184615384615385,-0.169230769230769,
-0.153846153846154,-0.138461538461538,-0.123076923076923,-0.107692307692308,
-0.0923076923076923,-0.0769230769230769,-0.0615384615384615,-0.0461538461538462,
-0.0307692307692308,-0.0153846153846154,0.),(-1.,1.),.UNSPECIFIED.)
GEOMETRIC_REPRESENTATION_ITEM()
RATIONAL_B_SPLINE_SURFACE(((1.,1.),(1.,1.),(1.,1.),(1.,1.),(1.,1.),(1.,
1.),(1.,1.),(1.,1.),(1.,1.),(1.,1.),(1.,1.),(1.,1.),(1.,1.),(1.,1.),(1.,
1.),(1.,1.),(1.,1.),(1.,1.),(1.,1.),(1.,1.),(1.,1.),(1.,1.),(1.,1.),(1.,
1.),(1.,1.),(1.,1.),(1.,1.),(1.,1.),(1.,1.),(1.,1.),(1.,1.),(1.,1.),(1.,
1.),(1.,1.),(1.,1.),(1.,1.),(1.,1.),(1.,1.),(1.,1.),(1.,1.),(1.,1.),(1.,
1.),(1.,1.),(1.,1.),(1.,1.),(1.,1.),(1.,1.),(1.,1.),(1.,1.),(1.,1.),(1.,
1.),(1.,1.),(1.,1.),(1.,1.),(1.,1.),(1.,1.),(1.,1.),(1.,1.),(1.,1.),(1.,
1.),(1.,1.),(1.,1.),(1.,1.),(1.,1.),(1.,1.),(1.,1.),(1.,1.),(1.,1.),(1.,
1.),(1.,1.)))
REPRESENTATION_ITEM('')
SURFACE()
);
#124=(
BOUNDED_SURFACE()
B_SPLINE_SURFACE(5,1,((#52130,#52131),(#52132,#52133),(#52134,#52135),(#52136,
#52137),(#52138,#52139),(#52140,#52141),(#52142,#52143),(#52144,#52145),
(#52146,#52147),(#52148,#52149),(#52150,#52151),(#52152,#52153),(#52154,
#52155),(#52156,#52157),(#52158,#52159),(#52160,#52161),(#52162,#52163),
(#52164,#52165),(#52166,#52167),(#52168,#52169),(#52170,#52171),(#52172,
#52173),(#52174,#52175),(#52176,#52177),(#52178,#52179),(#52180,#52181),
(#52182,#52183),(#52184,#52185),(#52186,#52187),(#52188,#52189),(#52190,
#52191),(#52192,#52193),(#52194,#52195),(#52196,#52197),(#52198,#52199),
(#52200,#52201),(#52202,#52203),(#52204,#52205),(#52206,#52207),(#52208,
#52209),(#52210,#52211),(#52212,#52213),(#52214,#52215),(#52216,#52217),
(#52218,#52219),(#52220,#52221),(#52222,#52223),(#52224,#52225),(#52226,
#52227),(#52228,#52229),(#52230,#52231),(#52232,#52233),(#52234,#52235),
(#52236,#52237),(#52238,#52239),(#52240,#52241),(#52242,#52243),(#52244,
#52245),(#52246,#52247),(#52248,#52249),(#52250,#52251),(#52252,#52253),
(#52254,#52255),(#52256,#52257),(#52258,#52259),(#52260,#52261),(#52262,
#52263),(#52264,#52265),(#52266,#52267),(#52268,#52269)),.UNSPECIFIED.,
 .F.,.F.,.F.)
B_SPLINE_SURFACE_WITH_KNOTS((6,1,1,1,1,1,1,1,1,1,1,1,1,1,1,1,1,1,1,1,1,
1,1,1,1,1,1,1,1,1,1,1,1,1,1,1,1,1,1,1,1,1,1,1,1,1,1,1,1,1,1,1,1,1,1,1,1,
1,1,1,1,1,1,1,1,6),(2,2),(-1.,-0.984615384615383,-0.969230769230768,-0.953846153846152,
-0.938461538461537,-0.923076923076922,-0.907692307692306,-0.892307692307691,
-0.876923076923076,-0.86153846153846,-0.846153846153845,-0.83076923076923,
-0.815384615384614,-0.799999999999999,-0.784615384615384,-0.769230769230768,
-0.753846153846153,-0.738461538461538,-0.723076923076922,-0.707692307692307,
-0.692307692307692,-0.676923076923076,-0.661538461538461,-0.646153846153846,
-0.63076923076923,-0.615384615384615,-0.6,-0.584615384615384,-0.569230769230769,
-0.553846153846154,-0.538461538461538,-0.523076923076923,-0.507692307692308,
-0.492307692307692,-0.476923076923077,-0.461538461538462,-0.446153846153846,
-0.430769230769231,-0.415384615384615,-0.4,-0.384615384615385,-0.369230769230769,
-0.353846153846154,-0.338461538461538,-0.323076923076923,-0.307692307692308,
-0.292307692307692,-0.276923076923077,-0.261538461538462,-0.246153846153846,
-0.230769230769231,-0.215384615384615,-0.2,-0.184615384615385,-0.169230769230769,
-0.153846153846154,-0.138461538461538,-0.123076923076923,-0.107692307692308,
-0.0923076923076923,-0.0769230769230769,-0.0615384615384615,-0.0461538461538462,
-0.0307692307692308,-0.0153846153846154,0.),(-1.,1.),.UNSPECIFIED.)
GEOMETRIC_REPRESENTATION_ITEM()
RATIONAL_B_SPLINE_SURFACE(((1.,1.),(1.,1.),(1.,1.),(1.,1.),(1.,1.),(1.,
1.),(1.,1.),(1.,1.),(1.,1.),(1.,1.),(1.,1.),(1.,1.),(1.,1.),(1.,1.),(1.,
1.),(1.,1.),(1.,1.),(1.,1.),(1.,1.),(1.,1.),(1.,1.),(1.,1.),(1.,1.),(1.,
1.),(1.,1.),(1.,1.),(1.,1.),(1.,1.),(1.,1.),(1.,1.),(1.,1.),(1.,1.),(1.,
1.),(1.,1.),(1.,1.),(1.,1.),(1.,1.),(1.,1.),(1.,1.),(1.,1.),(1.,1.),(1.,
1.),(1.,1.),(1.,1.),(1.,1.),(1.,1.),(1.,1.),(1.,1.),(1.,1.),(1.,1.),(1.,
1.),(1.,1.),(1.,1.),(1.,1.),(1.,1.),(1.,1.),(1.,1.),(1.,1.),(1.,1.),(1.,
1.),(1.,1.),(1.,1.),(1.,1.),(1.,1.),(1.,1.),(1.,1.),(1.,1.),(1.,1.),(1.,
1.),(1.,1.)))
REPRESENTATION_ITEM('')
SURFACE()
);
#125=(
BOUNDED_SURFACE()
B_SPLINE_SURFACE(5,1,((#52360,#52361),(#52362,#52363),(#52364,#52365),(#52366,
#52367),(#52368,#52369),(#52370,#52371),(#52372,#52373),(#52374,#52375),
(#52376,#52377),(#52378,#52379),(#52380,#52381),(#52382,#52383),(#52384,
#52385),(#52386,#52387),(#52388,#52389),(#52390,#52391),(#52392,#52393),
(#52394,#52395),(#52396,#52397),(#52398,#52399),(#52400,#52401),(#52402,
#52403),(#52404,#52405),(#52406,#52407),(#52408,#52409),(#52410,#52411),
(#52412,#52413),(#52414,#52415),(#52416,#52417),(#52418,#52419),(#52420,
#52421),(#52422,#52423),(#52424,#52425),(#52426,#52427),(#52428,#52429),
(#52430,#52431),(#52432,#52433),(#52434,#52435),(#52436,#52437),(#52438,
#52439),(#52440,#52441),(#52442,#52443),(#52444,#52445),(#52446,#52447),
(#52448,#52449),(#52450,#52451),(#52452,#52453),(#52454,#52455),(#52456,
#52457),(#52458,#52459),(#52460,#52461),(#52462,#52463),(#52464,#52465),
(#52466,#52467),(#52468,#52469),(#52470,#52471),(#52472,#52473),(#52474,
#52475),(#52476,#52477),(#52478,#52479),(#52480,#52481),(#52482,#52483),
(#52484,#52485),(#52486,#52487),(#52488,#52489),(#52490,#52491),(#52492,
#52493),(#52494,#52495),(#52496,#52497),(#52498,#52499)),.UNSPECIFIED.,
 .F.,.F.,.F.)
B_SPLINE_SURFACE_WITH_KNOTS((6,1,1,1,1,1,1,1,1,1,1,1,1,1,1,1,1,1,1,1,1,
1,1,1,1,1,1,1,1,1,1,1,1,1,1,1,1,1,1,1,1,1,1,1,1,1,1,1,1,1,1,1,1,1,1,1,1,
1,1,1,1,1,1,1,1,6),(2,2),(-1.,-0.984615384615383,-0.969230769230768,-0.953846153846152,
-0.938461538461537,-0.923076923076922,-0.907692307692306,-0.892307692307691,
-0.876923076923076,-0.86153846153846,-0.846153846153845,-0.83076923076923,
-0.815384615384614,-0.799999999999999,-0.784615384615384,-0.769230769230768,
-0.753846153846153,-0.738461538461538,-0.723076923076922,-0.707692307692307,
-0.692307692307692,-0.676923076923076,-0.661538461538461,-0.646153846153846,
-0.63076923076923,-0.615384615384615,-0.6,-0.584615384615384,-0.569230769230769,
-0.553846153846154,-0.538461538461538,-0.523076923076923,-0.507692307692308,
-0.492307692307692,-0.476923076923077,-0.461538461538462,-0.446153846153846,
-0.430769230769231,-0.415384615384615,-0.4,-0.384615384615385,-0.369230769230769,
-0.353846153846154,-0.338461538461538,-0.323076923076923,-0.307692307692308,
-0.292307692307692,-0.276923076923077,-0.261538461538462,-0.246153846153846,
-0.230769230769231,-0.215384615384615,-0.2,-0.184615384615385,-0.169230769230769,
-0.153846153846154,-0.138461538461538,-0.123076923076923,-0.107692307692308,
-0.0923076923076923,-0.0769230769230769,-0.0615384615384615,-0.0461538461538462,
-0.0307692307692308,-0.0153846153846154,0.),(-1.,1.),.UNSPECIFIED.)
GEOMETRIC_REPRESENTATION_ITEM()
RATIONAL_B_SPLINE_SURFACE(((1.,1.),(1.,1.),(1.,1.),(1.,1.),(1.,1.),(1.,
1.),(1.,1.),(1.,1.),(1.,1.),(1.,1.),(1.,1.),(1.,1.),(1.,1.),(1.,1.),(1.,
1.),(1.,1.),(1.,1.),(1.,1.),(1.,1.),(1.,1.),(1.,1.),(1.,1.),(1.,1.),(1.,
1.),(1.,1.),(1.,1.),(1.,1.),(1.,1.),(1.,1.),(1.,1.),(1.,1.),(1.,1.),(1.,
1.),(1.,1.),(1.,1.),(1.,1.),(1.,1.),(1.,1.),(1.,1.),(1.,1.),(1.,1.),(1.,
1.),(1.,1.),(1.,1.),(1.,1.),(1.,1.),(1.,1.),(1.,1.),(1.,1.),(1.,1.),(1.,
1.),(1.,1.),(1.,1.),(1.,1.),(1.,1.),(1.,1.),(1.,1.),(1.,1.),(1.,1.),(1.,
1.),(1.,1.),(1.,1.),(1.,1.),(1.,1.),(1.,1.),(1.,1.),(1.,1.),(1.,1.),(1.,
1.),(1.,1.)))
REPRESENTATION_ITEM('')
SURFACE()
);
#126=(
BOUNDED_SURFACE()
B_SPLINE_SURFACE(5,1,((#52572,#52573),(#52574,#52575),(#52576,#52577),(#52578,
#52579),(#52580,#52581),(#52582,#52583),(#52584,#52585),(#52586,#52587),
(#52588,#52589),(#52590,#52591),(#52592,#52593),(#52594,#52595),(#52596,
#52597),(#52598,#52599),(#52600,#52601),(#52602,#52603),(#52604,#52605),
(#52606,#52607),(#52608,#52609),(#52610,#52611),(#52612,#52613),(#52614,
#52615),(#52616,#52617),(#52618,#52619),(#52620,#52621),(#52622,#52623),
(#52624,#52625),(#52626,#52627),(#52628,#52629),(#52630,#52631),(#52632,
#52633),(#52634,#52635),(#52636,#52637),(#52638,#52639),(#52640,#52641),
(#52642,#52643),(#52644,#52645),(#52646,#52647),(#52648,#52649),(#52650,
#52651),(#52652,#52653),(#52654,#52655),(#52656,#52657),(#52658,#52659),
(#52660,#52661),(#52662,#52663),(#52664,#52665),(#52666,#52667),(#52668,
#52669),(#52670,#52671),(#52672,#52673),(#52674,#52675),(#52676,#52677),
(#52678,#52679),(#52680,#52681),(#52682,#52683),(#52684,#52685),(#52686,
#52687),(#52688,#52689),(#52690,#52691),(#52692,#52693),(#52694,#52695),
(#52696,#52697),(#52698,#52699),(#52700,#52701),(#52702,#52703),(#52704,
#52705),(#52706,#52707),(#52708,#52709),(#52710,#52711)),.UNSPECIFIED.,
 .F.,.F.,.F.)
B_SPLINE_SURFACE_WITH_KNOTS((6,1,1,1,1,1,1,1,1,1,1,1,1,1,1,1,1,1,1,1,1,
1,1,1,1,1,1,1,1,1,1,1,1,1,1,1,1,1,1,1,1,1,1,1,1,1,1,1,1,1,1,1,1,1,1,1,1,
1,1,1,1,1,1,1,1,6),(2,2),(-1.,-0.984615384615383,-0.969230769230768,-0.953846153846152,
-0.938461538461537,-0.923076923076922,-0.907692307692306,-0.892307692307691,
-0.876923076923076,-0.86153846153846,-0.846153846153845,-0.83076923076923,
-0.815384615384614,-0.799999999999999,-0.784615384615384,-0.769230769230768,
-0.753846153846153,-0.738461538461538,-0.723076923076922,-0.707692307692307,
-0.692307692307692,-0.676923076923076,-0.661538461538461,-0.646153846153846,
-0.63076923076923,-0.615384615384615,-0.6,-0.584615384615384,-0.569230769230769,
-0.553846153846154,-0.538461538461538,-0.523076923076923,-0.507692307692308,
-0.492307692307692,-0.476923076923077,-0.461538461538462,-0.446153846153846,
-0.430769230769231,-0.415384615384615,-0.4,-0.384615384615385,-0.369230769230769,
-0.353846153846154,-0.338461538461538,-0.323076923076923,-0.307692307692308,
-0.292307692307692,-0.276923076923077,-0.261538461538462,-0.246153846153846,
-0.230769230769231,-0.215384615384615,-0.2,-0.184615384615385,-0.169230769230769,
-0.153846153846154,-0.138461538461538,-0.123076923076923,-0.107692307692308,
-0.0923076923076923,-0.0769230769230769,-0.0615384615384615,-0.0461538461538462,
-0.0307692307692308,-0.0153846153846154,0.),(-1.,1.),.UNSPECIFIED.)
GEOMETRIC_REPRESENTATION_ITEM()
RATIONAL_B_SPLINE_SURFACE(((1.,1.),(1.,1.),(1.,1.),(1.,1.),(1.,1.),(1.,
1.),(1.,1.),(1.,1.),(1.,1.),(1.,1.),(1.,1.),(1.,1.),(1.,1.),(1.,1.),(1.,
1.),(1.,1.),(1.,1.),(1.,1.),(1.,1.),(1.,1.),(1.,1.),(1.,1.),(1.,1.),(1.,
1.),(1.,1.),(1.,1.),(1.,1.),(1.,1.),(1.,1.),(1.,1.),(1.,1.),(1.,1.),(1.,
1.),(1.,1.),(1.,1.),(1.,1.),(1.,1.),(1.,1.),(1.,1.),(1.,1.),(1.,1.),(1.,
1.),(1.,1.),(1.,1.),(1.,1.),(1.,1.),(1.,1.),(1.,1.),(1.,1.),(1.,1.),(1.,
1.),(1.,1.),(1.,1.),(1.,1.),(1.,1.),(1.,1.),(1.,1.),(1.,1.),(1.,1.),(1.,
1.),(1.,1.),(1.,1.),(1.,1.),(1.,1.),(1.,1.),(1.,1.),(1.,1.),(1.,1.),(1.,
1.),(1.,1.)))
REPRESENTATION_ITEM('')
SURFACE()
);
#127=(
BOUNDED_SURFACE()
B_SPLINE_SURFACE(5,1,((#52802,#52803),(#52804,#52805),(#52806,#52807),(#52808,
#52809),(#52810,#52811),(#52812,#52813),(#52814,#52815),(#52816,#52817),
(#52818,#52819),(#52820,#52821),(#52822,#52823),(#52824,#52825),(#52826,
#52827),(#52828,#52829),(#52830,#52831),(#52832,#52833),(#52834,#52835),
(#52836,#52837),(#52838,#52839),(#52840,#52841),(#52842,#52843),(#52844,
#52845),(#52846,#52847),(#52848,#52849),(#52850,#52851),(#52852,#52853),
(#52854,#52855),(#52856,#52857),(#52858,#52859),(#52860,#52861),(#52862,
#52863),(#52864,#52865),(#52866,#52867),(#52868,#52869),(#52870,#52871),
(#52872,#52873),(#52874,#52875),(#52876,#52877),(#52878,#52879),(#52880,
#52881),(#52882,#52883),(#52884,#52885),(#52886,#52887),(#52888,#52889),
(#52890,#52891),(#52892,#52893),(#52894,#52895),(#52896,#52897),(#52898,
#52899),(#52900,#52901),(#52902,#52903),(#52904,#52905),(#52906,#52907),
(#52908,#52909),(#52910,#52911),(#52912,#52913),(#52914,#52915),(#52916,
#52917),(#52918,#52919),(#52920,#52921),(#52922,#52923),(#52924,#52925),
(#52926,#52927),(#52928,#52929),(#52930,#52931),(#52932,#52933),(#52934,
#52935),(#52936,#52937),(#52938,#52939),(#52940,#52941)),.UNSPECIFIED.,
 .F.,.F.,.F.)
B_SPLINE_SURFACE_WITH_KNOTS((6,1,1,1,1,1,1,1,1,1,1,1,1,1,1,1,1,1,1,1,1,
1,1,1,1,1,1,1,1,1,1,1,1,1,1,1,1,1,1,1,1,1,1,1,1,1,1,1,1,1,1,1,1,1,1,1,1,
1,1,1,1,1,1,1,1,6),(2,2),(-1.,-0.984615384615383,-0.969230769230768,-0.953846153846152,
-0.938461538461537,-0.923076923076922,-0.907692307692306,-0.892307692307691,
-0.876923076923076,-0.86153846153846,-0.846153846153845,-0.83076923076923,
-0.815384615384614,-0.799999999999999,-0.784615384615384,-0.769230769230768,
-0.753846153846153,-0.738461538461538,-0.723076923076922,-0.707692307692307,
-0.692307692307692,-0.676923076923076,-0.661538461538461,-0.646153846153846,
-0.63076923076923,-0.615384615384615,-0.6,-0.584615384615384,-0.569230769230769,
-0.553846153846154,-0.538461538461538,-0.523076923076923,-0.507692307692308,
-0.492307692307692,-0.476923076923077,-0.461538461538462,-0.446153846153846,
-0.430769230769231,-0.415384615384615,-0.4,-0.384615384615385,-0.369230769230769,
-0.353846153846154,-0.338461538461538,-0.323076923076923,-0.307692307692308,
-0.292307692307692,-0.276923076923077,-0.261538461538462,-0.246153846153846,
-0.230769230769231,-0.215384615384615,-0.2,-0.184615384615385,-0.169230769230769,
-0.153846153846154,-0.138461538461538,-0.123076923076923,-0.107692307692308,
-0.0923076923076923,-0.0769230769230769,-0.0615384615384615,-0.0461538461538462,
-0.0307692307692308,-0.0153846153846154,0.),(-1.,1.),.UNSPECIFIED.)
GEOMETRIC_REPRESENTATION_ITEM()
RATIONAL_B_SPLINE_SURFACE(((1.,1.),(1.,1.),(1.,1.),(1.,1.),(1.,1.),(1.,
1.),(1.,1.),(1.,1.),(1.,1.),(1.,1.),(1.,1.),(1.,1.),(1.,1.),(1.,1.),(1.,
1.),(1.,1.),(1.,1.),(1.,1.),(1.,1.),(1.,1.),(1.,1.),(1.,1.),(1.,1.),(1.,
1.),(1.,1.),(1.,1.),(1.,1.),(1.,1.),(1.,1.),(1.,1.),(1.,1.),(1.,1.),(1.,
1.),(1.,1.),(1.,1.),(1.,1.),(1.,1.),(1.,1.),(1.,1.),(1.,1.),(1.,1.),(1.,
1.),(1.,1.),(1.,1.),(1.,1.),(1.,1.),(1.,1.),(1.,1.),(1.,1.),(1.,1.),(1.,
1.),(1.,1.),(1.,1.),(1.,1.),(1.,1.),(1.,1.),(1.,1.),(1.,1.),(1.,1.),(1.,
1.),(1.,1.),(1.,1.),(1.,1.),(1.,1.),(1.,1.),(1.,1.),(1.,1.),(1.,1.),(1.,
1.),(1.,1.)))
REPRESENTATION_ITEM('')
SURFACE()
);
#128=(
BOUNDED_SURFACE()
B_SPLINE_SURFACE(5,1,((#53018,#53019),(#53020,#53021),(#53022,#53023),(#53024,
#53025),(#53026,#53027),(#53028,#53029),(#53030,#53031),(#53032,#53033),
(#53034,#53035),(#53036,#53037),(#53038,#53039),(#53040,#53041),(#53042,
#53043),(#53044,#53045),(#53046,#53047),(#53048,#53049),(#53050,#53051),
(#53052,#53053),(#53054,#53055),(#53056,#53057),(#53058,#53059),(#53060,
#53061),(#53062,#53063),(#53064,#53065),(#53066,#53067),(#53068,#53069),
(#53070,#53071),(#53072,#53073),(#53074,#53075),(#53076,#53077),(#53078,
#53079),(#53080,#53081),(#53082,#53083),(#53084,#53085),(#53086,#53087),
(#53088,#53089),(#53090,#53091),(#53092,#53093),(#53094,#53095),(#53096,
#53097),(#53098,#53099),(#53100,#53101),(#53102,#53103),(#53104,#53105),
(#53106,#53107),(#53108,#53109),(#53110,#53111),(#53112,#53113),(#53114,
#53115),(#53116,#53117),(#53118,#53119),(#53120,#53121),(#53122,#53123),
(#53124,#53125),(#53126,#53127),(#53128,#53129),(#53130,#53131),(#53132,
#53133),(#53134,#53135),(#53136,#53137),(#53138,#53139),(#53140,#53141),
(#53142,#53143),(#53144,#53145),(#53146,#53147),(#53148,#53149),(#53150,
#53151),(#53152,#53153),(#53154,#53155),(#53156,#53157)),.UNSPECIFIED.,
 .F.,.F.,.F.)
B_SPLINE_SURFACE_WITH_KNOTS((6,1,1,1,1,1,1,1,1,1,1,1,1,1,1,1,1,1,1,1,1,
1,1,1,1,1,1,1,1,1,1,1,1,1,1,1,1,1,1,1,1,1,1,1,1,1,1,1,1,1,1,1,1,1,1,1,1,
1,1,1,1,1,1,1,1,6),(2,2),(-1.,-0.984615384615383,-0.969230769230768,-0.953846153846152,
-0.938461538461537,-0.923076923076922,-0.907692307692306,-0.892307692307691,
-0.876923076923076,-0.86153846153846,-0.846153846153845,-0.83076923076923,
-0.815384615384614,-0.799999999999999,-0.784615384615384,-0.769230769230768,
-0.753846153846153,-0.738461538461538,-0.723076923076922,-0.707692307692307,
-0.692307692307692,-0.676923076923076,-0.661538461538461,-0.646153846153846,
-0.63076923076923,-0.615384615384615,-0.6,-0.584615384615384,-0.569230769230769,
-0.553846153846154,-0.538461538461538,-0.523076923076923,-0.507692307692308,
-0.492307692307692,-0.476923076923077,-0.461538461538462,-0.446153846153846,
-0.430769230769231,-0.415384615384615,-0.4,-0.384615384615385,-0.369230769230769,
-0.353846153846154,-0.338461538461538,-0.323076923076923,-0.307692307692308,
-0.292307692307692,-0.276923076923077,-0.261538461538462,-0.246153846153846,
-0.230769230769231,-0.215384615384615,-0.2,-0.184615384615385,-0.169230769230769,
-0.153846153846154,-0.138461538461538,-0.123076923076923,-0.107692307692308,
-0.0923076923076923,-0.0769230769230769,-0.0615384615384615,-0.0461538461538462,
-0.0307692307692308,-0.0153846153846154,0.),(-1.,1.),.UNSPECIFIED.)
GEOMETRIC_REPRESENTATION_ITEM()
RATIONAL_B_SPLINE_SURFACE(((1.,1.),(1.,1.),(1.,1.),(1.,1.),(1.,1.),(1.,
1.),(1.,1.),(1.,1.),(1.,1.),(1.,1.),(1.,1.),(1.,1.),(1.,1.),(1.,1.),(1.,
1.),(1.,1.),(1.,1.),(1.,1.),(1.,1.),(1.,1.),(1.,1.),(1.,1.),(1.,1.),(1.,
1.),(1.,1.),(1.,1.),(1.,1.),(1.,1.),(1.,1.),(1.,1.),(1.,1.),(1.,1.),(1.,
1.),(1.,1.),(1.,1.),(1.,1.),(1.,1.),(1.,1.),(1.,1.),(1.,1.),(1.,1.),(1.,
1.),(1.,1.),(1.,1.),(1.,1.),(1.,1.),(1.,1.),(1.,1.),(1.,1.),(1.,1.),(1.,
1.),(1.,1.),(1.,1.),(1.,1.),(1.,1.),(1.,1.),(1.,1.),(1.,1.),(1.,1.),(1.,
1.),(1.,1.),(1.,1.),(1.,1.),(1.,1.),(1.,1.),(1.,1.),(1.,1.),(1.,1.),(1.,
1.),(1.,1.)))
REPRESENTATION_ITEM('')
SURFACE()
);
#129=(
BOUNDED_SURFACE()
B_SPLINE_SURFACE(5,1,((#53244,#53245),(#53246,#53247),(#53248,#53249),(#53250,
#53251),(#53252,#53253),(#53254,#53255),(#53256,#53257),(#53258,#53259),
(#53260,#53261),(#53262,#53263),(#53264,#53265),(#53266,#53267),(#53268,
#53269),(#53270,#53271),(#53272,#53273),(#53274,#53275),(#53276,#53277),
(#53278,#53279),(#53280,#53281),(#53282,#53283),(#53284,#53285),(#53286,
#53287),(#53288,#53289),(#53290,#53291),(#53292,#53293),(#53294,#53295),
(#53296,#53297),(#53298,#53299),(#53300,#53301),(#53302,#53303),(#53304,
#53305),(#53306,#53307),(#53308,#53309),(#53310,#53311),(#53312,#53313),
(#53314,#53315),(#53316,#53317),(#53318,#53319),(#53320,#53321),(#53322,
#53323),(#53324,#53325),(#53326,#53327),(#53328,#53329),(#53330,#53331),
(#53332,#53333),(#53334,#53335),(#53336,#53337),(#53338,#53339),(#53340,
#53341),(#53342,#53343),(#53344,#53345),(#53346,#53347),(#53348,#53349),
(#53350,#53351),(#53352,#53353),(#53354,#53355),(#53356,#53357),(#53358,
#53359),(#53360,#53361),(#53362,#53363),(#53364,#53365),(#53366,#53367),
(#53368,#53369),(#53370,#53371),(#53372,#53373),(#53374,#53375),(#53376,
#53377),(#53378,#53379),(#53380,#53381),(#53382,#53383)),.UNSPECIFIED.,
 .F.,.F.,.F.)
B_SPLINE_SURFACE_WITH_KNOTS((6,1,1,1,1,1,1,1,1,1,1,1,1,1,1,1,1,1,1,1,1,
1,1,1,1,1,1,1,1,1,1,1,1,1,1,1,1,1,1,1,1,1,1,1,1,1,1,1,1,1,1,1,1,1,1,1,1,
1,1,1,1,1,1,1,1,6),(2,2),(-1.,-0.984615384615383,-0.969230769230768,-0.953846153846152,
-0.938461538461537,-0.923076923076922,-0.907692307692306,-0.892307692307691,
-0.876923076923076,-0.86153846153846,-0.846153846153845,-0.83076923076923,
-0.815384615384614,-0.799999999999999,-0.784615384615384,-0.769230769230768,
-0.753846153846153,-0.738461538461538,-0.723076923076922,-0.707692307692307,
-0.692307692307692,-0.676923076923076,-0.661538461538461,-0.646153846153846,
-0.63076923076923,-0.615384615384615,-0.6,-0.584615384615384,-0.569230769230769,
-0.553846153846154,-0.538461538461538,-0.523076923076923,-0.507692307692308,
-0.492307692307692,-0.476923076923077,-0.461538461538462,-0.446153846153846,
-0.430769230769231,-0.415384615384615,-0.4,-0.384615384615385,-0.369230769230769,
-0.353846153846154,-0.338461538461538,-0.323076923076923,-0.307692307692308,
-0.292307692307692,-0.276923076923077,-0.261538461538462,-0.246153846153846,
-0.230769230769231,-0.215384615384615,-0.2,-0.184615384615385,-0.169230769230769,
-0.153846153846154,-0.138461538461538,-0.123076923076923,-0.107692307692308,
-0.0923076923076923,-0.0769230769230769,-0.0615384615384615,-0.0461538461538462,
-0.0307692307692308,-0.0153846153846154,0.),(-1.,1.),.UNSPECIFIED.)
GEOMETRIC_REPRESENTATION_ITEM()
RATIONAL_B_SPLINE_SURFACE(((1.,1.),(1.,1.),(1.,1.),(1.,1.),(1.,1.),(1.,
1.),(1.,1.),(1.,1.),(1.,1.),(1.,1.),(1.,1.),(1.,1.),(1.,1.),(1.,1.),(1.,
1.),(1.,1.),(1.,1.),(1.,1.),(1.,1.),(1.,1.),(1.,1.),(1.,1.),(1.,1.),(1.,
1.),(1.,1.),(1.,1.),(1.,1.),(1.,1.),(1.,1.),(1.,1.),(1.,1.),(1.,1.),(1.,
1.),(1.,1.),(1.,1.),(1.,1.),(1.,1.),(1.,1.),(1.,1.),(1.,1.),(1.,1.),(1.,
1.),(1.,1.),(1.,1.),(1.,1.),(1.,1.),(1.,1.),(1.,1.),(1.,1.),(1.,1.),(1.,
1.),(1.,1.),(1.,1.),(1.,1.),(1.,1.),(1.,1.),(1.,1.),(1.,1.),(1.,1.),(1.,
1.),(1.,1.),(1.,1.),(1.,1.),(1.,1.),(1.,1.),(1.,1.),(1.,1.),(1.,1.),(1.,
1.),(1.,1.)))
REPRESENTATION_ITEM('')
SURFACE()
);
#130=(
BOUNDED_SURFACE()
B_SPLINE_SURFACE(5,1,((#53463,#53464),(#53465,#53466),(#53467,#53468),(#53469,
#53470),(#53471,#53472),(#53473,#53474),(#53475,#53476),(#53477,#53478),
(#53479,#53480),(#53481,#53482),(#53483,#53484),(#53485,#53486),(#53487,
#53488),(#53489,#53490),(#53491,#53492),(#53493,#53494),(#53495,#53496),
(#53497,#53498),(#53499,#53500),(#53501,#53502),(#53503,#53504),(#53505,
#53506),(#53507,#53508),(#53509,#53510),(#53511,#53512),(#53513,#53514),
(#53515,#53516),(#53517,#53518),(#53519,#53520),(#53521,#53522),(#53523,
#53524),(#53525,#53526),(#53527,#53528),(#53529,#53530),(#53531,#53532),
(#53533,#53534),(#53535,#53536),(#53537,#53538),(#53539,#53540),(#53541,
#53542),(#53543,#53544),(#53545,#53546),(#53547,#53548),(#53549,#53550),
(#53551,#53552),(#53553,#53554),(#53555,#53556),(#53557,#53558),(#53559,
#53560),(#53561,#53562),(#53563,#53564),(#53565,#53566),(#53567,#53568),
(#53569,#53570),(#53571,#53572),(#53573,#53574),(#53575,#53576),(#53577,
#53578),(#53579,#53580),(#53581,#53582),(#53583,#53584),(#53585,#53586),
(#53587,#53588),(#53589,#53590),(#53591,#53592),(#53593,#53594),(#53595,
#53596),(#53597,#53598),(#53599,#53600),(#53601,#53602)),.UNSPECIFIED.,
 .F.,.F.,.F.)
B_SPLINE_SURFACE_WITH_KNOTS((6,1,1,1,1,1,1,1,1,1,1,1,1,1,1,1,1,1,1,1,1,
1,1,1,1,1,1,1,1,1,1,1,1,1,1,1,1,1,1,1,1,1,1,1,1,1,1,1,1,1,1,1,1,1,1,1,1,
1,1,1,1,1,1,1,1,6),(2,2),(-1.,-0.984615384615383,-0.969230769230768,-0.953846153846152,
-0.938461538461537,-0.923076923076922,-0.907692307692306,-0.892307692307691,
-0.876923076923076,-0.86153846153846,-0.846153846153845,-0.83076923076923,
-0.815384615384614,-0.799999999999999,-0.784615384615384,-0.769230769230768,
-0.753846153846153,-0.738461538461538,-0.723076923076922,-0.707692307692307,
-0.692307692307692,-0.676923076923076,-0.661538461538461,-0.646153846153846,
-0.63076923076923,-0.615384615384615,-0.6,-0.584615384615384,-0.569230769230769,
-0.553846153846154,-0.538461538461538,-0.523076923076923,-0.507692307692308,
-0.492307692307692,-0.476923076923077,-0.461538461538462,-0.446153846153846,
-0.430769230769231,-0.415384615384615,-0.4,-0.384615384615385,-0.369230769230769,
-0.353846153846154,-0.338461538461538,-0.323076923076923,-0.307692307692308,
-0.292307692307692,-0.276923076923077,-0.261538461538462,-0.246153846153846,
-0.230769230769231,-0.215384615384615,-0.2,-0.184615384615385,-0.169230769230769,
-0.153846153846154,-0.138461538461538,-0.123076923076923,-0.107692307692308,
-0.0923076923076923,-0.0769230769230769,-0.0615384615384615,-0.0461538461538462,
-0.0307692307692308,-0.0153846153846154,0.),(-1.,1.),.UNSPECIFIED.)
GEOMETRIC_REPRESENTATION_ITEM()
RATIONAL_B_SPLINE_SURFACE(((1.,1.),(1.,1.),(1.,1.),(1.,1.),(1.,1.),(1.,
1.),(1.,1.),(1.,1.),(1.,1.),(1.,1.),(1.,1.),(1.,1.),(1.,1.),(1.,1.),(1.,
1.),(1.,1.),(1.,1.),(1.,1.),(1.,1.),(1.,1.),(1.,1.),(1.,1.),(1.,1.),(1.,
1.),(1.,1.),(1.,1.),(1.,1.),(1.,1.),(1.,1.),(1.,1.),(1.,1.),(1.,1.),(1.,
1.),(1.,1.),(1.,1.),(1.,1.),(1.,1.),(1.,1.),(1.,1.),(1.,1.),(1.,1.),(1.,
1.),(1.,1.),(1.,1.),(1.,1.),(1.,1.),(1.,1.),(1.,1.),(1.,1.),(1.,1.),(1.,
1.),(1.,1.),(1.,1.),(1.,1.),(1.,1.),(1.,1.),(1.,1.),(1.,1.),(1.,1.),(1.,
1.),(1.,1.),(1.,1.),(1.,1.),(1.,1.),(1.,1.),(1.,1.),(1.,1.),(1.,1.),(1.,
1.),(1.,1.)))
REPRESENTATION_ITEM('')
SURFACE()
);
#211=(
BOUNDED_CURVE()
B_SPLINE_CURVE(5,(#30153,#30154,#30155,#30156,#30157,#30158,#30159,#30160,
#30161,#30162,#30163,#30164,#30165,#30166,#30167,#30168,#30169,#30170,#30171,
#30172,#30173,#30174,#30175,#30176,#30177,#30178,#30179,#30180,#30181,#30182,
#30183,#30184,#30185,#30186,#30187,#30188,#30189,#30190,#30191,#30192,#30193,
#30194,#30195,#30196,#30197,#30198,#30199,#30200,#30201,#30202,#30203,#30204,
#30205,#30206,#30207,#30208,#30209,#30210,#30211,#30212,#30213,#30214,#30215,
#30216,#30217,#30218,#30219,#30220,#30221,#30222),.UNSPECIFIED.,.F.,.F.)
B_SPLINE_CURVE_WITH_KNOTS((6,1,1,1,1,1,1,1,1,1,1,1,1,1,1,1,1,1,1,1,1,1,
1,1,1,1,1,1,1,1,1,1,1,1,1,1,1,1,1,1,1,1,1,1,1,1,1,1,1,1,1,1,1,1,1,1,1,1,
1,1,1,1,1,1,1,6),(0.00577184337450058,0.0153846153846154,0.0307692307692308,
0.0461538461538462,0.0615384615384615,0.0769230769230769,0.0923076923076923,
0.107692307692308,0.123076923076923,0.138461538461538,0.153846153846154,
0.169230769230769,0.184615384615385,0.2,0.215384615384615,0.230769230769231,
0.246153846153846,0.261538461538462,0.276923076923077,0.292307692307692,
0.307692307692308,0.323076923076923,0.338461538461538,0.353846153846154,
0.369230769230769,0.384615384615385,0.4,0.415384615384615,0.430769230769231,
0.446153846153846,0.461538461538462,0.476923076923077,0.492307692307692,
0.507692307692308,0.523076923076923,0.538461538461538,0.553846153846154,
0.569230769230769,0.584615384615384,0.6,0.615384615384615,0.63076923076923,
0.646153846153846,0.661538461538461,0.676923076923076,0.692307692307692,
0.707692307692307,0.723076923076922,0.738461538461538,0.753846153846153,
0.769230769230768,0.784615384615384,0.799999999999999,0.815384615384614,
0.83076923076923,0.846153846153845,0.86153846153846,0.876923076923076,0.892307692307691,
0.907692307692306,0.923076923076922,0.938461538461537,0.953846153846152,
0.969230769230768,0.984615384615383,1.),.UNSPECIFIED.)
CURVE()
GEOMETRIC_REPRESENTATION_ITEM()
RATIONAL_B_SPLINE_CURVE((1.,1.,1.,1.,1.,1.,1.,1.,1.,1.,1.,1.,1.,1.,1.,1.,
1.,1.,1.,1.,1.,1.,1.,1.,1.,1.,1.,1.,1.,1.,1.,1.,1.,1.,1.,1.,1.,1.,1.,1.,
1.,1.,1.,1.,1.,1.,1.,1.,1.,1.,1.,1.,1.,1.,1.,1.,1.,1.,1.,1.,1.,1.,1.,1.,
1.,1.,1.,1.,1.,1.))
REPRESENTATION_ITEM('')
);
#212=(
BOUNDED_CURVE()
B_SPLINE_CURVE(5,(#30226,#30227,#30228,#30229,#30230,#30231,#30232,#30233,
#30234,#30235,#30236,#30237,#30238,#30239,#30240,#30241,#30242,#30243,#30244,
#30245,#30246,#30247,#30248,#30249,#30250,#30251,#30252,#30253,#30254,#30255,
#30256,#30257,#30258,#30259,#30260,#30261,#30262,#30263,#30264,#30265,#30266,
#30267,#30268,#30269,#30270,#30271,#30272,#30273,#30274,#30275,#30276,#30277,
#30278,#30279,#30280,#30281,#30282,#30283,#30284,#30285,#30286,#30287,#30288,
#30289,#30290,#30291,#30292,#30293,#30294,#30295),.UNSPECIFIED.,.F.,.F.)
B_SPLINE_CURVE_WITH_KNOTS((6,1,1,1,1,1,1,1,1,1,1,1,1,1,1,1,1,1,1,1,1,1,
1,1,1,1,1,1,1,1,1,1,1,1,1,1,1,1,1,1,1,1,1,1,1,1,1,1,1,1,1,1,1,1,1,1,1,1,
1,1,1,1,1,1,1,6),(0.,0.0153846153846154,0.0307692307692308,0.0461538461538462,
0.0615384615384615,0.0769230769230769,0.0923076923076923,0.107692307692308,
0.123076923076923,0.138461538461538,0.153846153846154,0.169230769230769,
0.184615384615385,0.2,0.215384615384615,0.230769230769231,0.246153846153846,
0.261538461538462,0.276923076923077,0.292307692307692,0.307692307692308,
0.323076923076923,0.338461538461538,0.353846153846154,0.369230769230769,
0.384615384615385,0.4,0.415384615384615,0.430769230769231,0.446153846153846,
0.461538461538462,0.476923076923077,0.492307692307692,0.507692307692308,
0.523076923076923,0.538461538461538,0.553846153846154,0.569230769230769,
0.584615384615384,0.6,0.615384615384615,0.63076923076923,0.646153846153846,
0.661538461538461,0.676923076923076,0.692307692307692,0.707692307692307,
0.723076923076922,0.738461538461538,0.753846153846153,0.769230769230768,
0.784615384615384,0.799999999999999,0.815384615384614,0.83076923076923,
0.846153846153845,0.86153846153846,0.876923076923076,0.892307692307691,
0.907692307692306,0.923076923076922,0.938461538461537,0.953846153846152,
0.969230769230768,0.984615384615383,0.994228156739708),.UNSPECIFIED.)
CURVE()
GEOMETRIC_REPRESENTATION_ITEM()
RATIONAL_B_SPLINE_CURVE((1.,1.,1.,1.,1.,1.,1.,1.,1.,1.,1.,1.,1.,1.,1.,1.,
1.,1.,1.,1.,1.,1.,1.,1.,1.,1.,1.,1.,1.,1.,1.,1.,1.,1.,1.,1.,1.,1.,1.,1.,
1.,1.,1.,1.,1.,1.,1.,1.,1.,1.,1.,1.,1.,1.,1.,1.,1.,1.,1.,1.,1.,1.,1.,1.,
1.,1.,1.,1.,1.,1.))
REPRESENTATION_ITEM('')
);
#213=(
BOUNDED_CURVE()
B_SPLINE_CURVE(5,(#30299,#30300,#30301,#30302,#30303,#30304,#30305,#30306,
#30307,#30308,#30309,#30310,#30311,#30312,#30313,#30314,#30315,#30316,#30317,
#30318,#30319,#30320,#30321,#30322,#30323,#30324,#30325,#30326,#30327,#30328,
#30329,#30330,#30331,#30332,#30333,#30334,#30335,#30336,#30337,#30338,#30339,
#30340,#30341,#30342,#30343,#30344,#30345,#30346,#30347,#30348,#30349,#30350,
#30351,#30352,#30353,#30354,#30355,#30356,#30357,#30358,#30359,#30360,#30361,
#30362,#30363,#30364,#30365,#30366,#30367,#30368),.UNSPECIFIED.,.F.,.F.)
B_SPLINE_CURVE_WITH_KNOTS((6,1,1,1,1,1,1,1,1,1,1,1,1,1,1,1,1,1,1,1,1,1,
1,1,1,1,1,1,1,1,1,1,1,1,1,1,1,1,1,1,1,1,1,1,1,1,1,1,1,1,1,1,1,1,1,1,1,1,
1,1,1,1,1,1,1,6),(0.0057718433745091,0.0153846153846154,0.0307692307692308,
0.0461538461538462,0.0615384615384615,0.0769230769230769,0.0923076923076923,
0.107692307692308,0.123076923076923,0.138461538461538,0.153846153846154,
0.169230769230769,0.184615384615385,0.2,0.215384615384615,0.230769230769231,
0.246153846153846,0.261538461538462,0.276923076923077,0.292307692307692,
0.307692307692308,0.323076923076923,0.338461538461538,0.353846153846154,
0.369230769230769,0.384615384615385,0.4,0.415384615384615,0.430769230769231,
0.446153846153846,0.461538461538462,0.476923076923077,0.492307692307692,
0.507692307692308,0.523076923076923,0.538461538461538,0.553846153846154,
0.569230769230769,0.584615384615384,0.6,0.615384615384615,0.63076923076923,
0.646153846153846,0.661538461538461,0.676923076923076,0.692307692307692,
0.707692307692307,0.723076923076922,0.738461538461538,0.753846153846153,
0.769230769230768,0.784615384615384,0.799999999999999,0.815384615384614,
0.83076923076923,0.846153846153845,0.86153846153846,0.876923076923076,0.892307692307691,
0.907692307692306,0.923076923076922,0.938461538461537,0.953846153846152,
0.969230769230768,0.984615384615383,1.),.UNSPECIFIED.)
CURVE()
GEOMETRIC_REPRESENTATION_ITEM()
RATIONAL_B_SPLINE_CURVE((1.,1.,1.,1.,1.,1.,1.,1.,1.,1.,1.,1.,1.,1.,1.,1.,
1.,1.,1.,1.,1.,1.,1.,1.,1.,1.,1.,1.,1.,1.,1.,1.,1.,1.,1.,1.,1.,1.,1.,1.,
1.,1.,1.,1.,1.,1.,1.,1.,1.,1.,1.,1.,1.,1.,1.,1.,1.,1.,1.,1.,1.,1.,1.,1.,
1.,1.,1.,1.,1.,1.))
REPRESENTATION_ITEM('')
);
#214=(
BOUNDED_CURVE()
B_SPLINE_CURVE(5,(#30372,#30373,#30374,#30375,#30376,#30377,#30378,#30379,
#30380,#30381,#30382,#30383,#30384,#30385,#30386,#30387,#30388,#30389,#30390,
#30391,#30392,#30393,#30394,#30395,#30396,#30397,#30398,#30399,#30400,#30401,
#30402,#30403,#30404,#30405,#30406,#30407,#30408,#30409,#30410,#30411,#30412,
#30413,#30414,#30415,#30416,#30417,#30418,#30419,#30420,#30421,#30422,#30423,
#30424,#30425,#30426,#30427,#30428,#30429,#30430,#30431,#30432,#30433,#30434,
#30435,#30436,#30437,#30438,#30439,#30440,#30441),.UNSPECIFIED.,.F.,.F.)
B_SPLINE_CURVE_WITH_KNOTS((6,1,1,1,1,1,1,1,1,1,1,1,1,1,1,1,1,1,1,1,1,1,
1,1,1,1,1,1,1,1,1,1,1,1,1,1,1,1,1,1,1,1,1,1,1,1,1,1,1,1,1,1,1,1,1,1,1,1,
1,1,1,1,1,1,1,6),(0.,0.0153846153846154,0.0307692307692308,0.0461538461538462,
0.0615384615384615,0.0769230769230769,0.0923076923076923,0.107692307692308,
0.123076923076923,0.138461538461538,0.153846153846154,0.169230769230769,
0.184615384615385,0.2,0.215384615384615,0.230769230769231,0.246153846153846,
0.261538461538462,0.276923076923077,0.292307692307692,0.307692307692308,
0.323076923076923,0.338461538461538,0.353846153846154,0.369230769230769,
0.384615384615385,0.4,0.415384615384615,0.430769230769231,0.446153846153846,
0.461538461538462,0.476923076923077,0.492307692307692,0.507692307692308,
0.523076923076923,0.538461538461538,0.553846153846154,0.569230769230769,
0.584615384615384,0.6,0.615384615384615,0.63076923076923,0.646153846153846,
0.661538461538461,0.676923076923076,0.692307692307692,0.707692307692307,
0.723076923076922,0.738461538461538,0.753846153846153,0.769230769230768,
0.784615384615384,0.799999999999999,0.815384615384614,0.83076923076923,
0.846153846153845,0.86153846153846,0.876923076923076,0.892307692307691,
0.907692307692306,0.923076923076922,0.938461538461537,0.953846153846152,
0.969230769230768,0.984615384615383,0.994228156739689),.UNSPECIFIED.)
CURVE()
GEOMETRIC_REPRESENTATION_ITEM()
RATIONAL_B_SPLINE_CURVE((1.,1.,1.,1.,1.,1.,1.,1.,1.,1.,1.,1.,1.,1.,1.,1.,
1.,1.,1.,1.,1.,1.,1.,1.,1.,1.,1.,1.,1.,1.,1.,1.,1.,1.,1.,1.,1.,1.,1.,1.,
1.,1.,1.,1.,1.,1.,1.,1.,1.,1.,1.,1.,1.,1.,1.,1.,1.,1.,1.,1.,1.,1.,1.,1.,
1.,1.,1.,1.,1.,1.))
REPRESENTATION_ITEM('')
);
#215=(
BOUNDED_CURVE()
B_SPLINE_CURVE(5,(#30445,#30446,#30447,#30448,#30449,#30450,#30451,#30452,
#30453,#30454,#30455,#30456,#30457,#30458,#30459,#30460,#30461,#30462,#30463,
#30464,#30465,#30466,#30467,#30468,#30469,#30470,#30471,#30472,#30473,#30474,
#30475,#30476,#30477,#30478,#30479,#30480,#30481,#30482,#30483,#30484,#30485,
#30486,#30487,#30488,#30489,#30490,#30491,#30492,#30493,#30494,#30495,#30496,
#30497,#30498,#30499,#30500,#30501,#30502,#30503,#30504,#30505,#30506,#30507,
#30508,#30509,#30510,#30511,#30512,#30513,#30514),.UNSPECIFIED.,.F.,.F.)
B_SPLINE_CURVE_WITH_KNOTS((6,1,1,1,1,1,1,1,1,1,1,1,1,1,1,1,1,1,1,1,1,1,
1,1,1,1,1,1,1,1,1,1,1,1,1,1,1,1,1,1,1,1,1,1,1,1,1,1,1,1,1,1,1,1,1,1,1,1,
1,1,1,1,1,1,1,6),(0.00577184337448946,0.0153846153846154,0.0307692307692308,
0.0461538461538462,0.0615384615384615,0.0769230769230769,0.0923076923076923,
0.107692307692308,0.123076923076923,0.138461538461538,0.153846153846154,
0.169230769230769,0.184615384615385,0.2,0.215384615384615,0.230769230769231,
0.246153846153846,0.261538461538462,0.276923076923077,0.292307692307692,
0.307692307692308,0.323076923076923,0.338461538461538,0.353846153846154,
0.369230769230769,0.384615384615385,0.4,0.415384615384615,0.430769230769231,
0.446153846153846,0.461538461538462,0.476923076923077,0.492307692307692,
0.507692307692308,0.523076923076923,0.538461538461538,0.553846153846154,
0.569230769230769,0.584615384615384,0.6,0.615384615384615,0.63076923076923,
0.646153846153846,0.661538461538461,0.676923076923076,0.692307692307692,
0.707692307692307,0.723076923076922,0.738461538461538,0.753846153846153,
0.769230769230768,0.784615384615384,0.799999999999999,0.815384615384614,
0.83076923076923,0.846153846153845,0.86153846153846,0.876923076923076,0.892307692307691,
0.907692307692306,0.923076923076922,0.938461538461537,0.953846153846152,
0.969230769230768,0.984615384615383,1.),.UNSPECIFIED.)
CURVE()
GEOMETRIC_REPRESENTATION_ITEM()
RATIONAL_B_SPLINE_CURVE((1.,1.,1.,1.,1.,1.,1.,1.,1.,1.,1.,1.,1.,1.,1.,1.,
1.,1.,1.,1.,1.,1.,1.,1.,1.,1.,1.,1.,1.,1.,1.,1.,1.,1.,1.,1.,1.,1.,1.,1.,
1.,1.,1.,1.,1.,1.,1.,1.,1.,1.,1.,1.,1.,1.,1.,1.,1.,1.,1.,1.,1.,1.,1.,1.,
1.,1.,1.,1.,1.,1.))
REPRESENTATION_ITEM('')
);
#216=(
BOUNDED_CURVE()
B_SPLINE_CURVE(5,(#30518,#30519,#30520,#30521,#30522,#30523,#30524,#30525,
#30526,#30527,#30528,#30529,#30530,#30531,#30532,#30533,#30534,#30535,#30536,
#30537,#30538,#30539,#30540,#30541,#30542,#30543,#30544,#30545,#30546,#30547,
#30548,#30549,#30550,#30551,#30552,#30553,#30554,#30555,#30556,#30557,#30558,
#30559,#30560,#30561,#30562,#30563,#30564,#30565,#30566,#30567,#30568,#30569,
#30570,#30571,#30572,#30573,#30574,#30575,#30576,#30577,#30578,#30579,#30580,
#30581,#30582,#30583,#30584,#30585,#30586,#30587),.UNSPECIFIED.,.F.,.F.)
B_SPLINE_CURVE_WITH_KNOTS((6,1,1,1,1,1,1,1,1,1,1,1,1,1,1,1,1,1,1,1,1,1,
1,1,1,1,1,1,1,1,1,1,1,1,1,1,1,1,1,1,1,1,1,1,1,1,1,1,1,1,1,1,1,1,1,1,1,1,
1,1,1,1,1,1,1,6),(0.,0.0153846153846154,0.0307692307692308,0.0461538461538462,
0.0615384615384615,0.0769230769230769,0.0923076923076923,0.107692307692308,
0.123076923076923,0.138461538461538,0.153846153846154,0.169230769230769,
0.184615384615385,0.2,0.215384615384615,0.230769230769231,0.246153846153846,
0.261538461538462,0.276923076923077,0.292307692307692,0.307692307692308,
0.323076923076923,0.338461538461538,0.353846153846154,0.369230769230769,
0.384615384615385,0.4,0.415384615384615,0.430769230769231,0.446153846153846,
0.461538461538462,0.476923076923077,0.492307692307692,0.507692307692308,
0.523076923076923,0.538461538461538,0.553846153846154,0.569230769230769,
0.584615384615384,0.6,0.615384615384615,0.63076923076923,0.646153846153846,
0.661538461538461,0.676923076923076,0.692307692307692,0.707692307692307,
0.723076923076922,0.738461538461538,0.753846153846153,0.769230769230768,
0.784615384615384,0.799999999999999,0.815384615384614,0.83076923076923,
0.846153846153845,0.86153846153846,0.876923076923076,0.892307692307691,
0.907692307692306,0.923076923076922,0.938461538461537,0.953846153846152,
0.969230769230768,0.984615384615383,0.994228156739718),.UNSPECIFIED.)
CURVE()
GEOMETRIC_REPRESENTATION_ITEM()
RATIONAL_B_SPLINE_CURVE((1.,1.,1.,1.,1.,1.,1.,1.,1.,1.,1.,1.,1.,1.,1.,1.,
1.,1.,1.,1.,1.,1.,1.,1.,1.,1.,1.,1.,1.,1.,1.,1.,1.,1.,1.,1.,1.,1.,1.,1.,
1.,1.,1.,1.,1.,1.,1.,1.,1.,1.,1.,1.,1.,1.,1.,1.,1.,1.,1.,1.,1.,1.,1.,1.,
1.,1.,1.,1.,1.,1.))
REPRESENTATION_ITEM('')
);
#217=(
BOUNDED_CURVE()
B_SPLINE_CURVE(5,(#30591,#30592,#30593,#30594,#30595,#30596,#30597,#30598,
#30599,#30600,#30601,#30602,#30603,#30604,#30605,#30606,#30607,#30608,#30609,
#30610,#30611,#30612,#30613,#30614,#30615,#30616,#30617,#30618,#30619,#30620,
#30621,#30622,#30623,#30624,#30625,#30626,#30627,#30628,#30629,#30630,#30631,
#30632,#30633,#30634,#30635,#30636,#30637,#30638,#30639,#30640,#30641,#30642,
#30643,#30644,#30645,#30646,#30647,#30648,#30649,#30650,#30651,#30652,#30653,
#30654,#30655,#30656,#30657,#30658,#30659,#30660),.UNSPECIFIED.,.F.,.F.)
B_SPLINE_CURVE_WITH_KNOTS((6,1,1,1,1,1,1,1,1,1,1,1,1,1,1,1,1,1,1,1,1,1,
1,1,1,1,1,1,1,1,1,1,1,1,1,1,1,1,1,1,1,1,1,1,1,1,1,1,1,1,1,1,1,1,1,1,1,1,
1,1,1,1,1,1,1,6),(0.00577184337450897,0.0153846153846154,0.0307692307692308,
0.0461538461538462,0.0615384615384615,0.0769230769230769,0.0923076923076923,
0.107692307692308,0.123076923076923,0.138461538461538,0.153846153846154,
0.169230769230769,0.184615384615385,0.2,0.215384615384615,0.230769230769231,
0.246153846153846,0.261538461538462,0.276923076923077,0.292307692307692,
0.307692307692308,0.323076923076923,0.338461538461538,0.353846153846154,
0.369230769230769,0.384615384615385,0.4,0.415384615384615,0.430769230769231,
0.446153846153846,0.461538461538462,0.476923076923077,0.492307692307692,
0.507692307692308,0.523076923076923,0.538461538461538,0.553846153846154,
0.569230769230769,0.584615384615384,0.6,0.615384615384615,0.63076923076923,
0.646153846153846,0.661538461538461,0.676923076923076,0.692307692307692,
0.707692307692307,0.723076923076922,0.738461538461538,0.753846153846153,
0.769230769230768,0.784615384615384,0.799999999999999,0.815384615384614,
0.83076923076923,0.846153846153845,0.86153846153846,0.876923076923076,0.892307692307691,
0.907692307692306,0.923076923076922,0.938461538461537,0.953846153846152,
0.969230769230768,0.984615384615383,1.),.UNSPECIFIED.)
CURVE()
GEOMETRIC_REPRESENTATION_ITEM()
RATIONAL_B_SPLINE_CURVE((1.,1.,1.,1.,1.,1.,1.,1.,1.,1.,1.,1.,1.,1.,1.,1.,
1.,1.,1.,1.,1.,1.,1.,1.,1.,1.,1.,1.,1.,1.,1.,1.,1.,1.,1.,1.,1.,1.,1.,1.,
1.,1.,1.,1.,1.,1.,1.,1.,1.,1.,1.,1.,1.,1.,1.,1.,1.,1.,1.,1.,1.,1.,1.,1.,
1.,1.,1.,1.,1.,1.))
REPRESENTATION_ITEM('')
);
#218=(
BOUNDED_CURVE()
B_SPLINE_CURVE(5,(#30664,#30665,#30666,#30667,#30668,#30669,#30670,#30671,
#30672,#30673,#30674,#30675,#30676,#30677,#30678,#30679,#30680,#30681,#30682,
#30683,#30684,#30685,#30686,#30687,#30688,#30689,#30690,#30691,#30692,#30693,
#30694,#30695,#30696,#30697,#30698,#30699,#30700,#30701,#30702,#30703,#30704,
#30705,#30706,#30707,#30708,#30709,#30710,#30711,#30712,#30713,#30714,#30715,
#30716,#30717,#30718,#30719,#30720,#30721,#30722,#30723,#30724,#30725,#30726,
#30727,#30728,#30729,#30730,#30731,#30732,#30733),.UNSPECIFIED.,.F.,.F.)
B_SPLINE_CURVE_WITH_KNOTS((6,1,1,1,1,1,1,1,1,1,1,1,1,1,1,1,1,1,1,1,1,1,
1,1,1,1,1,1,1,1,1,1,1,1,1,1,1,1,1,1,1,1,1,1,1,1,1,1,1,1,1,1,1,1,1,1,1,1,
1,1,1,1,1,1,1,6),(0.,0.0153846153846154,0.0307692307692308,0.0461538461538462,
0.0615384615384615,0.0769230769230769,0.0923076923076923,0.107692307692308,
0.123076923076923,0.138461538461538,0.153846153846154,0.169230769230769,
0.184615384615385,0.2,0.215384615384615,0.230769230769231,0.246153846153846,
0.261538461538462,0.276923076923077,0.292307692307692,0.307692307692308,
0.323076923076923,0.338461538461538,0.353846153846154,0.369230769230769,
0.384615384615385,0.4,0.415384615384615,0.430769230769231,0.446153846153846,
0.461538461538462,0.476923076923077,0.492307692307692,0.507692307692308,
0.523076923076923,0.538461538461538,0.553846153846154,0.569230769230769,
0.584615384615384,0.6,0.615384615384615,0.63076923076923,0.646153846153846,
0.661538461538461,0.676923076923076,0.692307692307692,0.707692307692307,
0.723076923076922,0.738461538461538,0.753846153846153,0.769230769230768,
0.784615384615384,0.799999999999999,0.815384615384614,0.83076923076923,
0.846153846153845,0.86153846153846,0.876923076923076,0.892307692307691,
0.907692307692306,0.923076923076922,0.938461538461537,0.953846153846152,
0.969230769230768,0.984615384615383,0.994228156739701),.UNSPECIFIED.)
CURVE()
GEOMETRIC_REPRESENTATION_ITEM()
RATIONAL_B_SPLINE_CURVE((1.,1.,1.,1.,1.,1.,1.,1.,1.,1.,1.,1.,1.,1.,1.,1.,
1.,1.,1.,1.,1.,1.,1.,1.,1.,1.,1.,1.,1.,1.,1.,1.,1.,1.,1.,1.,1.,1.,1.,1.,
1.,1.,1.,1.,1.,1.,1.,1.,1.,1.,1.,1.,1.,1.,1.,1.,1.,1.,1.,1.,1.,1.,1.,1.,
1.,1.,1.,1.,1.,1.))
REPRESENTATION_ITEM('')
);
#219=(
BOUNDED_CURVE()
B_SPLINE_CURVE(5,(#30737,#30738,#30739,#30740,#30741,#30742,#30743,#30744,
#30745,#30746,#30747,#30748,#30749,#30750,#30751,#30752,#30753,#30754,#30755,
#30756,#30757,#30758,#30759,#30760,#30761,#30762,#30763,#30764,#30765,#30766,
#30767,#30768,#30769,#30770,#30771,#30772,#30773,#30774,#30775,#30776,#30777,
#30778,#30779,#30780,#30781,#30782,#30783,#30784,#30785,#30786,#30787,#30788,
#30789,#30790,#30791,#30792,#30793,#30794,#30795,#30796,#30797,#30798,#30799,
#30800,#30801,#30802,#30803,#30804,#30805,#30806),.UNSPECIFIED.,.F.,.F.)
B_SPLINE_CURVE_WITH_KNOTS((6,1,1,1,1,1,1,1,1,1,1,1,1,1,1,1,1,1,1,1,1,1,
1,1,1,1,1,1,1,1,1,1,1,1,1,1,1,1,1,1,1,1,1,1,1,1,1,1,1,1,1,1,1,1,1,1,1,1,
1,1,1,1,1,1,1,6),(0.00577184337451001,0.0153846153846154,0.0307692307692308,
0.0461538461538462,0.0615384615384615,0.0769230769230769,0.0923076923076923,
0.107692307692308,0.123076923076923,0.138461538461538,0.153846153846154,
0.169230769230769,0.184615384615385,0.2,0.215384615384615,0.230769230769231,
0.246153846153846,0.261538461538462,0.276923076923077,0.292307692307692,
0.307692307692308,0.323076923076923,0.338461538461538,0.353846153846154,
0.369230769230769,0.384615384615385,0.4,0.415384615384615,0.430769230769231,
0.446153846153846,0.461538461538462,0.476923076923077,0.492307692307692,
0.507692307692308,0.523076923076923,0.538461538461538,0.553846153846154,
0.569230769230769,0.584615384615384,0.6,0.615384615384615,0.63076923076923,
0.646153846153846,0.661538461538461,0.676923076923076,0.692307692307692,
0.707692307692307,0.723076923076922,0.738461538461538,0.753846153846153,
0.769230769230768,0.784615384615384,0.799999999999999,0.815384615384614,
0.83076923076923,0.846153846153845,0.86153846153846,0.876923076923076,0.892307692307691,
0.907692307692306,0.923076923076922,0.938461538461537,0.953846153846152,
0.969230769230768,0.984615384615383,1.),.UNSPECIFIED.)
CURVE()
GEOMETRIC_REPRESENTATION_ITEM()
RATIONAL_B_SPLINE_CURVE((1.,1.,1.,1.,1.,1.,1.,1.,1.,1.,1.,1.,1.,1.,1.,1.,
1.,1.,1.,1.,1.,1.,1.,1.,1.,1.,1.,1.,1.,1.,1.,1.,1.,1.,1.,1.,1.,1.,1.,1.,
1.,1.,1.,1.,1.,1.,1.,1.,1.,1.,1.,1.,1.,1.,1.,1.,1.,1.,1.,1.,1.,1.,1.,1.,
1.,1.,1.,1.,1.,1.))
REPRESENTATION_ITEM('')
);
#220=(
BOUNDED_CURVE()
B_SPLINE_CURVE(5,(#30810,#30811,#30812,#30813,#30814,#30815,#30816,#30817,
#30818,#30819,#30820,#30821,#30822,#30823,#30824,#30825,#30826,#30827,#30828,
#30829,#30830,#30831,#30832,#30833,#30834,#30835,#30836,#30837,#30838,#30839,
#30840,#30841,#30842,#30843,#30844,#30845,#30846,#30847,#30848,#30849,#30850,
#30851,#30852,#30853,#30854,#30855,#30856,#30857,#30858,#30859,#30860,#30861,
#30862,#30863,#30864,#30865,#30866,#30867,#30868,#30869,#30870,#30871,#30872,
#30873,#30874,#30875,#30876,#30877,#30878,#30879),.UNSPECIFIED.,.F.,.F.)
B_SPLINE_CURVE_WITH_KNOTS((6,1,1,1,1,1,1,1,1,1,1,1,1,1,1,1,1,1,1,1,1,1,
1,1,1,1,1,1,1,1,1,1,1,1,1,1,1,1,1,1,1,1,1,1,1,1,1,1,1,1,1,1,1,1,1,1,1,1,
1,1,1,1,1,1,1,6),(0.,0.0153846153846154,0.0307692307692308,0.0461538461538462,
0.0615384615384615,0.0769230769230769,0.0923076923076923,0.107692307692308,
0.123076923076923,0.138461538461538,0.153846153846154,0.169230769230769,
0.184615384615385,0.2,0.215384615384615,0.230769230769231,0.246153846153846,
0.261538461538462,0.276923076923077,0.292307692307692,0.307692307692308,
0.323076923076923,0.338461538461538,0.353846153846154,0.369230769230769,
0.384615384615385,0.4,0.415384615384615,0.430769230769231,0.446153846153846,
0.461538461538462,0.476923076923077,0.492307692307692,0.507692307692308,
0.523076923076923,0.538461538461538,0.553846153846154,0.569230769230769,
0.584615384615384,0.6,0.615384615384615,0.63076923076923,0.646153846153846,
0.661538461538461,0.676923076923076,0.692307692307692,0.707692307692307,
0.723076923076922,0.738461538461538,0.753846153846153,0.769230769230768,
0.784615384615384,0.799999999999999,0.815384615384614,0.83076923076923,
0.846153846153845,0.86153846153846,0.876923076923076,0.892307692307691,
0.907692307692306,0.923076923076922,0.938461538461537,0.953846153846152,
0.969230769230768,0.984615384615383,0.994228156739697),.UNSPECIFIED.)
CURVE()
GEOMETRIC_REPRESENTATION_ITEM()
RATIONAL_B_SPLINE_CURVE((1.,1.,1.,1.,1.,1.,1.,1.,1.,1.,1.,1.,1.,1.,1.,1.,
1.,1.,1.,1.,1.,1.,1.,1.,1.,1.,1.,1.,1.,1.,1.,1.,1.,1.,1.,1.,1.,1.,1.,1.,
1.,1.,1.,1.,1.,1.,1.,1.,1.,1.,1.,1.,1.,1.,1.,1.,1.,1.,1.,1.,1.,1.,1.,1.,
1.,1.,1.,1.,1.,1.))
REPRESENTATION_ITEM('')
);
#221=(
BOUNDED_CURVE()
B_SPLINE_CURVE(5,(#30883,#30884,#30885,#30886,#30887,#30888,#30889,#30890,
#30891,#30892,#30893,#30894,#30895,#30896,#30897,#30898,#30899,#30900,#30901,
#30902,#30903,#30904,#30905,#30906,#30907,#30908,#30909,#30910,#30911,#30912,
#30913,#30914,#30915,#30916,#30917,#30918,#30919,#30920,#30921,#30922,#30923,
#30924,#30925,#30926,#30927,#30928,#30929,#30930,#30931,#30932,#30933,#30934,
#30935,#30936,#30937,#30938,#30939,#30940,#30941,#30942,#30943,#30944,#30945,
#30946,#30947,#30948,#30949,#30950,#30951,#30952),.UNSPECIFIED.,.F.,.F.)
B_SPLINE_CURVE_WITH_KNOTS((6,1,1,1,1,1,1,1,1,1,1,1,1,1,1,1,1,1,1,1,1,1,
1,1,1,1,1,1,1,1,1,1,1,1,1,1,1,1,1,1,1,1,1,1,1,1,1,1,1,1,1,1,1,1,1,1,1,1,
1,1,1,1,1,1,1,6),(0.00577184337452306,0.0153846153846154,0.0307692307692308,
0.0461538461538462,0.0615384615384615,0.0769230769230769,0.0923076923076923,
0.107692307692308,0.123076923076923,0.138461538461538,0.153846153846154,
0.169230769230769,0.184615384615385,0.2,0.215384615384615,0.230769230769231,
0.246153846153846,0.261538461538462,0.276923076923077,0.292307692307692,
0.307692307692308,0.323076923076923,0.338461538461538,0.353846153846154,
0.369230769230769,0.384615384615385,0.4,0.415384615384615,0.430769230769231,
0.446153846153846,0.461538461538462,0.476923076923077,0.492307692307692,
0.507692307692308,0.523076923076923,0.538461538461538,0.553846153846154,
0.569230769230769,0.584615384615384,0.6,0.615384615384615,0.63076923076923,
0.646153846153846,0.661538461538461,0.676923076923076,0.692307692307692,
0.707692307692307,0.723076923076922,0.738461538461538,0.753846153846153,
0.769230769230768,0.784615384615384,0.799999999999999,0.815384615384614,
0.83076923076923,0.846153846153845,0.86153846153846,0.876923076923076,0.892307692307691,
0.907692307692306,0.923076923076922,0.938461538461537,0.953846153846152,
0.969230769230768,0.984615384615383,1.),.UNSPECIFIED.)
CURVE()
GEOMETRIC_REPRESENTATION_ITEM()
RATIONAL_B_SPLINE_CURVE((1.,1.,1.,1.,1.,1.,1.,1.,1.,1.,1.,1.,1.,1.,1.,1.,
1.,1.,1.,1.,1.,1.,1.,1.,1.,1.,1.,1.,1.,1.,1.,1.,1.,1.,1.,1.,1.,1.,1.,1.,
1.,1.,1.,1.,1.,1.,1.,1.,1.,1.,1.,1.,1.,1.,1.,1.,1.,1.,1.,1.,1.,1.,1.,1.,
1.,1.,1.,1.,1.,1.))
REPRESENTATION_ITEM('')
);
#222=(
BOUNDED_CURVE()
B_SPLINE_CURVE(5,(#30956,#30957,#30958,#30959,#30960,#30961,#30962,#30963,
#30964,#30965,#30966,#30967,#30968,#30969,#30970,#30971,#30972,#30973,#30974,
#30975,#30976,#30977,#30978,#30979,#30980,#30981,#30982,#30983,#30984,#30985,
#30986,#30987,#30988,#30989,#30990,#30991,#30992,#30993,#30994,#30995,#30996,
#30997,#30998,#30999,#31000,#31001,#31002,#31003,#31004,#31005,#31006,#31007,
#31008,#31009,#31010,#31011,#31012,#31013,#31014,#31015,#31016,#31017,#31018,
#31019,#31020,#31021,#31022,#31023,#31024,#31025),.UNSPECIFIED.,.F.,.F.)
B_SPLINE_CURVE_WITH_KNOTS((6,1,1,1,1,1,1,1,1,1,1,1,1,1,1,1,1,1,1,1,1,1,
1,1,1,1,1,1,1,1,1,1,1,1,1,1,1,1,1,1,1,1,1,1,1,1,1,1,1,1,1,1,1,1,1,1,1,1,
1,1,1,1,1,1,1,6),(0.,0.0153846153846154,0.0307692307692308,0.0461538461538462,
0.0615384615384615,0.0769230769230769,0.0923076923076923,0.107692307692308,
0.123076923076923,0.138461538461538,0.153846153846154,0.169230769230769,
0.184615384615385,0.2,0.215384615384615,0.230769230769231,0.246153846153846,
0.261538461538462,0.276923076923077,0.292307692307692,0.307692307692308,
0.323076923076923,0.338461538461538,0.353846153846154,0.369230769230769,
0.384615384615385,0.4,0.415384615384615,0.430769230769231,0.446153846153846,
0.461538461538462,0.476923076923077,0.492307692307692,0.507692307692308,
0.523076923076923,0.538461538461538,0.553846153846154,0.569230769230769,
0.584615384615384,0.6,0.615384615384615,0.63076923076923,0.646153846153846,
0.661538461538461,0.676923076923076,0.692307692307692,0.707692307692307,
0.723076923076922,0.738461538461538,0.753846153846153,0.769230769230768,
0.784615384615384,0.799999999999999,0.815384615384614,0.83076923076923,
0.846153846153845,0.86153846153846,0.876923076923076,0.892307692307691,
0.907692307692306,0.923076923076922,0.938461538461537,0.953846153846152,
0.969230769230768,0.984615384615383,0.994228156739688),.UNSPECIFIED.)
CURVE()
GEOMETRIC_REPRESENTATION_ITEM()
RATIONAL_B_SPLINE_CURVE((1.,1.,1.,1.,1.,1.,1.,1.,1.,1.,1.,1.,1.,1.,1.,1.,
1.,1.,1.,1.,1.,1.,1.,1.,1.,1.,1.,1.,1.,1.,1.,1.,1.,1.,1.,1.,1.,1.,1.,1.,
1.,1.,1.,1.,1.,1.,1.,1.,1.,1.,1.,1.,1.,1.,1.,1.,1.,1.,1.,1.,1.,1.,1.,1.,
1.,1.,1.,1.,1.,1.))
REPRESENTATION_ITEM('')
);
#223=(
BOUNDED_CURVE()
B_SPLINE_CURVE(5,(#31029,#31030,#31031,#31032,#31033,#31034,#31035,#31036,
#31037,#31038,#31039,#31040,#31041,#31042,#31043,#31044,#31045,#31046,#31047,
#31048,#31049,#31050,#31051,#31052,#31053,#31054,#31055,#31056,#31057,#31058,
#31059,#31060,#31061,#31062,#31063,#31064,#31065,#31066,#31067,#31068,#31069,
#31070,#31071,#31072,#31073,#31074,#31075,#31076,#31077,#31078,#31079,#31080,
#31081,#31082,#31083,#31084,#31085,#31086,#31087,#31088,#31089,#31090,#31091,
#31092,#31093,#31094,#31095,#31096,#31097,#31098),.UNSPECIFIED.,.F.,.F.)
B_SPLINE_CURVE_WITH_KNOTS((6,1,1,1,1,1,1,1,1,1,1,1,1,1,1,1,1,1,1,1,1,1,
1,1,1,1,1,1,1,1,1,1,1,1,1,1,1,1,1,1,1,1,1,1,1,1,1,1,1,1,1,1,1,1,1,1,1,1,
1,1,1,1,1,1,1,6),(0.00577184337449862,0.0153846153846154,0.0307692307692308,
0.0461538461538462,0.0615384615384615,0.0769230769230769,0.0923076923076923,
0.107692307692308,0.123076923076923,0.138461538461538,0.153846153846154,
0.169230769230769,0.184615384615385,0.2,0.215384615384615,0.230769230769231,
0.246153846153846,0.261538461538462,0.276923076923077,0.292307692307692,
0.307692307692308,0.323076923076923,0.338461538461538,0.353846153846154,
0.369230769230769,0.384615384615385,0.4,0.415384615384615,0.430769230769231,
0.446153846153846,0.461538461538462,0.476923076923077,0.492307692307692,
0.507692307692308,0.523076923076923,0.538461538461538,0.553846153846154,
0.569230769230769,0.584615384615384,0.6,0.615384615384615,0.63076923076923,
0.646153846153846,0.661538461538461,0.676923076923076,0.692307692307692,
0.707692307692307,0.723076923076922,0.738461538461538,0.753846153846153,
0.769230769230768,0.784615384615384,0.799999999999999,0.815384615384614,
0.83076923076923,0.846153846153845,0.86153846153846,0.876923076923076,0.892307692307691,
0.907692307692306,0.923076923076922,0.938461538461537,0.953846153846152,
0.969230769230768,0.984615384615383,1.),.UNSPECIFIED.)
CURVE()
GEOMETRIC_REPRESENTATION_ITEM()
RATIONAL_B_SPLINE_CURVE((1.,1.,1.,1.,1.,1.,1.,1.,1.,1.,1.,1.,1.,1.,1.,1.,
1.,1.,1.,1.,1.,1.,1.,1.,1.,1.,1.,1.,1.,1.,1.,1.,1.,1.,1.,1.,1.,1.,1.,1.,
1.,1.,1.,1.,1.,1.,1.,1.,1.,1.,1.,1.,1.,1.,1.,1.,1.,1.,1.,1.,1.,1.,1.,1.,
1.,1.,1.,1.,1.,1.))
REPRESENTATION_ITEM('')
);
#224=(
BOUNDED_CURVE()
B_SPLINE_CURVE(5,(#31102,#31103,#31104,#31105,#31106,#31107,#31108,#31109,
#31110,#31111,#31112,#31113,#31114,#31115,#31116,#31117,#31118,#31119,#31120,
#31121,#31122,#31123,#31124,#31125,#31126,#31127,#31128,#31129,#31130,#31131,
#31132,#31133,#31134,#31135,#31136,#31137,#31138,#31139,#31140,#31141,#31142,
#31143,#31144,#31145,#31146,#31147,#31148,#31149,#31150,#31151,#31152,#31153,
#31154,#31155,#31156,#31157,#31158,#31159,#31160,#31161,#31162,#31163,#31164,
#31165,#31166,#31167,#31168,#31169,#31170,#31171),.UNSPECIFIED.,.F.,.F.)
B_SPLINE_CURVE_WITH_KNOTS((6,1,1,1,1,1,1,1,1,1,1,1,1,1,1,1,1,1,1,1,1,1,
1,1,1,1,1,1,1,1,1,1,1,1,1,1,1,1,1,1,1,1,1,1,1,1,1,1,1,1,1,1,1,1,1,1,1,1,
1,1,1,1,1,1,1,6),(0.,0.0153846153846154,0.0307692307692308,0.0461538461538462,
0.0615384615384615,0.0769230769230769,0.0923076923076923,0.107692307692308,
0.123076923076923,0.138461538461538,0.153846153846154,0.169230769230769,
0.184615384615385,0.2,0.215384615384615,0.230769230769231,0.246153846153846,
0.261538461538462,0.276923076923077,0.292307692307692,0.307692307692308,
0.323076923076923,0.338461538461538,0.353846153846154,0.369230769230769,
0.384615384615385,0.4,0.415384615384615,0.430769230769231,0.446153846153846,
0.461538461538462,0.476923076923077,0.492307692307692,0.507692307692308,
0.523076923076923,0.538461538461538,0.553846153846154,0.569230769230769,
0.584615384615384,0.6,0.615384615384615,0.63076923076923,0.646153846153846,
0.661538461538461,0.676923076923076,0.692307692307692,0.707692307692307,
0.723076923076922,0.738461538461538,0.753846153846153,0.769230769230768,
0.784615384615384,0.799999999999999,0.815384615384614,0.83076923076923,
0.846153846153845,0.86153846153846,0.876923076923076,0.892307692307691,
0.907692307692306,0.923076923076922,0.938461538461537,0.953846153846152,
0.969230769230768,0.984615384615383,0.994228156739696),.UNSPECIFIED.)
CURVE()
GEOMETRIC_REPRESENTATION_ITEM()
RATIONAL_B_SPLINE_CURVE((1.,1.,1.,1.,1.,1.,1.,1.,1.,1.,1.,1.,1.,1.,1.,1.,
1.,1.,1.,1.,1.,1.,1.,1.,1.,1.,1.,1.,1.,1.,1.,1.,1.,1.,1.,1.,1.,1.,1.,1.,
1.,1.,1.,1.,1.,1.,1.,1.,1.,1.,1.,1.,1.,1.,1.,1.,1.,1.,1.,1.,1.,1.,1.,1.,
1.,1.,1.,1.,1.,1.))
REPRESENTATION_ITEM('')
);
#225=(
BOUNDED_CURVE()
B_SPLINE_CURVE(5,(#31175,#31176,#31177,#31178,#31179,#31180,#31181,#31182,
#31183,#31184,#31185,#31186,#31187,#31188,#31189,#31190,#31191,#31192,#31193,
#31194,#31195,#31196,#31197,#31198,#31199,#31200,#31201,#31202,#31203,#31204,
#31205,#31206,#31207,#31208,#31209,#31210,#31211,#31212,#31213,#31214,#31215,
#31216,#31217,#31218,#31219,#31220,#31221,#31222,#31223,#31224,#31225,#31226,
#31227,#31228,#31229,#31230,#31231,#31232,#31233,#31234,#31235,#31236,#31237,
#31238,#31239,#31240,#31241,#31242,#31243,#31244),.UNSPECIFIED.,.F.,.F.)
B_SPLINE_CURVE_WITH_KNOTS((6,1,1,1,1,1,1,1,1,1,1,1,1,1,1,1,1,1,1,1,1,1,
1,1,1,1,1,1,1,1,1,1,1,1,1,1,1,1,1,1,1,1,1,1,1,1,1,1,1,1,1,1,1,1,1,1,1,1,
1,1,1,1,1,1,1,6),(0.00577184337452068,0.0153846153846154,0.0307692307692308,
0.0461538461538462,0.0615384615384615,0.0769230769230769,0.0923076923076923,
0.107692307692308,0.123076923076923,0.138461538461538,0.153846153846154,
0.169230769230769,0.184615384615385,0.2,0.215384615384615,0.230769230769231,
0.246153846153846,0.261538461538462,0.276923076923077,0.292307692307692,
0.307692307692308,0.323076923076923,0.338461538461538,0.353846153846154,
0.369230769230769,0.384615384615385,0.4,0.415384615384615,0.430769230769231,
0.446153846153846,0.461538461538462,0.476923076923077,0.492307692307692,
0.507692307692308,0.523076923076923,0.538461538461538,0.553846153846154,
0.569230769230769,0.584615384615384,0.6,0.615384615384615,0.63076923076923,
0.646153846153846,0.661538461538461,0.676923076923076,0.692307692307692,
0.707692307692307,0.723076923076922,0.738461538461538,0.753846153846153,
0.769230769230768,0.784615384615384,0.799999999999999,0.815384615384614,
0.83076923076923,0.846153846153845,0.86153846153846,0.876923076923076,0.892307692307691,
0.907692307692306,0.923076923076922,0.938461538461537,0.953846153846152,
0.969230769230768,0.984615384615383,1.),.UNSPECIFIED.)
CURVE()
GEOMETRIC_REPRESENTATION_ITEM()
RATIONAL_B_SPLINE_CURVE((1.,1.,1.,1.,1.,1.,1.,1.,1.,1.,1.,1.,1.,1.,1.,1.,
1.,1.,1.,1.,1.,1.,1.,1.,1.,1.,1.,1.,1.,1.,1.,1.,1.,1.,1.,1.,1.,1.,1.,1.,
1.,1.,1.,1.,1.,1.,1.,1.,1.,1.,1.,1.,1.,1.,1.,1.,1.,1.,1.,1.,1.,1.,1.,1.,
1.,1.,1.,1.,1.,1.))
REPRESENTATION_ITEM('')
);
#226=(
BOUNDED_CURVE()
B_SPLINE_CURVE(5,(#31248,#31249,#31250,#31251,#31252,#31253,#31254,#31255,
#31256,#31257,#31258,#31259,#31260,#31261,#31262,#31263,#31264,#31265,#31266,
#31267,#31268,#31269,#31270,#31271,#31272,#31273,#31274,#31275,#31276,#31277,
#31278,#31279,#31280,#31281,#31282,#31283,#31284,#31285,#31286,#31287,#31288,
#31289,#31290,#31291,#31292,#31293,#31294,#31295,#31296,#31297,#31298,#31299,
#31300,#31301,#31302,#31303,#31304,#31305,#31306,#31307,#31308,#31309,#31310,
#31311,#31312,#31313,#31314,#31315,#31316,#31317),.UNSPECIFIED.,.F.,.F.)
B_SPLINE_CURVE_WITH_KNOTS((6,1,1,1,1,1,1,1,1,1,1,1,1,1,1,1,1,1,1,1,1,1,
1,1,1,1,1,1,1,1,1,1,1,1,1,1,1,1,1,1,1,1,1,1,1,1,1,1,1,1,1,1,1,1,1,1,1,1,
1,1,1,1,1,1,1,6),(0.,0.0153846153846154,0.0307692307692308,0.0461538461538462,
0.0615384615384615,0.0769230769230769,0.0923076923076923,0.107692307692308,
0.123076923076923,0.138461538461538,0.153846153846154,0.169230769230769,
0.184615384615385,0.2,0.215384615384615,0.230769230769231,0.246153846153846,
0.261538461538462,0.276923076923077,0.292307692307692,0.307692307692308,
0.323076923076923,0.338461538461538,0.353846153846154,0.369230769230769,
0.384615384615385,0.4,0.415384615384615,0.430769230769231,0.446153846153846,
0.461538461538462,0.476923076923077,0.492307692307692,0.507692307692308,
0.523076923076923,0.538461538461538,0.553846153846154,0.569230769230769,
0.584615384615384,0.6,0.615384615384615,0.63076923076923,0.646153846153846,
0.661538461538461,0.676923076923076,0.692307692307692,0.707692307692307,
0.723076923076922,0.738461538461538,0.753846153846153,0.769230769230768,
0.784615384615384,0.799999999999999,0.815384615384614,0.83076923076923,
0.846153846153845,0.86153846153846,0.876923076923076,0.892307692307691,
0.907692307692306,0.923076923076922,0.938461538461537,0.953846153846152,
0.969230769230768,0.984615384615383,0.994228156739698),.UNSPECIFIED.)
CURVE()
GEOMETRIC_REPRESENTATION_ITEM()
RATIONAL_B_SPLINE_CURVE((1.,1.,1.,1.,1.,1.,1.,1.,1.,1.,1.,1.,1.,1.,1.,1.,
1.,1.,1.,1.,1.,1.,1.,1.,1.,1.,1.,1.,1.,1.,1.,1.,1.,1.,1.,1.,1.,1.,1.,1.,
1.,1.,1.,1.,1.,1.,1.,1.,1.,1.,1.,1.,1.,1.,1.,1.,1.,1.,1.,1.,1.,1.,1.,1.,
1.,1.,1.,1.,1.,1.))
REPRESENTATION_ITEM('')
);
#227=(
BOUNDED_CURVE()
B_SPLINE_CURVE(5,(#31321,#31322,#31323,#31324,#31325,#31326,#31327,#31328,
#31329,#31330,#31331,#31332,#31333,#31334,#31335,#31336,#31337,#31338,#31339,
#31340,#31341,#31342,#31343,#31344,#31345,#31346,#31347,#31348,#31349,#31350,
#31351,#31352,#31353,#31354,#31355,#31356,#31357,#31358,#31359,#31360,#31361,
#31362,#31363,#31364,#31365,#31366,#31367,#31368,#31369,#31370,#31371,#31372,
#31373,#31374,#31375,#31376,#31377,#31378,#31379,#31380,#31381,#31382,#31383,
#31384,#31385,#31386,#31387,#31388,#31389,#31390),.UNSPECIFIED.,.F.,.F.)
B_SPLINE_CURVE_WITH_KNOTS((6,1,1,1,1,1,1,1,1,1,1,1,1,1,1,1,1,1,1,1,1,1,
1,1,1,1,1,1,1,1,1,1,1,1,1,1,1,1,1,1,1,1,1,1,1,1,1,1,1,1,1,1,1,1,1,1,1,1,
1,1,1,1,1,1,1,6),(0.00577184337451607,0.0153846153846154,0.0307692307692308,
0.0461538461538462,0.0615384615384615,0.0769230769230769,0.0923076923076923,
0.107692307692308,0.123076923076923,0.138461538461538,0.153846153846154,
0.169230769230769,0.184615384615385,0.2,0.215384615384615,0.230769230769231,
0.246153846153846,0.261538461538462,0.276923076923077,0.292307692307692,
0.307692307692308,0.323076923076923,0.338461538461538,0.353846153846154,
0.369230769230769,0.384615384615385,0.4,0.415384615384615,0.430769230769231,
0.446153846153846,0.461538461538462,0.476923076923077,0.492307692307692,
0.507692307692308,0.523076923076923,0.538461538461538,0.553846153846154,
0.569230769230769,0.584615384615384,0.6,0.615384615384615,0.63076923076923,
0.646153846153846,0.661538461538461,0.676923076923076,0.692307692307692,
0.707692307692307,0.723076923076922,0.738461538461538,0.753846153846153,
0.769230769230768,0.784615384615384,0.799999999999999,0.815384615384614,
0.83076923076923,0.846153846153845,0.86153846153846,0.876923076923076,0.892307692307691,
0.907692307692306,0.923076923076922,0.938461538461537,0.953846153846152,
0.969230769230768,0.984615384615383,1.),.UNSPECIFIED.)
CURVE()
GEOMETRIC_REPRESENTATION_ITEM()
RATIONAL_B_SPLINE_CURVE((1.,1.,1.,1.,1.,1.,1.,1.,1.,1.,1.,1.,1.,1.,1.,1.,
1.,1.,1.,1.,1.,1.,1.,1.,1.,1.,1.,1.,1.,1.,1.,1.,1.,1.,1.,1.,1.,1.,1.,1.,
1.,1.,1.,1.,1.,1.,1.,1.,1.,1.,1.,1.,1.,1.,1.,1.,1.,1.,1.,1.,1.,1.,1.,1.,
1.,1.,1.,1.,1.,1.))
REPRESENTATION_ITEM('')
);
#228=(
BOUNDED_CURVE()
B_SPLINE_CURVE(5,(#31394,#31395,#31396,#31397,#31398,#31399,#31400,#31401,
#31402,#31403,#31404,#31405,#31406,#31407,#31408,#31409,#31410,#31411,#31412,
#31413,#31414,#31415,#31416,#31417,#31418,#31419,#31420,#31421,#31422,#31423,
#31424,#31425,#31426,#31427,#31428,#31429,#31430,#31431,#31432,#31433,#31434,
#31435,#31436,#31437,#31438,#31439,#31440,#31441,#31442,#31443,#31444,#31445,
#31446,#31447,#31448,#31449,#31450,#31451,#31452,#31453,#31454,#31455,#31456,
#31457,#31458,#31459,#31460,#31461,#31462,#31463),.UNSPECIFIED.,.F.,.F.)
B_SPLINE_CURVE_WITH_KNOTS((6,1,1,1,1,1,1,1,1,1,1,1,1,1,1,1,1,1,1,1,1,1,
1,1,1,1,1,1,1,1,1,1,1,1,1,1,1,1,1,1,1,1,1,1,1,1,1,1,1,1,1,1,1,1,1,1,1,1,
1,1,1,1,1,1,1,6),(0.,0.0153846153846154,0.0307692307692308,0.0461538461538462,
0.0615384615384615,0.0769230769230769,0.0923076923076923,0.107692307692308,
0.123076923076923,0.138461538461538,0.153846153846154,0.169230769230769,
0.184615384615385,0.2,0.215384615384615,0.230769230769231,0.246153846153846,
0.261538461538462,0.276923076923077,0.292307692307692,0.307692307692308,
0.323076923076923,0.338461538461538,0.353846153846154,0.369230769230769,
0.384615384615385,0.4,0.415384615384615,0.430769230769231,0.446153846153846,
0.461538461538462,0.476923076923077,0.492307692307692,0.507692307692308,
0.523076923076923,0.538461538461538,0.553846153846154,0.569230769230769,
0.584615384615384,0.6,0.615384615384615,0.63076923076923,0.646153846153846,
0.661538461538461,0.676923076923076,0.692307692307692,0.707692307692307,
0.723076923076922,0.738461538461538,0.753846153846153,0.769230769230768,
0.784615384615384,0.799999999999999,0.815384615384614,0.83076923076923,
0.846153846153845,0.86153846153846,0.876923076923076,0.892307692307691,
0.907692307692306,0.923076923076922,0.938461538461537,0.953846153846152,
0.969230769230768,0.984615384615383,0.994228156739704),.UNSPECIFIED.)
CURVE()
GEOMETRIC_REPRESENTATION_ITEM()
RATIONAL_B_SPLINE_CURVE((1.,1.,1.,1.,1.,1.,1.,1.,1.,1.,1.,1.,1.,1.,1.,1.,
1.,1.,1.,1.,1.,1.,1.,1.,1.,1.,1.,1.,1.,1.,1.,1.,1.,1.,1.,1.,1.,1.,1.,1.,
1.,1.,1.,1.,1.,1.,1.,1.,1.,1.,1.,1.,1.,1.,1.,1.,1.,1.,1.,1.,1.,1.,1.,1.,
1.,1.,1.,1.,1.,1.))
REPRESENTATION_ITEM('')
);
#229=(
BOUNDED_CURVE()
B_SPLINE_CURVE(5,(#31467,#31468,#31469,#31470,#31471,#31472,#31473,#31474,
#31475,#31476,#31477,#31478,#31479,#31480,#31481,#31482,#31483,#31484,#31485,
#31486,#31487,#31488,#31489,#31490,#31491,#31492,#31493,#31494,#31495,#31496,
#31497,#31498,#31499,#31500,#31501,#31502,#31503,#31504,#31505,#31506,#31507,
#31508,#31509,#31510,#31511,#31512,#31513,#31514,#31515,#31516,#31517,#31518,
#31519,#31520,#31521,#31522,#31523,#31524,#31525,#31526,#31527,#31528,#31529,
#31530,#31531,#31532,#31533,#31534,#31535,#31536),.UNSPECIFIED.,.F.,.F.)
B_SPLINE_CURVE_WITH_KNOTS((6,1,1,1,1,1,1,1,1,1,1,1,1,1,1,1,1,1,1,1,1,1,
1,1,1,1,1,1,1,1,1,1,1,1,1,1,1,1,1,1,1,1,1,1,1,1,1,1,1,1,1,1,1,1,1,1,1,1,
1,1,1,1,1,1,1,6),(0.00577184337449692,0.0153846153846154,0.0307692307692308,
0.0461538461538462,0.0615384615384615,0.0769230769230769,0.0923076923076923,
0.107692307692308,0.123076923076923,0.138461538461538,0.153846153846154,
0.169230769230769,0.184615384615385,0.2,0.215384615384615,0.230769230769231,
0.246153846153846,0.261538461538462,0.276923076923077,0.292307692307692,
0.307692307692308,0.323076923076923,0.338461538461538,0.353846153846154,
0.369230769230769,0.384615384615385,0.4,0.415384615384615,0.430769230769231,
0.446153846153846,0.461538461538462,0.476923076923077,0.492307692307692,
0.507692307692308,0.523076923076923,0.538461538461538,0.553846153846154,
0.569230769230769,0.584615384615384,0.6,0.615384615384615,0.63076923076923,
0.646153846153846,0.661538461538461,0.676923076923076,0.692307692307692,
0.707692307692307,0.723076923076922,0.738461538461538,0.753846153846153,
0.769230769230768,0.784615384615384,0.799999999999999,0.815384615384614,
0.83076923076923,0.846153846153845,0.86153846153846,0.876923076923076,0.892307692307691,
0.907692307692306,0.923076923076922,0.938461538461537,0.953846153846152,
0.969230769230768,0.984615384615383,1.),.UNSPECIFIED.)
CURVE()
GEOMETRIC_REPRESENTATION_ITEM()
RATIONAL_B_SPLINE_CURVE((1.,1.,1.,1.,1.,1.,1.,1.,1.,1.,1.,1.,1.,1.,1.,1.,
1.,1.,1.,1.,1.,1.,1.,1.,1.,1.,1.,1.,1.,1.,1.,1.,1.,1.,1.,1.,1.,1.,1.,1.,
1.,1.,1.,1.,1.,1.,1.,1.,1.,1.,1.,1.,1.,1.,1.,1.,1.,1.,1.,1.,1.,1.,1.,1.,
1.,1.,1.,1.,1.,1.))
REPRESENTATION_ITEM('')
);
#230=(
BOUNDED_CURVE()
B_SPLINE_CURVE(5,(#31540,#31541,#31542,#31543,#31544,#31545,#31546,#31547,
#31548,#31549,#31550,#31551,#31552,#31553,#31554,#31555,#31556,#31557,#31558,
#31559,#31560,#31561,#31562,#31563,#31564,#31565,#31566,#31567,#31568,#31569,
#31570,#31571,#31572,#31573,#31574,#31575,#31576,#31577,#31578,#31579,#31580,
#31581,#31582,#31583,#31584,#31585,#31586,#31587,#31588,#31589,#31590,#31591,
#31592,#31593,#31594,#31595,#31596,#31597,#31598,#31599,#31600,#31601,#31602,
#31603,#31604,#31605,#31606,#31607,#31608,#31609),.UNSPECIFIED.,.F.,.F.)
B_SPLINE_CURVE_WITH_KNOTS((6,1,1,1,1,1,1,1,1,1,1,1,1,1,1,1,1,1,1,1,1,1,
1,1,1,1,1,1,1,1,1,1,1,1,1,1,1,1,1,1,1,1,1,1,1,1,1,1,1,1,1,1,1,1,1,1,1,1,
1,1,1,1,1,1,1,6),(0.,0.0153846153846154,0.0307692307692308,0.0461538461538462,
0.0615384615384615,0.0769230769230769,0.0923076923076923,0.107692307692308,
0.123076923076923,0.138461538461538,0.153846153846154,0.169230769230769,
0.184615384615385,0.2,0.215384615384615,0.230769230769231,0.246153846153846,
0.261538461538462,0.276923076923077,0.292307692307692,0.307692307692308,
0.323076923076923,0.338461538461538,0.353846153846154,0.369230769230769,
0.384615384615385,0.4,0.415384615384615,0.430769230769231,0.446153846153846,
0.461538461538462,0.476923076923077,0.492307692307692,0.507692307692308,
0.523076923076923,0.538461538461538,0.553846153846154,0.569230769230769,
0.584615384615384,0.6,0.615384615384615,0.63076923076923,0.646153846153846,
0.661538461538461,0.676923076923076,0.692307692307692,0.707692307692307,
0.723076923076922,0.738461538461538,0.753846153846153,0.769230769230768,
0.784615384615384,0.799999999999999,0.815384615384614,0.83076923076923,
0.846153846153845,0.86153846153846,0.876923076923076,0.892307692307691,
0.907692307692306,0.923076923076922,0.938461538461537,0.953846153846152,
0.969230769230768,0.984615384615383,0.994228156739711),.UNSPECIFIED.)
CURVE()
GEOMETRIC_REPRESENTATION_ITEM()
RATIONAL_B_SPLINE_CURVE((1.,1.,1.,1.,1.,1.,1.,1.,1.,1.,1.,1.,1.,1.,1.,1.,
1.,1.,1.,1.,1.,1.,1.,1.,1.,1.,1.,1.,1.,1.,1.,1.,1.,1.,1.,1.,1.,1.,1.,1.,
1.,1.,1.,1.,1.,1.,1.,1.,1.,1.,1.,1.,1.,1.,1.,1.,1.,1.,1.,1.,1.,1.,1.,1.,
1.,1.,1.,1.,1.,1.))
REPRESENTATION_ITEM('')
);
#231=(
BOUNDED_CURVE()
B_SPLINE_CURVE(5,(#31613,#31614,#31615,#31616,#31617,#31618,#31619,#31620,
#31621,#31622,#31623,#31624,#31625,#31626,#31627,#31628,#31629,#31630,#31631,
#31632,#31633,#31634,#31635,#31636,#31637,#31638,#31639,#31640,#31641,#31642,
#31643,#31644,#31645,#31646,#31647,#31648,#31649,#31650,#31651,#31652,#31653,
#31654,#31655,#31656,#31657,#31658,#31659,#31660,#31661,#31662,#31663,#31664,
#31665,#31666,#31667,#31668,#31669,#31670,#31671,#31672,#31673,#31674,#31675,
#31676,#31677,#31678,#31679,#31680,#31681,#31682),.UNSPECIFIED.,.F.,.F.)
B_SPLINE_CURVE_WITH_KNOTS((6,1,1,1,1,1,1,1,1,1,1,1,1,1,1,1,1,1,1,1,1,1,
1,1,1,1,1,1,1,1,1,1,1,1,1,1,1,1,1,1,1,1,1,1,1,1,1,1,1,1,1,1,1,1,1,1,1,1,
1,1,1,1,1,1,1,6),(0.00577184337450058,0.0153846153846154,0.0307692307692308,
0.0461538461538462,0.0615384615384615,0.0769230769230769,0.0923076923076923,
0.107692307692308,0.123076923076923,0.138461538461538,0.153846153846154,
0.169230769230769,0.184615384615385,0.2,0.215384615384615,0.230769230769231,
0.246153846153846,0.261538461538462,0.276923076923077,0.292307692307692,
0.307692307692308,0.323076923076923,0.338461538461538,0.353846153846154,
0.369230769230769,0.384615384615385,0.4,0.415384615384615,0.430769230769231,
0.446153846153846,0.461538461538462,0.476923076923077,0.492307692307692,
0.507692307692308,0.523076923076923,0.538461538461538,0.553846153846154,
0.569230769230769,0.584615384615384,0.6,0.615384615384615,0.63076923076923,
0.646153846153846,0.661538461538461,0.676923076923076,0.692307692307692,
0.707692307692307,0.723076923076922,0.738461538461538,0.753846153846153,
0.769230769230768,0.784615384615384,0.799999999999999,0.815384615384614,
0.83076923076923,0.846153846153845,0.86153846153846,0.876923076923076,0.892307692307691,
0.907692307692306,0.923076923076922,0.938461538461537,0.953846153846152,
0.969230769230768,0.984615384615383,1.),.UNSPECIFIED.)
CURVE()
GEOMETRIC_REPRESENTATION_ITEM()
RATIONAL_B_SPLINE_CURVE((1.,1.,1.,1.,1.,1.,1.,1.,1.,1.,1.,1.,1.,1.,1.,1.,
1.,1.,1.,1.,1.,1.,1.,1.,1.,1.,1.,1.,1.,1.,1.,1.,1.,1.,1.,1.,1.,1.,1.,1.,
1.,1.,1.,1.,1.,1.,1.,1.,1.,1.,1.,1.,1.,1.,1.,1.,1.,1.,1.,1.,1.,1.,1.,1.,
1.,1.,1.,1.,1.,1.))
REPRESENTATION_ITEM('')
);
#232=(
BOUNDED_CURVE()
B_SPLINE_CURVE(5,(#31686,#31687,#31688,#31689,#31690,#31691,#31692,#31693,
#31694,#31695,#31696,#31697,#31698,#31699,#31700,#31701,#31702,#31703,#31704,
#31705,#31706,#31707,#31708,#31709,#31710,#31711,#31712,#31713,#31714,#31715,
#31716,#31717,#31718,#31719,#31720,#31721,#31722,#31723,#31724,#31725,#31726,
#31727,#31728,#31729,#31730,#31731,#31732,#31733,#31734,#31735,#31736,#31737,
#31738,#31739,#31740,#31741,#31742,#31743,#31744,#31745,#31746,#31747,#31748,
#31749,#31750,#31751,#31752,#31753,#31754,#31755),.UNSPECIFIED.,.F.,.F.)
B_SPLINE_CURVE_WITH_KNOTS((6,1,1,1,1,1,1,1,1,1,1,1,1,1,1,1,1,1,1,1,1,1,
1,1,1,1,1,1,1,1,1,1,1,1,1,1,1,1,1,1,1,1,1,1,1,1,1,1,1,1,1,1,1,1,1,1,1,1,
1,1,1,1,1,1,1,6),(0.,0.0153846153846154,0.0307692307692308,0.0461538461538462,
0.0615384615384615,0.0769230769230769,0.0923076923076923,0.107692307692308,
0.123076923076923,0.138461538461538,0.153846153846154,0.169230769230769,
0.184615384615385,0.2,0.215384615384615,0.230769230769231,0.246153846153846,
0.261538461538462,0.276923076923077,0.292307692307692,0.307692307692308,
0.323076923076923,0.338461538461538,0.353846153846154,0.369230769230769,
0.384615384615385,0.4,0.415384615384615,0.430769230769231,0.446153846153846,
0.461538461538462,0.476923076923077,0.492307692307692,0.507692307692308,
0.523076923076923,0.538461538461538,0.553846153846154,0.569230769230769,
0.584615384615384,0.6,0.615384615384615,0.63076923076923,0.646153846153846,
0.661538461538461,0.676923076923076,0.692307692307692,0.707692307692307,
0.723076923076922,0.738461538461538,0.753846153846153,0.769230769230768,
0.784615384615384,0.799999999999999,0.815384615384614,0.83076923076923,
0.846153846153845,0.86153846153846,0.876923076923076,0.892307692307691,
0.907692307692306,0.923076923076922,0.938461538461537,0.953846153846152,
0.969230769230768,0.984615384615383,0.994228156739701),.UNSPECIFIED.)
CURVE()
GEOMETRIC_REPRESENTATION_ITEM()
RATIONAL_B_SPLINE_CURVE((1.,1.,1.,1.,1.,1.,1.,1.,1.,1.,1.,1.,1.,1.,1.,1.,
1.,1.,1.,1.,1.,1.,1.,1.,1.,1.,1.,1.,1.,1.,1.,1.,1.,1.,1.,1.,1.,1.,1.,1.,
1.,1.,1.,1.,1.,1.,1.,1.,1.,1.,1.,1.,1.,1.,1.,1.,1.,1.,1.,1.,1.,1.,1.,1.,
1.,1.,1.,1.,1.,1.))
REPRESENTATION_ITEM('')
);
#233=(
BOUNDED_CURVE()
B_SPLINE_CURVE(5,(#31759,#31760,#31761,#31762,#31763,#31764,#31765,#31766,
#31767,#31768,#31769,#31770,#31771,#31772,#31773,#31774,#31775,#31776,#31777,
#31778,#31779,#31780,#31781,#31782,#31783,#31784,#31785,#31786,#31787,#31788,
#31789,#31790,#31791,#31792,#31793,#31794,#31795,#31796,#31797,#31798,#31799,
#31800,#31801,#31802,#31803,#31804,#31805,#31806,#31807,#31808,#31809,#31810,
#31811,#31812,#31813,#31814,#31815,#31816,#31817,#31818,#31819,#31820,#31821,
#31822,#31823,#31824,#31825,#31826,#31827,#31828),.UNSPECIFIED.,.F.,.F.)
B_SPLINE_CURVE_WITH_KNOTS((6,1,1,1,1,1,1,1,1,1,1,1,1,1,1,1,1,1,1,1,1,1,
1,1,1,1,1,1,1,1,1,1,1,1,1,1,1,1,1,1,1,1,1,1,1,1,1,1,1,1,1,1,1,1,1,1,1,1,
1,1,1,1,1,1,1,6),(0.0057718433745091,0.0153846153846154,0.0307692307692308,
0.0461538461538462,0.0615384615384615,0.0769230769230769,0.0923076923076923,
0.107692307692308,0.123076923076923,0.138461538461538,0.153846153846154,
0.169230769230769,0.184615384615385,0.2,0.215384615384615,0.230769230769231,
0.246153846153846,0.261538461538462,0.276923076923077,0.292307692307692,
0.307692307692308,0.323076923076923,0.338461538461538,0.353846153846154,
0.369230769230769,0.384615384615385,0.4,0.415384615384615,0.430769230769231,
0.446153846153846,0.461538461538462,0.476923076923077,0.492307692307692,
0.507692307692308,0.523076923076923,0.538461538461538,0.553846153846154,
0.569230769230769,0.584615384615384,0.6,0.615384615384615,0.63076923076923,
0.646153846153846,0.661538461538461,0.676923076923076,0.692307692307692,
0.707692307692307,0.723076923076922,0.738461538461538,0.753846153846153,
0.769230769230768,0.784615384615384,0.799999999999999,0.815384615384614,
0.83076923076923,0.846153846153845,0.86153846153846,0.876923076923076,0.892307692307691,
0.907692307692306,0.923076923076922,0.938461538461537,0.953846153846152,
0.969230769230768,0.984615384615383,1.),.UNSPECIFIED.)
CURVE()
GEOMETRIC_REPRESENTATION_ITEM()
RATIONAL_B_SPLINE_CURVE((1.,1.,1.,1.,1.,1.,1.,1.,1.,1.,1.,1.,1.,1.,1.,1.,
1.,1.,1.,1.,1.,1.,1.,1.,1.,1.,1.,1.,1.,1.,1.,1.,1.,1.,1.,1.,1.,1.,1.,1.,
1.,1.,1.,1.,1.,1.,1.,1.,1.,1.,1.,1.,1.,1.,1.,1.,1.,1.,1.,1.,1.,1.,1.,1.,
1.,1.,1.,1.,1.,1.))
REPRESENTATION_ITEM('')
);
#234=(
BOUNDED_CURVE()
B_SPLINE_CURVE(5,(#31832,#31833,#31834,#31835,#31836,#31837,#31838,#31839,
#31840,#31841,#31842,#31843,#31844,#31845,#31846,#31847,#31848,#31849,#31850,
#31851,#31852,#31853,#31854,#31855,#31856,#31857,#31858,#31859,#31860,#31861,
#31862,#31863,#31864,#31865,#31866,#31867,#31868,#31869,#31870,#31871,#31872,
#31873,#31874,#31875,#31876,#31877,#31878,#31879,#31880,#31881,#31882,#31883,
#31884,#31885,#31886,#31887,#31888,#31889,#31890,#31891,#31892,#31893,#31894,
#31895,#31896,#31897,#31898,#31899,#31900,#31901),.UNSPECIFIED.,.F.,.F.)
B_SPLINE_CURVE_WITH_KNOTS((6,1,1,1,1,1,1,1,1,1,1,1,1,1,1,1,1,1,1,1,1,1,
1,1,1,1,1,1,1,1,1,1,1,1,1,1,1,1,1,1,1,1,1,1,1,1,1,1,1,1,1,1,1,1,1,1,1,1,
1,1,1,1,1,1,1,6),(0.,0.0153846153846154,0.0307692307692308,0.0461538461538462,
0.0615384615384615,0.0769230769230769,0.0923076923076923,0.107692307692308,
0.123076923076923,0.138461538461538,0.153846153846154,0.169230769230769,
0.184615384615385,0.2,0.215384615384615,0.230769230769231,0.246153846153846,
0.261538461538462,0.276923076923077,0.292307692307692,0.307692307692308,
0.323076923076923,0.338461538461538,0.353846153846154,0.369230769230769,
0.384615384615385,0.4,0.415384615384615,0.430769230769231,0.446153846153846,
0.461538461538462,0.476923076923077,0.492307692307692,0.507692307692308,
0.523076923076923,0.538461538461538,0.553846153846154,0.569230769230769,
0.584615384615384,0.6,0.615384615384615,0.63076923076923,0.646153846153846,
0.661538461538461,0.676923076923076,0.692307692307692,0.707692307692307,
0.723076923076922,0.738461538461538,0.753846153846153,0.769230769230768,
0.784615384615384,0.799999999999999,0.815384615384614,0.83076923076923,
0.846153846153845,0.86153846153846,0.876923076923076,0.892307692307691,
0.907692307692306,0.923076923076922,0.938461538461537,0.953846153846152,
0.969230769230768,0.984615384615383,0.994228156739689),.UNSPECIFIED.)
CURVE()
GEOMETRIC_REPRESENTATION_ITEM()
RATIONAL_B_SPLINE_CURVE((1.,1.,1.,1.,1.,1.,1.,1.,1.,1.,1.,1.,1.,1.,1.,1.,
1.,1.,1.,1.,1.,1.,1.,1.,1.,1.,1.,1.,1.,1.,1.,1.,1.,1.,1.,1.,1.,1.,1.,1.,
1.,1.,1.,1.,1.,1.,1.,1.,1.,1.,1.,1.,1.,1.,1.,1.,1.,1.,1.,1.,1.,1.,1.,1.,
1.,1.,1.,1.,1.,1.))
REPRESENTATION_ITEM('')
);
#235=(
BOUNDED_CURVE()
B_SPLINE_CURVE(5,(#31905,#31906,#31907,#31908,#31909,#31910,#31911,#31912,
#31913,#31914,#31915,#31916,#31917,#31918,#31919,#31920,#31921,#31922,#31923,
#31924,#31925,#31926,#31927,#31928,#31929,#31930,#31931,#31932,#31933,#31934,
#31935,#31936,#31937,#31938,#31939,#31940,#31941,#31942,#31943,#31944,#31945,
#31946,#31947,#31948,#31949,#31950,#31951,#31952,#31953,#31954,#31955,#31956,
#31957,#31958,#31959,#31960,#31961,#31962,#31963,#31964,#31965,#31966,#31967,
#31968,#31969,#31970,#31971,#31972,#31973,#31974),.UNSPECIFIED.,.F.,.F.)
B_SPLINE_CURVE_WITH_KNOTS((6,1,1,1,1,1,1,1,1,1,1,1,1,1,1,1,1,1,1,1,1,1,
1,1,1,1,1,1,1,1,1,1,1,1,1,1,1,1,1,1,1,1,1,1,1,1,1,1,1,1,1,1,1,1,1,1,1,1,
1,1,1,1,1,1,1,6),(0.00577184337450777,0.0153846153846154,0.0307692307692308,
0.0461538461538462,0.0615384615384615,0.0769230769230769,0.0923076923076923,
0.107692307692308,0.123076923076923,0.138461538461538,0.153846153846154,
0.169230769230769,0.184615384615385,0.2,0.215384615384615,0.230769230769231,
0.246153846153846,0.261538461538462,0.276923076923077,0.292307692307692,
0.307692307692308,0.323076923076923,0.338461538461538,0.353846153846154,
0.369230769230769,0.384615384615385,0.4,0.415384615384615,0.430769230769231,
0.446153846153846,0.461538461538462,0.476923076923077,0.492307692307692,
0.507692307692308,0.523076923076923,0.538461538461538,0.553846153846154,
0.569230769230769,0.584615384615384,0.6,0.615384615384615,0.63076923076923,
0.646153846153846,0.661538461538461,0.676923076923076,0.692307692307692,
0.707692307692307,0.723076923076922,0.738461538461538,0.753846153846153,
0.769230769230768,0.784615384615384,0.799999999999999,0.815384615384614,
0.83076923076923,0.846153846153845,0.86153846153846,0.876923076923076,0.892307692307691,
0.907692307692306,0.923076923076922,0.938461538461537,0.953846153846152,
0.969230769230768,0.984615384615383,1.),.UNSPECIFIED.)
CURVE()
GEOMETRIC_REPRESENTATION_ITEM()
RATIONAL_B_SPLINE_CURVE((1.,1.,1.,1.,1.,1.,1.,1.,1.,1.,1.,1.,1.,1.,1.,1.,
1.,1.,1.,1.,1.,1.,1.,1.,1.,1.,1.,1.,1.,1.,1.,1.,1.,1.,1.,1.,1.,1.,1.,1.,
1.,1.,1.,1.,1.,1.,1.,1.,1.,1.,1.,1.,1.,1.,1.,1.,1.,1.,1.,1.,1.,1.,1.,1.,
1.,1.,1.,1.,1.,1.))
REPRESENTATION_ITEM('')
);
#236=(
BOUNDED_CURVE()
B_SPLINE_CURVE(5,(#31978,#31979,#31980,#31981,#31982,#31983,#31984,#31985,
#31986,#31987,#31988,#31989,#31990,#31991,#31992,#31993,#31994,#31995,#31996,
#31997,#31998,#31999,#32000,#32001,#32002,#32003,#32004,#32005,#32006,#32007,
#32008,#32009,#32010,#32011,#32012,#32013,#32014,#32015,#32016,#32017,#32018,
#32019,#32020,#32021,#32022,#32023,#32024,#32025,#32026,#32027,#32028,#32029,
#32030,#32031,#32032,#32033,#32034,#32035,#32036,#32037,#32038,#32039,#32040,
#32041,#32042,#32043,#32044,#32045,#32046,#32047),.UNSPECIFIED.,.F.,.F.)
B_SPLINE_CURVE_WITH_KNOTS((6,1,1,1,1,1,1,1,1,1,1,1,1,1,1,1,1,1,1,1,1,1,
1,1,1,1,1,1,1,1,1,1,1,1,1,1,1,1,1,1,1,1,1,1,1,1,1,1,1,1,1,1,1,1,1,1,1,1,
1,1,1,1,1,1,1,6),(0.,0.0153846153846154,0.0307692307692308,0.0461538461538462,
0.0615384615384615,0.0769230769230769,0.0923076923076923,0.107692307692308,
0.123076923076923,0.138461538461538,0.153846153846154,0.169230769230769,
0.184615384615385,0.2,0.215384615384615,0.230769230769231,0.246153846153846,
0.261538461538462,0.276923076923077,0.292307692307692,0.307692307692308,
0.323076923076923,0.338461538461538,0.353846153846154,0.369230769230769,
0.384615384615385,0.4,0.415384615384615,0.430769230769231,0.446153846153846,
0.461538461538462,0.476923076923077,0.492307692307692,0.507692307692308,
0.523076923076923,0.538461538461538,0.553846153846154,0.569230769230769,
0.584615384615384,0.6,0.615384615384615,0.63076923076923,0.646153846153846,
0.661538461538461,0.676923076923076,0.692307692307692,0.707692307692307,
0.723076923076922,0.738461538461538,0.753846153846153,0.769230769230768,
0.784615384615384,0.799999999999999,0.815384615384614,0.83076923076923,
0.846153846153845,0.86153846153846,0.876923076923076,0.892307692307691,
0.907692307692306,0.923076923076922,0.938461538461537,0.953846153846152,
0.969230769230768,0.984615384615383,0.994228156739701),.UNSPECIFIED.)
CURVE()
GEOMETRIC_REPRESENTATION_ITEM()
RATIONAL_B_SPLINE_CURVE((1.,1.,1.,1.,1.,1.,1.,1.,1.,1.,1.,1.,1.,1.,1.,1.,
1.,1.,1.,1.,1.,1.,1.,1.,1.,1.,1.,1.,1.,1.,1.,1.,1.,1.,1.,1.,1.,1.,1.,1.,
1.,1.,1.,1.,1.,1.,1.,1.,1.,1.,1.,1.,1.,1.,1.,1.,1.,1.,1.,1.,1.,1.,1.,1.,
1.,1.,1.,1.,1.,1.))
REPRESENTATION_ITEM('')
);
#237=(
BOUNDED_CURVE()
B_SPLINE_CURVE(5,(#32051,#32052,#32053,#32054,#32055,#32056,#32057,#32058,
#32059,#32060,#32061,#32062,#32063,#32064,#32065,#32066,#32067,#32068,#32069,
#32070,#32071,#32072,#32073,#32074,#32075,#32076,#32077,#32078,#32079,#32080,
#32081,#32082,#32083,#32084,#32085,#32086,#32087,#32088,#32089,#32090,#32091,
#32092,#32093,#32094,#32095,#32096,#32097,#32098,#32099,#32100,#32101,#32102,
#32103,#32104,#32105,#32106,#32107,#32108,#32109,#32110,#32111,#32112,#32113,
#32114,#32115,#32116,#32117,#32118,#32119,#32120),.UNSPECIFIED.,.F.,.F.)
B_SPLINE_CURVE_WITH_KNOTS((6,1,1,1,1,1,1,1,1,1,1,1,1,1,1,1,1,1,1,1,1,1,
1,1,1,1,1,1,1,1,1,1,1,1,1,1,1,1,1,1,1,1,1,1,1,1,1,1,1,1,1,1,1,1,1,1,1,1,
1,1,1,1,1,1,1,6),(0.00577184337450172,0.0153846153846154,0.0307692307692308,
0.0461538461538462,0.0615384615384615,0.0769230769230769,0.0923076923076923,
0.107692307692308,0.123076923076923,0.138461538461538,0.153846153846154,
0.169230769230769,0.184615384615385,0.2,0.215384615384615,0.230769230769231,
0.246153846153846,0.261538461538462,0.276923076923077,0.292307692307692,
0.307692307692308,0.323076923076923,0.338461538461538,0.353846153846154,
0.369230769230769,0.384615384615385,0.4,0.415384615384615,0.430769230769231,
0.446153846153846,0.461538461538462,0.476923076923077,0.492307692307692,
0.507692307692308,0.523076923076923,0.538461538461538,0.553846153846154,
0.569230769230769,0.584615384615384,0.6,0.615384615384615,0.63076923076923,
0.646153846153846,0.661538461538461,0.676923076923076,0.692307692307692,
0.707692307692307,0.723076923076922,0.738461538461538,0.753846153846153,
0.769230769230768,0.784615384615384,0.799999999999999,0.815384615384614,
0.83076923076923,0.846153846153845,0.86153846153846,0.876923076923076,0.892307692307691,
0.907692307692306,0.923076923076922,0.938461538461537,0.953846153846152,
0.969230769230768,0.984615384615383,1.),.UNSPECIFIED.)
CURVE()
GEOMETRIC_REPRESENTATION_ITEM()
RATIONAL_B_SPLINE_CURVE((1.,1.,1.,1.,1.,1.,1.,1.,1.,1.,1.,1.,1.,1.,1.,1.,
1.,1.,1.,1.,1.,1.,1.,1.,1.,1.,1.,1.,1.,1.,1.,1.,1.,1.,1.,1.,1.,1.,1.,1.,
1.,1.,1.,1.,1.,1.,1.,1.,1.,1.,1.,1.,1.,1.,1.,1.,1.,1.,1.,1.,1.,1.,1.,1.,
1.,1.,1.,1.,1.,1.))
REPRESENTATION_ITEM('')
);
#238=(
BOUNDED_CURVE()
B_SPLINE_CURVE(5,(#32124,#32125,#32126,#32127,#32128,#32129,#32130,#32131,
#32132,#32133,#32134,#32135,#32136,#32137,#32138,#32139,#32140,#32141,#32142,
#32143,#32144,#32145,#32146,#32147,#32148,#32149,#32150,#32151,#32152,#32153,
#32154,#32155,#32156,#32157,#32158,#32159,#32160,#32161,#32162,#32163,#32164,
#32165,#32166,#32167,#32168,#32169,#32170,#32171,#32172,#32173,#32174,#32175,
#32176,#32177,#32178,#32179,#32180,#32181,#32182,#32183,#32184,#32185,#32186,
#32187,#32188,#32189,#32190,#32191,#32192,#32193),.UNSPECIFIED.,.F.,.F.)
B_SPLINE_CURVE_WITH_KNOTS((6,1,1,1,1,1,1,1,1,1,1,1,1,1,1,1,1,1,1,1,1,1,
1,1,1,1,1,1,1,1,1,1,1,1,1,1,1,1,1,1,1,1,1,1,1,1,1,1,1,1,1,1,1,1,1,1,1,1,
1,1,1,1,1,1,1,6),(0.,0.0153846153846154,0.0307692307692308,0.0461538461538462,
0.0615384615384615,0.0769230769230769,0.0923076923076923,0.107692307692308,
0.123076923076923,0.138461538461538,0.153846153846154,0.169230769230769,
0.184615384615385,0.2,0.215384615384615,0.230769230769231,0.246153846153846,
0.261538461538462,0.276923076923077,0.292307692307692,0.307692307692308,
0.323076923076923,0.338461538461538,0.353846153846154,0.369230769230769,
0.384615384615385,0.4,0.415384615384615,0.430769230769231,0.446153846153846,
0.461538461538462,0.476923076923077,0.492307692307692,0.507692307692308,
0.523076923076923,0.538461538461538,0.553846153846154,0.569230769230769,
0.584615384615384,0.6,0.615384615384615,0.63076923076923,0.646153846153846,
0.661538461538461,0.676923076923076,0.692307692307692,0.707692307692307,
0.723076923076922,0.738461538461538,0.753846153846153,0.769230769230768,
0.784615384615384,0.799999999999999,0.815384615384614,0.83076923076923,
0.846153846153845,0.86153846153846,0.876923076923076,0.892307692307691,
0.907692307692306,0.923076923076922,0.938461538461537,0.953846153846152,
0.969230769230768,0.984615384615383,0.99422815673971),.UNSPECIFIED.)
CURVE()
GEOMETRIC_REPRESENTATION_ITEM()
RATIONAL_B_SPLINE_CURVE((1.,1.,1.,1.,1.,1.,1.,1.,1.,1.,1.,1.,1.,1.,1.,1.,
1.,1.,1.,1.,1.,1.,1.,1.,1.,1.,1.,1.,1.,1.,1.,1.,1.,1.,1.,1.,1.,1.,1.,1.,
1.,1.,1.,1.,1.,1.,1.,1.,1.,1.,1.,1.,1.,1.,1.,1.,1.,1.,1.,1.,1.,1.,1.,1.,
1.,1.,1.,1.,1.,1.))
REPRESENTATION_ITEM('')
);
#239=(
BOUNDED_CURVE()
B_SPLINE_CURVE(5,(#32197,#32198,#32199,#32200,#32201,#32202,#32203,#32204,
#32205,#32206,#32207,#32208,#32209,#32210,#32211,#32212,#32213,#32214,#32215,
#32216,#32217,#32218,#32219,#32220,#32221,#32222,#32223,#32224,#32225,#32226,
#32227,#32228,#32229,#32230,#32231,#32232,#32233,#32234,#32235,#32236,#32237,
#32238,#32239,#32240,#32241,#32242,#32243,#32244,#32245,#32246,#32247,#32248,
#32249,#32250,#32251,#32252,#32253,#32254,#32255,#32256,#32257,#32258,#32259,
#32260,#32261,#32262,#32263,#32264,#32265,#32266),.UNSPECIFIED.,.F.,.F.)
B_SPLINE_CURVE_WITH_KNOTS((6,1,1,1,1,1,1,1,1,1,1,1,1,1,1,1,1,1,1,1,1,1,
1,1,1,1,1,1,1,1,1,1,1,1,1,1,1,1,1,1,1,1,1,1,1,1,1,1,1,1,1,1,1,1,1,1,1,1,
1,1,1,1,1,1,1,6),(0.00577184337448657,0.0153846153846154,0.0307692307692308,
0.0461538461538462,0.0615384615384615,0.0769230769230769,0.0923076923076923,
0.107692307692308,0.123076923076923,0.138461538461538,0.153846153846154,
0.169230769230769,0.184615384615385,0.2,0.215384615384615,0.230769230769231,
0.246153846153846,0.261538461538462,0.276923076923077,0.292307692307692,
0.307692307692308,0.323076923076923,0.338461538461538,0.353846153846154,
0.369230769230769,0.384615384615385,0.4,0.415384615384615,0.430769230769231,
0.446153846153846,0.461538461538462,0.476923076923077,0.492307692307692,
0.507692307692308,0.523076923076923,0.538461538461538,0.553846153846154,
0.569230769230769,0.584615384615384,0.6,0.615384615384615,0.63076923076923,
0.646153846153846,0.661538461538461,0.676923076923076,0.692307692307692,
0.707692307692307,0.723076923076922,0.738461538461538,0.753846153846153,
0.769230769230768,0.784615384615384,0.799999999999999,0.815384615384614,
0.83076923076923,0.846153846153845,0.86153846153846,0.876923076923076,0.892307692307691,
0.907692307692306,0.923076923076922,0.938461538461537,0.953846153846152,
0.969230769230768,0.984615384615383,1.),.UNSPECIFIED.)
CURVE()
GEOMETRIC_REPRESENTATION_ITEM()
RATIONAL_B_SPLINE_CURVE((1.,1.,1.,1.,1.,1.,1.,1.,1.,1.,1.,1.,1.,1.,1.,1.,
1.,1.,1.,1.,1.,1.,1.,1.,1.,1.,1.,1.,1.,1.,1.,1.,1.,1.,1.,1.,1.,1.,1.,1.,
1.,1.,1.,1.,1.,1.,1.,1.,1.,1.,1.,1.,1.,1.,1.,1.,1.,1.,1.,1.,1.,1.,1.,1.,
1.,1.,1.,1.,1.,1.))
REPRESENTATION_ITEM('')
);
#240=(
BOUNDED_CURVE()
B_SPLINE_CURVE(5,(#32270,#32271,#32272,#32273,#32274,#32275,#32276,#32277,
#32278,#32279,#32280,#32281,#32282,#32283,#32284,#32285,#32286,#32287,#32288,
#32289,#32290,#32291,#32292,#32293,#32294,#32295,#32296,#32297,#32298,#32299,
#32300,#32301,#32302,#32303,#32304,#32305,#32306,#32307,#32308,#32309,#32310,
#32311,#32312,#32313,#32314,#32315,#32316,#32317,#32318,#32319,#32320,#32321,
#32322,#32323,#32324,#32325,#32326,#32327,#32328,#32329,#32330,#32331,#32332,
#32333,#32334,#32335,#32336,#32337,#32338,#32339),.UNSPECIFIED.,.F.,.F.)
B_SPLINE_CURVE_WITH_KNOTS((6,1,1,1,1,1,1,1,1,1,1,1,1,1,1,1,1,1,1,1,1,1,
1,1,1,1,1,1,1,1,1,1,1,1,1,1,1,1,1,1,1,1,1,1,1,1,1,1,1,1,1,1,1,1,1,1,1,1,
1,1,1,1,1,1,1,6),(0.,0.0153846153846154,0.0307692307692308,0.0461538461538462,
0.0615384615384615,0.0769230769230769,0.0923076923076923,0.107692307692308,
0.123076923076923,0.138461538461538,0.153846153846154,0.169230769230769,
0.184615384615385,0.2,0.215384615384615,0.230769230769231,0.246153846153846,
0.261538461538462,0.276923076923077,0.292307692307692,0.307692307692308,
0.323076923076923,0.338461538461538,0.353846153846154,0.369230769230769,
0.384615384615385,0.4,0.415384615384615,0.430769230769231,0.446153846153846,
0.461538461538462,0.476923076923077,0.492307692307692,0.507692307692308,
0.523076923076923,0.538461538461538,0.553846153846154,0.569230769230769,
0.584615384615384,0.6,0.615384615384615,0.63076923076923,0.646153846153846,
0.661538461538461,0.676923076923076,0.692307692307692,0.707692307692307,
0.723076923076922,0.738461538461538,0.753846153846153,0.769230769230768,
0.784615384615384,0.799999999999999,0.815384615384614,0.83076923076923,
0.846153846153845,0.86153846153846,0.876923076923076,0.892307692307691,
0.907692307692306,0.923076923076922,0.938461538461537,0.953846153846152,
0.969230769230768,0.984615384615383,0.994228156739709),.UNSPECIFIED.)
CURVE()
GEOMETRIC_REPRESENTATION_ITEM()
RATIONAL_B_SPLINE_CURVE((1.,1.,1.,1.,1.,1.,1.,1.,1.,1.,1.,1.,1.,1.,1.,1.,
1.,1.,1.,1.,1.,1.,1.,1.,1.,1.,1.,1.,1.,1.,1.,1.,1.,1.,1.,1.,1.,1.,1.,1.,
1.,1.,1.,1.,1.,1.,1.,1.,1.,1.,1.,1.,1.,1.,1.,1.,1.,1.,1.,1.,1.,1.,1.,1.,
1.,1.,1.,1.,1.,1.))
REPRESENTATION_ITEM('')
);
#241=(
BOUNDED_CURVE()
B_SPLINE_CURVE(5,(#32343,#32344,#32345,#32346,#32347,#32348,#32349,#32350,
#32351,#32352,#32353,#32354,#32355,#32356,#32357,#32358,#32359,#32360,#32361,
#32362,#32363,#32364,#32365,#32366,#32367,#32368,#32369,#32370,#32371,#32372,
#32373,#32374,#32375,#32376,#32377,#32378,#32379,#32380,#32381,#32382,#32383,
#32384,#32385,#32386,#32387,#32388,#32389,#32390,#32391,#32392,#32393,#32394,
#32395,#32396,#32397,#32398,#32399,#32400,#32401,#32402,#32403,#32404,#32405,
#32406,#32407,#32408,#32409,#32410,#32411,#32412),.UNSPECIFIED.,.F.,.F.)
B_SPLINE_CURVE_WITH_KNOTS((6,1,1,1,1,1,1,1,1,1,1,1,1,1,1,1,1,1,1,1,1,1,
1,1,1,1,1,1,1,1,1,1,1,1,1,1,1,1,1,1,1,1,1,1,1,1,1,1,1,1,1,1,1,1,1,1,1,1,
1,1,1,1,1,1,1,6),(0.00577184337451094,0.0153846153846154,0.0307692307692308,
0.0461538461538462,0.0615384615384615,0.0769230769230769,0.0923076923076923,
0.107692307692308,0.123076923076923,0.138461538461538,0.153846153846154,
0.169230769230769,0.184615384615385,0.2,0.215384615384615,0.230769230769231,
0.246153846153846,0.261538461538462,0.276923076923077,0.292307692307692,
0.307692307692308,0.323076923076923,0.338461538461538,0.353846153846154,
0.369230769230769,0.384615384615385,0.4,0.415384615384615,0.430769230769231,
0.446153846153846,0.461538461538462,0.476923076923077,0.492307692307692,
0.507692307692308,0.523076923076923,0.538461538461538,0.553846153846154,
0.569230769230769,0.584615384615384,0.6,0.615384615384615,0.63076923076923,
0.646153846153846,0.661538461538461,0.676923076923076,0.692307692307692,
0.707692307692307,0.723076923076922,0.738461538461538,0.753846153846153,
0.769230769230768,0.784615384615384,0.799999999999999,0.815384615384614,
0.83076923076923,0.846153846153845,0.86153846153846,0.876923076923076,0.892307692307691,
0.907692307692306,0.923076923076922,0.938461538461537,0.953846153846152,
0.969230769230768,0.984615384615383,1.),.UNSPECIFIED.)
CURVE()
GEOMETRIC_REPRESENTATION_ITEM()
RATIONAL_B_SPLINE_CURVE((1.,1.,1.,1.,1.,1.,1.,1.,1.,1.,1.,1.,1.,1.,1.,1.,
1.,1.,1.,1.,1.,1.,1.,1.,1.,1.,1.,1.,1.,1.,1.,1.,1.,1.,1.,1.,1.,1.,1.,1.,
1.,1.,1.,1.,1.,1.,1.,1.,1.,1.,1.,1.,1.,1.,1.,1.,1.,1.,1.,1.,1.,1.,1.,1.,
1.,1.,1.,1.,1.,1.))
REPRESENTATION_ITEM('')
);
#242=(
BOUNDED_CURVE()
B_SPLINE_CURVE(5,(#32416,#32417,#32418,#32419,#32420,#32421,#32422,#32423,
#32424,#32425,#32426,#32427,#32428,#32429,#32430,#32431,#32432,#32433,#32434,
#32435,#32436,#32437,#32438,#32439,#32440,#32441,#32442,#32443,#32444,#32445,
#32446,#32447,#32448,#32449,#32450,#32451,#32452,#32453,#32454,#32455,#32456,
#32457,#32458,#32459,#32460,#32461,#32462,#32463,#32464,#32465,#32466,#32467,
#32468,#32469,#32470,#32471,#32472,#32473,#32474,#32475,#32476,#32477,#32478,
#32479,#32480,#32481,#32482,#32483,#32484,#32485),.UNSPECIFIED.,.F.,.F.)
B_SPLINE_CURVE_WITH_KNOTS((6,1,1,1,1,1,1,1,1,1,1,1,1,1,1,1,1,1,1,1,1,1,
1,1,1,1,1,1,1,1,1,1,1,1,1,1,1,1,1,1,1,1,1,1,1,1,1,1,1,1,1,1,1,1,1,1,1,1,
1,1,1,1,1,1,1,6),(0.,0.0153846153846154,0.0307692307692308,0.0461538461538462,
0.0615384615384615,0.0769230769230769,0.0923076923076923,0.107692307692308,
0.123076923076923,0.138461538461538,0.153846153846154,0.169230769230769,
0.184615384615385,0.2,0.215384615384615,0.230769230769231,0.246153846153846,
0.261538461538462,0.276923076923077,0.292307692307692,0.307692307692308,
0.323076923076923,0.338461538461538,0.353846153846154,0.369230769230769,
0.384615384615385,0.4,0.415384615384615,0.430769230769231,0.446153846153846,
0.461538461538462,0.476923076923077,0.492307692307692,0.507692307692308,
0.523076923076923,0.538461538461538,0.553846153846154,0.569230769230769,
0.584615384615384,0.6,0.615384615384615,0.63076923076923,0.646153846153846,
0.661538461538461,0.676923076923076,0.692307692307692,0.707692307692307,
0.723076923076922,0.738461538461538,0.753846153846153,0.769230769230768,
0.784615384615384,0.799999999999999,0.815384615384614,0.83076923076923,
0.846153846153845,0.86153846153846,0.876923076923076,0.892307692307691,
0.907692307692306,0.923076923076922,0.938461538461537,0.953846153846152,
0.969230769230768,0.984615384615383,0.994228156739701),.UNSPECIFIED.)
CURVE()
GEOMETRIC_REPRESENTATION_ITEM()
RATIONAL_B_SPLINE_CURVE((1.,1.,1.,1.,1.,1.,1.,1.,1.,1.,1.,1.,1.,1.,1.,1.,
1.,1.,1.,1.,1.,1.,1.,1.,1.,1.,1.,1.,1.,1.,1.,1.,1.,1.,1.,1.,1.,1.,1.,1.,
1.,1.,1.,1.,1.,1.,1.,1.,1.,1.,1.,1.,1.,1.,1.,1.,1.,1.,1.,1.,1.,1.,1.,1.,
1.,1.,1.,1.,1.,1.))
REPRESENTATION_ITEM('')
);
#243=(
BOUNDED_CURVE()
B_SPLINE_CURVE(5,(#32489,#32490,#32491,#32492,#32493,#32494,#32495,#32496,
#32497,#32498,#32499,#32500,#32501,#32502,#32503,#32504,#32505,#32506,#32507,
#32508,#32509,#32510,#32511,#32512,#32513,#32514,#32515,#32516,#32517,#32518,
#32519,#32520,#32521,#32522,#32523,#32524,#32525,#32526,#32527,#32528,#32529,
#32530,#32531,#32532,#32533,#32534,#32535,#32536,#32537,#32538,#32539,#32540,
#32541,#32542,#32543,#32544,#32545,#32546,#32547,#32548,#32549,#32550,#32551,
#32552,#32553,#32554,#32555,#32556,#32557,#32558),.UNSPECIFIED.,.F.,.F.)
B_SPLINE_CURVE_WITH_KNOTS((6,1,1,1,1,1,1,1,1,1,1,1,1,1,1,1,1,1,1,1,1,1,
1,1,1,1,1,1,1,1,1,1,1,1,1,1,1,1,1,1,1,1,1,1,1,1,1,1,1,1,1,1,1,1,1,1,1,1,
1,1,1,1,1,1,1,6),(0.0057718433745102,0.0153846153846154,0.0307692307692308,
0.0461538461538462,0.0615384615384615,0.0769230769230769,0.0923076923076923,
0.107692307692308,0.123076923076923,0.138461538461538,0.153846153846154,
0.169230769230769,0.184615384615385,0.2,0.215384615384615,0.230769230769231,
0.246153846153846,0.261538461538462,0.276923076923077,0.292307692307692,
0.307692307692308,0.323076923076923,0.338461538461538,0.353846153846154,
0.369230769230769,0.384615384615385,0.4,0.415384615384615,0.430769230769231,
0.446153846153846,0.461538461538462,0.476923076923077,0.492307692307692,
0.507692307692308,0.523076923076923,0.538461538461538,0.553846153846154,
0.569230769230769,0.584615384615384,0.6,0.615384615384615,0.63076923076923,
0.646153846153846,0.661538461538461,0.676923076923076,0.692307692307692,
0.707692307692307,0.723076923076922,0.738461538461538,0.753846153846153,
0.769230769230768,0.784615384615384,0.799999999999999,0.815384615384614,
0.83076923076923,0.846153846153845,0.86153846153846,0.876923076923076,0.892307692307691,
0.907692307692306,0.923076923076922,0.938461538461537,0.953846153846152,
0.969230769230768,0.984615384615383,1.),.UNSPECIFIED.)
CURVE()
GEOMETRIC_REPRESENTATION_ITEM()
RATIONAL_B_SPLINE_CURVE((1.,1.,1.,1.,1.,1.,1.,1.,1.,1.,1.,1.,1.,1.,1.,1.,
1.,1.,1.,1.,1.,1.,1.,1.,1.,1.,1.,1.,1.,1.,1.,1.,1.,1.,1.,1.,1.,1.,1.,1.,
1.,1.,1.,1.,1.,1.,1.,1.,1.,1.,1.,1.,1.,1.,1.,1.,1.,1.,1.,1.,1.,1.,1.,1.,
1.,1.,1.,1.,1.,1.))
REPRESENTATION_ITEM('')
);
#244=(
BOUNDED_CURVE()
B_SPLINE_CURVE(5,(#32562,#32563,#32564,#32565,#32566,#32567,#32568,#32569,
#32570,#32571,#32572,#32573,#32574,#32575,#32576,#32577,#32578,#32579,#32580,
#32581,#32582,#32583,#32584,#32585,#32586,#32587,#32588,#32589,#32590,#32591,
#32592,#32593,#32594,#32595,#32596,#32597,#32598,#32599,#32600,#32601,#32602,
#32603,#32604,#32605,#32606,#32607,#32608,#32609,#32610,#32611,#32612,#32613,
#32614,#32615,#32616,#32617,#32618,#32619,#32620,#32621,#32622,#32623,#32624,
#32625,#32626,#32627,#32628,#32629,#32630,#32631),.UNSPECIFIED.,.F.,.F.)
B_SPLINE_CURVE_WITH_KNOTS((6,1,1,1,1,1,1,1,1,1,1,1,1,1,1,1,1,1,1,1,1,1,
1,1,1,1,1,1,1,1,1,1,1,1,1,1,1,1,1,1,1,1,1,1,1,1,1,1,1,1,1,1,1,1,1,1,1,1,
1,1,1,1,1,1,1,6),(0.,0.0153846153846154,0.0307692307692308,0.0461538461538462,
0.0615384615384615,0.0769230769230769,0.0923076923076923,0.107692307692308,
0.123076923076923,0.138461538461538,0.153846153846154,0.169230769230769,
0.184615384615385,0.2,0.215384615384615,0.230769230769231,0.246153846153846,
0.261538461538462,0.276923076923077,0.292307692307692,0.307692307692308,
0.323076923076923,0.338461538461538,0.353846153846154,0.369230769230769,
0.384615384615385,0.4,0.415384615384615,0.430769230769231,0.446153846153846,
0.461538461538462,0.476923076923077,0.492307692307692,0.507692307692308,
0.523076923076923,0.538461538461538,0.553846153846154,0.569230769230769,
0.584615384615384,0.6,0.615384615384615,0.63076923076923,0.646153846153846,
0.661538461538461,0.676923076923076,0.692307692307692,0.707692307692307,
0.723076923076922,0.738461538461538,0.753846153846153,0.769230769230768,
0.784615384615384,0.799999999999999,0.815384615384614,0.83076923076923,
0.846153846153845,0.86153846153846,0.876923076923076,0.892307692307691,
0.907692307692306,0.923076923076922,0.938461538461537,0.953846153846152,
0.969230769230768,0.984615384615383,0.994228156739694),.UNSPECIFIED.)
CURVE()
GEOMETRIC_REPRESENTATION_ITEM()
RATIONAL_B_SPLINE_CURVE((1.,1.,1.,1.,1.,1.,1.,1.,1.,1.,1.,1.,1.,1.,1.,1.,
1.,1.,1.,1.,1.,1.,1.,1.,1.,1.,1.,1.,1.,1.,1.,1.,1.,1.,1.,1.,1.,1.,1.,1.,
1.,1.,1.,1.,1.,1.,1.,1.,1.,1.,1.,1.,1.,1.,1.,1.,1.,1.,1.,1.,1.,1.,1.,1.,
1.,1.,1.,1.,1.,1.))
REPRESENTATION_ITEM('')
);
#245=(
BOUNDED_CURVE()
B_SPLINE_CURVE(5,(#32635,#32636,#32637,#32638,#32639,#32640,#32641,#32642,
#32643,#32644,#32645,#32646,#32647,#32648,#32649,#32650,#32651,#32652,#32653,
#32654,#32655,#32656,#32657,#32658,#32659,#32660,#32661,#32662,#32663,#32664,
#32665,#32666,#32667,#32668,#32669,#32670,#32671,#32672,#32673,#32674,#32675,
#32676,#32677,#32678,#32679,#32680,#32681,#32682,#32683,#32684,#32685,#32686,
#32687,#32688,#32689,#32690,#32691,#32692,#32693,#32694,#32695,#32696,#32697,
#32698,#32699,#32700,#32701,#32702,#32703,#32704),.UNSPECIFIED.,.F.,.F.)
B_SPLINE_CURVE_WITH_KNOTS((6,1,1,1,1,1,1,1,1,1,1,1,1,1,1,1,1,1,1,1,1,1,
1,1,1,1,1,1,1,1,1,1,1,1,1,1,1,1,1,1,1,1,1,1,1,1,1,1,1,1,1,1,1,1,1,1,1,1,
1,1,1,1,1,1,1,6),(0.00577184337452044,0.0153846153846154,0.0307692307692308,
0.0461538461538462,0.0615384615384615,0.0769230769230769,0.0923076923076923,
0.107692307692308,0.123076923076923,0.138461538461538,0.153846153846154,
0.169230769230769,0.184615384615385,0.2,0.215384615384615,0.230769230769231,
0.246153846153846,0.261538461538462,0.276923076923077,0.292307692307692,
0.307692307692308,0.323076923076923,0.338461538461538,0.353846153846154,
0.369230769230769,0.384615384615385,0.4,0.415384615384615,0.430769230769231,
0.446153846153846,0.461538461538462,0.476923076923077,0.492307692307692,
0.507692307692308,0.523076923076923,0.538461538461538,0.553846153846154,
0.569230769230769,0.584615384615384,0.6,0.615384615384615,0.63076923076923,
0.646153846153846,0.661538461538461,0.676923076923076,0.692307692307692,
0.707692307692307,0.723076923076922,0.738461538461538,0.753846153846153,
0.769230769230768,0.784615384615384,0.799999999999999,0.815384615384614,
0.83076923076923,0.846153846153845,0.86153846153846,0.876923076923076,0.892307692307691,
0.907692307692306,0.923076923076922,0.938461538461537,0.953846153846152,
0.969230769230768,0.984615384615383,1.),.UNSPECIFIED.)
CURVE()
GEOMETRIC_REPRESENTATION_ITEM()
RATIONAL_B_SPLINE_CURVE((1.,1.,1.,1.,1.,1.,1.,1.,1.,1.,1.,1.,1.,1.,1.,1.,
1.,1.,1.,1.,1.,1.,1.,1.,1.,1.,1.,1.,1.,1.,1.,1.,1.,1.,1.,1.,1.,1.,1.,1.,
1.,1.,1.,1.,1.,1.,1.,1.,1.,1.,1.,1.,1.,1.,1.,1.,1.,1.,1.,1.,1.,1.,1.,1.,
1.,1.,1.,1.,1.,1.))
REPRESENTATION_ITEM('')
);
#246=(
BOUNDED_CURVE()
B_SPLINE_CURVE(5,(#32708,#32709,#32710,#32711,#32712,#32713,#32714,#32715,
#32716,#32717,#32718,#32719,#32720,#32721,#32722,#32723,#32724,#32725,#32726,
#32727,#32728,#32729,#32730,#32731,#32732,#32733,#32734,#32735,#32736,#32737,
#32738,#32739,#32740,#32741,#32742,#32743,#32744,#32745,#32746,#32747,#32748,
#32749,#32750,#32751,#32752,#32753,#32754,#32755,#32756,#32757,#32758,#32759,
#32760,#32761,#32762,#32763,#32764,#32765,#32766,#32767,#32768,#32769,#32770,
#32771,#32772,#32773,#32774,#32775,#32776,#32777),.UNSPECIFIED.,.F.,.F.)
B_SPLINE_CURVE_WITH_KNOTS((6,1,1,1,1,1,1,1,1,1,1,1,1,1,1,1,1,1,1,1,1,1,
1,1,1,1,1,1,1,1,1,1,1,1,1,1,1,1,1,1,1,1,1,1,1,1,1,1,1,1,1,1,1,1,1,1,1,1,
1,1,1,1,1,1,1,6),(0.,0.0153846153846154,0.0307692307692308,0.0461538461538462,
0.0615384615384615,0.0769230769230769,0.0923076923076923,0.107692307692308,
0.123076923076923,0.138461538461538,0.153846153846154,0.169230769230769,
0.184615384615385,0.2,0.215384615384615,0.230769230769231,0.246153846153846,
0.261538461538462,0.276923076923077,0.292307692307692,0.307692307692308,
0.323076923076923,0.338461538461538,0.353846153846154,0.369230769230769,
0.384615384615385,0.4,0.415384615384615,0.430769230769231,0.446153846153846,
0.461538461538462,0.476923076923077,0.492307692307692,0.507692307692308,
0.523076923076923,0.538461538461538,0.553846153846154,0.569230769230769,
0.584615384615384,0.6,0.615384615384615,0.63076923076923,0.646153846153846,
0.661538461538461,0.676923076923076,0.692307692307692,0.707692307692307,
0.723076923076922,0.738461538461538,0.753846153846153,0.769230769230768,
0.784615384615384,0.799999999999999,0.815384615384614,0.83076923076923,
0.846153846153845,0.86153846153846,0.876923076923076,0.892307692307691,
0.907692307692306,0.923076923076922,0.938461538461537,0.953846153846152,
0.969230769230768,0.984615384615383,0.994228156739698),.UNSPECIFIED.)
CURVE()
GEOMETRIC_REPRESENTATION_ITEM()
RATIONAL_B_SPLINE_CURVE((1.,1.,1.,1.,1.,1.,1.,1.,1.,1.,1.,1.,1.,1.,1.,1.,
1.,1.,1.,1.,1.,1.,1.,1.,1.,1.,1.,1.,1.,1.,1.,1.,1.,1.,1.,1.,1.,1.,1.,1.,
1.,1.,1.,1.,1.,1.,1.,1.,1.,1.,1.,1.,1.,1.,1.,1.,1.,1.,1.,1.,1.,1.,1.,1.,
1.,1.,1.,1.,1.,1.))
REPRESENTATION_ITEM('')
);
#247=(
BOUNDED_CURVE()
B_SPLINE_CURVE(5,(#32781,#32782,#32783,#32784,#32785,#32786,#32787,#32788,
#32789,#32790,#32791,#32792,#32793,#32794,#32795,#32796,#32797,#32798,#32799,
#32800,#32801,#32802,#32803,#32804,#32805,#32806,#32807,#32808,#32809,#32810,
#32811,#32812,#32813,#32814,#32815,#32816,#32817,#32818,#32819,#32820,#32821,
#32822,#32823,#32824,#32825,#32826,#32827,#32828,#32829,#32830,#32831,#32832,
#32833,#32834,#32835,#32836,#32837,#32838,#32839,#32840,#32841,#32842,#32843,
#32844,#32845,#32846,#32847,#32848,#32849,#32850),.UNSPECIFIED.,.F.,.F.)
B_SPLINE_CURVE_WITH_KNOTS((6,1,1,1,1,1,1,1,1,1,1,1,1,1,1,1,1,1,1,1,1,1,
1,1,1,1,1,1,1,1,1,1,1,1,1,1,1,1,1,1,1,1,1,1,1,1,1,1,1,1,1,1,1,1,1,1,1,1,
1,1,1,1,1,1,1,6),(0.00577184337451607,0.0153846153846154,0.0307692307692308,
0.0461538461538462,0.0615384615384615,0.0769230769230769,0.0923076923076923,
0.107692307692308,0.123076923076923,0.138461538461538,0.153846153846154,
0.169230769230769,0.184615384615385,0.2,0.215384615384615,0.230769230769231,
0.246153846153846,0.261538461538462,0.276923076923077,0.292307692307692,
0.307692307692308,0.323076923076923,0.338461538461538,0.353846153846154,
0.369230769230769,0.384615384615385,0.4,0.415384615384615,0.430769230769231,
0.446153846153846,0.461538461538462,0.476923076923077,0.492307692307692,
0.507692307692308,0.523076923076923,0.538461538461538,0.553846153846154,
0.569230769230769,0.584615384615384,0.6,0.615384615384615,0.63076923076923,
0.646153846153846,0.661538461538461,0.676923076923076,0.692307692307692,
0.707692307692307,0.723076923076922,0.738461538461538,0.753846153846153,
0.769230769230768,0.784615384615384,0.799999999999999,0.815384615384614,
0.83076923076923,0.846153846153845,0.86153846153846,0.876923076923076,0.892307692307691,
0.907692307692306,0.923076923076922,0.938461538461537,0.953846153846152,
0.969230769230768,0.984615384615383,1.),.UNSPECIFIED.)
CURVE()
GEOMETRIC_REPRESENTATION_ITEM()
RATIONAL_B_SPLINE_CURVE((1.,1.,1.,1.,1.,1.,1.,1.,1.,1.,1.,1.,1.,1.,1.,1.,
1.,1.,1.,1.,1.,1.,1.,1.,1.,1.,1.,1.,1.,1.,1.,1.,1.,1.,1.,1.,1.,1.,1.,1.,
1.,1.,1.,1.,1.,1.,1.,1.,1.,1.,1.,1.,1.,1.,1.,1.,1.,1.,1.,1.,1.,1.,1.,1.,
1.,1.,1.,1.,1.,1.))
REPRESENTATION_ITEM('')
);
#248=(
BOUNDED_CURVE()
B_SPLINE_CURVE(5,(#32854,#32855,#32856,#32857,#32858,#32859,#32860,#32861,
#32862,#32863,#32864,#32865,#32866,#32867,#32868,#32869,#32870,#32871,#32872,
#32873,#32874,#32875,#32876,#32877,#32878,#32879,#32880,#32881,#32882,#32883,
#32884,#32885,#32886,#32887,#32888,#32889,#32890,#32891,#32892,#32893,#32894,
#32895,#32896,#32897,#32898,#32899,#32900,#32901,#32902,#32903,#32904,#32905,
#32906,#32907,#32908,#32909,#32910,#32911,#32912,#32913,#32914,#32915,#32916,
#32917,#32918,#32919,#32920,#32921,#32922,#32923),.UNSPECIFIED.,.F.,.F.)
B_SPLINE_CURVE_WITH_KNOTS((6,1,1,1,1,1,1,1,1,1,1,1,1,1,1,1,1,1,1,1,1,1,
1,1,1,1,1,1,1,1,1,1,1,1,1,1,1,1,1,1,1,1,1,1,1,1,1,1,1,1,1,1,1,1,1,1,1,1,
1,1,1,1,1,1,1,6),(0.,0.0153846153846154,0.0307692307692308,0.0461538461538462,
0.0615384615384615,0.0769230769230769,0.0923076923076923,0.107692307692308,
0.123076923076923,0.138461538461538,0.153846153846154,0.169230769230769,
0.184615384615385,0.2,0.215384615384615,0.230769230769231,0.246153846153846,
0.261538461538462,0.276923076923077,0.292307692307692,0.307692307692308,
0.323076923076923,0.338461538461538,0.353846153846154,0.369230769230769,
0.384615384615385,0.4,0.415384615384615,0.430769230769231,0.446153846153846,
0.461538461538462,0.476923076923077,0.492307692307692,0.507692307692308,
0.523076923076923,0.538461538461538,0.553846153846154,0.569230769230769,
0.584615384615384,0.6,0.615384615384615,0.63076923076923,0.646153846153846,
0.661538461538461,0.676923076923076,0.692307692307692,0.707692307692307,
0.723076923076922,0.738461538461538,0.753846153846153,0.769230769230768,
0.784615384615384,0.799999999999999,0.815384615384614,0.83076923076923,
0.846153846153845,0.86153846153846,0.876923076923076,0.892307692307691,
0.907692307692306,0.923076923076922,0.938461538461537,0.953846153846152,
0.969230769230768,0.984615384615383,0.994228156739704),.UNSPECIFIED.)
CURVE()
GEOMETRIC_REPRESENTATION_ITEM()
RATIONAL_B_SPLINE_CURVE((1.,1.,1.,1.,1.,1.,1.,1.,1.,1.,1.,1.,1.,1.,1.,1.,
1.,1.,1.,1.,1.,1.,1.,1.,1.,1.,1.,1.,1.,1.,1.,1.,1.,1.,1.,1.,1.,1.,1.,1.,
1.,1.,1.,1.,1.,1.,1.,1.,1.,1.,1.,1.,1.,1.,1.,1.,1.,1.,1.,1.,1.,1.,1.,1.,
1.,1.,1.,1.,1.,1.))
REPRESENTATION_ITEM('')
);
#249=(
BOUNDED_CURVE()
B_SPLINE_CURVE(5,(#32927,#32928,#32929,#32930,#32931,#32932,#32933,#32934,
#32935,#32936,#32937,#32938,#32939,#32940,#32941,#32942,#32943,#32944,#32945,
#32946,#32947,#32948,#32949,#32950,#32951,#32952,#32953,#32954,#32955,#32956,
#32957,#32958,#32959,#32960,#32961,#32962,#32963,#32964,#32965,#32966,#32967,
#32968,#32969,#32970,#32971,#32972,#32973,#32974,#32975,#32976,#32977,#32978,
#32979,#32980,#32981,#32982,#32983,#32984,#32985,#32986,#32987,#32988,#32989,
#32990,#32991,#32992,#32993,#32994,#32995,#32996),.UNSPECIFIED.,.F.,.F.)
B_SPLINE_CURVE_WITH_KNOTS((6,1,1,1,1,1,1,1,1,1,1,1,1,1,1,1,1,1,1,1,1,1,
1,1,1,1,1,1,1,1,1,1,1,1,1,1,1,1,1,1,1,1,1,1,1,1,1,1,1,1,1,1,1,1,1,1,1,1,
1,1,1,1,1,1,1,6),(0.00577184337449682,0.0153846153846154,0.0307692307692308,
0.0461538461538462,0.0615384615384615,0.0769230769230769,0.0923076923076923,
0.107692307692308,0.123076923076923,0.138461538461538,0.153846153846154,
0.169230769230769,0.184615384615385,0.2,0.215384615384615,0.230769230769231,
0.246153846153846,0.261538461538462,0.276923076923077,0.292307692307692,
0.307692307692308,0.323076923076923,0.338461538461538,0.353846153846154,
0.369230769230769,0.384615384615385,0.4,0.415384615384615,0.430769230769231,
0.446153846153846,0.461538461538462,0.476923076923077,0.492307692307692,
0.507692307692308,0.523076923076923,0.538461538461538,0.553846153846154,
0.569230769230769,0.584615384615384,0.6,0.615384615384615,0.63076923076923,
0.646153846153846,0.661538461538461,0.676923076923076,0.692307692307692,
0.707692307692307,0.723076923076922,0.738461538461538,0.753846153846153,
0.769230769230768,0.784615384615384,0.799999999999999,0.815384615384614,
0.83076923076923,0.846153846153845,0.86153846153846,0.876923076923076,0.892307692307691,
0.907692307692306,0.923076923076922,0.938461538461537,0.953846153846152,
0.969230769230768,0.984615384615383,1.),.UNSPECIFIED.)
CURVE()
GEOMETRIC_REPRESENTATION_ITEM()
RATIONAL_B_SPLINE_CURVE((1.,1.,1.,1.,1.,1.,1.,1.,1.,1.,1.,1.,1.,1.,1.,1.,
1.,1.,1.,1.,1.,1.,1.,1.,1.,1.,1.,1.,1.,1.,1.,1.,1.,1.,1.,1.,1.,1.,1.,1.,
1.,1.,1.,1.,1.,1.,1.,1.,1.,1.,1.,1.,1.,1.,1.,1.,1.,1.,1.,1.,1.,1.,1.,1.,
1.,1.,1.,1.,1.,1.))
REPRESENTATION_ITEM('')
);
#250=(
BOUNDED_CURVE()
B_SPLINE_CURVE(5,(#33000,#33001,#33002,#33003,#33004,#33005,#33006,#33007,
#33008,#33009,#33010,#33011,#33012,#33013,#33014,#33015,#33016,#33017,#33018,
#33019,#33020,#33021,#33022,#33023,#33024,#33025,#33026,#33027,#33028,#33029,
#33030,#33031,#33032,#33033,#33034,#33035,#33036,#33037,#33038,#33039,#33040,
#33041,#33042,#33043,#33044,#33045,#33046,#33047,#33048,#33049,#33050,#33051,
#33052,#33053,#33054,#33055,#33056,#33057,#33058,#33059,#33060,#33061,#33062,
#33063,#33064,#33065,#33066,#33067,#33068,#33069),.UNSPECIFIED.,.F.,.F.)
B_SPLINE_CURVE_WITH_KNOTS((6,1,1,1,1,1,1,1,1,1,1,1,1,1,1,1,1,1,1,1,1,1,
1,1,1,1,1,1,1,1,1,1,1,1,1,1,1,1,1,1,1,1,1,1,1,1,1,1,1,1,1,1,1,1,1,1,1,1,
1,1,1,1,1,1,1,6),(0.,0.0153846153846154,0.0307692307692308,0.0461538461538462,
0.0615384615384615,0.0769230769230769,0.0923076923076923,0.107692307692308,
0.123076923076923,0.138461538461538,0.153846153846154,0.169230769230769,
0.184615384615385,0.2,0.215384615384615,0.230769230769231,0.246153846153846,
0.261538461538462,0.276923076923077,0.292307692307692,0.307692307692308,
0.323076923076923,0.338461538461538,0.353846153846154,0.369230769230769,
0.384615384615385,0.4,0.415384615384615,0.430769230769231,0.446153846153846,
0.461538461538462,0.476923076923077,0.492307692307692,0.507692307692308,
0.523076923076923,0.538461538461538,0.553846153846154,0.569230769230769,
0.584615384615384,0.6,0.615384615384615,0.63076923076923,0.646153846153846,
0.661538461538461,0.676923076923076,0.692307692307692,0.707692307692307,
0.723076923076922,0.738461538461538,0.753846153846153,0.769230769230768,
0.784615384615384,0.799999999999999,0.815384615384614,0.83076923076923,
0.846153846153845,0.86153846153846,0.876923076923076,0.892307692307691,
0.907692307692306,0.923076923076922,0.938461538461537,0.953846153846152,
0.969230769230768,0.984615384615383,0.994228156739711),.UNSPECIFIED.)
CURVE()
GEOMETRIC_REPRESENTATION_ITEM()
RATIONAL_B_SPLINE_CURVE((1.,1.,1.,1.,1.,1.,1.,1.,1.,1.,1.,1.,1.,1.,1.,1.,
1.,1.,1.,1.,1.,1.,1.,1.,1.,1.,1.,1.,1.,1.,1.,1.,1.,1.,1.,1.,1.,1.,1.,1.,
1.,1.,1.,1.,1.,1.,1.,1.,1.,1.,1.,1.,1.,1.,1.,1.,1.,1.,1.,1.,1.,1.,1.,1.,
1.,1.,1.,1.,1.,1.))
REPRESENTATION_ITEM('')
);
#251=(
BOUNDED_CURVE()
B_SPLINE_CURVE(5,(#33073,#33074,#33075,#33076,#33077,#33078,#33079,#33080,
#33081,#33082,#33083,#33084,#33085,#33086,#33087,#33088,#33089,#33090,#33091,
#33092,#33093,#33094,#33095,#33096,#33097,#33098,#33099,#33100,#33101,#33102,
#33103,#33104,#33105,#33106,#33107,#33108,#33109,#33110,#33111,#33112,#33113,
#33114,#33115,#33116,#33117,#33118,#33119,#33120,#33121,#33122,#33123,#33124,
#33125,#33126,#33127,#33128,#33129,#33130,#33131,#33132,#33133,#33134,#33135,
#33136,#33137,#33138,#33139,#33140,#33141,#33142),.UNSPECIFIED.,.F.,.F.)
B_SPLINE_CURVE_WITH_KNOTS((6,1,1,1,1,1,1,1,1,1,1,1,1,1,1,1,1,1,1,1,1,1,
1,1,1,1,1,1,1,1,1,1,1,1,1,1,1,1,1,1,1,1,1,1,1,1,1,1,1,1,1,1,1,1,1,1,1,1,
1,1,1,1,1,1,1,6),(0.00577184337450313,0.0153846153846154,0.0307692307692308,
0.0461538461538462,0.0615384615384615,0.0769230769230769,0.0923076923076923,
0.107692307692308,0.123076923076923,0.138461538461538,0.153846153846154,
0.169230769230769,0.184615384615385,0.2,0.215384615384615,0.230769230769231,
0.246153846153846,0.261538461538462,0.276923076923077,0.292307692307692,
0.307692307692308,0.323076923076923,0.338461538461538,0.353846153846154,
0.369230769230769,0.384615384615385,0.4,0.415384615384615,0.430769230769231,
0.446153846153846,0.461538461538462,0.476923076923077,0.492307692307692,
0.507692307692308,0.523076923076923,0.538461538461538,0.553846153846154,
0.569230769230769,0.584615384615384,0.6,0.615384615384615,0.63076923076923,
0.646153846153846,0.661538461538461,0.676923076923076,0.692307692307692,
0.707692307692307,0.723076923076922,0.738461538461538,0.753846153846153,
0.769230769230768,0.784615384615384,0.799999999999999,0.815384615384614,
0.83076923076923,0.846153846153845,0.86153846153846,0.876923076923076,0.892307692307691,
0.907692307692306,0.923076923076922,0.938461538461537,0.953846153846152,
0.969230769230768,0.984615384615383,1.),.UNSPECIFIED.)
CURVE()
GEOMETRIC_REPRESENTATION_ITEM()
RATIONAL_B_SPLINE_CURVE((1.,1.,1.,1.,1.,1.,1.,1.,1.,1.,1.,1.,1.,1.,1.,1.,
1.,1.,1.,1.,1.,1.,1.,1.,1.,1.,1.,1.,1.,1.,1.,1.,1.,1.,1.,1.,1.,1.,1.,1.,
1.,1.,1.,1.,1.,1.,1.,1.,1.,1.,1.,1.,1.,1.,1.,1.,1.,1.,1.,1.,1.,1.,1.,1.,
1.,1.,1.,1.,1.,1.))
REPRESENTATION_ITEM('')
);
#252=(
BOUNDED_CURVE()
B_SPLINE_CURVE(5,(#33146,#33147,#33148,#33149,#33150,#33151,#33152,#33153,
#33154,#33155,#33156,#33157,#33158,#33159,#33160,#33161,#33162,#33163,#33164,
#33165,#33166,#33167,#33168,#33169,#33170,#33171,#33172,#33173,#33174,#33175,
#33176,#33177,#33178,#33179,#33180,#33181,#33182,#33183,#33184,#33185,#33186,
#33187,#33188,#33189,#33190,#33191,#33192,#33193,#33194,#33195,#33196,#33197,
#33198,#33199,#33200,#33201,#33202,#33203,#33204,#33205,#33206,#33207,#33208,
#33209,#33210,#33211,#33212,#33213,#33214,#33215),.UNSPECIFIED.,.F.,.F.)
B_SPLINE_CURVE_WITH_KNOTS((6,1,1,1,1,1,1,1,1,1,1,1,1,1,1,1,1,1,1,1,1,1,
1,1,1,1,1,1,1,1,1,1,1,1,1,1,1,1,1,1,1,1,1,1,1,1,1,1,1,1,1,1,1,1,1,1,1,1,
1,1,1,1,1,1,1,6),(0.,0.0153846153846154,0.0307692307692308,0.0461538461538462,
0.0615384615384615,0.0769230769230769,0.0923076923076923,0.107692307692308,
0.123076923076923,0.138461538461538,0.153846153846154,0.169230769230769,
0.184615384615385,0.2,0.215384615384615,0.230769230769231,0.246153846153846,
0.261538461538462,0.276923076923077,0.292307692307692,0.307692307692308,
0.323076923076923,0.338461538461538,0.353846153846154,0.369230769230769,
0.384615384615385,0.4,0.415384615384615,0.430769230769231,0.446153846153846,
0.461538461538462,0.476923076923077,0.492307692307692,0.507692307692308,
0.523076923076923,0.538461538461538,0.553846153846154,0.569230769230769,
0.584615384615384,0.6,0.615384615384615,0.63076923076923,0.646153846153846,
0.661538461538461,0.676923076923076,0.692307692307692,0.707692307692307,
0.723076923076922,0.738461538461538,0.753846153846153,0.769230769230768,
0.784615384615384,0.799999999999999,0.815384615384614,0.83076923076923,
0.846153846153845,0.86153846153846,0.876923076923076,0.892307692307691,
0.907692307692306,0.923076923076922,0.938461538461537,0.953846153846152,
0.969230769230768,0.984615384615383,0.9942281567397),.UNSPECIFIED.)
CURVE()
GEOMETRIC_REPRESENTATION_ITEM()
RATIONAL_B_SPLINE_CURVE((1.,1.,1.,1.,1.,1.,1.,1.,1.,1.,1.,1.,1.,1.,1.,1.,
1.,1.,1.,1.,1.,1.,1.,1.,1.,1.,1.,1.,1.,1.,1.,1.,1.,1.,1.,1.,1.,1.,1.,1.,
1.,1.,1.,1.,1.,1.,1.,1.,1.,1.,1.,1.,1.,1.,1.,1.,1.,1.,1.,1.,1.,1.,1.,1.,
1.,1.,1.,1.,1.,1.))
REPRESENTATION_ITEM('')
);
#253=(
BOUNDED_CURVE()
B_SPLINE_CURVE(5,(#33219,#33220,#33221,#33222,#33223,#33224,#33225,#33226,
#33227,#33228,#33229,#33230,#33231,#33232,#33233,#33234,#33235,#33236,#33237,
#33238,#33239,#33240,#33241,#33242,#33243,#33244,#33245,#33246,#33247,#33248,
#33249,#33250,#33251,#33252,#33253,#33254,#33255,#33256,#33257,#33258,#33259,
#33260,#33261,#33262,#33263,#33264,#33265,#33266,#33267,#33268,#33269,#33270,
#33271,#33272,#33273,#33274,#33275,#33276,#33277,#33278,#33279,#33280,#33281,
#33282,#33283,#33284,#33285,#33286,#33287,#33288),.UNSPECIFIED.,.F.,.F.)
B_SPLINE_CURVE_WITH_KNOTS((6,1,1,1,1,1,1,1,1,1,1,1,1,1,1,1,1,1,1,1,1,1,
1,1,1,1,1,1,1,1,1,1,1,1,1,1,1,1,1,1,1,1,1,1,1,1,1,1,1,1,1,1,1,1,1,1,1,1,
1,1,1,1,1,1,1,6),(0.00577184337452087,0.0153846153846154,0.0307692307692308,
0.0461538461538462,0.0615384615384615,0.0769230769230769,0.0923076923076923,
0.107692307692308,0.123076923076923,0.138461538461538,0.153846153846154,
0.169230769230769,0.184615384615385,0.2,0.215384615384615,0.230769230769231,
0.246153846153846,0.261538461538462,0.276923076923077,0.292307692307692,
0.307692307692308,0.323076923076923,0.338461538461538,0.353846153846154,
0.369230769230769,0.384615384615385,0.4,0.415384615384615,0.430769230769231,
0.446153846153846,0.461538461538462,0.476923076923077,0.492307692307692,
0.507692307692308,0.523076923076923,0.538461538461538,0.553846153846154,
0.569230769230769,0.584615384615384,0.6,0.615384615384615,0.63076923076923,
0.646153846153846,0.661538461538461,0.676923076923076,0.692307692307692,
0.707692307692307,0.723076923076922,0.738461538461538,0.753846153846153,
0.769230769230768,0.784615384615384,0.799999999999999,0.815384615384614,
0.83076923076923,0.846153846153845,0.86153846153846,0.876923076923076,0.892307692307691,
0.907692307692306,0.923076923076922,0.938461538461537,0.953846153846152,
0.969230769230768,0.984615384615383,1.),.UNSPECIFIED.)
CURVE()
GEOMETRIC_REPRESENTATION_ITEM()
RATIONAL_B_SPLINE_CURVE((1.,1.,1.,1.,1.,1.,1.,1.,1.,1.,1.,1.,1.,1.,1.,1.,
1.,1.,1.,1.,1.,1.,1.,1.,1.,1.,1.,1.,1.,1.,1.,1.,1.,1.,1.,1.,1.,1.,1.,1.,
1.,1.,1.,1.,1.,1.,1.,1.,1.,1.,1.,1.,1.,1.,1.,1.,1.,1.,1.,1.,1.,1.,1.,1.,
1.,1.,1.,1.,1.,1.))
REPRESENTATION_ITEM('')
);
#254=(
BOUNDED_CURVE()
B_SPLINE_CURVE(5,(#33292,#33293,#33294,#33295,#33296,#33297,#33298,#33299,
#33300,#33301,#33302,#33303,#33304,#33305,#33306,#33307,#33308,#33309,#33310,
#33311,#33312,#33313,#33314,#33315,#33316,#33317,#33318,#33319,#33320,#33321,
#33322,#33323,#33324,#33325,#33326,#33327,#33328,#33329,#33330,#33331,#33332,
#33333,#33334,#33335,#33336,#33337,#33338,#33339,#33340,#33341,#33342,#33343,
#33344,#33345,#33346,#33347,#33348,#33349,#33350,#33351,#33352,#33353,#33354,
#33355,#33356,#33357,#33358,#33359,#33360,#33361),.UNSPECIFIED.,.F.,.F.)
B_SPLINE_CURVE_WITH_KNOTS((6,1,1,1,1,1,1,1,1,1,1,1,1,1,1,1,1,1,1,1,1,1,
1,1,1,1,1,1,1,1,1,1,1,1,1,1,1,1,1,1,1,1,1,1,1,1,1,1,1,1,1,1,1,1,1,1,1,1,
1,1,1,1,1,1,1,6),(0.,0.0153846153846154,0.0307692307692308,0.0461538461538462,
0.0615384615384615,0.0769230769230769,0.0923076923076923,0.107692307692308,
0.123076923076923,0.138461538461538,0.153846153846154,0.169230769230769,
0.184615384615385,0.2,0.215384615384615,0.230769230769231,0.246153846153846,
0.261538461538462,0.276923076923077,0.292307692307692,0.307692307692308,
0.323076923076923,0.338461538461538,0.353846153846154,0.369230769230769,
0.384615384615385,0.4,0.415384615384615,0.430769230769231,0.446153846153846,
0.461538461538462,0.476923076923077,0.492307692307692,0.507692307692308,
0.523076923076923,0.538461538461538,0.553846153846154,0.569230769230769,
0.584615384615384,0.6,0.615384615384615,0.63076923076923,0.646153846153846,
0.661538461538461,0.676923076923076,0.692307692307692,0.707692307692307,
0.723076923076922,0.738461538461538,0.753846153846153,0.769230769230768,
0.784615384615384,0.799999999999999,0.815384615384614,0.83076923076923,
0.846153846153845,0.86153846153846,0.876923076923076,0.892307692307691,
0.907692307692306,0.923076923076922,0.938461538461537,0.953846153846152,
0.969230769230768,0.984615384615383,0.994228156739692),.UNSPECIFIED.)
CURVE()
GEOMETRIC_REPRESENTATION_ITEM()
RATIONAL_B_SPLINE_CURVE((1.,1.,1.,1.,1.,1.,1.,1.,1.,1.,1.,1.,1.,1.,1.,1.,
1.,1.,1.,1.,1.,1.,1.,1.,1.,1.,1.,1.,1.,1.,1.,1.,1.,1.,1.,1.,1.,1.,1.,1.,
1.,1.,1.,1.,1.,1.,1.,1.,1.,1.,1.,1.,1.,1.,1.,1.,1.,1.,1.,1.,1.,1.,1.,1.,
1.,1.,1.,1.,1.,1.))
REPRESENTATION_ITEM('')
);
#255=(
BOUNDED_CURVE()
B_SPLINE_CURVE(5,(#33365,#33366,#33367,#33368,#33369,#33370,#33371,#33372,
#33373,#33374,#33375,#33376,#33377,#33378,#33379,#33380,#33381,#33382,#33383,
#33384,#33385,#33386,#33387,#33388,#33389,#33390,#33391,#33392,#33393,#33394,
#33395,#33396,#33397,#33398,#33399,#33400,#33401,#33402,#33403,#33404,#33405,
#33406,#33407,#33408,#33409,#33410,#33411,#33412,#33413,#33414,#33415,#33416,
#33417,#33418,#33419,#33420,#33421,#33422,#33423,#33424,#33425,#33426,#33427,
#33428,#33429,#33430,#33431,#33432,#33433,#33434),.UNSPECIFIED.,.F.,.F.)
B_SPLINE_CURVE_WITH_KNOTS((6,1,1,1,1,1,1,1,1,1,1,1,1,1,1,1,1,1,1,1,1,1,
1,1,1,1,1,1,1,1,1,1,1,1,1,1,1,1,1,1,1,1,1,1,1,1,1,1,1,1,1,1,1,1,1,1,1,1,
1,1,1,1,1,1,1,6),(0.00577184337450777,0.0153846153846154,0.0307692307692308,
0.0461538461538462,0.0615384615384615,0.0769230769230769,0.0923076923076923,
0.107692307692308,0.123076923076923,0.138461538461538,0.153846153846154,
0.169230769230769,0.184615384615385,0.2,0.215384615384615,0.230769230769231,
0.246153846153846,0.261538461538462,0.276923076923077,0.292307692307692,
0.307692307692308,0.323076923076923,0.338461538461538,0.353846153846154,
0.369230769230769,0.384615384615385,0.4,0.415384615384615,0.430769230769231,
0.446153846153846,0.461538461538462,0.476923076923077,0.492307692307692,
0.507692307692308,0.523076923076923,0.538461538461538,0.553846153846154,
0.569230769230769,0.584615384615384,0.6,0.615384615384615,0.63076923076923,
0.646153846153846,0.661538461538461,0.676923076923076,0.692307692307692,
0.707692307692307,0.723076923076922,0.738461538461538,0.753846153846153,
0.769230769230768,0.784615384615384,0.799999999999999,0.815384615384614,
0.83076923076923,0.846153846153845,0.86153846153846,0.876923076923076,0.892307692307691,
0.907692307692306,0.923076923076922,0.938461538461537,0.953846153846152,
0.969230769230768,0.984615384615383,1.),.UNSPECIFIED.)
CURVE()
GEOMETRIC_REPRESENTATION_ITEM()
RATIONAL_B_SPLINE_CURVE((1.,1.,1.,1.,1.,1.,1.,1.,1.,1.,1.,1.,1.,1.,1.,1.,
1.,1.,1.,1.,1.,1.,1.,1.,1.,1.,1.,1.,1.,1.,1.,1.,1.,1.,1.,1.,1.,1.,1.,1.,
1.,1.,1.,1.,1.,1.,1.,1.,1.,1.,1.,1.,1.,1.,1.,1.,1.,1.,1.,1.,1.,1.,1.,1.,
1.,1.,1.,1.,1.,1.))
REPRESENTATION_ITEM('')
);
#256=(
BOUNDED_CURVE()
B_SPLINE_CURVE(5,(#33438,#33439,#33440,#33441,#33442,#33443,#33444,#33445,
#33446,#33447,#33448,#33449,#33450,#33451,#33452,#33453,#33454,#33455,#33456,
#33457,#33458,#33459,#33460,#33461,#33462,#33463,#33464,#33465,#33466,#33467,
#33468,#33469,#33470,#33471,#33472,#33473,#33474,#33475,#33476,#33477,#33478,
#33479,#33480,#33481,#33482,#33483,#33484,#33485,#33486,#33487,#33488,#33489,
#33490,#33491,#33492,#33493,#33494,#33495,#33496,#33497,#33498,#33499,#33500,
#33501,#33502,#33503,#33504,#33505,#33506,#33507),.UNSPECIFIED.,.F.,.F.)
B_SPLINE_CURVE_WITH_KNOTS((6,1,1,1,1,1,1,1,1,1,1,1,1,1,1,1,1,1,1,1,1,1,
1,1,1,1,1,1,1,1,1,1,1,1,1,1,1,1,1,1,1,1,1,1,1,1,1,1,1,1,1,1,1,1,1,1,1,1,
1,1,1,1,1,1,1,6),(0.,0.0153846153846154,0.0307692307692308,0.0461538461538462,
0.0615384615384615,0.0769230769230769,0.0923076923076923,0.107692307692308,
0.123076923076923,0.138461538461538,0.153846153846154,0.169230769230769,
0.184615384615385,0.2,0.215384615384615,0.230769230769231,0.246153846153846,
0.261538461538462,0.276923076923077,0.292307692307692,0.307692307692308,
0.323076923076923,0.338461538461538,0.353846153846154,0.369230769230769,
0.384615384615385,0.4,0.415384615384615,0.430769230769231,0.446153846153846,
0.461538461538462,0.476923076923077,0.492307692307692,0.507692307692308,
0.523076923076923,0.538461538461538,0.553846153846154,0.569230769230769,
0.584615384615384,0.6,0.615384615384615,0.63076923076923,0.646153846153846,
0.661538461538461,0.676923076923076,0.692307692307692,0.707692307692307,
0.723076923076922,0.738461538461538,0.753846153846153,0.769230769230768,
0.784615384615384,0.799999999999999,0.815384615384614,0.83076923076923,
0.846153846153845,0.86153846153846,0.876923076923076,0.892307692307691,
0.907692307692306,0.923076923076922,0.938461538461537,0.953846153846152,
0.969230769230768,0.984615384615383,0.994228156739701),.UNSPECIFIED.)
CURVE()
GEOMETRIC_REPRESENTATION_ITEM()
RATIONAL_B_SPLINE_CURVE((1.,1.,1.,1.,1.,1.,1.,1.,1.,1.,1.,1.,1.,1.,1.,1.,
1.,1.,1.,1.,1.,1.,1.,1.,1.,1.,1.,1.,1.,1.,1.,1.,1.,1.,1.,1.,1.,1.,1.,1.,
1.,1.,1.,1.,1.,1.,1.,1.,1.,1.,1.,1.,1.,1.,1.,1.,1.,1.,1.,1.,1.,1.,1.,1.,
1.,1.,1.,1.,1.,1.))
REPRESENTATION_ITEM('')
);
#257=(
BOUNDED_CURVE()
B_SPLINE_CURVE(5,(#33511,#33512,#33513,#33514,#33515,#33516,#33517,#33518,
#33519,#33520,#33521,#33522,#33523,#33524,#33525,#33526,#33527,#33528,#33529,
#33530,#33531,#33532,#33533,#33534,#33535,#33536,#33537,#33538,#33539,#33540,
#33541,#33542,#33543,#33544,#33545,#33546,#33547,#33548,#33549,#33550,#33551,
#33552,#33553,#33554,#33555,#33556,#33557,#33558,#33559,#33560,#33561,#33562,
#33563,#33564,#33565,#33566,#33567,#33568,#33569,#33570,#33571,#33572,#33573,
#33574,#33575,#33576,#33577,#33578,#33579,#33580),.UNSPECIFIED.,.F.,.F.)
B_SPLINE_CURVE_WITH_KNOTS((6,1,1,1,1,1,1,1,1,1,1,1,1,1,1,1,1,1,1,1,1,1,
1,1,1,1,1,1,1,1,1,1,1,1,1,1,1,1,1,1,1,1,1,1,1,1,1,1,1,1,1,1,1,1,1,1,1,1,
1,1,1,1,1,1,1,6),(0.00577184337450943,0.0153846153846154,0.0307692307692308,
0.0461538461538462,0.0615384615384615,0.0769230769230769,0.0923076923076923,
0.107692307692308,0.123076923076923,0.138461538461538,0.153846153846154,
0.169230769230769,0.184615384615385,0.2,0.215384615384615,0.230769230769231,
0.246153846153846,0.261538461538462,0.276923076923077,0.292307692307692,
0.307692307692308,0.323076923076923,0.338461538461538,0.353846153846154,
0.369230769230769,0.384615384615385,0.4,0.415384615384615,0.430769230769231,
0.446153846153846,0.461538461538462,0.476923076923077,0.492307692307692,
0.507692307692308,0.523076923076923,0.538461538461538,0.553846153846154,
0.569230769230769,0.584615384615384,0.6,0.615384615384615,0.63076923076923,
0.646153846153846,0.661538461538461,0.676923076923076,0.692307692307692,
0.707692307692307,0.723076923076922,0.738461538461538,0.753846153846153,
0.769230769230768,0.784615384615384,0.799999999999999,0.815384615384614,
0.83076923076923,0.846153846153845,0.86153846153846,0.876923076923076,0.892307692307691,
0.907692307692306,0.923076923076922,0.938461538461537,0.953846153846152,
0.969230769230768,0.984615384615383,1.),.UNSPECIFIED.)
CURVE()
GEOMETRIC_REPRESENTATION_ITEM()
RATIONAL_B_SPLINE_CURVE((1.,1.,1.,1.,1.,1.,1.,1.,1.,1.,1.,1.,1.,1.,1.,1.,
1.,1.,1.,1.,1.,1.,1.,1.,1.,1.,1.,1.,1.,1.,1.,1.,1.,1.,1.,1.,1.,1.,1.,1.,
1.,1.,1.,1.,1.,1.,1.,1.,1.,1.,1.,1.,1.,1.,1.,1.,1.,1.,1.,1.,1.,1.,1.,1.,
1.,1.,1.,1.,1.,1.))
REPRESENTATION_ITEM('')
);
#258=(
BOUNDED_CURVE()
B_SPLINE_CURVE(5,(#33584,#33585,#33586,#33587,#33588,#33589,#33590,#33591,
#33592,#33593,#33594,#33595,#33596,#33597,#33598,#33599,#33600,#33601,#33602,
#33603,#33604,#33605,#33606,#33607,#33608,#33609,#33610,#33611,#33612,#33613,
#33614,#33615,#33616,#33617,#33618,#33619,#33620,#33621,#33622,#33623,#33624,
#33625,#33626,#33627,#33628,#33629,#33630,#33631,#33632,#33633,#33634,#33635,
#33636,#33637,#33638,#33639,#33640,#33641,#33642,#33643,#33644,#33645,#33646,
#33647,#33648,#33649,#33650,#33651,#33652,#33653),.UNSPECIFIED.,.F.,.F.)
B_SPLINE_CURVE_WITH_KNOTS((6,1,1,1,1,1,1,1,1,1,1,1,1,1,1,1,1,1,1,1,1,1,
1,1,1,1,1,1,1,1,1,1,1,1,1,1,1,1,1,1,1,1,1,1,1,1,1,1,1,1,1,1,1,1,1,1,1,1,
1,1,1,1,1,1,1,6),(0.,0.0153846153846154,0.0307692307692308,0.0461538461538462,
0.0615384615384615,0.0769230769230769,0.0923076923076923,0.107692307692308,
0.123076923076923,0.138461538461538,0.153846153846154,0.169230769230769,
0.184615384615385,0.2,0.215384615384615,0.230769230769231,0.246153846153846,
0.261538461538462,0.276923076923077,0.292307692307692,0.307692307692308,
0.323076923076923,0.338461538461538,0.353846153846154,0.369230769230769,
0.384615384615385,0.4,0.415384615384615,0.430769230769231,0.446153846153846,
0.461538461538462,0.476923076923077,0.492307692307692,0.507692307692308,
0.523076923076923,0.538461538461538,0.553846153846154,0.569230769230769,
0.584615384615384,0.6,0.615384615384615,0.63076923076923,0.646153846153846,
0.661538461538461,0.676923076923076,0.692307692307692,0.707692307692307,
0.723076923076922,0.738461538461538,0.753846153846153,0.769230769230768,
0.784615384615384,0.799999999999999,0.815384615384614,0.83076923076923,
0.846153846153845,0.86153846153846,0.876923076923076,0.892307692307691,
0.907692307692306,0.923076923076922,0.938461538461537,0.953846153846152,
0.969230769230768,0.984615384615383,0.994228156739699),.UNSPECIFIED.)
CURVE()
GEOMETRIC_REPRESENTATION_ITEM()
RATIONAL_B_SPLINE_CURVE((1.,1.,1.,1.,1.,1.,1.,1.,1.,1.,1.,1.,1.,1.,1.,1.,
1.,1.,1.,1.,1.,1.,1.,1.,1.,1.,1.,1.,1.,1.,1.,1.,1.,1.,1.,1.,1.,1.,1.,1.,
1.,1.,1.,1.,1.,1.,1.,1.,1.,1.,1.,1.,1.,1.,1.,1.,1.,1.,1.,1.,1.,1.,1.,1.,
1.,1.,1.,1.,1.,1.))
REPRESENTATION_ITEM('')
);
#259=(
BOUNDED_CURVE()
B_SPLINE_CURVE(5,(#33657,#33658,#33659,#33660,#33661,#33662,#33663,#33664,
#33665,#33666,#33667,#33668,#33669,#33670,#33671,#33672,#33673,#33674,#33675,
#33676,#33677,#33678,#33679,#33680,#33681,#33682,#33683,#33684,#33685,#33686,
#33687,#33688,#33689,#33690,#33691,#33692,#33693,#33694,#33695,#33696,#33697,
#33698,#33699,#33700,#33701,#33702,#33703,#33704,#33705,#33706,#33707,#33708,
#33709,#33710,#33711,#33712,#33713,#33714,#33715,#33716,#33717,#33718,#33719,
#33720,#33721,#33722,#33723,#33724,#33725,#33726),.UNSPECIFIED.,.F.,.F.)
B_SPLINE_CURVE_WITH_KNOTS((6,1,1,1,1,1,1,1,1,1,1,1,1,1,1,1,1,1,1,1,1,1,
1,1,1,1,1,1,1,1,1,1,1,1,1,1,1,1,1,1,1,1,1,1,1,1,1,1,1,1,1,1,1,1,1,1,1,1,
1,1,1,1,1,1,1,6),(0.00577184337448657,0.0153846153846154,0.0307692307692308,
0.0461538461538462,0.0615384615384615,0.0769230769230769,0.0923076923076923,
0.107692307692308,0.123076923076923,0.138461538461538,0.153846153846154,
0.169230769230769,0.184615384615385,0.2,0.215384615384615,0.230769230769231,
0.246153846153846,0.261538461538462,0.276923076923077,0.292307692307692,
0.307692307692308,0.323076923076923,0.338461538461538,0.353846153846154,
0.369230769230769,0.384615384615385,0.4,0.415384615384615,0.430769230769231,
0.446153846153846,0.461538461538462,0.476923076923077,0.492307692307692,
0.507692307692308,0.523076923076923,0.538461538461538,0.553846153846154,
0.569230769230769,0.584615384615384,0.6,0.615384615384615,0.63076923076923,
0.646153846153846,0.661538461538461,0.676923076923076,0.692307692307692,
0.707692307692307,0.723076923076922,0.738461538461538,0.753846153846153,
0.769230769230768,0.784615384615384,0.799999999999999,0.815384615384614,
0.83076923076923,0.846153846153845,0.86153846153846,0.876923076923076,0.892307692307691,
0.907692307692306,0.923076923076922,0.938461538461537,0.953846153846152,
0.969230769230768,0.984615384615383,1.),.UNSPECIFIED.)
CURVE()
GEOMETRIC_REPRESENTATION_ITEM()
RATIONAL_B_SPLINE_CURVE((1.,1.,1.,1.,1.,1.,1.,1.,1.,1.,1.,1.,1.,1.,1.,1.,
1.,1.,1.,1.,1.,1.,1.,1.,1.,1.,1.,1.,1.,1.,1.,1.,1.,1.,1.,1.,1.,1.,1.,1.,
1.,1.,1.,1.,1.,1.,1.,1.,1.,1.,1.,1.,1.,1.,1.,1.,1.,1.,1.,1.,1.,1.,1.,1.,
1.,1.,1.,1.,1.,1.))
REPRESENTATION_ITEM('')
);
#260=(
BOUNDED_CURVE()
B_SPLINE_CURVE(5,(#33730,#33731,#33732,#33733,#33734,#33735,#33736,#33737,
#33738,#33739,#33740,#33741,#33742,#33743,#33744,#33745,#33746,#33747,#33748,
#33749,#33750,#33751,#33752,#33753,#33754,#33755,#33756,#33757,#33758,#33759,
#33760,#33761,#33762,#33763,#33764,#33765,#33766,#33767,#33768,#33769,#33770,
#33771,#33772,#33773,#33774,#33775,#33776,#33777,#33778,#33779,#33780,#33781,
#33782,#33783,#33784,#33785,#33786,#33787,#33788,#33789,#33790,#33791,#33792,
#33793,#33794,#33795,#33796,#33797,#33798,#33799),.UNSPECIFIED.,.F.,.F.)
B_SPLINE_CURVE_WITH_KNOTS((6,1,1,1,1,1,1,1,1,1,1,1,1,1,1,1,1,1,1,1,1,1,
1,1,1,1,1,1,1,1,1,1,1,1,1,1,1,1,1,1,1,1,1,1,1,1,1,1,1,1,1,1,1,1,1,1,1,1,
1,1,1,1,1,1,1,6),(0.,0.0153846153846154,0.0307692307692308,0.0461538461538462,
0.0615384615384615,0.0769230769230769,0.0923076923076923,0.107692307692308,
0.123076923076923,0.138461538461538,0.153846153846154,0.169230769230769,
0.184615384615385,0.2,0.215384615384615,0.230769230769231,0.246153846153846,
0.261538461538462,0.276923076923077,0.292307692307692,0.307692307692308,
0.323076923076923,0.338461538461538,0.353846153846154,0.369230769230769,
0.384615384615385,0.4,0.415384615384615,0.430769230769231,0.446153846153846,
0.461538461538462,0.476923076923077,0.492307692307692,0.507692307692308,
0.523076923076923,0.538461538461538,0.553846153846154,0.569230769230769,
0.584615384615384,0.6,0.615384615384615,0.63076923076923,0.646153846153846,
0.661538461538461,0.676923076923076,0.692307692307692,0.707692307692307,
0.723076923076922,0.738461538461538,0.753846153846153,0.769230769230768,
0.784615384615384,0.799999999999999,0.815384615384614,0.83076923076923,
0.846153846153845,0.86153846153846,0.876923076923076,0.892307692307691,
0.907692307692306,0.923076923076922,0.938461538461537,0.953846153846152,
0.969230769230768,0.984615384615383,0.994228156739709),.UNSPECIFIED.)
CURVE()
GEOMETRIC_REPRESENTATION_ITEM()
RATIONAL_B_SPLINE_CURVE((1.,1.,1.,1.,1.,1.,1.,1.,1.,1.,1.,1.,1.,1.,1.,1.,
1.,1.,1.,1.,1.,1.,1.,1.,1.,1.,1.,1.,1.,1.,1.,1.,1.,1.,1.,1.,1.,1.,1.,1.,
1.,1.,1.,1.,1.,1.,1.,1.,1.,1.,1.,1.,1.,1.,1.,1.,1.,1.,1.,1.,1.,1.,1.,1.,
1.,1.,1.,1.,1.,1.))
REPRESENTATION_ITEM('')
);
#261=(
BOUNDED_CURVE()
B_SPLINE_CURVE(5,(#33803,#33804,#33805,#33806,#33807,#33808,#33809,#33810,
#33811,#33812,#33813,#33814,#33815,#33816,#33817,#33818,#33819,#33820,#33821,
#33822,#33823,#33824,#33825,#33826,#33827,#33828,#33829,#33830,#33831,#33832,
#33833,#33834,#33835,#33836,#33837,#33838,#33839,#33840,#33841,#33842,#33843,
#33844,#33845,#33846,#33847,#33848,#33849,#33850,#33851,#33852,#33853,#33854,
#33855,#33856,#33857,#33858,#33859,#33860,#33861,#33862,#33863,#33864,#33865,
#33866,#33867,#33868,#33869,#33870,#33871,#33872),.UNSPECIFIED.,.F.,.F.)
B_SPLINE_CURVE_WITH_KNOTS((6,1,1,1,1,1,1,1,1,1,1,1,1,1,1,1,1,1,1,1,1,1,
1,1,1,1,1,1,1,1,1,1,1,1,1,1,1,1,1,1,1,1,1,1,1,1,1,1,1,1,1,1,1,1,1,1,1,1,
1,1,1,1,1,1,1,6),(0.00577184337451132,0.0153846153846154,0.0307692307692308,
0.0461538461538462,0.0615384615384615,0.0769230769230769,0.0923076923076923,
0.107692307692308,0.123076923076923,0.138461538461538,0.153846153846154,
0.169230769230769,0.184615384615385,0.2,0.215384615384615,0.230769230769231,
0.246153846153846,0.261538461538462,0.276923076923077,0.292307692307692,
0.307692307692308,0.323076923076923,0.338461538461538,0.353846153846154,
0.369230769230769,0.384615384615385,0.4,0.415384615384615,0.430769230769231,
0.446153846153846,0.461538461538462,0.476923076923077,0.492307692307692,
0.507692307692308,0.523076923076923,0.538461538461538,0.553846153846154,
0.569230769230769,0.584615384615384,0.6,0.615384615384615,0.63076923076923,
0.646153846153846,0.661538461538461,0.676923076923076,0.692307692307692,
0.707692307692307,0.723076923076922,0.738461538461538,0.753846153846153,
0.769230769230768,0.784615384615384,0.799999999999999,0.815384615384614,
0.83076923076923,0.846153846153845,0.86153846153846,0.876923076923076,0.892307692307691,
0.907692307692306,0.923076923076922,0.938461538461537,0.953846153846152,
0.969230769230768,0.984615384615383,1.),.UNSPECIFIED.)
CURVE()
GEOMETRIC_REPRESENTATION_ITEM()
RATIONAL_B_SPLINE_CURVE((1.,1.,1.,1.,1.,1.,1.,1.,1.,1.,1.,1.,1.,1.,1.,1.,
1.,1.,1.,1.,1.,1.,1.,1.,1.,1.,1.,1.,1.,1.,1.,1.,1.,1.,1.,1.,1.,1.,1.,1.,
1.,1.,1.,1.,1.,1.,1.,1.,1.,1.,1.,1.,1.,1.,1.,1.,1.,1.,1.,1.,1.,1.,1.,1.,
1.,1.,1.,1.,1.,1.))
REPRESENTATION_ITEM('')
);
#262=(
BOUNDED_CURVE()
B_SPLINE_CURVE(5,(#33876,#33877,#33878,#33879,#33880,#33881,#33882,#33883,
#33884,#33885,#33886,#33887,#33888,#33889,#33890,#33891,#33892,#33893,#33894,
#33895,#33896,#33897,#33898,#33899,#33900,#33901,#33902,#33903,#33904,#33905,
#33906,#33907,#33908,#33909,#33910,#33911,#33912,#33913,#33914,#33915,#33916,
#33917,#33918,#33919,#33920,#33921,#33922,#33923,#33924,#33925,#33926,#33927,
#33928,#33929,#33930,#33931,#33932,#33933,#33934,#33935,#33936,#33937,#33938,
#33939,#33940,#33941,#33942,#33943,#33944,#33945),.UNSPECIFIED.,.F.,.F.)
B_SPLINE_CURVE_WITH_KNOTS((6,1,1,1,1,1,1,1,1,1,1,1,1,1,1,1,1,1,1,1,1,1,
1,1,1,1,1,1,1,1,1,1,1,1,1,1,1,1,1,1,1,1,1,1,1,1,1,1,1,1,1,1,1,1,1,1,1,1,
1,1,1,1,1,1,1,6),(0.,0.0153846153846154,0.0307692307692308,0.0461538461538462,
0.0615384615384615,0.0769230769230769,0.0923076923076923,0.107692307692308,
0.123076923076923,0.138461538461538,0.153846153846154,0.169230769230769,
0.184615384615385,0.2,0.215384615384615,0.230769230769231,0.246153846153846,
0.261538461538462,0.276923076923077,0.292307692307692,0.307692307692308,
0.323076923076923,0.338461538461538,0.353846153846154,0.369230769230769,
0.384615384615385,0.4,0.415384615384615,0.430769230769231,0.446153846153846,
0.461538461538462,0.476923076923077,0.492307692307692,0.507692307692308,
0.523076923076923,0.538461538461538,0.553846153846154,0.569230769230769,
0.584615384615384,0.6,0.615384615384615,0.63076923076923,0.646153846153846,
0.661538461538461,0.676923076923076,0.692307692307692,0.707692307692307,
0.723076923076922,0.738461538461538,0.753846153846153,0.769230769230768,
0.784615384615384,0.799999999999999,0.815384615384614,0.83076923076923,
0.846153846153845,0.86153846153846,0.876923076923076,0.892307692307691,
0.907692307692306,0.923076923076922,0.938461538461537,0.953846153846152,
0.969230769230768,0.984615384615383,0.994228156739705),.UNSPECIFIED.)
CURVE()
GEOMETRIC_REPRESENTATION_ITEM()
RATIONAL_B_SPLINE_CURVE((1.,1.,1.,1.,1.,1.,1.,1.,1.,1.,1.,1.,1.,1.,1.,1.,
1.,1.,1.,1.,1.,1.,1.,1.,1.,1.,1.,1.,1.,1.,1.,1.,1.,1.,1.,1.,1.,1.,1.,1.,
1.,1.,1.,1.,1.,1.,1.,1.,1.,1.,1.,1.,1.,1.,1.,1.,1.,1.,1.,1.,1.,1.,1.,1.,
1.,1.,1.,1.,1.,1.))
REPRESENTATION_ITEM('')
);
#263=(
BOUNDED_CURVE()
B_SPLINE_CURVE(5,(#33949,#33950,#33951,#33952,#33953,#33954,#33955,#33956,
#33957,#33958,#33959,#33960,#33961,#33962,#33963,#33964,#33965,#33966,#33967,
#33968,#33969,#33970,#33971,#33972,#33973,#33974,#33975,#33976,#33977,#33978,
#33979,#33980,#33981,#33982,#33983,#33984,#33985,#33986,#33987,#33988,#33989,
#33990,#33991,#33992,#33993,#33994,#33995,#33996,#33997,#33998,#33999,#34000,
#34001,#34002,#34003,#34004,#34005,#34006,#34007,#34008,#34009,#34010,#34011,
#34012,#34013,#34014,#34015,#34016,#34017,#34018),.UNSPECIFIED.,.F.,.F.)
B_SPLINE_CURVE_WITH_KNOTS((6,1,1,1,1,1,1,1,1,1,1,1,1,1,1,1,1,1,1,1,1,1,
1,1,1,1,1,1,1,1,1,1,1,1,1,1,1,1,1,1,1,1,1,1,1,1,1,1,1,1,1,1,1,1,1,1,1,1,
1,1,1,1,1,1,1,6),(0.00577184337450072,0.0153846153846154,0.0307692307692308,
0.0461538461538462,0.0615384615384615,0.0769230769230769,0.0923076923076923,
0.107692307692308,0.123076923076923,0.138461538461538,0.153846153846154,
0.169230769230769,0.184615384615385,0.2,0.215384615384615,0.230769230769231,
0.246153846153846,0.261538461538462,0.276923076923077,0.292307692307692,
0.307692307692308,0.323076923076923,0.338461538461538,0.353846153846154,
0.369230769230769,0.384615384615385,0.4,0.415384615384615,0.430769230769231,
0.446153846153846,0.461538461538462,0.476923076923077,0.492307692307692,
0.507692307692308,0.523076923076923,0.538461538461538,0.553846153846154,
0.569230769230769,0.584615384615384,0.6,0.615384615384615,0.63076923076923,
0.646153846153846,0.661538461538461,0.676923076923076,0.692307692307692,
0.707692307692307,0.723076923076922,0.738461538461538,0.753846153846153,
0.769230769230768,0.784615384615384,0.799999999999999,0.815384615384614,
0.83076923076923,0.846153846153845,0.86153846153846,0.876923076923076,0.892307692307691,
0.907692307692306,0.923076923076922,0.938461538461537,0.953846153846152,
0.969230769230768,0.984615384615383,1.),.UNSPECIFIED.)
CURVE()
GEOMETRIC_REPRESENTATION_ITEM()
RATIONAL_B_SPLINE_CURVE((1.,1.,1.,1.,1.,1.,1.,1.,1.,1.,1.,1.,1.,1.,1.,1.,
1.,1.,1.,1.,1.,1.,1.,1.,1.,1.,1.,1.,1.,1.,1.,1.,1.,1.,1.,1.,1.,1.,1.,1.,
1.,1.,1.,1.,1.,1.,1.,1.,1.,1.,1.,1.,1.,1.,1.,1.,1.,1.,1.,1.,1.,1.,1.,1.,
1.,1.,1.,1.,1.,1.))
REPRESENTATION_ITEM('')
);
#264=(
BOUNDED_CURVE()
B_SPLINE_CURVE(5,(#34022,#34023,#34024,#34025,#34026,#34027,#34028,#34029,
#34030,#34031,#34032,#34033,#34034,#34035,#34036,#34037,#34038,#34039,#34040,
#34041,#34042,#34043,#34044,#34045,#34046,#34047,#34048,#34049,#34050,#34051,
#34052,#34053,#34054,#34055,#34056,#34057,#34058,#34059,#34060,#34061,#34062,
#34063,#34064,#34065,#34066,#34067,#34068,#34069,#34070,#34071,#34072,#34073,
#34074,#34075,#34076,#34077,#34078,#34079,#34080,#34081,#34082,#34083,#34084,
#34085,#34086,#34087,#34088,#34089,#34090,#34091),.UNSPECIFIED.,.F.,.F.)
B_SPLINE_CURVE_WITH_KNOTS((6,1,1,1,1,1,1,1,1,1,1,1,1,1,1,1,1,1,1,1,1,1,
1,1,1,1,1,1,1,1,1,1,1,1,1,1,1,1,1,1,1,1,1,1,1,1,1,1,1,1,1,1,1,1,1,1,1,1,
1,1,1,1,1,1,1,6),(0.,0.0153846153846154,0.0307692307692308,0.0461538461538462,
0.0615384615384615,0.0769230769230769,0.0923076923076923,0.107692307692308,
0.123076923076923,0.138461538461538,0.153846153846154,0.169230769230769,
0.184615384615385,0.2,0.215384615384615,0.230769230769231,0.246153846153846,
0.261538461538462,0.276923076923077,0.292307692307692,0.307692307692308,
0.323076923076923,0.338461538461538,0.353846153846154,0.369230769230769,
0.384615384615385,0.4,0.415384615384615,0.430769230769231,0.446153846153846,
0.461538461538462,0.476923076923077,0.492307692307692,0.507692307692308,
0.523076923076923,0.538461538461538,0.553846153846154,0.569230769230769,
0.584615384615384,0.6,0.615384615384615,0.63076923076923,0.646153846153846,
0.661538461538461,0.676923076923076,0.692307692307692,0.707692307692307,
0.723076923076922,0.738461538461538,0.753846153846153,0.769230769230768,
0.784615384615384,0.799999999999999,0.815384615384614,0.83076923076923,
0.846153846153845,0.86153846153846,0.876923076923076,0.892307692307691,
0.907692307692306,0.923076923076922,0.938461538461537,0.953846153846152,
0.969230769230768,0.984615384615383,0.994228156739706),.UNSPECIFIED.)
CURVE()
GEOMETRIC_REPRESENTATION_ITEM()
RATIONAL_B_SPLINE_CURVE((1.,1.,1.,1.,1.,1.,1.,1.,1.,1.,1.,1.,1.,1.,1.,1.,
1.,1.,1.,1.,1.,1.,1.,1.,1.,1.,1.,1.,1.,1.,1.,1.,1.,1.,1.,1.,1.,1.,1.,1.,
1.,1.,1.,1.,1.,1.,1.,1.,1.,1.,1.,1.,1.,1.,1.,1.,1.,1.,1.,1.,1.,1.,1.,1.,
1.,1.,1.,1.,1.,1.))
REPRESENTATION_ITEM('')
);
#265=(
BOUNDED_CURVE()
B_SPLINE_CURVE(5,(#34095,#34096,#34097,#34098,#34099,#34100,#34101,#34102,
#34103,#34104,#34105,#34106,#34107,#34108,#34109,#34110,#34111,#34112,#34113,
#34114,#34115,#34116,#34117,#34118,#34119,#34120,#34121,#34122,#34123,#34124,
#34125,#34126,#34127,#34128,#34129,#34130,#34131,#34132,#34133,#34134,#34135,
#34136,#34137,#34138,#34139,#34140,#34141,#34142,#34143,#34144,#34145,#34146,
#34147,#34148,#34149,#34150,#34151,#34152,#34153,#34154,#34155,#34156,#34157,
#34158,#34159,#34160,#34161,#34162,#34163,#34164),.UNSPECIFIED.,.F.,.F.)
B_SPLINE_CURVE_WITH_KNOTS((6,1,1,1,1,1,1,1,1,1,1,1,1,1,1,1,1,1,1,1,1,1,
1,1,1,1,1,1,1,1,1,1,1,1,1,1,1,1,1,1,1,1,1,1,1,1,1,1,1,1,1,1,1,1,1,1,1,1,
1,1,1,1,1,1,1,6),(0.00577184337450902,0.0153846153846154,0.0307692307692308,
0.0461538461538462,0.0615384615384615,0.0769230769230769,0.0923076923076923,
0.107692307692308,0.123076923076923,0.138461538461538,0.153846153846154,
0.169230769230769,0.184615384615385,0.2,0.215384615384615,0.230769230769231,
0.246153846153846,0.261538461538462,0.276923076923077,0.292307692307692,
0.307692307692308,0.323076923076923,0.338461538461538,0.353846153846154,
0.369230769230769,0.384615384615385,0.4,0.415384615384615,0.430769230769231,
0.446153846153846,0.461538461538462,0.476923076923077,0.492307692307692,
0.507692307692308,0.523076923076923,0.538461538461538,0.553846153846154,
0.569230769230769,0.584615384615384,0.6,0.615384615384615,0.63076923076923,
0.646153846153846,0.661538461538461,0.676923076923076,0.692307692307692,
0.707692307692307,0.723076923076922,0.738461538461538,0.753846153846153,
0.769230769230768,0.784615384615384,0.799999999999999,0.815384615384614,
0.83076923076923,0.846153846153845,0.86153846153846,0.876923076923076,0.892307692307691,
0.907692307692306,0.923076923076922,0.938461538461537,0.953846153846152,
0.969230769230768,0.984615384615383,1.),.UNSPECIFIED.)
CURVE()
GEOMETRIC_REPRESENTATION_ITEM()
RATIONAL_B_SPLINE_CURVE((1.,1.,1.,1.,1.,1.,1.,1.,1.,1.,1.,1.,1.,1.,1.,1.,
1.,1.,1.,1.,1.,1.,1.,1.,1.,1.,1.,1.,1.,1.,1.,1.,1.,1.,1.,1.,1.,1.,1.,1.,
1.,1.,1.,1.,1.,1.,1.,1.,1.,1.,1.,1.,1.,1.,1.,1.,1.,1.,1.,1.,1.,1.,1.,1.,
1.,1.,1.,1.,1.,1.))
REPRESENTATION_ITEM('')
);
#266=(
BOUNDED_CURVE()
B_SPLINE_CURVE(5,(#34168,#34169,#34170,#34171,#34172,#34173,#34174,#34175,
#34176,#34177,#34178,#34179,#34180,#34181,#34182,#34183,#34184,#34185,#34186,
#34187,#34188,#34189,#34190,#34191,#34192,#34193,#34194,#34195,#34196,#34197,
#34198,#34199,#34200,#34201,#34202,#34203,#34204,#34205,#34206,#34207,#34208,
#34209,#34210,#34211,#34212,#34213,#34214,#34215,#34216,#34217,#34218,#34219,
#34220,#34221,#34222,#34223,#34224,#34225,#34226,#34227,#34228,#34229,#34230,
#34231,#34232,#34233,#34234,#34235,#34236,#34237),.UNSPECIFIED.,.F.,.F.)
B_SPLINE_CURVE_WITH_KNOTS((6,1,1,1,1,1,1,1,1,1,1,1,1,1,1,1,1,1,1,1,1,1,
1,1,1,1,1,1,1,1,1,1,1,1,1,1,1,1,1,1,1,1,1,1,1,1,1,1,1,1,1,1,1,1,1,1,1,1,
1,1,1,1,1,1,1,6),(0.,0.0153846153846154,0.0307692307692308,0.0461538461538462,
0.0615384615384615,0.0769230769230769,0.0923076923076923,0.107692307692308,
0.123076923076923,0.138461538461538,0.153846153846154,0.169230769230769,
0.184615384615385,0.2,0.215384615384615,0.230769230769231,0.246153846153846,
0.261538461538462,0.276923076923077,0.292307692307692,0.307692307692308,
0.323076923076923,0.338461538461538,0.353846153846154,0.369230769230769,
0.384615384615385,0.4,0.415384615384615,0.430769230769231,0.446153846153846,
0.461538461538462,0.476923076923077,0.492307692307692,0.507692307692308,
0.523076923076923,0.538461538461538,0.553846153846154,0.569230769230769,
0.584615384615384,0.6,0.615384615384615,0.63076923076923,0.646153846153846,
0.661538461538461,0.676923076923076,0.692307692307692,0.707692307692307,
0.723076923076922,0.738461538461538,0.753846153846153,0.769230769230768,
0.784615384615384,0.799999999999999,0.815384615384614,0.83076923076923,
0.846153846153845,0.86153846153846,0.876923076923076,0.892307692307691,
0.907692307692306,0.923076923076922,0.938461538461537,0.953846153846152,
0.969230769230768,0.984615384615383,0.994228156739698),.UNSPECIFIED.)
CURVE()
GEOMETRIC_REPRESENTATION_ITEM()
RATIONAL_B_SPLINE_CURVE((1.,1.,1.,1.,1.,1.,1.,1.,1.,1.,1.,1.,1.,1.,1.,1.,
1.,1.,1.,1.,1.,1.,1.,1.,1.,1.,1.,1.,1.,1.,1.,1.,1.,1.,1.,1.,1.,1.,1.,1.,
1.,1.,1.,1.,1.,1.,1.,1.,1.,1.,1.,1.,1.,1.,1.,1.,1.,1.,1.,1.,1.,1.,1.,1.,
1.,1.,1.,1.,1.,1.))
REPRESENTATION_ITEM('')
);
#267=(
BOUNDED_CURVE()
B_SPLINE_CURVE(5,(#34241,#34242,#34243,#34244,#34245,#34246,#34247,#34248,
#34249,#34250,#34251,#34252,#34253,#34254,#34255,#34256,#34257,#34258,#34259,
#34260,#34261,#34262,#34263,#34264,#34265,#34266,#34267,#34268,#34269,#34270,
#34271,#34272,#34273,#34274,#34275,#34276,#34277,#34278,#34279,#34280,#34281,
#34282,#34283,#34284,#34285,#34286,#34287,#34288,#34289,#34290,#34291,#34292,
#34293,#34294,#34295,#34296,#34297,#34298,#34299,#34300,#34301,#34302,#34303,
#34304,#34305,#34306,#34307,#34308,#34309,#34310),.UNSPECIFIED.,.F.,.F.)
B_SPLINE_CURVE_WITH_KNOTS((6,1,1,1,1,1,1,1,1,1,1,1,1,1,1,1,1,1,1,1,1,1,
1,1,1,1,1,1,1,1,1,1,1,1,1,1,1,1,1,1,1,1,1,1,1,1,1,1,1,1,1,1,1,1,1,1,1,1,
1,1,1,1,1,1,1,6),(0.00577184337451611,0.0153846153846154,0.0307692307692308,
0.0461538461538462,0.0615384615384615,0.0769230769230769,0.0923076923076923,
0.107692307692308,0.123076923076923,0.138461538461538,0.153846153846154,
0.169230769230769,0.184615384615385,0.2,0.215384615384615,0.230769230769231,
0.246153846153846,0.261538461538462,0.276923076923077,0.292307692307692,
0.307692307692308,0.323076923076923,0.338461538461538,0.353846153846154,
0.369230769230769,0.384615384615385,0.4,0.415384615384615,0.430769230769231,
0.446153846153846,0.461538461538462,0.476923076923077,0.492307692307692,
0.507692307692308,0.523076923076923,0.538461538461538,0.553846153846154,
0.569230769230769,0.584615384615384,0.6,0.615384615384615,0.63076923076923,
0.646153846153846,0.661538461538461,0.676923076923076,0.692307692307692,
0.707692307692307,0.723076923076922,0.738461538461538,0.753846153846153,
0.769230769230768,0.784615384615384,0.799999999999999,0.815384615384614,
0.83076923076923,0.846153846153845,0.86153846153846,0.876923076923076,0.892307692307691,
0.907692307692306,0.923076923076922,0.938461538461537,0.953846153846152,
0.969230769230768,0.984615384615383,1.),.UNSPECIFIED.)
CURVE()
GEOMETRIC_REPRESENTATION_ITEM()
RATIONAL_B_SPLINE_CURVE((1.,1.,1.,1.,1.,1.,1.,1.,1.,1.,1.,1.,1.,1.,1.,1.,
1.,1.,1.,1.,1.,1.,1.,1.,1.,1.,1.,1.,1.,1.,1.,1.,1.,1.,1.,1.,1.,1.,1.,1.,
1.,1.,1.,1.,1.,1.,1.,1.,1.,1.,1.,1.,1.,1.,1.,1.,1.,1.,1.,1.,1.,1.,1.,1.,
1.,1.,1.,1.,1.,1.))
REPRESENTATION_ITEM('')
);
#268=(
BOUNDED_CURVE()
B_SPLINE_CURVE(5,(#34314,#34315,#34316,#34317,#34318,#34319,#34320,#34321,
#34322,#34323,#34324,#34325,#34326,#34327,#34328,#34329,#34330,#34331,#34332,
#34333,#34334,#34335,#34336,#34337,#34338,#34339,#34340,#34341,#34342,#34343,
#34344,#34345,#34346,#34347,#34348,#34349,#34350,#34351,#34352,#34353,#34354,
#34355,#34356,#34357,#34358,#34359,#34360,#34361,#34362,#34363,#34364,#34365,
#34366,#34367,#34368,#34369,#34370,#34371,#34372,#34373,#34374,#34375,#34376,
#34377,#34378,#34379,#34380,#34381,#34382,#34383),.UNSPECIFIED.,.F.,.F.)
B_SPLINE_CURVE_WITH_KNOTS((6,1,1,1,1,1,1,1,1,1,1,1,1,1,1,1,1,1,1,1,1,1,
1,1,1,1,1,1,1,1,1,1,1,1,1,1,1,1,1,1,1,1,1,1,1,1,1,1,1,1,1,1,1,1,1,1,1,1,
1,1,1,1,1,1,1,6),(0.,0.0153846153846154,0.0307692307692308,0.0461538461538462,
0.0615384615384615,0.0769230769230769,0.0923076923076923,0.107692307692308,
0.123076923076923,0.138461538461538,0.153846153846154,0.169230769230769,
0.184615384615385,0.2,0.215384615384615,0.230769230769231,0.246153846153846,
0.261538461538462,0.276923076923077,0.292307692307692,0.307692307692308,
0.323076923076923,0.338461538461538,0.353846153846154,0.369230769230769,
0.384615384615385,0.4,0.415384615384615,0.430769230769231,0.446153846153846,
0.461538461538462,0.476923076923077,0.492307692307692,0.507692307692308,
0.523076923076923,0.538461538461538,0.553846153846154,0.569230769230769,
0.584615384615384,0.6,0.615384615384615,0.63076923076923,0.646153846153846,
0.661538461538461,0.676923076923076,0.692307692307692,0.707692307692307,
0.723076923076922,0.738461538461538,0.753846153846153,0.769230769230768,
0.784615384615384,0.799999999999999,0.815384615384614,0.83076923076923,
0.846153846153845,0.86153846153846,0.876923076923076,0.892307692307691,
0.907692307692306,0.923076923076922,0.938461538461537,0.953846153846152,
0.969230769230768,0.984615384615383,0.994228156739704),.UNSPECIFIED.)
CURVE()
GEOMETRIC_REPRESENTATION_ITEM()
RATIONAL_B_SPLINE_CURVE((1.,1.,1.,1.,1.,1.,1.,1.,1.,1.,1.,1.,1.,1.,1.,1.,
1.,1.,1.,1.,1.,1.,1.,1.,1.,1.,1.,1.,1.,1.,1.,1.,1.,1.,1.,1.,1.,1.,1.,1.,
1.,1.,1.,1.,1.,1.,1.,1.,1.,1.,1.,1.,1.,1.,1.,1.,1.,1.,1.,1.,1.,1.,1.,1.,
1.,1.,1.,1.,1.,1.))
REPRESENTATION_ITEM('')
);
#269=(
BOUNDED_CURVE()
B_SPLINE_CURVE(5,(#34387,#34388,#34389,#34390,#34391,#34392,#34393,#34394,
#34395,#34396,#34397,#34398,#34399,#34400,#34401,#34402,#34403,#34404,#34405,
#34406,#34407,#34408,#34409,#34410,#34411,#34412,#34413,#34414,#34415,#34416,
#34417,#34418,#34419,#34420,#34421,#34422,#34423,#34424,#34425,#34426,#34427,
#34428,#34429,#34430,#34431,#34432,#34433,#34434,#34435,#34436,#34437,#34438,
#34439,#34440,#34441,#34442,#34443,#34444,#34445,#34446,#34447,#34448,#34449,
#34450,#34451,#34452,#34453,#34454,#34455,#34456),.UNSPECIFIED.,.F.,.F.)
B_SPLINE_CURVE_WITH_KNOTS((6,1,1,1,1,1,1,1,1,1,1,1,1,1,1,1,1,1,1,1,1,1,
1,1,1,1,1,1,1,1,1,1,1,1,1,1,1,1,1,1,1,1,1,1,1,1,1,1,1,1,1,1,1,1,1,1,1,1,
1,1,1,1,1,1,1,6),(0.00577184337449682,0.0153846153846154,0.0307692307692308,
0.0461538461538462,0.0615384615384615,0.0769230769230769,0.0923076923076923,
0.107692307692308,0.123076923076923,0.138461538461538,0.153846153846154,
0.169230769230769,0.184615384615385,0.2,0.215384615384615,0.230769230769231,
0.246153846153846,0.261538461538462,0.276923076923077,0.292307692307692,
0.307692307692308,0.323076923076923,0.338461538461538,0.353846153846154,
0.369230769230769,0.384615384615385,0.4,0.415384615384615,0.430769230769231,
0.446153846153846,0.461538461538462,0.476923076923077,0.492307692307692,
0.507692307692308,0.523076923076923,0.538461538461538,0.553846153846154,
0.569230769230769,0.584615384615384,0.6,0.615384615384615,0.63076923076923,
0.646153846153846,0.661538461538461,0.676923076923076,0.692307692307692,
0.707692307692307,0.723076923076922,0.738461538461538,0.753846153846153,
0.769230769230768,0.784615384615384,0.799999999999999,0.815384615384614,
0.83076923076923,0.846153846153845,0.86153846153846,0.876923076923076,0.892307692307691,
0.907692307692306,0.923076923076922,0.938461538461537,0.953846153846152,
0.969230769230768,0.984615384615383,1.),.UNSPECIFIED.)
CURVE()
GEOMETRIC_REPRESENTATION_ITEM()
RATIONAL_B_SPLINE_CURVE((1.,1.,1.,1.,1.,1.,1.,1.,1.,1.,1.,1.,1.,1.,1.,1.,
1.,1.,1.,1.,1.,1.,1.,1.,1.,1.,1.,1.,1.,1.,1.,1.,1.,1.,1.,1.,1.,1.,1.,1.,
1.,1.,1.,1.,1.,1.,1.,1.,1.,1.,1.,1.,1.,1.,1.,1.,1.,1.,1.,1.,1.,1.,1.,1.,
1.,1.,1.,1.,1.,1.))
REPRESENTATION_ITEM('')
);
#270=(
BOUNDED_CURVE()
B_SPLINE_CURVE(5,(#34460,#34461,#34462,#34463,#34464,#34465,#34466,#34467,
#34468,#34469,#34470,#34471,#34472,#34473,#34474,#34475,#34476,#34477,#34478,
#34479,#34480,#34481,#34482,#34483,#34484,#34485,#34486,#34487,#34488,#34489,
#34490,#34491,#34492,#34493,#34494,#34495,#34496,#34497,#34498,#34499,#34500,
#34501,#34502,#34503,#34504,#34505,#34506,#34507,#34508,#34509,#34510,#34511,
#34512,#34513,#34514,#34515,#34516,#34517,#34518,#34519,#34520,#34521,#34522,
#34523,#34524,#34525,#34526,#34527,#34528,#34529),.UNSPECIFIED.,.F.,.F.)
B_SPLINE_CURVE_WITH_KNOTS((6,1,1,1,1,1,1,1,1,1,1,1,1,1,1,1,1,1,1,1,1,1,
1,1,1,1,1,1,1,1,1,1,1,1,1,1,1,1,1,1,1,1,1,1,1,1,1,1,1,1,1,1,1,1,1,1,1,1,
1,1,1,1,1,1,1,6),(0.,0.0153846153846154,0.0307692307692308,0.0461538461538462,
0.0615384615384615,0.0769230769230769,0.0923076923076923,0.107692307692308,
0.123076923076923,0.138461538461538,0.153846153846154,0.169230769230769,
0.184615384615385,0.2,0.215384615384615,0.230769230769231,0.246153846153846,
0.261538461538462,0.276923076923077,0.292307692307692,0.307692307692308,
0.323076923076923,0.338461538461538,0.353846153846154,0.369230769230769,
0.384615384615385,0.4,0.415384615384615,0.430769230769231,0.446153846153846,
0.461538461538462,0.476923076923077,0.492307692307692,0.507692307692308,
0.523076923076923,0.538461538461538,0.553846153846154,0.569230769230769,
0.584615384615384,0.6,0.615384615384615,0.63076923076923,0.646153846153846,
0.661538461538461,0.676923076923076,0.692307692307692,0.707692307692307,
0.723076923076922,0.738461538461538,0.753846153846153,0.769230769230768,
0.784615384615384,0.799999999999999,0.815384615384614,0.83076923076923,
0.846153846153845,0.86153846153846,0.876923076923076,0.892307692307691,
0.907692307692306,0.923076923076922,0.938461538461537,0.953846153846152,
0.969230769230768,0.984615384615383,0.994228156739711),.UNSPECIFIED.)
CURVE()
GEOMETRIC_REPRESENTATION_ITEM()
RATIONAL_B_SPLINE_CURVE((1.,1.,1.,1.,1.,1.,1.,1.,1.,1.,1.,1.,1.,1.,1.,1.,
1.,1.,1.,1.,1.,1.,1.,1.,1.,1.,1.,1.,1.,1.,1.,1.,1.,1.,1.,1.,1.,1.,1.,1.,
1.,1.,1.,1.,1.,1.,1.,1.,1.,1.,1.,1.,1.,1.,1.,1.,1.,1.,1.,1.,1.,1.,1.,1.,
1.,1.,1.,1.,1.,1.))
REPRESENTATION_ITEM('')
);
#271=(
BOUNDED_CURVE()
B_SPLINE_CURVE(5,(#34533,#34534,#34535,#34536,#34537,#34538,#34539,#34540,
#34541,#34542,#34543,#34544,#34545,#34546,#34547,#34548,#34549,#34550,#34551,
#34552,#34553,#34554,#34555,#34556,#34557,#34558,#34559,#34560,#34561,#34562,
#34563,#34564,#34565,#34566,#34567,#34568,#34569,#34570,#34571,#34572,#34573,
#34574,#34575,#34576,#34577,#34578,#34579,#34580,#34581,#34582,#34583,#34584,
#34585,#34586,#34587,#34588,#34589,#34590,#34591,#34592,#34593,#34594,#34595,
#34596,#34597,#34598,#34599,#34600,#34601,#34602),.UNSPECIFIED.,.F.,.F.)
B_SPLINE_CURVE_WITH_KNOTS((6,1,1,1,1,1,1,1,1,1,1,1,1,1,1,1,1,1,1,1,1,1,
1,1,1,1,1,1,1,1,1,1,1,1,1,1,1,1,1,1,1,1,1,1,1,1,1,1,1,1,1,1,1,1,1,1,1,1,
1,1,1,1,1,1,1,6),(0.00577184337449159,0.0153846153846154,0.0307692307692308,
0.0461538461538462,0.0615384615384615,0.0769230769230769,0.0923076923076923,
0.107692307692308,0.123076923076923,0.138461538461538,0.153846153846154,
0.169230769230769,0.184615384615385,0.2,0.215384615384615,0.230769230769231,
0.246153846153846,0.261538461538462,0.276923076923077,0.292307692307692,
0.307692307692308,0.323076923076923,0.338461538461538,0.353846153846154,
0.369230769230769,0.384615384615385,0.4,0.415384615384615,0.430769230769231,
0.446153846153846,0.461538461538462,0.476923076923077,0.492307692307692,
0.507692307692308,0.523076923076923,0.538461538461538,0.553846153846154,
0.569230769230769,0.584615384615384,0.6,0.615384615384615,0.63076923076923,
0.646153846153846,0.661538461538461,0.676923076923076,0.692307692307692,
0.707692307692307,0.723076923076922,0.738461538461538,0.753846153846153,
0.769230769230768,0.784615384615384,0.799999999999999,0.815384615384614,
0.83076923076923,0.846153846153845,0.86153846153846,0.876923076923076,0.892307692307691,
0.907692307692306,0.923076923076922,0.938461538461537,0.953846153846152,
0.969230769230768,0.984615384615383,1.),.UNSPECIFIED.)
CURVE()
GEOMETRIC_REPRESENTATION_ITEM()
RATIONAL_B_SPLINE_CURVE((1.,1.,1.,1.,1.,1.,1.,1.,1.,1.,1.,1.,1.,1.,1.,1.,
1.,1.,1.,1.,1.,1.,1.,1.,1.,1.,1.,1.,1.,1.,1.,1.,1.,1.,1.,1.,1.,1.,1.,1.,
1.,1.,1.,1.,1.,1.,1.,1.,1.,1.,1.,1.,1.,1.,1.,1.,1.,1.,1.,1.,1.,1.,1.,1.,
1.,1.,1.,1.,1.,1.))
REPRESENTATION_ITEM('')
);
#272=(
BOUNDED_CURVE()
B_SPLINE_CURVE(5,(#34606,#34607,#34608,#34609,#34610,#34611,#34612,#34613,
#34614,#34615,#34616,#34617,#34618,#34619,#34620,#34621,#34622,#34623,#34624,
#34625,#34626,#34627,#34628,#34629,#34630,#34631,#34632,#34633,#34634,#34635,
#34636,#34637,#34638,#34639,#34640,#34641,#34642,#34643,#34644,#34645,#34646,
#34647,#34648,#34649,#34650,#34651,#34652,#34653,#34654,#34655,#34656,#34657,
#34658,#34659,#34660,#34661,#34662,#34663,#34664,#34665,#34666,#34667,#34668,
#34669,#34670,#34671,#34672,#34673,#34674,#34675),.UNSPECIFIED.,.F.,.F.)
B_SPLINE_CURVE_WITH_KNOTS((6,1,1,1,1,1,1,1,1,1,1,1,1,1,1,1,1,1,1,1,1,1,
1,1,1,1,1,1,1,1,1,1,1,1,1,1,1,1,1,1,1,1,1,1,1,1,1,1,1,1,1,1,1,1,1,1,1,1,
1,1,1,1,1,1,1,6),(0.,0.0153846153846154,0.0307692307692308,0.0461538461538462,
0.0615384615384615,0.0769230769230769,0.0923076923076923,0.107692307692308,
0.123076923076923,0.138461538461538,0.153846153846154,0.169230769230769,
0.184615384615385,0.2,0.215384615384615,0.230769230769231,0.246153846153846,
0.261538461538462,0.276923076923077,0.292307692307692,0.307692307692308,
0.323076923076923,0.338461538461538,0.353846153846154,0.369230769230769,
0.384615384615385,0.4,0.415384615384615,0.430769230769231,0.446153846153846,
0.461538461538462,0.476923076923077,0.492307692307692,0.507692307692308,
0.523076923076923,0.538461538461538,0.553846153846154,0.569230769230769,
0.584615384615384,0.6,0.615384615384615,0.63076923076923,0.646153846153846,
0.661538461538461,0.676923076923076,0.692307692307692,0.707692307692307,
0.723076923076922,0.738461538461538,0.753846153846153,0.769230769230768,
0.784615384615384,0.799999999999999,0.815384615384614,0.83076923076923,
0.846153846153845,0.86153846153846,0.876923076923076,0.892307692307691,
0.907692307692306,0.923076923076922,0.938461538461537,0.953846153846152,
0.969230769230768,0.984615384615383,0.994228156739723),.UNSPECIFIED.)
CURVE()
GEOMETRIC_REPRESENTATION_ITEM()
RATIONAL_B_SPLINE_CURVE((1.,1.,1.,1.,1.,1.,1.,1.,1.,1.,1.,1.,1.,1.,1.,1.,
1.,1.,1.,1.,1.,1.,1.,1.,1.,1.,1.,1.,1.,1.,1.,1.,1.,1.,1.,1.,1.,1.,1.,1.,
1.,1.,1.,1.,1.,1.,1.,1.,1.,1.,1.,1.,1.,1.,1.,1.,1.,1.,1.,1.,1.,1.,1.,1.,
1.,1.,1.,1.,1.,1.))
REPRESENTATION_ITEM('')
);
#273=(
BOUNDED_CURVE()
B_SPLINE_CURVE(5,(#34679,#34680,#34681,#34682,#34683,#34684,#34685,#34686,
#34687,#34688,#34689,#34690,#34691,#34692,#34693,#34694,#34695,#34696,#34697,
#34698,#34699,#34700,#34701,#34702,#34703,#34704,#34705,#34706,#34707,#34708,
#34709,#34710,#34711,#34712,#34713,#34714,#34715,#34716,#34717,#34718,#34719,
#34720,#34721,#34722,#34723,#34724,#34725,#34726,#34727,#34728,#34729,#34730,
#34731,#34732,#34733,#34734,#34735,#34736,#34737,#34738,#34739,#34740,#34741,
#34742,#34743,#34744,#34745,#34746,#34747,#34748),.UNSPECIFIED.,.F.,.F.)
B_SPLINE_CURVE_WITH_KNOTS((6,1,1,1,1,1,1,1,1,1,1,1,1,1,1,1,1,1,1,1,1,1,
1,1,1,1,1,1,1,1,1,1,1,1,1,1,1,1,1,1,1,1,1,1,1,1,1,1,1,1,1,1,1,1,1,1,1,1,
1,1,1,1,1,1,1,6),(0.00577184337450718,0.0153846153846154,0.0307692307692308,
0.0461538461538462,0.0615384615384615,0.0769230769230769,0.0923076923076923,
0.107692307692308,0.123076923076923,0.138461538461538,0.153846153846154,
0.169230769230769,0.184615384615385,0.2,0.215384615384615,0.230769230769231,
0.246153846153846,0.261538461538462,0.276923076923077,0.292307692307692,
0.307692307692308,0.323076923076923,0.338461538461538,0.353846153846154,
0.369230769230769,0.384615384615385,0.4,0.415384615384615,0.430769230769231,
0.446153846153846,0.461538461538462,0.476923076923077,0.492307692307692,
0.507692307692308,0.523076923076923,0.538461538461538,0.553846153846154,
0.569230769230769,0.584615384615384,0.6,0.615384615384615,0.63076923076923,
0.646153846153846,0.661538461538461,0.676923076923076,0.692307692307692,
0.707692307692307,0.723076923076922,0.738461538461538,0.753846153846153,
0.769230769230768,0.784615384615384,0.799999999999999,0.815384615384614,
0.83076923076923,0.846153846153845,0.86153846153846,0.876923076923076,0.892307692307691,
0.907692307692306,0.923076923076922,0.938461538461537,0.953846153846152,
0.969230769230768,0.984615384615383,1.),.UNSPECIFIED.)
CURVE()
GEOMETRIC_REPRESENTATION_ITEM()
RATIONAL_B_SPLINE_CURVE((1.,1.,1.,1.,1.,1.,1.,1.,1.,1.,1.,1.,1.,1.,1.,1.,
1.,1.,1.,1.,1.,1.,1.,1.,1.,1.,1.,1.,1.,1.,1.,1.,1.,1.,1.,1.,1.,1.,1.,1.,
1.,1.,1.,1.,1.,1.,1.,1.,1.,1.,1.,1.,1.,1.,1.,1.,1.,1.,1.,1.,1.,1.,1.,1.,
1.,1.,1.,1.,1.,1.))
REPRESENTATION_ITEM('')
);
#274=(
BOUNDED_CURVE()
B_SPLINE_CURVE(5,(#34752,#34753,#34754,#34755,#34756,#34757,#34758,#34759,
#34760,#34761,#34762,#34763,#34764,#34765,#34766,#34767,#34768,#34769,#34770,
#34771,#34772,#34773,#34774,#34775,#34776,#34777,#34778,#34779,#34780,#34781,
#34782,#34783,#34784,#34785,#34786,#34787,#34788,#34789,#34790,#34791,#34792,
#34793,#34794,#34795,#34796,#34797,#34798,#34799,#34800,#34801,#34802,#34803,
#34804,#34805,#34806,#34807,#34808,#34809,#34810,#34811,#34812,#34813,#34814,
#34815,#34816,#34817,#34818,#34819,#34820,#34821),.UNSPECIFIED.,.F.,.F.)
B_SPLINE_CURVE_WITH_KNOTS((6,1,1,1,1,1,1,1,1,1,1,1,1,1,1,1,1,1,1,1,1,1,
1,1,1,1,1,1,1,1,1,1,1,1,1,1,1,1,1,1,1,1,1,1,1,1,1,1,1,1,1,1,1,1,1,1,1,1,
1,1,1,1,1,1,1,6),(0.,0.0153846153846154,0.0307692307692308,0.0461538461538462,
0.0615384615384615,0.0769230769230769,0.0923076923076923,0.107692307692308,
0.123076923076923,0.138461538461538,0.153846153846154,0.169230769230769,
0.184615384615385,0.2,0.215384615384615,0.230769230769231,0.246153846153846,
0.261538461538462,0.276923076923077,0.292307692307692,0.307692307692308,
0.323076923076923,0.338461538461538,0.353846153846154,0.369230769230769,
0.384615384615385,0.4,0.415384615384615,0.430769230769231,0.446153846153846,
0.461538461538462,0.476923076923077,0.492307692307692,0.507692307692308,
0.523076923076923,0.538461538461538,0.553846153846154,0.569230769230769,
0.584615384615384,0.6,0.615384615384615,0.63076923076923,0.646153846153846,
0.661538461538461,0.676923076923076,0.692307692307692,0.707692307692307,
0.723076923076922,0.738461538461538,0.753846153846153,0.769230769230768,
0.784615384615384,0.799999999999999,0.815384615384614,0.83076923076923,
0.846153846153845,0.86153846153846,0.876923076923076,0.892307692307691,
0.907692307692306,0.923076923076922,0.938461538461537,0.953846153846152,
0.969230769230768,0.984615384615383,0.994228156739716),.UNSPECIFIED.)
CURVE()
GEOMETRIC_REPRESENTATION_ITEM()
RATIONAL_B_SPLINE_CURVE((1.,1.,1.,1.,1.,1.,1.,1.,1.,1.,1.,1.,1.,1.,1.,1.,
1.,1.,1.,1.,1.,1.,1.,1.,1.,1.,1.,1.,1.,1.,1.,1.,1.,1.,1.,1.,1.,1.,1.,1.,
1.,1.,1.,1.,1.,1.,1.,1.,1.,1.,1.,1.,1.,1.,1.,1.,1.,1.,1.,1.,1.,1.,1.,1.,
1.,1.,1.,1.,1.,1.))
REPRESENTATION_ITEM('')
);
#275=(
BOUNDED_CURVE()
B_SPLINE_CURVE(5,(#34825,#34826,#34827,#34828,#34829,#34830,#34831,#34832,
#34833,#34834,#34835,#34836,#34837,#34838,#34839,#34840,#34841,#34842,#34843,
#34844,#34845,#34846,#34847,#34848,#34849,#34850,#34851,#34852,#34853,#34854,
#34855,#34856,#34857,#34858,#34859,#34860,#34861,#34862,#34863,#34864,#34865,
#34866,#34867,#34868,#34869,#34870,#34871,#34872,#34873,#34874,#34875,#34876,
#34877,#34878,#34879,#34880,#34881,#34882,#34883,#34884,#34885,#34886,#34887,
#34888,#34889,#34890,#34891,#34892,#34893,#34894),.UNSPECIFIED.,.F.,.F.)
B_SPLINE_CURVE_WITH_KNOTS((6,1,1,1,1,1,1,1,1,1,1,1,1,1,1,1,1,1,1,1,1,1,
1,1,1,1,1,1,1,1,1,1,1,1,1,1,1,1,1,1,1,1,1,1,1,1,1,1,1,1,1,1,1,1,1,1,1,1,
1,1,1,1,1,1,1,6),(0.00577184337450174,0.0153846153846154,0.0307692307692308,
0.0461538461538462,0.0615384615384615,0.0769230769230769,0.0923076923076923,
0.107692307692308,0.123076923076923,0.138461538461538,0.153846153846154,
0.169230769230769,0.184615384615385,0.2,0.215384615384615,0.230769230769231,
0.246153846153846,0.261538461538462,0.276923076923077,0.292307692307692,
0.307692307692308,0.323076923076923,0.338461538461538,0.353846153846154,
0.369230769230769,0.384615384615385,0.4,0.415384615384615,0.430769230769231,
0.446153846153846,0.461538461538462,0.476923076923077,0.492307692307692,
0.507692307692308,0.523076923076923,0.538461538461538,0.553846153846154,
0.569230769230769,0.584615384615384,0.6,0.615384615384615,0.63076923076923,
0.646153846153846,0.661538461538461,0.676923076923076,0.692307692307692,
0.707692307692307,0.723076923076922,0.738461538461538,0.753846153846153,
0.769230769230768,0.784615384615384,0.799999999999999,0.815384615384614,
0.83076923076923,0.846153846153845,0.86153846153846,0.876923076923076,0.892307692307691,
0.907692307692306,0.923076923076922,0.938461538461537,0.953846153846152,
0.969230769230768,0.984615384615383,1.),.UNSPECIFIED.)
CURVE()
GEOMETRIC_REPRESENTATION_ITEM()
RATIONAL_B_SPLINE_CURVE((1.,1.,1.,1.,1.,1.,1.,1.,1.,1.,1.,1.,1.,1.,1.,1.,
1.,1.,1.,1.,1.,1.,1.,1.,1.,1.,1.,1.,1.,1.,1.,1.,1.,1.,1.,1.,1.,1.,1.,1.,
1.,1.,1.,1.,1.,1.,1.,1.,1.,1.,1.,1.,1.,1.,1.,1.,1.,1.,1.,1.,1.,1.,1.,1.,
1.,1.,1.,1.,1.,1.))
REPRESENTATION_ITEM('')
);
#276=(
BOUNDED_CURVE()
B_SPLINE_CURVE(5,(#34898,#34899,#34900,#34901,#34902,#34903,#34904,#34905,
#34906,#34907,#34908,#34909,#34910,#34911,#34912,#34913,#34914,#34915,#34916,
#34917,#34918,#34919,#34920,#34921,#34922,#34923,#34924,#34925,#34926,#34927,
#34928,#34929,#34930,#34931,#34932,#34933,#34934,#34935,#34936,#34937,#34938,
#34939,#34940,#34941,#34942,#34943,#34944,#34945,#34946,#34947,#34948,#34949,
#34950,#34951,#34952,#34953,#34954,#34955,#34956,#34957,#34958,#34959,#34960,
#34961,#34962,#34963,#34964,#34965,#34966,#34967),.UNSPECIFIED.,.F.,.F.)
B_SPLINE_CURVE_WITH_KNOTS((6,1,1,1,1,1,1,1,1,1,1,1,1,1,1,1,1,1,1,1,1,1,
1,1,1,1,1,1,1,1,1,1,1,1,1,1,1,1,1,1,1,1,1,1,1,1,1,1,1,1,1,1,1,1,1,1,1,1,
1,1,1,1,1,1,1,6),(0.,0.0153846153846154,0.0307692307692308,0.0461538461538462,
0.0615384615384615,0.0769230769230769,0.0923076923076923,0.107692307692308,
0.123076923076923,0.138461538461538,0.153846153846154,0.169230769230769,
0.184615384615385,0.2,0.215384615384615,0.230769230769231,0.246153846153846,
0.261538461538462,0.276923076923077,0.292307692307692,0.307692307692308,
0.323076923076923,0.338461538461538,0.353846153846154,0.369230769230769,
0.384615384615385,0.4,0.415384615384615,0.430769230769231,0.446153846153846,
0.461538461538462,0.476923076923077,0.492307692307692,0.507692307692308,
0.523076923076923,0.538461538461538,0.553846153846154,0.569230769230769,
0.584615384615384,0.6,0.615384615384615,0.63076923076923,0.646153846153846,
0.661538461538461,0.676923076923076,0.692307692307692,0.707692307692307,
0.723076923076922,0.738461538461538,0.753846153846153,0.769230769230768,
0.784615384615384,0.799999999999999,0.815384615384614,0.83076923076923,
0.846153846153845,0.86153846153846,0.876923076923076,0.892307692307691,
0.907692307692306,0.923076923076922,0.938461538461537,0.953846153846152,
0.969230769230768,0.984615384615383,0.994228156739722),.UNSPECIFIED.)
CURVE()
GEOMETRIC_REPRESENTATION_ITEM()
RATIONAL_B_SPLINE_CURVE((1.,1.,1.,1.,1.,1.,1.,1.,1.,1.,1.,1.,1.,1.,1.,1.,
1.,1.,1.,1.,1.,1.,1.,1.,1.,1.,1.,1.,1.,1.,1.,1.,1.,1.,1.,1.,1.,1.,1.,1.,
1.,1.,1.,1.,1.,1.,1.,1.,1.,1.,1.,1.,1.,1.,1.,1.,1.,1.,1.,1.,1.,1.,1.,1.,
1.,1.,1.,1.,1.,1.))
REPRESENTATION_ITEM('')
);
#277=(
BOUNDED_CURVE()
B_SPLINE_CURVE(5,(#34971,#34972,#34973,#34974,#34975,#34976,#34977,#34978,
#34979,#34980,#34981,#34982,#34983,#34984,#34985,#34986,#34987,#34988,#34989,
#34990,#34991,#34992,#34993,#34994,#34995,#34996,#34997,#34998,#34999,#35000,
#35001,#35002,#35003,#35004,#35005,#35006,#35007,#35008,#35009,#35010,#35011,
#35012,#35013,#35014,#35015,#35016,#35017,#35018,#35019,#35020,#35021,#35022,
#35023,#35024,#35025,#35026,#35027,#35028,#35029,#35030,#35031,#35032,#35033,
#35034,#35035,#35036,#35037,#35038,#35039,#35040),.UNSPECIFIED.,.F.,.F.)
B_SPLINE_CURVE_WITH_KNOTS((6,1,1,1,1,1,1,1,1,1,1,1,1,1,1,1,1,1,1,1,1,1,
1,1,1,1,1,1,1,1,1,1,1,1,1,1,1,1,1,1,1,1,1,1,1,1,1,1,1,1,1,1,1,1,1,1,1,1,
1,1,1,1,1,1,1,6),(0.00577184337450943,0.0153846153846154,0.0307692307692308,
0.0461538461538462,0.0615384615384615,0.0769230769230769,0.0923076923076923,
0.107692307692308,0.123076923076923,0.138461538461538,0.153846153846154,
0.169230769230769,0.184615384615385,0.2,0.215384615384615,0.230769230769231,
0.246153846153846,0.261538461538462,0.276923076923077,0.292307692307692,
0.307692307692308,0.323076923076923,0.338461538461538,0.353846153846154,
0.369230769230769,0.384615384615385,0.4,0.415384615384615,0.430769230769231,
0.446153846153846,0.461538461538462,0.476923076923077,0.492307692307692,
0.507692307692308,0.523076923076923,0.538461538461538,0.553846153846154,
0.569230769230769,0.584615384615384,0.6,0.615384615384615,0.63076923076923,
0.646153846153846,0.661538461538461,0.676923076923076,0.692307692307692,
0.707692307692307,0.723076923076922,0.738461538461538,0.753846153846153,
0.769230769230768,0.784615384615384,0.799999999999999,0.815384615384614,
0.83076923076923,0.846153846153845,0.86153846153846,0.876923076923076,0.892307692307691,
0.907692307692306,0.923076923076922,0.938461538461537,0.953846153846152,
0.969230769230768,0.984615384615383,1.),.UNSPECIFIED.)
CURVE()
GEOMETRIC_REPRESENTATION_ITEM()
RATIONAL_B_SPLINE_CURVE((1.,1.,1.,1.,1.,1.,1.,1.,1.,1.,1.,1.,1.,1.,1.,1.,
1.,1.,1.,1.,1.,1.,1.,1.,1.,1.,1.,1.,1.,1.,1.,1.,1.,1.,1.,1.,1.,1.,1.,1.,
1.,1.,1.,1.,1.,1.,1.,1.,1.,1.,1.,1.,1.,1.,1.,1.,1.,1.,1.,1.,1.,1.,1.,1.,
1.,1.,1.,1.,1.,1.))
REPRESENTATION_ITEM('')
);
#278=(
BOUNDED_CURVE()
B_SPLINE_CURVE(5,(#35044,#35045,#35046,#35047,#35048,#35049,#35050,#35051,
#35052,#35053,#35054,#35055,#35056,#35057,#35058,#35059,#35060,#35061,#35062,
#35063,#35064,#35065,#35066,#35067,#35068,#35069,#35070,#35071,#35072,#35073,
#35074,#35075,#35076,#35077,#35078,#35079,#35080,#35081,#35082,#35083,#35084,
#35085,#35086,#35087,#35088,#35089,#35090,#35091,#35092,#35093,#35094,#35095,
#35096,#35097,#35098,#35099,#35100,#35101,#35102,#35103,#35104,#35105,#35106,
#35107,#35108,#35109,#35110,#35111,#35112,#35113),.UNSPECIFIED.,.F.,.F.)
B_SPLINE_CURVE_WITH_KNOTS((6,1,1,1,1,1,1,1,1,1,1,1,1,1,1,1,1,1,1,1,1,1,
1,1,1,1,1,1,1,1,1,1,1,1,1,1,1,1,1,1,1,1,1,1,1,1,1,1,1,1,1,1,1,1,1,1,1,1,
1,1,1,1,1,1,1,6),(0.,0.0153846153846154,0.0307692307692308,0.0461538461538462,
0.0615384615384615,0.0769230769230769,0.0923076923076923,0.107692307692308,
0.123076923076923,0.138461538461538,0.153846153846154,0.169230769230769,
0.184615384615385,0.2,0.215384615384615,0.230769230769231,0.246153846153846,
0.261538461538462,0.276923076923077,0.292307692307692,0.307692307692308,
0.323076923076923,0.338461538461538,0.353846153846154,0.369230769230769,
0.384615384615385,0.4,0.415384615384615,0.430769230769231,0.446153846153846,
0.461538461538462,0.476923076923077,0.492307692307692,0.507692307692308,
0.523076923076923,0.538461538461538,0.553846153846154,0.569230769230769,
0.584615384615384,0.6,0.615384615384615,0.63076923076923,0.646153846153846,
0.661538461538461,0.676923076923076,0.692307692307692,0.707692307692307,
0.723076923076922,0.738461538461538,0.753846153846153,0.769230769230768,
0.784615384615384,0.799999999999999,0.815384615384614,0.83076923076923,
0.846153846153845,0.86153846153846,0.876923076923076,0.892307692307691,
0.907692307692306,0.923076923076922,0.938461538461537,0.953846153846152,
0.969230769230768,0.984615384615383,0.994228156739699),.UNSPECIFIED.)
CURVE()
GEOMETRIC_REPRESENTATION_ITEM()
RATIONAL_B_SPLINE_CURVE((1.,1.,1.,1.,1.,1.,1.,1.,1.,1.,1.,1.,1.,1.,1.,1.,
1.,1.,1.,1.,1.,1.,1.,1.,1.,1.,1.,1.,1.,1.,1.,1.,1.,1.,1.,1.,1.,1.,1.,1.,
1.,1.,1.,1.,1.,1.,1.,1.,1.,1.,1.,1.,1.,1.,1.,1.,1.,1.,1.,1.,1.,1.,1.,1.,
1.,1.,1.,1.,1.,1.))
REPRESENTATION_ITEM('')
);
#279=(
BOUNDED_CURVE()
B_SPLINE_CURVE(5,(#35117,#35118,#35119,#35120,#35121,#35122,#35123,#35124,
#35125,#35126,#35127,#35128,#35129,#35130,#35131,#35132,#35133,#35134,#35135,
#35136,#35137,#35138,#35139,#35140,#35141,#35142,#35143,#35144,#35145,#35146,
#35147,#35148,#35149,#35150,#35151,#35152,#35153,#35154,#35155,#35156,#35157,
#35158,#35159,#35160,#35161,#35162,#35163,#35164,#35165,#35166,#35167,#35168,
#35169,#35170,#35171,#35172,#35173,#35174,#35175,#35176,#35177,#35178,#35179,
#35180,#35181,#35182,#35183,#35184,#35185,#35186),.UNSPECIFIED.,.F.,.F.)
B_SPLINE_CURVE_WITH_KNOTS((6,1,1,1,1,1,1,1,1,1,1,1,1,1,1,1,1,1,1,1,1,1,
1,1,1,1,1,1,1,1,1,1,1,1,1,1,1,1,1,1,1,1,1,1,1,1,1,1,1,1,1,1,1,1,1,1,1,1,
1,1,1,1,1,1,1,6),(0.00577184337450665,0.0153846153846154,0.0307692307692308,
0.0461538461538462,0.0615384615384615,0.0769230769230769,0.0923076923076923,
0.107692307692308,0.123076923076923,0.138461538461538,0.153846153846154,
0.169230769230769,0.184615384615385,0.2,0.215384615384615,0.230769230769231,
0.246153846153846,0.261538461538462,0.276923076923077,0.292307692307692,
0.307692307692308,0.323076923076923,0.338461538461538,0.353846153846154,
0.369230769230769,0.384615384615385,0.4,0.415384615384615,0.430769230769231,
0.446153846153846,0.461538461538462,0.476923076923077,0.492307692307692,
0.507692307692308,0.523076923076923,0.538461538461538,0.553846153846154,
0.569230769230769,0.584615384615384,0.6,0.615384615384615,0.63076923076923,
0.646153846153846,0.661538461538461,0.676923076923076,0.692307692307692,
0.707692307692307,0.723076923076922,0.738461538461538,0.753846153846153,
0.769230769230768,0.784615384615384,0.799999999999999,0.815384615384614,
0.83076923076923,0.846153846153845,0.86153846153846,0.876923076923076,0.892307692307691,
0.907692307692306,0.923076923076922,0.938461538461537,0.953846153846152,
0.969230769230768,0.984615384615383,1.),.UNSPECIFIED.)
CURVE()
GEOMETRIC_REPRESENTATION_ITEM()
RATIONAL_B_SPLINE_CURVE((1.,1.,1.,1.,1.,1.,1.,1.,1.,1.,1.,1.,1.,1.,1.,1.,
1.,1.,1.,1.,1.,1.,1.,1.,1.,1.,1.,1.,1.,1.,1.,1.,1.,1.,1.,1.,1.,1.,1.,1.,
1.,1.,1.,1.,1.,1.,1.,1.,1.,1.,1.,1.,1.,1.,1.,1.,1.,1.,1.,1.,1.,1.,1.,1.,
1.,1.,1.,1.,1.,1.))
REPRESENTATION_ITEM('')
);
#280=(
BOUNDED_CURVE()
B_SPLINE_CURVE(5,(#35190,#35191,#35192,#35193,#35194,#35195,#35196,#35197,
#35198,#35199,#35200,#35201,#35202,#35203,#35204,#35205,#35206,#35207,#35208,
#35209,#35210,#35211,#35212,#35213,#35214,#35215,#35216,#35217,#35218,#35219,
#35220,#35221,#35222,#35223,#35224,#35225,#35226,#35227,#35228,#35229,#35230,
#35231,#35232,#35233,#35234,#35235,#35236,#35237,#35238,#35239,#35240,#35241,
#35242,#35243,#35244,#35245,#35246,#35247,#35248,#35249,#35250,#35251,#35252,
#35253,#35254,#35255,#35256,#35257,#35258,#35259),.UNSPECIFIED.,.F.,.F.)
B_SPLINE_CURVE_WITH_KNOTS((6,1,1,1,1,1,1,1,1,1,1,1,1,1,1,1,1,1,1,1,1,1,
1,1,1,1,1,1,1,1,1,1,1,1,1,1,1,1,1,1,1,1,1,1,1,1,1,1,1,1,1,1,1,1,1,1,1,1,
1,1,1,1,1,1,1,6),(0.,0.0153846153846154,0.0307692307692308,0.0461538461538462,
0.0615384615384615,0.0769230769230769,0.0923076923076923,0.107692307692308,
0.123076923076923,0.138461538461538,0.153846153846154,0.169230769230769,
0.184615384615385,0.2,0.215384615384615,0.230769230769231,0.246153846153846,
0.261538461538462,0.276923076923077,0.292307692307692,0.307692307692308,
0.323076923076923,0.338461538461538,0.353846153846154,0.369230769230769,
0.384615384615385,0.4,0.415384615384615,0.430769230769231,0.446153846153846,
0.461538461538462,0.476923076923077,0.492307692307692,0.507692307692308,
0.523076923076923,0.538461538461538,0.553846153846154,0.569230769230769,
0.584615384615384,0.6,0.615384615384615,0.63076923076923,0.646153846153846,
0.661538461538461,0.676923076923076,0.692307692307692,0.707692307692307,
0.723076923076922,0.738461538461538,0.753846153846153,0.769230769230768,
0.784615384615384,0.799999999999999,0.815384615384614,0.83076923076923,
0.846153846153845,0.86153846153846,0.876923076923076,0.892307692307691,
0.907692307692306,0.923076923076922,0.938461538461537,0.953846153846152,
0.969230769230768,0.984615384615383,0.994228156739691),.UNSPECIFIED.)
CURVE()
GEOMETRIC_REPRESENTATION_ITEM()
RATIONAL_B_SPLINE_CURVE((1.,1.,1.,1.,1.,1.,1.,1.,1.,1.,1.,1.,1.,1.,1.,1.,
1.,1.,1.,1.,1.,1.,1.,1.,1.,1.,1.,1.,1.,1.,1.,1.,1.,1.,1.,1.,1.,1.,1.,1.,
1.,1.,1.,1.,1.,1.,1.,1.,1.,1.,1.,1.,1.,1.,1.,1.,1.,1.,1.,1.,1.,1.,1.,1.,
1.,1.,1.,1.,1.,1.))
REPRESENTATION_ITEM('')
);
#281=(
BOUNDED_CURVE()
B_SPLINE_CURVE(5,(#35263,#35264,#35265,#35266,#35267,#35268,#35269,#35270,
#35271,#35272,#35273,#35274,#35275,#35276,#35277,#35278,#35279,#35280,#35281,
#35282,#35283,#35284,#35285,#35286,#35287,#35288,#35289,#35290,#35291,#35292,
#35293,#35294,#35295,#35296,#35297,#35298,#35299,#35300,#35301,#35302,#35303,
#35304,#35305,#35306,#35307,#35308,#35309,#35310,#35311,#35312,#35313,#35314,
#35315,#35316,#35317,#35318,#35319,#35320,#35321,#35322,#35323,#35324,#35325,
#35326,#35327,#35328,#35329,#35330,#35331,#35332),.UNSPECIFIED.,.F.,.F.)
B_SPLINE_CURVE_WITH_KNOTS((6,1,1,1,1,1,1,1,1,1,1,1,1,1,1,1,1,1,1,1,1,1,
1,1,1,1,1,1,1,1,1,1,1,1,1,1,1,1,1,1,1,1,1,1,1,1,1,1,1,1,1,1,1,1,1,1,1,1,
1,1,1,1,1,1,1,6),(0.00577184337450785,0.0153846153846154,0.0307692307692308,
0.0461538461538462,0.0615384615384615,0.0769230769230769,0.0923076923076923,
0.107692307692308,0.123076923076923,0.138461538461538,0.153846153846154,
0.169230769230769,0.184615384615385,0.2,0.215384615384615,0.230769230769231,
0.246153846153846,0.261538461538462,0.276923076923077,0.292307692307692,
0.307692307692308,0.323076923076923,0.338461538461538,0.353846153846154,
0.369230769230769,0.384615384615385,0.4,0.415384615384615,0.430769230769231,
0.446153846153846,0.461538461538462,0.476923076923077,0.492307692307692,
0.507692307692308,0.523076923076923,0.538461538461538,0.553846153846154,
0.569230769230769,0.584615384615384,0.6,0.615384615384615,0.63076923076923,
0.646153846153846,0.661538461538461,0.676923076923076,0.692307692307692,
0.707692307692307,0.723076923076922,0.738461538461538,0.753846153846153,
0.769230769230768,0.784615384615384,0.799999999999999,0.815384615384614,
0.83076923076923,0.846153846153845,0.86153846153846,0.876923076923076,0.892307692307691,
0.907692307692306,0.923076923076922,0.938461538461537,0.953846153846152,
0.969230769230768,0.984615384615383,1.),.UNSPECIFIED.)
CURVE()
GEOMETRIC_REPRESENTATION_ITEM()
RATIONAL_B_SPLINE_CURVE((1.,1.,1.,1.,1.,1.,1.,1.,1.,1.,1.,1.,1.,1.,1.,1.,
1.,1.,1.,1.,1.,1.,1.,1.,1.,1.,1.,1.,1.,1.,1.,1.,1.,1.,1.,1.,1.,1.,1.,1.,
1.,1.,1.,1.,1.,1.,1.,1.,1.,1.,1.,1.,1.,1.,1.,1.,1.,1.,1.,1.,1.,1.,1.,1.,
1.,1.,1.,1.,1.,1.))
REPRESENTATION_ITEM('')
);
#282=(
BOUNDED_CURVE()
B_SPLINE_CURVE(5,(#35336,#35337,#35338,#35339,#35340,#35341,#35342,#35343,
#35344,#35345,#35346,#35347,#35348,#35349,#35350,#35351,#35352,#35353,#35354,
#35355,#35356,#35357,#35358,#35359,#35360,#35361,#35362,#35363,#35364,#35365,
#35366,#35367,#35368,#35369,#35370,#35371,#35372,#35373,#35374,#35375,#35376,
#35377,#35378,#35379,#35380,#35381,#35382,#35383,#35384,#35385,#35386,#35387,
#35388,#35389,#35390,#35391,#35392,#35393,#35394,#35395,#35396,#35397,#35398,
#35399,#35400,#35401,#35402,#35403,#35404,#35405),.UNSPECIFIED.,.F.,.F.)
B_SPLINE_CURVE_WITH_KNOTS((6,1,1,1,1,1,1,1,1,1,1,1,1,1,1,1,1,1,1,1,1,1,
1,1,1,1,1,1,1,1,1,1,1,1,1,1,1,1,1,1,1,1,1,1,1,1,1,1,1,1,1,1,1,1,1,1,1,1,
1,1,1,1,1,1,1,6),(0.,0.0153846153846154,0.0307692307692308,0.0461538461538462,
0.0615384615384615,0.0769230769230769,0.0923076923076923,0.107692307692308,
0.123076923076923,0.138461538461538,0.153846153846154,0.169230769230769,
0.184615384615385,0.2,0.215384615384615,0.230769230769231,0.246153846153846,
0.261538461538462,0.276923076923077,0.292307692307692,0.307692307692308,
0.323076923076923,0.338461538461538,0.353846153846154,0.369230769230769,
0.384615384615385,0.4,0.415384615384615,0.430769230769231,0.446153846153846,
0.461538461538462,0.476923076923077,0.492307692307692,0.507692307692308,
0.523076923076923,0.538461538461538,0.553846153846154,0.569230769230769,
0.584615384615384,0.6,0.615384615384615,0.63076923076923,0.646153846153846,
0.661538461538461,0.676923076923076,0.692307692307692,0.707692307692307,
0.723076923076922,0.738461538461538,0.753846153846153,0.769230769230768,
0.784615384615384,0.799999999999999,0.815384615384614,0.83076923076923,
0.846153846153845,0.86153846153846,0.876923076923076,0.892307692307691,
0.907692307692306,0.923076923076922,0.938461538461537,0.953846153846152,
0.969230769230768,0.984615384615383,0.994228156739708),.UNSPECIFIED.)
CURVE()
GEOMETRIC_REPRESENTATION_ITEM()
RATIONAL_B_SPLINE_CURVE((1.,1.,1.,1.,1.,1.,1.,1.,1.,1.,1.,1.,1.,1.,1.,1.,
1.,1.,1.,1.,1.,1.,1.,1.,1.,1.,1.,1.,1.,1.,1.,1.,1.,1.,1.,1.,1.,1.,1.,1.,
1.,1.,1.,1.,1.,1.,1.,1.,1.,1.,1.,1.,1.,1.,1.,1.,1.,1.,1.,1.,1.,1.,1.,1.,
1.,1.,1.,1.,1.,1.))
REPRESENTATION_ITEM('')
);
#283=(
BOUNDED_CURVE()
B_SPLINE_CURVE(5,(#35409,#35410,#35411,#35412,#35413,#35414,#35415,#35416,
#35417,#35418,#35419,#35420,#35421,#35422,#35423,#35424,#35425,#35426,#35427,
#35428,#35429,#35430,#35431,#35432,#35433,#35434,#35435,#35436,#35437,#35438,
#35439,#35440,#35441,#35442,#35443,#35444,#35445,#35446,#35447,#35448,#35449,
#35450,#35451,#35452,#35453,#35454,#35455,#35456,#35457,#35458,#35459,#35460,
#35461,#35462,#35463,#35464,#35465,#35466,#35467,#35468,#35469,#35470,#35471,
#35472,#35473,#35474,#35475,#35476,#35477,#35478),.UNSPECIFIED.,.F.,.F.)
B_SPLINE_CURVE_WITH_KNOTS((6,1,1,1,1,1,1,1,1,1,1,1,1,1,1,1,1,1,1,1,1,1,
1,1,1,1,1,1,1,1,1,1,1,1,1,1,1,1,1,1,1,1,1,1,1,1,1,1,1,1,1,1,1,1,1,1,1,1,
1,1,1,1,1,1,1,6),(0.00577184337450072,0.0153846153846154,0.0307692307692308,
0.0461538461538462,0.0615384615384615,0.0769230769230769,0.0923076923076923,
0.107692307692308,0.123076923076923,0.138461538461538,0.153846153846154,
0.169230769230769,0.184615384615385,0.2,0.215384615384615,0.230769230769231,
0.246153846153846,0.261538461538462,0.276923076923077,0.292307692307692,
0.307692307692308,0.323076923076923,0.338461538461538,0.353846153846154,
0.369230769230769,0.384615384615385,0.4,0.415384615384615,0.430769230769231,
0.446153846153846,0.461538461538462,0.476923076923077,0.492307692307692,
0.507692307692308,0.523076923076923,0.538461538461538,0.553846153846154,
0.569230769230769,0.584615384615384,0.6,0.615384615384615,0.63076923076923,
0.646153846153846,0.661538461538461,0.676923076923076,0.692307692307692,
0.707692307692307,0.723076923076922,0.738461538461538,0.753846153846153,
0.769230769230768,0.784615384615384,0.799999999999999,0.815384615384614,
0.83076923076923,0.846153846153845,0.86153846153846,0.876923076923076,0.892307692307691,
0.907692307692306,0.923076923076922,0.938461538461537,0.953846153846152,
0.969230769230768,0.984615384615383,1.),.UNSPECIFIED.)
CURVE()
GEOMETRIC_REPRESENTATION_ITEM()
RATIONAL_B_SPLINE_CURVE((1.,1.,1.,1.,1.,1.,1.,1.,1.,1.,1.,1.,1.,1.,1.,1.,
1.,1.,1.,1.,1.,1.,1.,1.,1.,1.,1.,1.,1.,1.,1.,1.,1.,1.,1.,1.,1.,1.,1.,1.,
1.,1.,1.,1.,1.,1.,1.,1.,1.,1.,1.,1.,1.,1.,1.,1.,1.,1.,1.,1.,1.,1.,1.,1.,
1.,1.,1.,1.,1.,1.))
REPRESENTATION_ITEM('')
);
#284=(
BOUNDED_CURVE()
B_SPLINE_CURVE(5,(#35482,#35483,#35484,#35485,#35486,#35487,#35488,#35489,
#35490,#35491,#35492,#35493,#35494,#35495,#35496,#35497,#35498,#35499,#35500,
#35501,#35502,#35503,#35504,#35505,#35506,#35507,#35508,#35509,#35510,#35511,
#35512,#35513,#35514,#35515,#35516,#35517,#35518,#35519,#35520,#35521,#35522,
#35523,#35524,#35525,#35526,#35527,#35528,#35529,#35530,#35531,#35532,#35533,
#35534,#35535,#35536,#35537,#35538,#35539,#35540,#35541,#35542,#35543,#35544,
#35545,#35546,#35547,#35548,#35549,#35550,#35551),.UNSPECIFIED.,.F.,.F.)
B_SPLINE_CURVE_WITH_KNOTS((6,1,1,1,1,1,1,1,1,1,1,1,1,1,1,1,1,1,1,1,1,1,
1,1,1,1,1,1,1,1,1,1,1,1,1,1,1,1,1,1,1,1,1,1,1,1,1,1,1,1,1,1,1,1,1,1,1,1,
1,1,1,1,1,1,1,6),(0.,0.0153846153846154,0.0307692307692308,0.0461538461538462,
0.0615384615384615,0.0769230769230769,0.0923076923076923,0.107692307692308,
0.123076923076923,0.138461538461538,0.153846153846154,0.169230769230769,
0.184615384615385,0.2,0.215384615384615,0.230769230769231,0.246153846153846,
0.261538461538462,0.276923076923077,0.292307692307692,0.307692307692308,
0.323076923076923,0.338461538461538,0.353846153846154,0.369230769230769,
0.384615384615385,0.4,0.415384615384615,0.430769230769231,0.446153846153846,
0.461538461538462,0.476923076923077,0.492307692307692,0.507692307692308,
0.523076923076923,0.538461538461538,0.553846153846154,0.569230769230769,
0.584615384615384,0.6,0.615384615384615,0.63076923076923,0.646153846153846,
0.661538461538461,0.676923076923076,0.692307692307692,0.707692307692307,
0.723076923076922,0.738461538461538,0.753846153846153,0.769230769230768,
0.784615384615384,0.799999999999999,0.815384615384614,0.83076923076923,
0.846153846153845,0.86153846153846,0.876923076923076,0.892307692307691,
0.907692307692306,0.923076923076922,0.938461538461537,0.953846153846152,
0.969230769230768,0.984615384615383,0.994228156739706),.UNSPECIFIED.)
CURVE()
GEOMETRIC_REPRESENTATION_ITEM()
RATIONAL_B_SPLINE_CURVE((1.,1.,1.,1.,1.,1.,1.,1.,1.,1.,1.,1.,1.,1.,1.,1.,
1.,1.,1.,1.,1.,1.,1.,1.,1.,1.,1.,1.,1.,1.,1.,1.,1.,1.,1.,1.,1.,1.,1.,1.,
1.,1.,1.,1.,1.,1.,1.,1.,1.,1.,1.,1.,1.,1.,1.,1.,1.,1.,1.,1.,1.,1.,1.,1.,
1.,1.,1.,1.,1.,1.))
REPRESENTATION_ITEM('')
);
#285=(
BOUNDED_CURVE()
B_SPLINE_CURVE(5,(#35555,#35556,#35557,#35558,#35559,#35560,#35561,#35562,
#35563,#35564,#35565,#35566,#35567,#35568,#35569,#35570,#35571,#35572,#35573,
#35574,#35575,#35576,#35577,#35578,#35579,#35580,#35581,#35582,#35583,#35584,
#35585,#35586,#35587,#35588,#35589,#35590,#35591,#35592,#35593,#35594,#35595,
#35596,#35597,#35598,#35599,#35600,#35601,#35602,#35603,#35604,#35605,#35606,
#35607,#35608,#35609,#35610,#35611,#35612,#35613,#35614,#35615,#35616,#35617,
#35618,#35619,#35620,#35621,#35622,#35623,#35624),.UNSPECIFIED.,.F.,.F.)
B_SPLINE_CURVE_WITH_KNOTS((6,1,1,1,1,1,1,1,1,1,1,1,1,1,1,1,1,1,1,1,1,1,
1,1,1,1,1,1,1,1,1,1,1,1,1,1,1,1,1,1,1,1,1,1,1,1,1,1,1,1,1,1,1,1,1,1,1,1,
1,1,1,1,1,1,1,6),(0.00577184337450902,0.0153846153846154,0.0307692307692308,
0.0461538461538462,0.0615384615384615,0.0769230769230769,0.0923076923076923,
0.107692307692308,0.123076923076923,0.138461538461538,0.153846153846154,
0.169230769230769,0.184615384615385,0.2,0.215384615384615,0.230769230769231,
0.246153846153846,0.261538461538462,0.276923076923077,0.292307692307692,
0.307692307692308,0.323076923076923,0.338461538461538,0.353846153846154,
0.369230769230769,0.384615384615385,0.4,0.415384615384615,0.430769230769231,
0.446153846153846,0.461538461538462,0.476923076923077,0.492307692307692,
0.507692307692308,0.523076923076923,0.538461538461538,0.553846153846154,
0.569230769230769,0.584615384615384,0.6,0.615384615384615,0.63076923076923,
0.646153846153846,0.661538461538461,0.676923076923076,0.692307692307692,
0.707692307692307,0.723076923076922,0.738461538461538,0.753846153846153,
0.769230769230768,0.784615384615384,0.799999999999999,0.815384615384614,
0.83076923076923,0.846153846153845,0.86153846153846,0.876923076923076,0.892307692307691,
0.907692307692306,0.923076923076922,0.938461538461537,0.953846153846152,
0.969230769230768,0.984615384615383,1.),.UNSPECIFIED.)
CURVE()
GEOMETRIC_REPRESENTATION_ITEM()
RATIONAL_B_SPLINE_CURVE((1.,1.,1.,1.,1.,1.,1.,1.,1.,1.,1.,1.,1.,1.,1.,1.,
1.,1.,1.,1.,1.,1.,1.,1.,1.,1.,1.,1.,1.,1.,1.,1.,1.,1.,1.,1.,1.,1.,1.,1.,
1.,1.,1.,1.,1.,1.,1.,1.,1.,1.,1.,1.,1.,1.,1.,1.,1.,1.,1.,1.,1.,1.,1.,1.,
1.,1.,1.,1.,1.,1.))
REPRESENTATION_ITEM('')
);
#286=(
BOUNDED_CURVE()
B_SPLINE_CURVE(5,(#35628,#35629,#35630,#35631,#35632,#35633,#35634,#35635,
#35636,#35637,#35638,#35639,#35640,#35641,#35642,#35643,#35644,#35645,#35646,
#35647,#35648,#35649,#35650,#35651,#35652,#35653,#35654,#35655,#35656,#35657,
#35658,#35659,#35660,#35661,#35662,#35663,#35664,#35665,#35666,#35667,#35668,
#35669,#35670,#35671,#35672,#35673,#35674,#35675,#35676,#35677,#35678,#35679,
#35680,#35681,#35682,#35683,#35684,#35685,#35686,#35687,#35688,#35689,#35690,
#35691,#35692,#35693,#35694,#35695,#35696,#35697),.UNSPECIFIED.,.F.,.F.)
B_SPLINE_CURVE_WITH_KNOTS((6,1,1,1,1,1,1,1,1,1,1,1,1,1,1,1,1,1,1,1,1,1,
1,1,1,1,1,1,1,1,1,1,1,1,1,1,1,1,1,1,1,1,1,1,1,1,1,1,1,1,1,1,1,1,1,1,1,1,
1,1,1,1,1,1,1,6),(0.,0.0153846153846154,0.0307692307692308,0.0461538461538462,
0.0615384615384615,0.0769230769230769,0.0923076923076923,0.107692307692308,
0.123076923076923,0.138461538461538,0.153846153846154,0.169230769230769,
0.184615384615385,0.2,0.215384615384615,0.230769230769231,0.246153846153846,
0.261538461538462,0.276923076923077,0.292307692307692,0.307692307692308,
0.323076923076923,0.338461538461538,0.353846153846154,0.369230769230769,
0.384615384615385,0.4,0.415384615384615,0.430769230769231,0.446153846153846,
0.461538461538462,0.476923076923077,0.492307692307692,0.507692307692308,
0.523076923076923,0.538461538461538,0.553846153846154,0.569230769230769,
0.584615384615384,0.6,0.615384615384615,0.63076923076923,0.646153846153846,
0.661538461538461,0.676923076923076,0.692307692307692,0.707692307692307,
0.723076923076922,0.738461538461538,0.753846153846153,0.769230769230768,
0.784615384615384,0.799999999999999,0.815384615384614,0.83076923076923,
0.846153846153845,0.86153846153846,0.876923076923076,0.892307692307691,
0.907692307692306,0.923076923076922,0.938461538461537,0.953846153846152,
0.969230769230768,0.984615384615383,0.994228156739698),.UNSPECIFIED.)
CURVE()
GEOMETRIC_REPRESENTATION_ITEM()
RATIONAL_B_SPLINE_CURVE((1.,1.,1.,1.,1.,1.,1.,1.,1.,1.,1.,1.,1.,1.,1.,1.,
1.,1.,1.,1.,1.,1.,1.,1.,1.,1.,1.,1.,1.,1.,1.,1.,1.,1.,1.,1.,1.,1.,1.,1.,
1.,1.,1.,1.,1.,1.,1.,1.,1.,1.,1.,1.,1.,1.,1.,1.,1.,1.,1.,1.,1.,1.,1.,1.,
1.,1.,1.,1.,1.,1.))
REPRESENTATION_ITEM('')
);
#287=(
BOUNDED_CURVE()
B_SPLINE_CURVE(5,(#35701,#35702,#35703,#35704,#35705,#35706,#35707,#35708,
#35709,#35710,#35711,#35712,#35713,#35714,#35715,#35716,#35717,#35718,#35719,
#35720,#35721,#35722,#35723,#35724,#35725,#35726,#35727,#35728,#35729,#35730,
#35731,#35732,#35733,#35734,#35735,#35736,#35737,#35738,#35739,#35740,#35741,
#35742,#35743,#35744,#35745,#35746,#35747,#35748,#35749,#35750,#35751,#35752,
#35753,#35754,#35755,#35756,#35757,#35758,#35759,#35760,#35761,#35762,#35763,
#35764,#35765,#35766,#35767,#35768,#35769,#35770),.UNSPECIFIED.,.F.,.F.)
B_SPLINE_CURVE_WITH_KNOTS((6,1,1,1,1,1,1,1,1,1,1,1,1,1,1,1,1,1,1,1,1,1,
1,1,1,1,1,1,1,1,1,1,1,1,1,1,1,1,1,1,1,1,1,1,1,1,1,1,1,1,1,1,1,1,1,1,1,1,
1,1,1,1,1,1,1,6),(0.00577184337451611,0.0153846153846154,0.0307692307692308,
0.0461538461538462,0.0615384615384615,0.0769230769230769,0.0923076923076923,
0.107692307692308,0.123076923076923,0.138461538461538,0.153846153846154,
0.169230769230769,0.184615384615385,0.2,0.215384615384615,0.230769230769231,
0.246153846153846,0.261538461538462,0.276923076923077,0.292307692307692,
0.307692307692308,0.323076923076923,0.338461538461538,0.353846153846154,
0.369230769230769,0.384615384615385,0.4,0.415384615384615,0.430769230769231,
0.446153846153846,0.461538461538462,0.476923076923077,0.492307692307692,
0.507692307692308,0.523076923076923,0.538461538461538,0.553846153846154,
0.569230769230769,0.584615384615384,0.6,0.615384615384615,0.63076923076923,
0.646153846153846,0.661538461538461,0.676923076923076,0.692307692307692,
0.707692307692307,0.723076923076922,0.738461538461538,0.753846153846153,
0.769230769230768,0.784615384615384,0.799999999999999,0.815384615384614,
0.83076923076923,0.846153846153845,0.86153846153846,0.876923076923076,0.892307692307691,
0.907692307692306,0.923076923076922,0.938461538461537,0.953846153846152,
0.969230769230768,0.984615384615383,1.),.UNSPECIFIED.)
CURVE()
GEOMETRIC_REPRESENTATION_ITEM()
RATIONAL_B_SPLINE_CURVE((1.,1.,1.,1.,1.,1.,1.,1.,1.,1.,1.,1.,1.,1.,1.,1.,
1.,1.,1.,1.,1.,1.,1.,1.,1.,1.,1.,1.,1.,1.,1.,1.,1.,1.,1.,1.,1.,1.,1.,1.,
1.,1.,1.,1.,1.,1.,1.,1.,1.,1.,1.,1.,1.,1.,1.,1.,1.,1.,1.,1.,1.,1.,1.,1.,
1.,1.,1.,1.,1.,1.))
REPRESENTATION_ITEM('')
);
#288=(
BOUNDED_CURVE()
B_SPLINE_CURVE(5,(#35774,#35775,#35776,#35777,#35778,#35779,#35780,#35781,
#35782,#35783,#35784,#35785,#35786,#35787,#35788,#35789,#35790,#35791,#35792,
#35793,#35794,#35795,#35796,#35797,#35798,#35799,#35800,#35801,#35802,#35803,
#35804,#35805,#35806,#35807,#35808,#35809,#35810,#35811,#35812,#35813,#35814,
#35815,#35816,#35817,#35818,#35819,#35820,#35821,#35822,#35823,#35824,#35825,
#35826,#35827,#35828,#35829,#35830,#35831,#35832,#35833,#35834,#35835,#35836,
#35837,#35838,#35839,#35840,#35841,#35842,#35843),.UNSPECIFIED.,.F.,.F.)
B_SPLINE_CURVE_WITH_KNOTS((6,1,1,1,1,1,1,1,1,1,1,1,1,1,1,1,1,1,1,1,1,1,
1,1,1,1,1,1,1,1,1,1,1,1,1,1,1,1,1,1,1,1,1,1,1,1,1,1,1,1,1,1,1,1,1,1,1,1,
1,1,1,1,1,1,1,6),(0.,0.0153846153846154,0.0307692307692308,0.0461538461538462,
0.0615384615384615,0.0769230769230769,0.0923076923076923,0.107692307692308,
0.123076923076923,0.138461538461538,0.153846153846154,0.169230769230769,
0.184615384615385,0.2,0.215384615384615,0.230769230769231,0.246153846153846,
0.261538461538462,0.276923076923077,0.292307692307692,0.307692307692308,
0.323076923076923,0.338461538461538,0.353846153846154,0.369230769230769,
0.384615384615385,0.4,0.415384615384615,0.430769230769231,0.446153846153846,
0.461538461538462,0.476923076923077,0.492307692307692,0.507692307692308,
0.523076923076923,0.538461538461538,0.553846153846154,0.569230769230769,
0.584615384615384,0.6,0.615384615384615,0.63076923076923,0.646153846153846,
0.661538461538461,0.676923076923076,0.692307692307692,0.707692307692307,
0.723076923076922,0.738461538461538,0.753846153846153,0.769230769230768,
0.784615384615384,0.799999999999999,0.815384615384614,0.83076923076923,
0.846153846153845,0.86153846153846,0.876923076923076,0.892307692307691,
0.907692307692306,0.923076923076922,0.938461538461537,0.953846153846152,
0.969230769230768,0.984615384615383,0.994228156739704),.UNSPECIFIED.)
CURVE()
GEOMETRIC_REPRESENTATION_ITEM()
RATIONAL_B_SPLINE_CURVE((1.,1.,1.,1.,1.,1.,1.,1.,1.,1.,1.,1.,1.,1.,1.,1.,
1.,1.,1.,1.,1.,1.,1.,1.,1.,1.,1.,1.,1.,1.,1.,1.,1.,1.,1.,1.,1.,1.,1.,1.,
1.,1.,1.,1.,1.,1.,1.,1.,1.,1.,1.,1.,1.,1.,1.,1.,1.,1.,1.,1.,1.,1.,1.,1.,
1.,1.,1.,1.,1.,1.))
REPRESENTATION_ITEM('')
);
#289=(
BOUNDED_CURVE()
B_SPLINE_CURVE(5,(#35847,#35848,#35849,#35850,#35851,#35852,#35853,#35854,
#35855,#35856,#35857,#35858,#35859,#35860,#35861,#35862,#35863,#35864,#35865,
#35866,#35867,#35868,#35869,#35870,#35871,#35872,#35873,#35874,#35875,#35876,
#35877,#35878,#35879,#35880,#35881,#35882,#35883,#35884,#35885,#35886,#35887,
#35888,#35889,#35890,#35891,#35892,#35893,#35894,#35895,#35896,#35897,#35898,
#35899,#35900,#35901,#35902,#35903,#35904,#35905,#35906,#35907,#35908,#35909,
#35910,#35911,#35912,#35913,#35914,#35915,#35916),.UNSPECIFIED.,.F.,.F.)
B_SPLINE_CURVE_WITH_KNOTS((6,1,1,1,1,1,1,1,1,1,1,1,1,1,1,1,1,1,1,1,1,1,
1,1,1,1,1,1,1,1,1,1,1,1,1,1,1,1,1,1,1,1,1,1,1,1,1,1,1,1,1,1,1,1,1,1,1,1,
1,1,1,1,1,1,1,6),(0.00577184337449692,0.0153846153846154,0.0307692307692308,
0.0461538461538462,0.0615384615384615,0.0769230769230769,0.0923076923076923,
0.107692307692308,0.123076923076923,0.138461538461538,0.153846153846154,
0.169230769230769,0.184615384615385,0.2,0.215384615384615,0.230769230769231,
0.246153846153846,0.261538461538462,0.276923076923077,0.292307692307692,
0.307692307692308,0.323076923076923,0.338461538461538,0.353846153846154,
0.369230769230769,0.384615384615385,0.4,0.415384615384615,0.430769230769231,
0.446153846153846,0.461538461538462,0.476923076923077,0.492307692307692,
0.507692307692308,0.523076923076923,0.538461538461538,0.553846153846154,
0.569230769230769,0.584615384615384,0.6,0.615384615384615,0.63076923076923,
0.646153846153846,0.661538461538461,0.676923076923076,0.692307692307692,
0.707692307692307,0.723076923076922,0.738461538461538,0.753846153846153,
0.769230769230768,0.784615384615384,0.799999999999999,0.815384615384614,
0.83076923076923,0.846153846153845,0.86153846153846,0.876923076923076,0.892307692307691,
0.907692307692306,0.923076923076922,0.938461538461537,0.953846153846152,
0.969230769230768,0.984615384615383,1.),.UNSPECIFIED.)
CURVE()
GEOMETRIC_REPRESENTATION_ITEM()
RATIONAL_B_SPLINE_CURVE((1.,1.,1.,1.,1.,1.,1.,1.,1.,1.,1.,1.,1.,1.,1.,1.,
1.,1.,1.,1.,1.,1.,1.,1.,1.,1.,1.,1.,1.,1.,1.,1.,1.,1.,1.,1.,1.,1.,1.,1.,
1.,1.,1.,1.,1.,1.,1.,1.,1.,1.,1.,1.,1.,1.,1.,1.,1.,1.,1.,1.,1.,1.,1.,1.,
1.,1.,1.,1.,1.,1.))
REPRESENTATION_ITEM('')
);
#290=(
BOUNDED_CURVE()
B_SPLINE_CURVE(5,(#35919,#35920,#35921,#35922,#35923,#35924,#35925,#35926,
#35927,#35928,#35929,#35930,#35931,#35932,#35933,#35934,#35935,#35936,#35937,
#35938,#35939,#35940,#35941,#35942,#35943,#35944,#35945,#35946,#35947,#35948,
#35949,#35950,#35951,#35952,#35953,#35954,#35955,#35956,#35957,#35958,#35959,
#35960,#35961,#35962,#35963,#35964,#35965,#35966,#35967,#35968,#35969,#35970,
#35971,#35972,#35973,#35974,#35975,#35976,#35977,#35978,#35979,#35980,#35981,
#35982,#35983,#35984,#35985,#35986,#35987,#35988),.UNSPECIFIED.,.F.,.F.)
B_SPLINE_CURVE_WITH_KNOTS((6,1,1,1,1,1,1,1,1,1,1,1,1,1,1,1,1,1,1,1,1,1,
1,1,1,1,1,1,1,1,1,1,1,1,1,1,1,1,1,1,1,1,1,1,1,1,1,1,1,1,1,1,1,1,1,1,1,1,
1,1,1,1,1,1,1,6),(0.,0.0153846153846154,0.0307692307692308,0.0461538461538462,
0.0615384615384615,0.0769230769230769,0.0923076923076923,0.107692307692308,
0.123076923076923,0.138461538461538,0.153846153846154,0.169230769230769,
0.184615384615385,0.2,0.215384615384615,0.230769230769231,0.246153846153846,
0.261538461538462,0.276923076923077,0.292307692307692,0.307692307692308,
0.323076923076923,0.338461538461538,0.353846153846154,0.369230769230769,
0.384615384615385,0.4,0.415384615384615,0.430769230769231,0.446153846153846,
0.461538461538462,0.476923076923077,0.492307692307692,0.507692307692308,
0.523076923076923,0.538461538461538,0.553846153846154,0.569230769230769,
0.584615384615384,0.6,0.615384615384615,0.63076923076923,0.646153846153846,
0.661538461538461,0.676923076923076,0.692307692307692,0.707692307692307,
0.723076923076922,0.738461538461538,0.753846153846153,0.769230769230768,
0.784615384615384,0.799999999999999,0.815384615384614,0.83076923076923,
0.846153846153845,0.86153846153846,0.876923076923076,0.892307692307691,
0.907692307692306,0.923076923076922,0.938461538461537,0.953846153846152,
0.969230769230768,0.984615384615383,0.994228156739723),.UNSPECIFIED.)
CURVE()
GEOMETRIC_REPRESENTATION_ITEM()
RATIONAL_B_SPLINE_CURVE((1.,1.,1.,1.,1.,1.,1.,1.,1.,1.,1.,1.,1.,1.,1.,1.,
1.,1.,1.,1.,1.,1.,1.,1.,1.,1.,1.,1.,1.,1.,1.,1.,1.,1.,1.,1.,1.,1.,1.,1.,
1.,1.,1.,1.,1.,1.,1.,1.,1.,1.,1.,1.,1.,1.,1.,1.,1.,1.,1.,1.,1.,1.,1.,1.,
1.,1.,1.,1.,1.,1.))
REPRESENTATION_ITEM('')
);
#291=(
BOUNDED_CURVE()
B_SPLINE_CURVE(5,(#36147,#36148,#36149,#36150,#36151,#36152,#36153,#36154,
#36155,#36156,#36157,#36158,#36159,#36160,#36161,#36162,#36163,#36164,#36165,
#36166,#36167,#36168,#36169,#36170,#36171,#36172,#36173,#36174,#36175,#36176,
#36177,#36178,#36179,#36180,#36181,#36182,#36183,#36184,#36185,#36186,#36187,
#36188,#36189,#36190,#36191,#36192,#36193,#36194,#36195,#36196,#36197,#36198,
#36199,#36200,#36201,#36202,#36203,#36204,#36205,#36206,#36207,#36208,#36209,
#36210,#36211,#36212,#36213,#36214,#36215,#36216),.UNSPECIFIED.,.F.,.F.)
B_SPLINE_CURVE_WITH_KNOTS((6,1,1,1,1,1,1,1,1,1,1,1,1,1,1,1,1,1,1,1,1,1,
1,1,1,1,1,1,1,1,1,1,1,1,1,1,1,1,1,1,1,1,1,1,1,1,1,1,1,1,1,1,1,1,1,1,1,1,
1,1,1,1,1,1,1,6),(-1.,-0.984615384615383,-0.969230769230768,-0.953846153846152,
-0.938461538461537,-0.923076923076922,-0.907692307692306,-0.892307692307691,
-0.876923076923076,-0.86153846153846,-0.846153846153845,-0.83076923076923,
-0.815384615384614,-0.799999999999999,-0.784615384615384,-0.769230769230768,
-0.753846153846153,-0.738461538461538,-0.723076923076922,-0.707692307692307,
-0.692307692307692,-0.676923076923076,-0.661538461538461,-0.646153846153846,
-0.63076923076923,-0.615384615384615,-0.6,-0.584615384615384,-0.569230769230769,
-0.553846153846154,-0.538461538461538,-0.523076923076923,-0.507692307692308,
-0.492307692307692,-0.476923076923077,-0.461538461538462,-0.446153846153846,
-0.430769230769231,-0.415384615384615,-0.4,-0.384615384615385,-0.369230769230769,
-0.353846153846154,-0.338461538461538,-0.323076923076923,-0.307692307692308,
-0.292307692307692,-0.276923076923077,-0.261538461538462,-0.246153846153846,
-0.230769230769231,-0.215384615384615,-0.2,-0.184615384615385,-0.169230769230769,
-0.153846153846154,-0.138461538461538,-0.123076923076923,-0.107692307692308,
-0.0923076923076923,-0.0769230769230769,-0.0615384615384615,-0.0461538461538462,
-0.0307692307692308,-0.0153846153846154,-0.00577184337448906),
 .UNSPECIFIED.)
CURVE()
GEOMETRIC_REPRESENTATION_ITEM()
RATIONAL_B_SPLINE_CURVE((1.,1.,1.,1.,1.,1.,1.,1.,1.,1.,1.,1.,1.,1.,1.,1.,
1.,1.,1.,1.,1.,1.,1.,1.,1.,1.,1.,1.,1.,1.,1.,1.,1.,1.,1.,1.,1.,1.,1.,1.,
1.,1.,1.,1.,1.,1.,1.,1.,1.,1.,1.,1.,1.,1.,1.,1.,1.,1.,1.,1.,1.,1.,1.,1.,
1.,1.,1.,1.,1.,1.))
REPRESENTATION_ITEM('')
);
#292=(
BOUNDED_CURVE()
B_SPLINE_CURVE(5,(#36367,#36368,#36369,#36370,#36371,#36372,#36373,#36374,
#36375,#36376,#36377,#36378,#36379,#36380,#36381,#36382,#36383,#36384,#36385,
#36386,#36387,#36388,#36389,#36390,#36391,#36392,#36393,#36394,#36395,#36396,
#36397,#36398,#36399,#36400,#36401,#36402,#36403,#36404,#36405,#36406,#36407,
#36408,#36409,#36410,#36411,#36412,#36413,#36414,#36415,#36416,#36417,#36418,
#36419,#36420,#36421,#36422,#36423,#36424,#36425,#36426,#36427,#36428,#36429,
#36430,#36431,#36432,#36433,#36434,#36435,#36436),.UNSPECIFIED.,.F.,.F.)
B_SPLINE_CURVE_WITH_KNOTS((6,1,1,1,1,1,1,1,1,1,1,1,1,1,1,1,1,1,1,1,1,1,
1,1,1,1,1,1,1,1,1,1,1,1,1,1,1,1,1,1,1,1,1,1,1,1,1,1,1,1,1,1,1,1,1,1,1,1,
1,1,1,1,1,1,1,6),(-0.994228156739728,-0.984615384615383,-0.969230769230768,
-0.953846153846152,-0.938461538461537,-0.923076923076922,-0.907692307692306,
-0.892307692307691,-0.876923076923076,-0.86153846153846,-0.846153846153845,
-0.83076923076923,-0.815384615384614,-0.799999999999999,-0.784615384615384,
-0.769230769230768,-0.753846153846153,-0.738461538461538,-0.723076923076922,
-0.707692307692307,-0.692307692307692,-0.676923076923076,-0.661538461538461,
-0.646153846153846,-0.63076923076923,-0.615384615384615,-0.6,-0.584615384615384,
-0.569230769230769,-0.553846153846154,-0.538461538461538,-0.523076923076923,
-0.507692307692308,-0.492307692307692,-0.476923076923077,-0.461538461538462,
-0.446153846153846,-0.430769230769231,-0.415384615384615,-0.4,-0.384615384615385,
-0.369230769230769,-0.353846153846154,-0.338461538461538,-0.323076923076923,
-0.307692307692308,-0.292307692307692,-0.276923076923077,-0.261538461538462,
-0.246153846153846,-0.230769230769231,-0.215384615384615,-0.2,-0.184615384615385,
-0.169230769230769,-0.153846153846154,-0.138461538461538,-0.123076923076923,
-0.107692307692308,-0.0923076923076923,-0.0769230769230769,-0.0615384615384615,
-0.0461538461538462,-0.0307692307692308,-0.0153846153846154,0.),
 .UNSPECIFIED.)
CURVE()
GEOMETRIC_REPRESENTATION_ITEM()
RATIONAL_B_SPLINE_CURVE((1.,1.,1.,1.,1.,1.,1.,1.,1.,1.,1.,1.,1.,1.,1.,1.,
1.,1.,1.,1.,1.,1.,1.,1.,1.,1.,1.,1.,1.,1.,1.,1.,1.,1.,1.,1.,1.,1.,1.,1.,
1.,1.,1.,1.,1.,1.,1.,1.,1.,1.,1.,1.,1.,1.,1.,1.,1.,1.,1.,1.,1.,1.,1.,1.,
1.,1.,1.,1.,1.,1.))
REPRESENTATION_ITEM('')
);
#293=(
BOUNDED_CURVE()
B_SPLINE_CURVE(5,(#36589,#36590,#36591,#36592,#36593,#36594,#36595,#36596,
#36597,#36598,#36599,#36600,#36601,#36602,#36603,#36604,#36605,#36606,#36607,
#36608,#36609,#36610,#36611,#36612,#36613,#36614,#36615,#36616,#36617,#36618,
#36619,#36620,#36621,#36622,#36623,#36624,#36625,#36626,#36627,#36628,#36629,
#36630,#36631,#36632,#36633,#36634,#36635,#36636,#36637,#36638,#36639,#36640,
#36641,#36642,#36643,#36644,#36645,#36646,#36647,#36648,#36649,#36650,#36651,
#36652,#36653,#36654,#36655,#36656,#36657,#36658),.UNSPECIFIED.,.F.,.F.)
B_SPLINE_CURVE_WITH_KNOTS((6,1,1,1,1,1,1,1,1,1,1,1,1,1,1,1,1,1,1,1,1,1,
1,1,1,1,1,1,1,1,1,1,1,1,1,1,1,1,1,1,1,1,1,1,1,1,1,1,1,1,1,1,1,1,1,1,1,1,
1,1,1,1,1,1,1,6),(-1.,-0.984615384615383,-0.969230769230768,-0.953846153846152,
-0.938461538461537,-0.923076923076922,-0.907692307692306,-0.892307692307691,
-0.876923076923076,-0.86153846153846,-0.846153846153845,-0.83076923076923,
-0.815384615384614,-0.799999999999999,-0.784615384615384,-0.769230769230768,
-0.753846153846153,-0.738461538461538,-0.723076923076922,-0.707692307692307,
-0.692307692307692,-0.676923076923076,-0.661538461538461,-0.646153846153846,
-0.63076923076923,-0.615384615384615,-0.6,-0.584615384615384,-0.569230769230769,
-0.553846153846154,-0.538461538461538,-0.523076923076923,-0.507692307692308,
-0.492307692307692,-0.476923076923077,-0.461538461538462,-0.446153846153846,
-0.430769230769231,-0.415384615384615,-0.4,-0.384615384615385,-0.369230769230769,
-0.353846153846154,-0.338461538461538,-0.323076923076923,-0.307692307692308,
-0.292307692307692,-0.276923076923077,-0.261538461538462,-0.246153846153846,
-0.230769230769231,-0.215384615384615,-0.2,-0.184615384615385,-0.169230769230769,
-0.153846153846154,-0.138461538461538,-0.123076923076923,-0.107692307692308,
-0.0923076923076923,-0.0769230769230769,-0.0615384615384615,-0.0461538461538462,
-0.0307692307692308,-0.0153846153846154,-0.0057718433744926),
 .UNSPECIFIED.)
CURVE()
GEOMETRIC_REPRESENTATION_ITEM()
RATIONAL_B_SPLINE_CURVE((1.,1.,1.,1.,1.,1.,1.,1.,1.,1.,1.,1.,1.,1.,1.,1.,
1.,1.,1.,1.,1.,1.,1.,1.,1.,1.,1.,1.,1.,1.,1.,1.,1.,1.,1.,1.,1.,1.,1.,1.,
1.,1.,1.,1.,1.,1.,1.,1.,1.,1.,1.,1.,1.,1.,1.,1.,1.,1.,1.,1.,1.,1.,1.,1.,
1.,1.,1.,1.,1.,1.))
REPRESENTATION_ITEM('')
);
#294=(
BOUNDED_CURVE()
B_SPLINE_CURVE(5,(#36809,#36810,#36811,#36812,#36813,#36814,#36815,#36816,
#36817,#36818,#36819,#36820,#36821,#36822,#36823,#36824,#36825,#36826,#36827,
#36828,#36829,#36830,#36831,#36832,#36833,#36834,#36835,#36836,#36837,#36838,
#36839,#36840,#36841,#36842,#36843,#36844,#36845,#36846,#36847,#36848,#36849,
#36850,#36851,#36852,#36853,#36854,#36855,#36856,#36857,#36858,#36859,#36860,
#36861,#36862,#36863,#36864,#36865,#36866,#36867,#36868,#36869,#36870,#36871,
#36872,#36873,#36874,#36875,#36876,#36877,#36878),.UNSPECIFIED.,.F.,.F.)
B_SPLINE_CURVE_WITH_KNOTS((6,1,1,1,1,1,1,1,1,1,1,1,1,1,1,1,1,1,1,1,1,1,
1,1,1,1,1,1,1,1,1,1,1,1,1,1,1,1,1,1,1,1,1,1,1,1,1,1,1,1,1,1,1,1,1,1,1,1,
1,1,1,1,1,1,1,6),(-0.994228156739718,-0.984615384615383,-0.969230769230768,
-0.953846153846152,-0.938461538461537,-0.923076923076922,-0.907692307692306,
-0.892307692307691,-0.876923076923076,-0.86153846153846,-0.846153846153845,
-0.83076923076923,-0.815384615384614,-0.799999999999999,-0.784615384615384,
-0.769230769230768,-0.753846153846153,-0.738461538461538,-0.723076923076922,
-0.707692307692307,-0.692307692307692,-0.676923076923076,-0.661538461538461,
-0.646153846153846,-0.63076923076923,-0.615384615384615,-0.6,-0.584615384615384,
-0.569230769230769,-0.553846153846154,-0.538461538461538,-0.523076923076923,
-0.507692307692308,-0.492307692307692,-0.476923076923077,-0.461538461538462,
-0.446153846153846,-0.430769230769231,-0.415384615384615,-0.4,-0.384615384615385,
-0.369230769230769,-0.353846153846154,-0.338461538461538,-0.323076923076923,
-0.307692307692308,-0.292307692307692,-0.276923076923077,-0.261538461538462,
-0.246153846153846,-0.230769230769231,-0.215384615384615,-0.2,-0.184615384615385,
-0.169230769230769,-0.153846153846154,-0.138461538461538,-0.123076923076923,
-0.107692307692308,-0.0923076923076923,-0.0769230769230769,-0.0615384615384615,
-0.0461538461538462,-0.0307692307692308,-0.0153846153846154,0.),
 .UNSPECIFIED.)
CURVE()
GEOMETRIC_REPRESENTATION_ITEM()
RATIONAL_B_SPLINE_CURVE((1.,1.,1.,1.,1.,1.,1.,1.,1.,1.,1.,1.,1.,1.,1.,1.,
1.,1.,1.,1.,1.,1.,1.,1.,1.,1.,1.,1.,1.,1.,1.,1.,1.,1.,1.,1.,1.,1.,1.,1.,
1.,1.,1.,1.,1.,1.,1.,1.,1.,1.,1.,1.,1.,1.,1.,1.,1.,1.,1.,1.,1.,1.,1.,1.,
1.,1.,1.,1.,1.,1.))
REPRESENTATION_ITEM('')
);
#295=(
BOUNDED_CURVE()
B_SPLINE_CURVE(5,(#37031,#37032,#37033,#37034,#37035,#37036,#37037,#37038,
#37039,#37040,#37041,#37042,#37043,#37044,#37045,#37046,#37047,#37048,#37049,
#37050,#37051,#37052,#37053,#37054,#37055,#37056,#37057,#37058,#37059,#37060,
#37061,#37062,#37063,#37064,#37065,#37066,#37067,#37068,#37069,#37070,#37071,
#37072,#37073,#37074,#37075,#37076,#37077,#37078,#37079,#37080,#37081,#37082,
#37083,#37084,#37085,#37086,#37087,#37088,#37089,#37090,#37091,#37092,#37093,
#37094,#37095,#37096,#37097,#37098,#37099,#37100),.UNSPECIFIED.,.F.,.F.)
B_SPLINE_CURVE_WITH_KNOTS((6,1,1,1,1,1,1,1,1,1,1,1,1,1,1,1,1,1,1,1,1,1,
1,1,1,1,1,1,1,1,1,1,1,1,1,1,1,1,1,1,1,1,1,1,1,1,1,1,1,1,1,1,1,1,1,1,1,1,
1,1,1,1,1,1,1,6),(-1.,-0.984615384615383,-0.969230769230768,-0.953846153846152,
-0.938461538461537,-0.923076923076922,-0.907692307692306,-0.892307692307691,
-0.876923076923076,-0.86153846153846,-0.846153846153845,-0.83076923076923,
-0.815384615384614,-0.799999999999999,-0.784615384615384,-0.769230769230768,
-0.753846153846153,-0.738461538461538,-0.723076923076922,-0.707692307692307,
-0.692307692307692,-0.676923076923076,-0.661538461538461,-0.646153846153846,
-0.63076923076923,-0.615384615384615,-0.6,-0.584615384615384,-0.569230769230769,
-0.553846153846154,-0.538461538461538,-0.523076923076923,-0.507692307692308,
-0.492307692307692,-0.476923076923077,-0.461538461538462,-0.446153846153846,
-0.430769230769231,-0.415384615384615,-0.4,-0.384615384615385,-0.369230769230769,
-0.353846153846154,-0.338461538461538,-0.323076923076923,-0.307692307692308,
-0.292307692307692,-0.276923076923077,-0.261538461538462,-0.246153846153846,
-0.230769230769231,-0.215384615384615,-0.2,-0.184615384615385,-0.169230769230769,
-0.153846153846154,-0.138461538461538,-0.123076923076923,-0.107692307692308,
-0.0923076923076923,-0.0769230769230769,-0.0615384615384615,-0.0461538461538462,
-0.0307692307692308,-0.0153846153846154,-0.00577184337449396),
 .UNSPECIFIED.)
CURVE()
GEOMETRIC_REPRESENTATION_ITEM()
RATIONAL_B_SPLINE_CURVE((1.,1.,1.,1.,1.,1.,1.,1.,1.,1.,1.,1.,1.,1.,1.,1.,
1.,1.,1.,1.,1.,1.,1.,1.,1.,1.,1.,1.,1.,1.,1.,1.,1.,1.,1.,1.,1.,1.,1.,1.,
1.,1.,1.,1.,1.,1.,1.,1.,1.,1.,1.,1.,1.,1.,1.,1.,1.,1.,1.,1.,1.,1.,1.,1.,
1.,1.,1.,1.,1.,1.))
REPRESENTATION_ITEM('')
);
#296=(
BOUNDED_CURVE()
B_SPLINE_CURVE(5,(#37251,#37252,#37253,#37254,#37255,#37256,#37257,#37258,
#37259,#37260,#37261,#37262,#37263,#37264,#37265,#37266,#37267,#37268,#37269,
#37270,#37271,#37272,#37273,#37274,#37275,#37276,#37277,#37278,#37279,#37280,
#37281,#37282,#37283,#37284,#37285,#37286,#37287,#37288,#37289,#37290,#37291,
#37292,#37293,#37294,#37295,#37296,#37297,#37298,#37299,#37300,#37301,#37302,
#37303,#37304,#37305,#37306,#37307,#37308,#37309,#37310,#37311,#37312,#37313,
#37314,#37315,#37316,#37317,#37318,#37319,#37320),.UNSPECIFIED.,.F.,.F.)
B_SPLINE_CURVE_WITH_KNOTS((6,1,1,1,1,1,1,1,1,1,1,1,1,1,1,1,1,1,1,1,1,1,
1,1,1,1,1,1,1,1,1,1,1,1,1,1,1,1,1,1,1,1,1,1,1,1,1,1,1,1,1,1,1,1,1,1,1,1,
1,1,1,1,1,1,1,6),(-0.994228156739702,-0.984615384615383,-0.969230769230768,
-0.953846153846152,-0.938461538461537,-0.923076923076922,-0.907692307692306,
-0.892307692307691,-0.876923076923076,-0.86153846153846,-0.846153846153845,
-0.83076923076923,-0.815384615384614,-0.799999999999999,-0.784615384615384,
-0.769230769230768,-0.753846153846153,-0.738461538461538,-0.723076923076922,
-0.707692307692307,-0.692307692307692,-0.676923076923076,-0.661538461538461,
-0.646153846153846,-0.63076923076923,-0.615384615384615,-0.6,-0.584615384615384,
-0.569230769230769,-0.553846153846154,-0.538461538461538,-0.523076923076923,
-0.507692307692308,-0.492307692307692,-0.476923076923077,-0.461538461538462,
-0.446153846153846,-0.430769230769231,-0.415384615384615,-0.4,-0.384615384615385,
-0.369230769230769,-0.353846153846154,-0.338461538461538,-0.323076923076923,
-0.307692307692308,-0.292307692307692,-0.276923076923077,-0.261538461538462,
-0.246153846153846,-0.230769230769231,-0.215384615384615,-0.2,-0.184615384615385,
-0.169230769230769,-0.153846153846154,-0.138461538461538,-0.123076923076923,
-0.107692307692308,-0.0923076923076923,-0.0769230769230769,-0.0615384615384615,
-0.0461538461538462,-0.0307692307692308,-0.0153846153846154,0.),
 .UNSPECIFIED.)
CURVE()
GEOMETRIC_REPRESENTATION_ITEM()
RATIONAL_B_SPLINE_CURVE((1.,1.,1.,1.,1.,1.,1.,1.,1.,1.,1.,1.,1.,1.,1.,1.,
1.,1.,1.,1.,1.,1.,1.,1.,1.,1.,1.,1.,1.,1.,1.,1.,1.,1.,1.,1.,1.,1.,1.,1.,
1.,1.,1.,1.,1.,1.,1.,1.,1.,1.,1.,1.,1.,1.,1.,1.,1.,1.,1.,1.,1.,1.,1.,1.,
1.,1.,1.,1.,1.,1.))
REPRESENTATION_ITEM('')
);
#297=(
BOUNDED_CURVE()
B_SPLINE_CURVE(5,(#37473,#37474,#37475,#37476,#37477,#37478,#37479,#37480,
#37481,#37482,#37483,#37484,#37485,#37486,#37487,#37488,#37489,#37490,#37491,
#37492,#37493,#37494,#37495,#37496,#37497,#37498,#37499,#37500,#37501,#37502,
#37503,#37504,#37505,#37506,#37507,#37508,#37509,#37510,#37511,#37512,#37513,
#37514,#37515,#37516,#37517,#37518,#37519,#37520,#37521,#37522,#37523,#37524,
#37525,#37526,#37527,#37528,#37529,#37530,#37531,#37532,#37533,#37534,#37535,
#37536,#37537,#37538,#37539,#37540,#37541,#37542),.UNSPECIFIED.,.F.,.F.)
B_SPLINE_CURVE_WITH_KNOTS((6,1,1,1,1,1,1,1,1,1,1,1,1,1,1,1,1,1,1,1,1,1,
1,1,1,1,1,1,1,1,1,1,1,1,1,1,1,1,1,1,1,1,1,1,1,1,1,1,1,1,1,1,1,1,1,1,1,1,
1,1,1,1,1,1,1,6),(-1.,-0.984615384615383,-0.969230769230768,-0.953846153846152,
-0.938461538461537,-0.923076923076922,-0.907692307692306,-0.892307692307691,
-0.876923076923076,-0.86153846153846,-0.846153846153845,-0.83076923076923,
-0.815384615384614,-0.799999999999999,-0.784615384615384,-0.769230769230768,
-0.753846153846153,-0.738461538461538,-0.723076923076922,-0.707692307692307,
-0.692307692307692,-0.676923076923076,-0.661538461538461,-0.646153846153846,
-0.63076923076923,-0.615384615384615,-0.6,-0.584615384615384,-0.569230769230769,
-0.553846153846154,-0.538461538461538,-0.523076923076923,-0.507692307692308,
-0.492307692307692,-0.476923076923077,-0.461538461538462,-0.446153846153846,
-0.430769230769231,-0.415384615384615,-0.4,-0.384615384615385,-0.369230769230769,
-0.353846153846154,-0.338461538461538,-0.323076923076923,-0.307692307692308,
-0.292307692307692,-0.276923076923077,-0.261538461538462,-0.246153846153846,
-0.230769230769231,-0.215384615384615,-0.2,-0.184615384615385,-0.169230769230769,
-0.153846153846154,-0.138461538461538,-0.123076923076923,-0.107692307692308,
-0.0923076923076923,-0.0769230769230769,-0.0615384615384615,-0.0461538461538462,
-0.0307692307692308,-0.0153846153846154,-0.00577184337450989),
 .UNSPECIFIED.)
CURVE()
GEOMETRIC_REPRESENTATION_ITEM()
RATIONAL_B_SPLINE_CURVE((1.,1.,1.,1.,1.,1.,1.,1.,1.,1.,1.,1.,1.,1.,1.,1.,
1.,1.,1.,1.,1.,1.,1.,1.,1.,1.,1.,1.,1.,1.,1.,1.,1.,1.,1.,1.,1.,1.,1.,1.,
1.,1.,1.,1.,1.,1.,1.,1.,1.,1.,1.,1.,1.,1.,1.,1.,1.,1.,1.,1.,1.,1.,1.,1.,
1.,1.,1.,1.,1.,1.))
REPRESENTATION_ITEM('')
);
#298=(
BOUNDED_CURVE()
B_SPLINE_CURVE(5,(#37693,#37694,#37695,#37696,#37697,#37698,#37699,#37700,
#37701,#37702,#37703,#37704,#37705,#37706,#37707,#37708,#37709,#37710,#37711,
#37712,#37713,#37714,#37715,#37716,#37717,#37718,#37719,#37720,#37721,#37722,
#37723,#37724,#37725,#37726,#37727,#37728,#37729,#37730,#37731,#37732,#37733,
#37734,#37735,#37736,#37737,#37738,#37739,#37740,#37741,#37742,#37743,#37744,
#37745,#37746,#37747,#37748,#37749,#37750,#37751,#37752,#37753,#37754,#37755,
#37756,#37757,#37758,#37759,#37760,#37761,#37762),.UNSPECIFIED.,.F.,.F.)
B_SPLINE_CURVE_WITH_KNOTS((6,1,1,1,1,1,1,1,1,1,1,1,1,1,1,1,1,1,1,1,1,1,
1,1,1,1,1,1,1,1,1,1,1,1,1,1,1,1,1,1,1,1,1,1,1,1,1,1,1,1,1,1,1,1,1,1,1,1,
1,1,1,1,1,1,1,6),(-0.994228156739736,-0.984615384615383,-0.969230769230768,
-0.953846153846152,-0.938461538461537,-0.923076923076922,-0.907692307692306,
-0.892307692307691,-0.876923076923076,-0.86153846153846,-0.846153846153845,
-0.83076923076923,-0.815384615384614,-0.799999999999999,-0.784615384615384,
-0.769230769230768,-0.753846153846153,-0.738461538461538,-0.723076923076922,
-0.707692307692307,-0.692307692307692,-0.676923076923076,-0.661538461538461,
-0.646153846153846,-0.63076923076923,-0.615384615384615,-0.6,-0.584615384615384,
-0.569230769230769,-0.553846153846154,-0.538461538461538,-0.523076923076923,
-0.507692307692308,-0.492307692307692,-0.476923076923077,-0.461538461538462,
-0.446153846153846,-0.430769230769231,-0.415384615384615,-0.4,-0.384615384615385,
-0.369230769230769,-0.353846153846154,-0.338461538461538,-0.323076923076923,
-0.307692307692308,-0.292307692307692,-0.276923076923077,-0.261538461538462,
-0.246153846153846,-0.230769230769231,-0.215384615384615,-0.2,-0.184615384615385,
-0.169230769230769,-0.153846153846154,-0.138461538461538,-0.123076923076923,
-0.107692307692308,-0.0923076923076923,-0.0769230769230769,-0.0615384615384615,
-0.0461538461538462,-0.0307692307692308,-0.0153846153846154,0.),
 .UNSPECIFIED.)
CURVE()
GEOMETRIC_REPRESENTATION_ITEM()
RATIONAL_B_SPLINE_CURVE((1.,1.,1.,1.,1.,1.,1.,1.,1.,1.,1.,1.,1.,1.,1.,1.,
1.,1.,1.,1.,1.,1.,1.,1.,1.,1.,1.,1.,1.,1.,1.,1.,1.,1.,1.,1.,1.,1.,1.,1.,
1.,1.,1.,1.,1.,1.,1.,1.,1.,1.,1.,1.,1.,1.,1.,1.,1.,1.,1.,1.,1.,1.,1.,1.,
1.,1.,1.,1.,1.,1.))
REPRESENTATION_ITEM('')
);
#299=(
BOUNDED_CURVE()
B_SPLINE_CURVE(5,(#37915,#37916,#37917,#37918,#37919,#37920,#37921,#37922,
#37923,#37924,#37925,#37926,#37927,#37928,#37929,#37930,#37931,#37932,#37933,
#37934,#37935,#37936,#37937,#37938,#37939,#37940,#37941,#37942,#37943,#37944,
#37945,#37946,#37947,#37948,#37949,#37950,#37951,#37952,#37953,#37954,#37955,
#37956,#37957,#37958,#37959,#37960,#37961,#37962,#37963,#37964,#37965,#37966,
#37967,#37968,#37969,#37970,#37971,#37972,#37973,#37974,#37975,#37976,#37977,
#37978,#37979,#37980,#37981,#37982,#37983,#37984),.UNSPECIFIED.,.F.,.F.)
B_SPLINE_CURVE_WITH_KNOTS((6,1,1,1,1,1,1,1,1,1,1,1,1,1,1,1,1,1,1,1,1,1,
1,1,1,1,1,1,1,1,1,1,1,1,1,1,1,1,1,1,1,1,1,1,1,1,1,1,1,1,1,1,1,1,1,1,1,1,
1,1,1,1,1,1,1,6),(-1.,-0.984615384615383,-0.969230769230768,-0.953846153846152,
-0.938461538461537,-0.923076923076922,-0.907692307692306,-0.892307692307691,
-0.876923076923076,-0.86153846153846,-0.846153846153845,-0.83076923076923,
-0.815384615384614,-0.799999999999999,-0.784615384615384,-0.769230769230768,
-0.753846153846153,-0.738461538461538,-0.723076923076922,-0.707692307692307,
-0.692307692307692,-0.676923076923076,-0.661538461538461,-0.646153846153846,
-0.63076923076923,-0.615384615384615,-0.6,-0.584615384615384,-0.569230769230769,
-0.553846153846154,-0.538461538461538,-0.523076923076923,-0.507692307692308,
-0.492307692307692,-0.476923076923077,-0.461538461538462,-0.446153846153846,
-0.430769230769231,-0.415384615384615,-0.4,-0.384615384615385,-0.369230769230769,
-0.353846153846154,-0.338461538461538,-0.323076923076923,-0.307692307692308,
-0.292307692307692,-0.276923076923077,-0.261538461538462,-0.246153846153846,
-0.230769230769231,-0.215384615384615,-0.2,-0.184615384615385,-0.169230769230769,
-0.153846153846154,-0.138461538461538,-0.123076923076923,-0.107692307692308,
-0.0923076923076923,-0.0769230769230769,-0.0615384615384615,-0.0461538461538462,
-0.0307692307692308,-0.0153846153846154,-0.00577184337452469),
 .UNSPECIFIED.)
CURVE()
GEOMETRIC_REPRESENTATION_ITEM()
RATIONAL_B_SPLINE_CURVE((1.,1.,1.,1.,1.,1.,1.,1.,1.,1.,1.,1.,1.,1.,1.,1.,
1.,1.,1.,1.,1.,1.,1.,1.,1.,1.,1.,1.,1.,1.,1.,1.,1.,1.,1.,1.,1.,1.,1.,1.,
1.,1.,1.,1.,1.,1.,1.,1.,1.,1.,1.,1.,1.,1.,1.,1.,1.,1.,1.,1.,1.,1.,1.,1.,
1.,1.,1.,1.,1.,1.))
REPRESENTATION_ITEM('')
);
#300=(
BOUNDED_CURVE()
B_SPLINE_CURVE(5,(#38135,#38136,#38137,#38138,#38139,#38140,#38141,#38142,
#38143,#38144,#38145,#38146,#38147,#38148,#38149,#38150,#38151,#38152,#38153,
#38154,#38155,#38156,#38157,#38158,#38159,#38160,#38161,#38162,#38163,#38164,
#38165,#38166,#38167,#38168,#38169,#38170,#38171,#38172,#38173,#38174,#38175,
#38176,#38177,#38178,#38179,#38180,#38181,#38182,#38183,#38184,#38185,#38186,
#38187,#38188,#38189,#38190,#38191,#38192,#38193,#38194,#38195,#38196,#38197,
#38198,#38199,#38200,#38201,#38202,#38203,#38204),.UNSPECIFIED.,.F.,.F.)
B_SPLINE_CURVE_WITH_KNOTS((6,1,1,1,1,1,1,1,1,1,1,1,1,1,1,1,1,1,1,1,1,1,
1,1,1,1,1,1,1,1,1,1,1,1,1,1,1,1,1,1,1,1,1,1,1,1,1,1,1,1,1,1,1,1,1,1,1,1,
1,1,1,1,1,1,1,6),(-0.994228156739717,-0.984615384615383,-0.969230769230768,
-0.953846153846152,-0.938461538461537,-0.923076923076922,-0.907692307692306,
-0.892307692307691,-0.876923076923076,-0.86153846153846,-0.846153846153845,
-0.83076923076923,-0.815384615384614,-0.799999999999999,-0.784615384615384,
-0.769230769230768,-0.753846153846153,-0.738461538461538,-0.723076923076922,
-0.707692307692307,-0.692307692307692,-0.676923076923076,-0.661538461538461,
-0.646153846153846,-0.63076923076923,-0.615384615384615,-0.6,-0.584615384615384,
-0.569230769230769,-0.553846153846154,-0.538461538461538,-0.523076923076923,
-0.507692307692308,-0.492307692307692,-0.476923076923077,-0.461538461538462,
-0.446153846153846,-0.430769230769231,-0.415384615384615,-0.4,-0.384615384615385,
-0.369230769230769,-0.353846153846154,-0.338461538461538,-0.323076923076923,
-0.307692307692308,-0.292307692307692,-0.276923076923077,-0.261538461538462,
-0.246153846153846,-0.230769230769231,-0.215384615384615,-0.2,-0.184615384615385,
-0.169230769230769,-0.153846153846154,-0.138461538461538,-0.123076923076923,
-0.107692307692308,-0.0923076923076923,-0.0769230769230769,-0.0615384615384615,
-0.0461538461538462,-0.0307692307692308,-0.0153846153846154,0.),
 .UNSPECIFIED.)
CURVE()
GEOMETRIC_REPRESENTATION_ITEM()
RATIONAL_B_SPLINE_CURVE((1.,1.,1.,1.,1.,1.,1.,1.,1.,1.,1.,1.,1.,1.,1.,1.,
1.,1.,1.,1.,1.,1.,1.,1.,1.,1.,1.,1.,1.,1.,1.,1.,1.,1.,1.,1.,1.,1.,1.,1.,
1.,1.,1.,1.,1.,1.,1.,1.,1.,1.,1.,1.,1.,1.,1.,1.,1.,1.,1.,1.,1.,1.,1.,1.,
1.,1.,1.,1.,1.,1.))
REPRESENTATION_ITEM('')
);
#301=(
BOUNDED_CURVE()
B_SPLINE_CURVE(5,(#38357,#38358,#38359,#38360,#38361,#38362,#38363,#38364,
#38365,#38366,#38367,#38368,#38369,#38370,#38371,#38372,#38373,#38374,#38375,
#38376,#38377,#38378,#38379,#38380,#38381,#38382,#38383,#38384,#38385,#38386,
#38387,#38388,#38389,#38390,#38391,#38392,#38393,#38394,#38395,#38396,#38397,
#38398,#38399,#38400,#38401,#38402,#38403,#38404,#38405,#38406,#38407,#38408,
#38409,#38410,#38411,#38412,#38413,#38414,#38415,#38416,#38417,#38418,#38419,
#38420,#38421,#38422,#38423,#38424,#38425,#38426),.UNSPECIFIED.,.F.,.F.)
B_SPLINE_CURVE_WITH_KNOTS((6,1,1,1,1,1,1,1,1,1,1,1,1,1,1,1,1,1,1,1,1,1,
1,1,1,1,1,1,1,1,1,1,1,1,1,1,1,1,1,1,1,1,1,1,1,1,1,1,1,1,1,1,1,1,1,1,1,1,
1,1,1,1,1,1,1,6),(-1.,-0.984615384615383,-0.969230769230768,-0.953846153846152,
-0.938461538461537,-0.923076923076922,-0.907692307692306,-0.892307692307691,
-0.876923076923076,-0.86153846153846,-0.846153846153845,-0.83076923076923,
-0.815384615384614,-0.799999999999999,-0.784615384615384,-0.769230769230768,
-0.753846153846153,-0.738461538461538,-0.723076923076922,-0.707692307692307,
-0.692307692307692,-0.676923076923076,-0.661538461538461,-0.646153846153846,
-0.63076923076923,-0.615384615384615,-0.6,-0.584615384615384,-0.569230769230769,
-0.553846153846154,-0.538461538461538,-0.523076923076923,-0.507692307692308,
-0.492307692307692,-0.476923076923077,-0.461538461538462,-0.446153846153846,
-0.430769230769231,-0.415384615384615,-0.4,-0.384615384615385,-0.369230769230769,
-0.353846153846154,-0.338461538461538,-0.323076923076923,-0.307692307692308,
-0.292307692307692,-0.276923076923077,-0.261538461538462,-0.246153846153846,
-0.230769230769231,-0.215384615384615,-0.2,-0.184615384615385,-0.169230769230769,
-0.153846153846154,-0.138461538461538,-0.123076923076923,-0.107692307692308,
-0.0923076923076923,-0.0769230769230769,-0.0615384615384615,-0.0461538461538462,
-0.0307692307692308,-0.0153846153846154,-0.00577184337453472),
 .UNSPECIFIED.)
CURVE()
GEOMETRIC_REPRESENTATION_ITEM()
RATIONAL_B_SPLINE_CURVE((1.,1.,1.,1.,1.,1.,1.,1.,1.,1.,1.,1.,1.,1.,1.,1.,
1.,1.,1.,1.,1.,1.,1.,1.,1.,1.,1.,1.,1.,1.,1.,1.,1.,1.,1.,1.,1.,1.,1.,1.,
1.,1.,1.,1.,1.,1.,1.,1.,1.,1.,1.,1.,1.,1.,1.,1.,1.,1.,1.,1.,1.,1.,1.,1.,
1.,1.,1.,1.,1.,1.))
REPRESENTATION_ITEM('')
);
#302=(
BOUNDED_CURVE()
B_SPLINE_CURVE(5,(#38577,#38578,#38579,#38580,#38581,#38582,#38583,#38584,
#38585,#38586,#38587,#38588,#38589,#38590,#38591,#38592,#38593,#38594,#38595,
#38596,#38597,#38598,#38599,#38600,#38601,#38602,#38603,#38604,#38605,#38606,
#38607,#38608,#38609,#38610,#38611,#38612,#38613,#38614,#38615,#38616,#38617,
#38618,#38619,#38620,#38621,#38622,#38623,#38624,#38625,#38626,#38627,#38628,
#38629,#38630,#38631,#38632,#38633,#38634,#38635,#38636,#38637,#38638,#38639,
#38640,#38641,#38642,#38643,#38644,#38645,#38646),.UNSPECIFIED.,.F.,.F.)
B_SPLINE_CURVE_WITH_KNOTS((6,1,1,1,1,1,1,1,1,1,1,1,1,1,1,1,1,1,1,1,1,1,
1,1,1,1,1,1,1,1,1,1,1,1,1,1,1,1,1,1,1,1,1,1,1,1,1,1,1,1,1,1,1,1,1,1,1,1,
1,1,1,1,1,1,1,6),(-0.994228156739652,-0.984615384615383,-0.969230769230768,
-0.953846153846152,-0.938461538461537,-0.923076923076922,-0.907692307692306,
-0.892307692307691,-0.876923076923076,-0.86153846153846,-0.846153846153845,
-0.83076923076923,-0.815384615384614,-0.799999999999999,-0.784615384615384,
-0.769230769230768,-0.753846153846153,-0.738461538461538,-0.723076923076922,
-0.707692307692307,-0.692307692307692,-0.676923076923076,-0.661538461538461,
-0.646153846153846,-0.63076923076923,-0.615384615384615,-0.6,-0.584615384615384,
-0.569230769230769,-0.553846153846154,-0.538461538461538,-0.523076923076923,
-0.507692307692308,-0.492307692307692,-0.476923076923077,-0.461538461538462,
-0.446153846153846,-0.430769230769231,-0.415384615384615,-0.4,-0.384615384615385,
-0.369230769230769,-0.353846153846154,-0.338461538461538,-0.323076923076923,
-0.307692307692308,-0.292307692307692,-0.276923076923077,-0.261538461538462,
-0.246153846153846,-0.230769230769231,-0.215384615384615,-0.2,-0.184615384615385,
-0.169230769230769,-0.153846153846154,-0.138461538461538,-0.123076923076923,
-0.107692307692308,-0.0923076923076923,-0.0769230769230769,-0.0615384615384615,
-0.0461538461538462,-0.0307692307692308,-0.0153846153846154,0.),
 .UNSPECIFIED.)
CURVE()
GEOMETRIC_REPRESENTATION_ITEM()
RATIONAL_B_SPLINE_CURVE((1.,1.,1.,1.,1.,1.,1.,1.,1.,1.,1.,1.,1.,1.,1.,1.,
1.,1.,1.,1.,1.,1.,1.,1.,1.,1.,1.,1.,1.,1.,1.,1.,1.,1.,1.,1.,1.,1.,1.,1.,
1.,1.,1.,1.,1.,1.,1.,1.,1.,1.,1.,1.,1.,1.,1.,1.,1.,1.,1.,1.,1.,1.,1.,1.,
1.,1.,1.,1.,1.,1.))
REPRESENTATION_ITEM('')
);
#303=(
BOUNDED_CURVE()
B_SPLINE_CURVE(5,(#38799,#38800,#38801,#38802,#38803,#38804,#38805,#38806,
#38807,#38808,#38809,#38810,#38811,#38812,#38813,#38814,#38815,#38816,#38817,
#38818,#38819,#38820,#38821,#38822,#38823,#38824,#38825,#38826,#38827,#38828,
#38829,#38830,#38831,#38832,#38833,#38834,#38835,#38836,#38837,#38838,#38839,
#38840,#38841,#38842,#38843,#38844,#38845,#38846,#38847,#38848,#38849,#38850,
#38851,#38852,#38853,#38854,#38855,#38856,#38857,#38858,#38859,#38860,#38861,
#38862,#38863,#38864,#38865,#38866,#38867,#38868),.UNSPECIFIED.,.F.,.F.)
B_SPLINE_CURVE_WITH_KNOTS((6,1,1,1,1,1,1,1,1,1,1,1,1,1,1,1,1,1,1,1,1,1,
1,1,1,1,1,1,1,1,1,1,1,1,1,1,1,1,1,1,1,1,1,1,1,1,1,1,1,1,1,1,1,1,1,1,1,1,
1,1,1,1,1,1,1,6),(-1.,-0.984615384615383,-0.969230769230768,-0.953846153846152,
-0.938461538461537,-0.923076923076922,-0.907692307692306,-0.892307692307691,
-0.876923076923076,-0.86153846153846,-0.846153846153845,-0.83076923076923,
-0.815384615384614,-0.799999999999999,-0.784615384615384,-0.769230769230768,
-0.753846153846153,-0.738461538461538,-0.723076923076922,-0.707692307692307,
-0.692307692307692,-0.676923076923076,-0.661538461538461,-0.646153846153846,
-0.63076923076923,-0.615384615384615,-0.6,-0.584615384615384,-0.569230769230769,
-0.553846153846154,-0.538461538461538,-0.523076923076923,-0.507692307692308,
-0.492307692307692,-0.476923076923077,-0.461538461538462,-0.446153846153846,
-0.430769230769231,-0.415384615384615,-0.4,-0.384615384615385,-0.369230769230769,
-0.353846153846154,-0.338461538461538,-0.323076923076923,-0.307692307692308,
-0.292307692307692,-0.276923076923077,-0.261538461538462,-0.246153846153846,
-0.230769230769231,-0.215384615384615,-0.2,-0.184615384615385,-0.169230769230769,
-0.153846153846154,-0.138461538461538,-0.123076923076923,-0.107692307692308,
-0.0923076923076923,-0.0769230769230769,-0.0615384615384615,-0.0461538461538462,
-0.0307692307692308,-0.0153846153846154,-0.00577184337450876),
 .UNSPECIFIED.)
CURVE()
GEOMETRIC_REPRESENTATION_ITEM()
RATIONAL_B_SPLINE_CURVE((1.,1.,1.,1.,1.,1.,1.,1.,1.,1.,1.,1.,1.,1.,1.,1.,
1.,1.,1.,1.,1.,1.,1.,1.,1.,1.,1.,1.,1.,1.,1.,1.,1.,1.,1.,1.,1.,1.,1.,1.,
1.,1.,1.,1.,1.,1.,1.,1.,1.,1.,1.,1.,1.,1.,1.,1.,1.,1.,1.,1.,1.,1.,1.,1.,
1.,1.,1.,1.,1.,1.))
REPRESENTATION_ITEM('')
);
#304=(
BOUNDED_CURVE()
B_SPLINE_CURVE(5,(#39019,#39020,#39021,#39022,#39023,#39024,#39025,#39026,
#39027,#39028,#39029,#39030,#39031,#39032,#39033,#39034,#39035,#39036,#39037,
#39038,#39039,#39040,#39041,#39042,#39043,#39044,#39045,#39046,#39047,#39048,
#39049,#39050,#39051,#39052,#39053,#39054,#39055,#39056,#39057,#39058,#39059,
#39060,#39061,#39062,#39063,#39064,#39065,#39066,#39067,#39068,#39069,#39070,
#39071,#39072,#39073,#39074,#39075,#39076,#39077,#39078,#39079,#39080,#39081,
#39082,#39083,#39084,#39085,#39086,#39087,#39088),.UNSPECIFIED.,.F.,.F.)
B_SPLINE_CURVE_WITH_KNOTS((6,1,1,1,1,1,1,1,1,1,1,1,1,1,1,1,1,1,1,1,1,1,
1,1,1,1,1,1,1,1,1,1,1,1,1,1,1,1,1,1,1,1,1,1,1,1,1,1,1,1,1,1,1,1,1,1,1,1,
1,1,1,1,1,1,1,6),(-0.994228156739683,-0.984615384615383,-0.969230769230768,
-0.953846153846152,-0.938461538461537,-0.923076923076922,-0.907692307692306,
-0.892307692307691,-0.876923076923076,-0.86153846153846,-0.846153846153845,
-0.83076923076923,-0.815384615384614,-0.799999999999999,-0.784615384615384,
-0.769230769230768,-0.753846153846153,-0.738461538461538,-0.723076923076922,
-0.707692307692307,-0.692307692307692,-0.676923076923076,-0.661538461538461,
-0.646153846153846,-0.63076923076923,-0.615384615384615,-0.6,-0.584615384615384,
-0.569230769230769,-0.553846153846154,-0.538461538461538,-0.523076923076923,
-0.507692307692308,-0.492307692307692,-0.476923076923077,-0.461538461538462,
-0.446153846153846,-0.430769230769231,-0.415384615384615,-0.4,-0.384615384615385,
-0.369230769230769,-0.353846153846154,-0.338461538461538,-0.323076923076923,
-0.307692307692308,-0.292307692307692,-0.276923076923077,-0.261538461538462,
-0.246153846153846,-0.230769230769231,-0.215384615384615,-0.2,-0.184615384615385,
-0.169230769230769,-0.153846153846154,-0.138461538461538,-0.123076923076923,
-0.107692307692308,-0.0923076923076923,-0.0769230769230769,-0.0615384615384615,
-0.0461538461538462,-0.0307692307692308,-0.0153846153846154,0.),
 .UNSPECIFIED.)
CURVE()
GEOMETRIC_REPRESENTATION_ITEM()
RATIONAL_B_SPLINE_CURVE((1.,1.,1.,1.,1.,1.,1.,1.,1.,1.,1.,1.,1.,1.,1.,1.,
1.,1.,1.,1.,1.,1.,1.,1.,1.,1.,1.,1.,1.,1.,1.,1.,1.,1.,1.,1.,1.,1.,1.,1.,
1.,1.,1.,1.,1.,1.,1.,1.,1.,1.,1.,1.,1.,1.,1.,1.,1.,1.,1.,1.,1.,1.,1.,1.,
1.,1.,1.,1.,1.,1.))
REPRESENTATION_ITEM('')
);
#305=(
BOUNDED_CURVE()
B_SPLINE_CURVE(5,(#39241,#39242,#39243,#39244,#39245,#39246,#39247,#39248,
#39249,#39250,#39251,#39252,#39253,#39254,#39255,#39256,#39257,#39258,#39259,
#39260,#39261,#39262,#39263,#39264,#39265,#39266,#39267,#39268,#39269,#39270,
#39271,#39272,#39273,#39274,#39275,#39276,#39277,#39278,#39279,#39280,#39281,
#39282,#39283,#39284,#39285,#39286,#39287,#39288,#39289,#39290,#39291,#39292,
#39293,#39294,#39295,#39296,#39297,#39298,#39299,#39300,#39301,#39302,#39303,
#39304,#39305,#39306,#39307,#39308,#39309,#39310),.UNSPECIFIED.,.F.,.F.)
B_SPLINE_CURVE_WITH_KNOTS((6,1,1,1,1,1,1,1,1,1,1,1,1,1,1,1,1,1,1,1,1,1,
1,1,1,1,1,1,1,1,1,1,1,1,1,1,1,1,1,1,1,1,1,1,1,1,1,1,1,1,1,1,1,1,1,1,1,1,
1,1,1,1,1,1,1,6),(-1.,-0.984615384615383,-0.969230769230768,-0.953846153846152,
-0.938461538461537,-0.923076923076922,-0.907692307692306,-0.892307692307691,
-0.876923076923076,-0.86153846153846,-0.846153846153845,-0.83076923076923,
-0.815384615384614,-0.799999999999999,-0.784615384615384,-0.769230769230768,
-0.753846153846153,-0.738461538461538,-0.723076923076922,-0.707692307692307,
-0.692307692307692,-0.676923076923076,-0.661538461538461,-0.646153846153846,
-0.63076923076923,-0.615384615384615,-0.6,-0.584615384615384,-0.569230769230769,
-0.553846153846154,-0.538461538461538,-0.523076923076923,-0.507692307692308,
-0.492307692307692,-0.476923076923077,-0.461538461538462,-0.446153846153846,
-0.430769230769231,-0.415384615384615,-0.4,-0.384615384615385,-0.369230769230769,
-0.353846153846154,-0.338461538461538,-0.323076923076923,-0.307692307692308,
-0.292307692307692,-0.276923076923077,-0.261538461538462,-0.246153846153846,
-0.230769230769231,-0.215384615384615,-0.2,-0.184615384615385,-0.169230769230769,
-0.153846153846154,-0.138461538461538,-0.123076923076923,-0.107692307692308,
-0.0923076923076923,-0.0769230769230769,-0.0615384615384615,-0.0461538461538462,
-0.0307692307692308,-0.0153846153846154,-0.00577184337450277),
 .UNSPECIFIED.)
CURVE()
GEOMETRIC_REPRESENTATION_ITEM()
RATIONAL_B_SPLINE_CURVE((1.,1.,1.,1.,1.,1.,1.,1.,1.,1.,1.,1.,1.,1.,1.,1.,
1.,1.,1.,1.,1.,1.,1.,1.,1.,1.,1.,1.,1.,1.,1.,1.,1.,1.,1.,1.,1.,1.,1.,1.,
1.,1.,1.,1.,1.,1.,1.,1.,1.,1.,1.,1.,1.,1.,1.,1.,1.,1.,1.,1.,1.,1.,1.,1.,
1.,1.,1.,1.,1.,1.))
REPRESENTATION_ITEM('')
);
#306=(
BOUNDED_CURVE()
B_SPLINE_CURVE(5,(#39461,#39462,#39463,#39464,#39465,#39466,#39467,#39468,
#39469,#39470,#39471,#39472,#39473,#39474,#39475,#39476,#39477,#39478,#39479,
#39480,#39481,#39482,#39483,#39484,#39485,#39486,#39487,#39488,#39489,#39490,
#39491,#39492,#39493,#39494,#39495,#39496,#39497,#39498,#39499,#39500,#39501,
#39502,#39503,#39504,#39505,#39506,#39507,#39508,#39509,#39510,#39511,#39512,
#39513,#39514,#39515,#39516,#39517,#39518,#39519,#39520,#39521,#39522,#39523,
#39524,#39525,#39526,#39527,#39528,#39529,#39530),.UNSPECIFIED.,.F.,.F.)
B_SPLINE_CURVE_WITH_KNOTS((6,1,1,1,1,1,1,1,1,1,1,1,1,1,1,1,1,1,1,1,1,1,
1,1,1,1,1,1,1,1,1,1,1,1,1,1,1,1,1,1,1,1,1,1,1,1,1,1,1,1,1,1,1,1,1,1,1,1,
1,1,1,1,1,1,1,6),(-0.994228156739689,-0.984615384615383,-0.969230769230768,
-0.953846153846152,-0.938461538461537,-0.923076923076922,-0.907692307692306,
-0.892307692307691,-0.876923076923076,-0.86153846153846,-0.846153846153845,
-0.83076923076923,-0.815384615384614,-0.799999999999999,-0.784615384615384,
-0.769230769230768,-0.753846153846153,-0.738461538461538,-0.723076923076922,
-0.707692307692307,-0.692307692307692,-0.676923076923076,-0.661538461538461,
-0.646153846153846,-0.63076923076923,-0.615384615384615,-0.6,-0.584615384615384,
-0.569230769230769,-0.553846153846154,-0.538461538461538,-0.523076923076923,
-0.507692307692308,-0.492307692307692,-0.476923076923077,-0.461538461538462,
-0.446153846153846,-0.430769230769231,-0.415384615384615,-0.4,-0.384615384615385,
-0.369230769230769,-0.353846153846154,-0.338461538461538,-0.323076923076923,
-0.307692307692308,-0.292307692307692,-0.276923076923077,-0.261538461538462,
-0.246153846153846,-0.230769230769231,-0.215384615384615,-0.2,-0.184615384615385,
-0.169230769230769,-0.153846153846154,-0.138461538461538,-0.123076923076923,
-0.107692307692308,-0.0923076923076923,-0.0769230769230769,-0.0615384615384615,
-0.0461538461538462,-0.0307692307692308,-0.0153846153846154,0.),
 .UNSPECIFIED.)
CURVE()
GEOMETRIC_REPRESENTATION_ITEM()
RATIONAL_B_SPLINE_CURVE((1.,1.,1.,1.,1.,1.,1.,1.,1.,1.,1.,1.,1.,1.,1.,1.,
1.,1.,1.,1.,1.,1.,1.,1.,1.,1.,1.,1.,1.,1.,1.,1.,1.,1.,1.,1.,1.,1.,1.,1.,
1.,1.,1.,1.,1.,1.,1.,1.,1.,1.,1.,1.,1.,1.,1.,1.,1.,1.,1.,1.,1.,1.,1.,1.,
1.,1.,1.,1.,1.,1.))
REPRESENTATION_ITEM('')
);
#307=(
BOUNDED_CURVE()
B_SPLINE_CURVE(5,(#39683,#39684,#39685,#39686,#39687,#39688,#39689,#39690,
#39691,#39692,#39693,#39694,#39695,#39696,#39697,#39698,#39699,#39700,#39701,
#39702,#39703,#39704,#39705,#39706,#39707,#39708,#39709,#39710,#39711,#39712,
#39713,#39714,#39715,#39716,#39717,#39718,#39719,#39720,#39721,#39722,#39723,
#39724,#39725,#39726,#39727,#39728,#39729,#39730,#39731,#39732,#39733,#39734,
#39735,#39736,#39737,#39738,#39739,#39740,#39741,#39742,#39743,#39744,#39745,
#39746,#39747,#39748,#39749,#39750,#39751,#39752),.UNSPECIFIED.,.F.,.F.)
B_SPLINE_CURVE_WITH_KNOTS((6,1,1,1,1,1,1,1,1,1,1,1,1,1,1,1,1,1,1,1,1,1,
1,1,1,1,1,1,1,1,1,1,1,1,1,1,1,1,1,1,1,1,1,1,1,1,1,1,1,1,1,1,1,1,1,1,1,1,
1,1,1,1,1,1,1,6),(-1.,-0.984615384615383,-0.969230769230768,-0.953846153846152,
-0.938461538461537,-0.923076923076922,-0.907692307692306,-0.892307692307691,
-0.876923076923076,-0.86153846153846,-0.846153846153845,-0.83076923076923,
-0.815384615384614,-0.799999999999999,-0.784615384615384,-0.769230769230768,
-0.753846153846153,-0.738461538461538,-0.723076923076922,-0.707692307692307,
-0.692307692307692,-0.676923076923076,-0.661538461538461,-0.646153846153846,
-0.63076923076923,-0.615384615384615,-0.6,-0.584615384615384,-0.569230769230769,
-0.553846153846154,-0.538461538461538,-0.523076923076923,-0.507692307692308,
-0.492307692307692,-0.476923076923077,-0.461538461538462,-0.446153846153846,
-0.430769230769231,-0.415384615384615,-0.4,-0.384615384615385,-0.369230769230769,
-0.353846153846154,-0.338461538461538,-0.323076923076923,-0.307692307692308,
-0.292307692307692,-0.276923076923077,-0.261538461538462,-0.246153846153846,
-0.230769230769231,-0.215384615384615,-0.2,-0.184615384615385,-0.169230769230769,
-0.153846153846154,-0.138461538461538,-0.123076923076923,-0.107692307692308,
-0.0923076923076923,-0.0769230769230769,-0.0615384615384615,-0.0461538461538462,
-0.0307692307692308,-0.0153846153846154,-0.00577184337451766),
 .UNSPECIFIED.)
CURVE()
GEOMETRIC_REPRESENTATION_ITEM()
RATIONAL_B_SPLINE_CURVE((1.,1.,1.,1.,1.,1.,1.,1.,1.,1.,1.,1.,1.,1.,1.,1.,
1.,1.,1.,1.,1.,1.,1.,1.,1.,1.,1.,1.,1.,1.,1.,1.,1.,1.,1.,1.,1.,1.,1.,1.,
1.,1.,1.,1.,1.,1.,1.,1.,1.,1.,1.,1.,1.,1.,1.,1.,1.,1.,1.,1.,1.,1.,1.,1.,
1.,1.,1.,1.,1.,1.))
REPRESENTATION_ITEM('')
);
#308=(
BOUNDED_CURVE()
B_SPLINE_CURVE(5,(#39903,#39904,#39905,#39906,#39907,#39908,#39909,#39910,
#39911,#39912,#39913,#39914,#39915,#39916,#39917,#39918,#39919,#39920,#39921,
#39922,#39923,#39924,#39925,#39926,#39927,#39928,#39929,#39930,#39931,#39932,
#39933,#39934,#39935,#39936,#39937,#39938,#39939,#39940,#39941,#39942,#39943,
#39944,#39945,#39946,#39947,#39948,#39949,#39950,#39951,#39952,#39953,#39954,
#39955,#39956,#39957,#39958,#39959,#39960,#39961,#39962,#39963,#39964,#39965,
#39966,#39967,#39968,#39969,#39970,#39971,#39972),.UNSPECIFIED.,.F.,.F.)
B_SPLINE_CURVE_WITH_KNOTS((6,1,1,1,1,1,1,1,1,1,1,1,1,1,1,1,1,1,1,1,1,1,
1,1,1,1,1,1,1,1,1,1,1,1,1,1,1,1,1,1,1,1,1,1,1,1,1,1,1,1,1,1,1,1,1,1,1,1,
1,1,1,1,1,1,1,6),(-0.994228156739687,-0.984615384615383,-0.969230769230768,
-0.953846153846152,-0.938461538461537,-0.923076923076922,-0.907692307692306,
-0.892307692307691,-0.876923076923076,-0.86153846153846,-0.846153846153845,
-0.83076923076923,-0.815384615384614,-0.799999999999999,-0.784615384615384,
-0.769230769230768,-0.753846153846153,-0.738461538461538,-0.723076923076922,
-0.707692307692307,-0.692307692307692,-0.676923076923076,-0.661538461538461,
-0.646153846153846,-0.63076923076923,-0.615384615384615,-0.6,-0.584615384615384,
-0.569230769230769,-0.553846153846154,-0.538461538461538,-0.523076923076923,
-0.507692307692308,-0.492307692307692,-0.476923076923077,-0.461538461538462,
-0.446153846153846,-0.430769230769231,-0.415384615384615,-0.4,-0.384615384615385,
-0.369230769230769,-0.353846153846154,-0.338461538461538,-0.323076923076923,
-0.307692307692308,-0.292307692307692,-0.276923076923077,-0.261538461538462,
-0.246153846153846,-0.230769230769231,-0.215384615384615,-0.2,-0.184615384615385,
-0.169230769230769,-0.153846153846154,-0.138461538461538,-0.123076923076923,
-0.107692307692308,-0.0923076923076923,-0.0769230769230769,-0.0615384615384615,
-0.0461538461538462,-0.0307692307692308,-0.0153846153846154,0.),
 .UNSPECIFIED.)
CURVE()
GEOMETRIC_REPRESENTATION_ITEM()
RATIONAL_B_SPLINE_CURVE((1.,1.,1.,1.,1.,1.,1.,1.,1.,1.,1.,1.,1.,1.,1.,1.,
1.,1.,1.,1.,1.,1.,1.,1.,1.,1.,1.,1.,1.,1.,1.,1.,1.,1.,1.,1.,1.,1.,1.,1.,
1.,1.,1.,1.,1.,1.,1.,1.,1.,1.,1.,1.,1.,1.,1.,1.,1.,1.,1.,1.,1.,1.,1.,1.,
1.,1.,1.,1.,1.,1.))
REPRESENTATION_ITEM('')
);
#309=(
BOUNDED_CURVE()
B_SPLINE_CURVE(5,(#40125,#40126,#40127,#40128,#40129,#40130,#40131,#40132,
#40133,#40134,#40135,#40136,#40137,#40138,#40139,#40140,#40141,#40142,#40143,
#40144,#40145,#40146,#40147,#40148,#40149,#40150,#40151,#40152,#40153,#40154,
#40155,#40156,#40157,#40158,#40159,#40160,#40161,#40162,#40163,#40164,#40165,
#40166,#40167,#40168,#40169,#40170,#40171,#40172,#40173,#40174,#40175,#40176,
#40177,#40178,#40179,#40180,#40181,#40182,#40183,#40184,#40185,#40186,#40187,
#40188,#40189,#40190,#40191,#40192,#40193,#40194),.UNSPECIFIED.,.F.,.F.)
B_SPLINE_CURVE_WITH_KNOTS((6,1,1,1,1,1,1,1,1,1,1,1,1,1,1,1,1,1,1,1,1,1,
1,1,1,1,1,1,1,1,1,1,1,1,1,1,1,1,1,1,1,1,1,1,1,1,1,1,1,1,1,1,1,1,1,1,1,1,
1,1,1,1,1,1,1,6),(-1.,-0.984615384615383,-0.969230769230768,-0.953846153846152,
-0.938461538461537,-0.923076923076922,-0.907692307692306,-0.892307692307691,
-0.876923076923076,-0.86153846153846,-0.846153846153845,-0.83076923076923,
-0.815384615384614,-0.799999999999999,-0.784615384615384,-0.769230769230768,
-0.753846153846153,-0.738461538461538,-0.723076923076922,-0.707692307692307,
-0.692307692307692,-0.676923076923076,-0.661538461538461,-0.646153846153846,
-0.63076923076923,-0.615384615384615,-0.6,-0.584615384615384,-0.569230769230769,
-0.553846153846154,-0.538461538461538,-0.523076923076923,-0.507692307692308,
-0.492307692307692,-0.476923076923077,-0.461538461538462,-0.446153846153846,
-0.430769230769231,-0.415384615384615,-0.4,-0.384615384615385,-0.369230769230769,
-0.353846153846154,-0.338461538461538,-0.323076923076923,-0.307692307692308,
-0.292307692307692,-0.276923076923077,-0.261538461538462,-0.246153846153846,
-0.230769230769231,-0.215384615384615,-0.2,-0.184615384615385,-0.169230769230769,
-0.153846153846154,-0.138461538461538,-0.123076923076923,-0.107692307692308,
-0.0923076923076923,-0.0769230769230769,-0.0615384615384615,-0.0461538461538462,
-0.0307692307692308,-0.0153846153846154,-0.00577184337452512),
 .UNSPECIFIED.)
CURVE()
GEOMETRIC_REPRESENTATION_ITEM()
RATIONAL_B_SPLINE_CURVE((1.,1.,1.,1.,1.,1.,1.,1.,1.,1.,1.,1.,1.,1.,1.,1.,
1.,1.,1.,1.,1.,1.,1.,1.,1.,1.,1.,1.,1.,1.,1.,1.,1.,1.,1.,1.,1.,1.,1.,1.,
1.,1.,1.,1.,1.,1.,1.,1.,1.,1.,1.,1.,1.,1.,1.,1.,1.,1.,1.,1.,1.,1.,1.,1.,
1.,1.,1.,1.,1.,1.))
REPRESENTATION_ITEM('')
);
#310=(
BOUNDED_CURVE()
B_SPLINE_CURVE(5,(#40345,#40346,#40347,#40348,#40349,#40350,#40351,#40352,
#40353,#40354,#40355,#40356,#40357,#40358,#40359,#40360,#40361,#40362,#40363,
#40364,#40365,#40366,#40367,#40368,#40369,#40370,#40371,#40372,#40373,#40374,
#40375,#40376,#40377,#40378,#40379,#40380,#40381,#40382,#40383,#40384,#40385,
#40386,#40387,#40388,#40389,#40390,#40391,#40392,#40393,#40394,#40395,#40396,
#40397,#40398,#40399,#40400,#40401,#40402,#40403,#40404,#40405,#40406,#40407,
#40408,#40409,#40410,#40411,#40412,#40413,#40414),.UNSPECIFIED.,.F.,.F.)
B_SPLINE_CURVE_WITH_KNOTS((6,1,1,1,1,1,1,1,1,1,1,1,1,1,1,1,1,1,1,1,1,1,
1,1,1,1,1,1,1,1,1,1,1,1,1,1,1,1,1,1,1,1,1,1,1,1,1,1,1,1,1,1,1,1,1,1,1,1,
1,1,1,1,1,1,1,6),(-0.994228156739691,-0.984615384615383,-0.969230769230768,
-0.953846153846152,-0.938461538461537,-0.923076923076922,-0.907692307692306,
-0.892307692307691,-0.876923076923076,-0.86153846153846,-0.846153846153845,
-0.83076923076923,-0.815384615384614,-0.799999999999999,-0.784615384615384,
-0.769230769230768,-0.753846153846153,-0.738461538461538,-0.723076923076922,
-0.707692307692307,-0.692307692307692,-0.676923076923076,-0.661538461538461,
-0.646153846153846,-0.63076923076923,-0.615384615384615,-0.6,-0.584615384615384,
-0.569230769230769,-0.553846153846154,-0.538461538461538,-0.523076923076923,
-0.507692307692308,-0.492307692307692,-0.476923076923077,-0.461538461538462,
-0.446153846153846,-0.430769230769231,-0.415384615384615,-0.4,-0.384615384615385,
-0.369230769230769,-0.353846153846154,-0.338461538461538,-0.323076923076923,
-0.307692307692308,-0.292307692307692,-0.276923076923077,-0.261538461538462,
-0.246153846153846,-0.230769230769231,-0.215384615384615,-0.2,-0.184615384615385,
-0.169230769230769,-0.153846153846154,-0.138461538461538,-0.123076923076923,
-0.107692307692308,-0.0923076923076923,-0.0769230769230769,-0.0615384615384615,
-0.0461538461538462,-0.0307692307692308,-0.0153846153846154,0.),
 .UNSPECIFIED.)
CURVE()
GEOMETRIC_REPRESENTATION_ITEM()
RATIONAL_B_SPLINE_CURVE((1.,1.,1.,1.,1.,1.,1.,1.,1.,1.,1.,1.,1.,1.,1.,1.,
1.,1.,1.,1.,1.,1.,1.,1.,1.,1.,1.,1.,1.,1.,1.,1.,1.,1.,1.,1.,1.,1.,1.,1.,
1.,1.,1.,1.,1.,1.,1.,1.,1.,1.,1.,1.,1.,1.,1.,1.,1.,1.,1.,1.,1.,1.,1.,1.,
1.,1.,1.,1.,1.,1.))
REPRESENTATION_ITEM('')
);
#311=(
BOUNDED_CURVE()
B_SPLINE_CURVE(5,(#40567,#40568,#40569,#40570,#40571,#40572,#40573,#40574,
#40575,#40576,#40577,#40578,#40579,#40580,#40581,#40582,#40583,#40584,#40585,
#40586,#40587,#40588,#40589,#40590,#40591,#40592,#40593,#40594,#40595,#40596,
#40597,#40598,#40599,#40600,#40601,#40602,#40603,#40604,#40605,#40606,#40607,
#40608,#40609,#40610,#40611,#40612,#40613,#40614,#40615,#40616,#40617,#40618,
#40619,#40620,#40621,#40622,#40623,#40624,#40625,#40626,#40627,#40628,#40629,
#40630,#40631,#40632,#40633,#40634,#40635,#40636),.UNSPECIFIED.,.F.,.F.)
B_SPLINE_CURVE_WITH_KNOTS((6,1,1,1,1,1,1,1,1,1,1,1,1,1,1,1,1,1,1,1,1,1,
1,1,1,1,1,1,1,1,1,1,1,1,1,1,1,1,1,1,1,1,1,1,1,1,1,1,1,1,1,1,1,1,1,1,1,1,
1,1,1,1,1,1,1,6),(-1.,-0.984615384615383,-0.969230769230768,-0.953846153846152,
-0.938461538461537,-0.923076923076922,-0.907692307692306,-0.892307692307691,
-0.876923076923076,-0.86153846153846,-0.846153846153845,-0.83076923076923,
-0.815384615384614,-0.799999999999999,-0.784615384615384,-0.769230769230768,
-0.753846153846153,-0.738461538461538,-0.723076923076922,-0.707692307692307,
-0.692307692307692,-0.676923076923076,-0.661538461538461,-0.646153846153846,
-0.63076923076923,-0.615384615384615,-0.6,-0.584615384615384,-0.569230769230769,
-0.553846153846154,-0.538461538461538,-0.523076923076923,-0.507692307692308,
-0.492307692307692,-0.476923076923077,-0.461538461538462,-0.446153846153846,
-0.430769230769231,-0.415384615384615,-0.4,-0.384615384615385,-0.369230769230769,
-0.353846153846154,-0.338461538461538,-0.323076923076923,-0.307692307692308,
-0.292307692307692,-0.276923076923077,-0.261538461538462,-0.246153846153846,
-0.230769230769231,-0.215384615384615,-0.2,-0.184615384615385,-0.169230769230769,
-0.153846153846154,-0.138461538461538,-0.123076923076923,-0.107692307692308,
-0.0923076923076923,-0.0769230769230769,-0.0615384615384615,-0.0461538461538462,
-0.0307692307692308,-0.0153846153846154,-0.00577184337448448),
 .UNSPECIFIED.)
CURVE()
GEOMETRIC_REPRESENTATION_ITEM()
RATIONAL_B_SPLINE_CURVE((1.,1.,1.,1.,1.,1.,1.,1.,1.,1.,1.,1.,1.,1.,1.,1.,
1.,1.,1.,1.,1.,1.,1.,1.,1.,1.,1.,1.,1.,1.,1.,1.,1.,1.,1.,1.,1.,1.,1.,1.,
1.,1.,1.,1.,1.,1.,1.,1.,1.,1.,1.,1.,1.,1.,1.,1.,1.,1.,1.,1.,1.,1.,1.,1.,
1.,1.,1.,1.,1.,1.))
REPRESENTATION_ITEM('')
);
#312=(
BOUNDED_CURVE()
B_SPLINE_CURVE(5,(#40787,#40788,#40789,#40790,#40791,#40792,#40793,#40794,
#40795,#40796,#40797,#40798,#40799,#40800,#40801,#40802,#40803,#40804,#40805,
#40806,#40807,#40808,#40809,#40810,#40811,#40812,#40813,#40814,#40815,#40816,
#40817,#40818,#40819,#40820,#40821,#40822,#40823,#40824,#40825,#40826,#40827,
#40828,#40829,#40830,#40831,#40832,#40833,#40834,#40835,#40836,#40837,#40838,
#40839,#40840,#40841,#40842,#40843,#40844,#40845,#40846,#40847,#40848,#40849,
#40850,#40851,#40852,#40853,#40854,#40855,#40856),.UNSPECIFIED.,.F.,.F.)
B_SPLINE_CURVE_WITH_KNOTS((6,1,1,1,1,1,1,1,1,1,1,1,1,1,1,1,1,1,1,1,1,1,
1,1,1,1,1,1,1,1,1,1,1,1,1,1,1,1,1,1,1,1,1,1,1,1,1,1,1,1,1,1,1,1,1,1,1,1,
1,1,1,1,1,1,1,6),(-0.99422815673972,-0.984615384615383,-0.969230769230768,
-0.953846153846152,-0.938461538461537,-0.923076923076922,-0.907692307692306,
-0.892307692307691,-0.876923076923076,-0.86153846153846,-0.846153846153845,
-0.83076923076923,-0.815384615384614,-0.799999999999999,-0.784615384615384,
-0.769230769230768,-0.753846153846153,-0.738461538461538,-0.723076923076922,
-0.707692307692307,-0.692307692307692,-0.676923076923076,-0.661538461538461,
-0.646153846153846,-0.63076923076923,-0.615384615384615,-0.6,-0.584615384615384,
-0.569230769230769,-0.553846153846154,-0.538461538461538,-0.523076923076923,
-0.507692307692308,-0.492307692307692,-0.476923076923077,-0.461538461538462,
-0.446153846153846,-0.430769230769231,-0.415384615384615,-0.4,-0.384615384615385,
-0.369230769230769,-0.353846153846154,-0.338461538461538,-0.323076923076923,
-0.307692307692308,-0.292307692307692,-0.276923076923077,-0.261538461538462,
-0.246153846153846,-0.230769230769231,-0.215384615384615,-0.2,-0.184615384615385,
-0.169230769230769,-0.153846153846154,-0.138461538461538,-0.123076923076923,
-0.107692307692308,-0.0923076923076923,-0.0769230769230769,-0.0615384615384615,
-0.0461538461538462,-0.0307692307692308,-0.0153846153846154,0.),
 .UNSPECIFIED.)
CURVE()
GEOMETRIC_REPRESENTATION_ITEM()
RATIONAL_B_SPLINE_CURVE((1.,1.,1.,1.,1.,1.,1.,1.,1.,1.,1.,1.,1.,1.,1.,1.,
1.,1.,1.,1.,1.,1.,1.,1.,1.,1.,1.,1.,1.,1.,1.,1.,1.,1.,1.,1.,1.,1.,1.,1.,
1.,1.,1.,1.,1.,1.,1.,1.,1.,1.,1.,1.,1.,1.,1.,1.,1.,1.,1.,1.,1.,1.,1.,1.,
1.,1.,1.,1.,1.,1.))
REPRESENTATION_ITEM('')
);
#313=(
BOUNDED_CURVE()
B_SPLINE_CURVE(5,(#41009,#41010,#41011,#41012,#41013,#41014,#41015,#41016,
#41017,#41018,#41019,#41020,#41021,#41022,#41023,#41024,#41025,#41026,#41027,
#41028,#41029,#41030,#41031,#41032,#41033,#41034,#41035,#41036,#41037,#41038,
#41039,#41040,#41041,#41042,#41043,#41044,#41045,#41046,#41047,#41048,#41049,
#41050,#41051,#41052,#41053,#41054,#41055,#41056,#41057,#41058,#41059,#41060,
#41061,#41062,#41063,#41064,#41065,#41066,#41067,#41068,#41069,#41070,#41071,
#41072,#41073,#41074,#41075,#41076,#41077,#41078),.UNSPECIFIED.,.F.,.F.)
B_SPLINE_CURVE_WITH_KNOTS((6,1,1,1,1,1,1,1,1,1,1,1,1,1,1,1,1,1,1,1,1,1,
1,1,1,1,1,1,1,1,1,1,1,1,1,1,1,1,1,1,1,1,1,1,1,1,1,1,1,1,1,1,1,1,1,1,1,1,
1,1,1,1,1,1,1,6),(-1.,-0.984615384615383,-0.969230769230768,-0.953846153846152,
-0.938461538461537,-0.923076923076922,-0.907692307692306,-0.892307692307691,
-0.876923076923076,-0.86153846153846,-0.846153846153845,-0.83076923076923,
-0.815384615384614,-0.799999999999999,-0.784615384615384,-0.769230769230768,
-0.753846153846153,-0.738461538461538,-0.723076923076922,-0.707692307692307,
-0.692307692307692,-0.676923076923076,-0.661538461538461,-0.646153846153846,
-0.63076923076923,-0.615384615384615,-0.6,-0.584615384615384,-0.569230769230769,
-0.553846153846154,-0.538461538461538,-0.523076923076923,-0.507692307692308,
-0.492307692307692,-0.476923076923077,-0.461538461538462,-0.446153846153846,
-0.430769230769231,-0.415384615384615,-0.4,-0.384615384615385,-0.369230769230769,
-0.353846153846154,-0.338461538461538,-0.323076923076923,-0.307692307692308,
-0.292307692307692,-0.276923076923077,-0.261538461538462,-0.246153846153846,
-0.230769230769231,-0.215384615384615,-0.2,-0.184615384615385,-0.169230769230769,
-0.153846153846154,-0.138461538461538,-0.123076923076923,-0.107692307692308,
-0.0923076923076923,-0.0769230769230769,-0.0615384615384615,-0.0461538461538462,
-0.0307692307692308,-0.0153846153846154,-0.00577184337448251),
 .UNSPECIFIED.)
CURVE()
GEOMETRIC_REPRESENTATION_ITEM()
RATIONAL_B_SPLINE_CURVE((1.,1.,1.,1.,1.,1.,1.,1.,1.,1.,1.,1.,1.,1.,1.,1.,
1.,1.,1.,1.,1.,1.,1.,1.,1.,1.,1.,1.,1.,1.,1.,1.,1.,1.,1.,1.,1.,1.,1.,1.,
1.,1.,1.,1.,1.,1.,1.,1.,1.,1.,1.,1.,1.,1.,1.,1.,1.,1.,1.,1.,1.,1.,1.,1.,
1.,1.,1.,1.,1.,1.))
REPRESENTATION_ITEM('')
);
#314=(
BOUNDED_CURVE()
B_SPLINE_CURVE(5,(#41229,#41230,#41231,#41232,#41233,#41234,#41235,#41236,
#41237,#41238,#41239,#41240,#41241,#41242,#41243,#41244,#41245,#41246,#41247,
#41248,#41249,#41250,#41251,#41252,#41253,#41254,#41255,#41256,#41257,#41258,
#41259,#41260,#41261,#41262,#41263,#41264,#41265,#41266,#41267,#41268,#41269,
#41270,#41271,#41272,#41273,#41274,#41275,#41276,#41277,#41278,#41279,#41280,
#41281,#41282,#41283,#41284,#41285,#41286,#41287,#41288,#41289,#41290,#41291,
#41292,#41293,#41294,#41295,#41296,#41297,#41298),.UNSPECIFIED.,.F.,.F.)
B_SPLINE_CURVE_WITH_KNOTS((6,1,1,1,1,1,1,1,1,1,1,1,1,1,1,1,1,1,1,1,1,1,
1,1,1,1,1,1,1,1,1,1,1,1,1,1,1,1,1,1,1,1,1,1,1,1,1,1,1,1,1,1,1,1,1,1,1,1,
1,1,1,1,1,1,1,6),(-0.994228156739703,-0.984615384615383,-0.969230769230768,
-0.953846153846152,-0.938461538461537,-0.923076923076922,-0.907692307692306,
-0.892307692307691,-0.876923076923076,-0.86153846153846,-0.846153846153845,
-0.83076923076923,-0.815384615384614,-0.799999999999999,-0.784615384615384,
-0.769230769230768,-0.753846153846153,-0.738461538461538,-0.723076923076922,
-0.707692307692307,-0.692307692307692,-0.676923076923076,-0.661538461538461,
-0.646153846153846,-0.63076923076923,-0.615384615384615,-0.6,-0.584615384615384,
-0.569230769230769,-0.553846153846154,-0.538461538461538,-0.523076923076923,
-0.507692307692308,-0.492307692307692,-0.476923076923077,-0.461538461538462,
-0.446153846153846,-0.430769230769231,-0.415384615384615,-0.4,-0.384615384615385,
-0.369230769230769,-0.353846153846154,-0.338461538461538,-0.323076923076923,
-0.307692307692308,-0.292307692307692,-0.276923076923077,-0.261538461538462,
-0.246153846153846,-0.230769230769231,-0.215384615384615,-0.2,-0.184615384615385,
-0.169230769230769,-0.153846153846154,-0.138461538461538,-0.123076923076923,
-0.107692307692308,-0.0923076923076923,-0.0769230769230769,-0.0615384615384615,
-0.0461538461538462,-0.0307692307692308,-0.0153846153846154,0.),
 .UNSPECIFIED.)
CURVE()
GEOMETRIC_REPRESENTATION_ITEM()
RATIONAL_B_SPLINE_CURVE((1.,1.,1.,1.,1.,1.,1.,1.,1.,1.,1.,1.,1.,1.,1.,1.,
1.,1.,1.,1.,1.,1.,1.,1.,1.,1.,1.,1.,1.,1.,1.,1.,1.,1.,1.,1.,1.,1.,1.,1.,
1.,1.,1.,1.,1.,1.,1.,1.,1.,1.,1.,1.,1.,1.,1.,1.,1.,1.,1.,1.,1.,1.,1.,1.,
1.,1.,1.,1.,1.,1.))
REPRESENTATION_ITEM('')
);
#315=(
BOUNDED_CURVE()
B_SPLINE_CURVE(5,(#41451,#41452,#41453,#41454,#41455,#41456,#41457,#41458,
#41459,#41460,#41461,#41462,#41463,#41464,#41465,#41466,#41467,#41468,#41469,
#41470,#41471,#41472,#41473,#41474,#41475,#41476,#41477,#41478,#41479,#41480,
#41481,#41482,#41483,#41484,#41485,#41486,#41487,#41488,#41489,#41490,#41491,
#41492,#41493,#41494,#41495,#41496,#41497,#41498,#41499,#41500,#41501,#41502,
#41503,#41504,#41505,#41506,#41507,#41508,#41509,#41510,#41511,#41512,#41513,
#41514,#41515,#41516,#41517,#41518,#41519,#41520),.UNSPECIFIED.,.F.,.F.)
B_SPLINE_CURVE_WITH_KNOTS((6,1,1,1,1,1,1,1,1,1,1,1,1,1,1,1,1,1,1,1,1,1,
1,1,1,1,1,1,1,1,1,1,1,1,1,1,1,1,1,1,1,1,1,1,1,1,1,1,1,1,1,1,1,1,1,1,1,1,
1,1,1,1,1,1,1,6),(-1.,-0.984615384615383,-0.969230769230768,-0.953846153846152,
-0.938461538461537,-0.923076923076922,-0.907692307692306,-0.892307692307691,
-0.876923076923076,-0.86153846153846,-0.846153846153845,-0.83076923076923,
-0.815384615384614,-0.799999999999999,-0.784615384615384,-0.769230769230768,
-0.753846153846153,-0.738461538461538,-0.723076923076922,-0.707692307692307,
-0.692307692307692,-0.676923076923076,-0.661538461538461,-0.646153846153846,
-0.63076923076923,-0.615384615384615,-0.6,-0.584615384615384,-0.569230769230769,
-0.553846153846154,-0.538461538461538,-0.523076923076923,-0.507692307692308,
-0.492307692307692,-0.476923076923077,-0.461538461538462,-0.446153846153846,
-0.430769230769231,-0.415384615384615,-0.4,-0.384615384615385,-0.369230769230769,
-0.353846153846154,-0.338461538461538,-0.323076923076923,-0.307692307692308,
-0.292307692307692,-0.276923076923077,-0.261538461538462,-0.246153846153846,
-0.230769230769231,-0.215384615384615,-0.2,-0.184615384615385,-0.169230769230769,
-0.153846153846154,-0.138461538461538,-0.123076923076923,-0.107692307692308,
-0.0923076923076923,-0.0769230769230769,-0.0615384615384615,-0.0461538461538462,
-0.0307692307692308,-0.0153846153846154,-0.00577184337449602),
 .UNSPECIFIED.)
CURVE()
GEOMETRIC_REPRESENTATION_ITEM()
RATIONAL_B_SPLINE_CURVE((1.,1.,1.,1.,1.,1.,1.,1.,1.,1.,1.,1.,1.,1.,1.,1.,
1.,1.,1.,1.,1.,1.,1.,1.,1.,1.,1.,1.,1.,1.,1.,1.,1.,1.,1.,1.,1.,1.,1.,1.,
1.,1.,1.,1.,1.,1.,1.,1.,1.,1.,1.,1.,1.,1.,1.,1.,1.,1.,1.,1.,1.,1.,1.,1.,
1.,1.,1.,1.,1.,1.))
REPRESENTATION_ITEM('')
);
#316=(
BOUNDED_CURVE()
B_SPLINE_CURVE(5,(#41671,#41672,#41673,#41674,#41675,#41676,#41677,#41678,
#41679,#41680,#41681,#41682,#41683,#41684,#41685,#41686,#41687,#41688,#41689,
#41690,#41691,#41692,#41693,#41694,#41695,#41696,#41697,#41698,#41699,#41700,
#41701,#41702,#41703,#41704,#41705,#41706,#41707,#41708,#41709,#41710,#41711,
#41712,#41713,#41714,#41715,#41716,#41717,#41718,#41719,#41720,#41721,#41722,
#41723,#41724,#41725,#41726,#41727,#41728,#41729,#41730,#41731,#41732,#41733,
#41734,#41735,#41736,#41737,#41738,#41739,#41740),.UNSPECIFIED.,.F.,.F.)
B_SPLINE_CURVE_WITH_KNOTS((6,1,1,1,1,1,1,1,1,1,1,1,1,1,1,1,1,1,1,1,1,1,
1,1,1,1,1,1,1,1,1,1,1,1,1,1,1,1,1,1,1,1,1,1,1,1,1,1,1,1,1,1,1,1,1,1,1,1,
1,1,1,1,1,1,1,6),(-0.994228156739695,-0.984615384615383,-0.969230769230768,
-0.953846153846152,-0.938461538461537,-0.923076923076922,-0.907692307692306,
-0.892307692307691,-0.876923076923076,-0.86153846153846,-0.846153846153845,
-0.83076923076923,-0.815384615384614,-0.799999999999999,-0.784615384615384,
-0.769230769230768,-0.753846153846153,-0.738461538461538,-0.723076923076922,
-0.707692307692307,-0.692307692307692,-0.676923076923076,-0.661538461538461,
-0.646153846153846,-0.63076923076923,-0.615384615384615,-0.6,-0.584615384615384,
-0.569230769230769,-0.553846153846154,-0.538461538461538,-0.523076923076923,
-0.507692307692308,-0.492307692307692,-0.476923076923077,-0.461538461538462,
-0.446153846153846,-0.430769230769231,-0.415384615384615,-0.4,-0.384615384615385,
-0.369230769230769,-0.353846153846154,-0.338461538461538,-0.323076923076923,
-0.307692307692308,-0.292307692307692,-0.276923076923077,-0.261538461538462,
-0.246153846153846,-0.230769230769231,-0.215384615384615,-0.2,-0.184615384615385,
-0.169230769230769,-0.153846153846154,-0.138461538461538,-0.123076923076923,
-0.107692307692308,-0.0923076923076923,-0.0769230769230769,-0.0615384615384615,
-0.0461538461538462,-0.0307692307692308,-0.0153846153846154,0.),
 .UNSPECIFIED.)
CURVE()
GEOMETRIC_REPRESENTATION_ITEM()
RATIONAL_B_SPLINE_CURVE((1.,1.,1.,1.,1.,1.,1.,1.,1.,1.,1.,1.,1.,1.,1.,1.,
1.,1.,1.,1.,1.,1.,1.,1.,1.,1.,1.,1.,1.,1.,1.,1.,1.,1.,1.,1.,1.,1.,1.,1.,
1.,1.,1.,1.,1.,1.,1.,1.,1.,1.,1.,1.,1.,1.,1.,1.,1.,1.,1.,1.,1.,1.,1.,1.,
1.,1.,1.,1.,1.,1.))
REPRESENTATION_ITEM('')
);
#317=(
BOUNDED_CURVE()
B_SPLINE_CURVE(5,(#41893,#41894,#41895,#41896,#41897,#41898,#41899,#41900,
#41901,#41902,#41903,#41904,#41905,#41906,#41907,#41908,#41909,#41910,#41911,
#41912,#41913,#41914,#41915,#41916,#41917,#41918,#41919,#41920,#41921,#41922,
#41923,#41924,#41925,#41926,#41927,#41928,#41929,#41930,#41931,#41932,#41933,
#41934,#41935,#41936,#41937,#41938,#41939,#41940,#41941,#41942,#41943,#41944,
#41945,#41946,#41947,#41948,#41949,#41950,#41951,#41952,#41953,#41954,#41955,
#41956,#41957,#41958,#41959,#41960,#41961,#41962),.UNSPECIFIED.,.F.,.F.)
B_SPLINE_CURVE_WITH_KNOTS((6,1,1,1,1,1,1,1,1,1,1,1,1,1,1,1,1,1,1,1,1,1,
1,1,1,1,1,1,1,1,1,1,1,1,1,1,1,1,1,1,1,1,1,1,1,1,1,1,1,1,1,1,1,1,1,1,1,1,
1,1,1,1,1,1,1,6),(-1.,-0.984615384615383,-0.969230769230768,-0.953846153846152,
-0.938461538461537,-0.923076923076922,-0.907692307692306,-0.892307692307691,
-0.876923076923076,-0.86153846153846,-0.846153846153845,-0.83076923076923,
-0.815384615384614,-0.799999999999999,-0.784615384615384,-0.769230769230768,
-0.753846153846153,-0.738461538461538,-0.723076923076922,-0.707692307692307,
-0.692307692307692,-0.676923076923076,-0.661538461538461,-0.646153846153846,
-0.63076923076923,-0.615384615384615,-0.6,-0.584615384615384,-0.569230769230769,
-0.553846153846154,-0.538461538461538,-0.523076923076923,-0.507692307692308,
-0.492307692307692,-0.476923076923077,-0.461538461538462,-0.446153846153846,
-0.430769230769231,-0.415384615384615,-0.4,-0.384615384615385,-0.369230769230769,
-0.353846153846154,-0.338461538461538,-0.323076923076923,-0.307692307692308,
-0.292307692307692,-0.276923076923077,-0.261538461538462,-0.246153846153846,
-0.230769230769231,-0.215384615384615,-0.2,-0.184615384615385,-0.169230769230769,
-0.153846153846154,-0.138461538461538,-0.123076923076923,-0.107692307692308,
-0.0923076923076923,-0.0769230769230769,-0.0615384615384615,-0.0461538461538462,
-0.0307692307692308,-0.0153846153846154,-0.00577184337450911),
 .UNSPECIFIED.)
CURVE()
GEOMETRIC_REPRESENTATION_ITEM()
RATIONAL_B_SPLINE_CURVE((1.,1.,1.,1.,1.,1.,1.,1.,1.,1.,1.,1.,1.,1.,1.,1.,
1.,1.,1.,1.,1.,1.,1.,1.,1.,1.,1.,1.,1.,1.,1.,1.,1.,1.,1.,1.,1.,1.,1.,1.,
1.,1.,1.,1.,1.,1.,1.,1.,1.,1.,1.,1.,1.,1.,1.,1.,1.,1.,1.,1.,1.,1.,1.,1.,
1.,1.,1.,1.,1.,1.))
REPRESENTATION_ITEM('')
);
#318=(
BOUNDED_CURVE()
B_SPLINE_CURVE(5,(#42113,#42114,#42115,#42116,#42117,#42118,#42119,#42120,
#42121,#42122,#42123,#42124,#42125,#42126,#42127,#42128,#42129,#42130,#42131,
#42132,#42133,#42134,#42135,#42136,#42137,#42138,#42139,#42140,#42141,#42142,
#42143,#42144,#42145,#42146,#42147,#42148,#42149,#42150,#42151,#42152,#42153,
#42154,#42155,#42156,#42157,#42158,#42159,#42160,#42161,#42162,#42163,#42164,
#42165,#42166,#42167,#42168,#42169,#42170,#42171,#42172,#42173,#42174,#42175,
#42176,#42177,#42178,#42179,#42180,#42181,#42182),.UNSPECIFIED.,.F.,.F.)
B_SPLINE_CURVE_WITH_KNOTS((6,1,1,1,1,1,1,1,1,1,1,1,1,1,1,1,1,1,1,1,1,1,
1,1,1,1,1,1,1,1,1,1,1,1,1,1,1,1,1,1,1,1,1,1,1,1,1,1,1,1,1,1,1,1,1,1,1,1,
1,1,1,1,1,1,1,6),(-0.994228156739712,-0.984615384615383,-0.969230769230768,
-0.953846153846152,-0.938461538461537,-0.923076923076922,-0.907692307692306,
-0.892307692307691,-0.876923076923076,-0.86153846153846,-0.846153846153845,
-0.83076923076923,-0.815384615384614,-0.799999999999999,-0.784615384615384,
-0.769230769230768,-0.753846153846153,-0.738461538461538,-0.723076923076922,
-0.707692307692307,-0.692307692307692,-0.676923076923076,-0.661538461538461,
-0.646153846153846,-0.63076923076923,-0.615384615384615,-0.6,-0.584615384615384,
-0.569230769230769,-0.553846153846154,-0.538461538461538,-0.523076923076923,
-0.507692307692308,-0.492307692307692,-0.476923076923077,-0.461538461538462,
-0.446153846153846,-0.430769230769231,-0.415384615384615,-0.4,-0.384615384615385,
-0.369230769230769,-0.353846153846154,-0.338461538461538,-0.323076923076923,
-0.307692307692308,-0.292307692307692,-0.276923076923077,-0.261538461538462,
-0.246153846153846,-0.230769230769231,-0.215384615384615,-0.2,-0.184615384615385,
-0.169230769230769,-0.153846153846154,-0.138461538461538,-0.123076923076923,
-0.107692307692308,-0.0923076923076923,-0.0769230769230769,-0.0615384615384615,
-0.0461538461538462,-0.0307692307692308,-0.0153846153846154,0.),
 .UNSPECIFIED.)
CURVE()
GEOMETRIC_REPRESENTATION_ITEM()
RATIONAL_B_SPLINE_CURVE((1.,1.,1.,1.,1.,1.,1.,1.,1.,1.,1.,1.,1.,1.,1.,1.,
1.,1.,1.,1.,1.,1.,1.,1.,1.,1.,1.,1.,1.,1.,1.,1.,1.,1.,1.,1.,1.,1.,1.,1.,
1.,1.,1.,1.,1.,1.,1.,1.,1.,1.,1.,1.,1.,1.,1.,1.,1.,1.,1.,1.,1.,1.,1.,1.,
1.,1.,1.,1.,1.,1.))
REPRESENTATION_ITEM('')
);
#319=(
BOUNDED_CURVE()
B_SPLINE_CURVE(5,(#42335,#42336,#42337,#42338,#42339,#42340,#42341,#42342,
#42343,#42344,#42345,#42346,#42347,#42348,#42349,#42350,#42351,#42352,#42353,
#42354,#42355,#42356,#42357,#42358,#42359,#42360,#42361,#42362,#42363,#42364,
#42365,#42366,#42367,#42368,#42369,#42370,#42371,#42372,#42373,#42374,#42375,
#42376,#42377,#42378,#42379,#42380,#42381,#42382,#42383,#42384,#42385,#42386,
#42387,#42388,#42389,#42390,#42391,#42392,#42393,#42394,#42395,#42396,#42397,
#42398,#42399,#42400,#42401,#42402,#42403,#42404),.UNSPECIFIED.,.F.,.F.)
B_SPLINE_CURVE_WITH_KNOTS((6,1,1,1,1,1,1,1,1,1,1,1,1,1,1,1,1,1,1,1,1,1,
1,1,1,1,1,1,1,1,1,1,1,1,1,1,1,1,1,1,1,1,1,1,1,1,1,1,1,1,1,1,1,1,1,1,1,1,
1,1,1,1,1,1,1,6),(-1.,-0.984615384615383,-0.969230769230768,-0.953846153846152,
-0.938461538461537,-0.923076923076922,-0.907692307692306,-0.892307692307691,
-0.876923076923076,-0.86153846153846,-0.846153846153845,-0.83076923076923,
-0.815384615384614,-0.799999999999999,-0.784615384615384,-0.769230769230768,
-0.753846153846153,-0.738461538461538,-0.723076923076922,-0.707692307692307,
-0.692307692307692,-0.676923076923076,-0.661538461538461,-0.646153846153846,
-0.63076923076923,-0.615384615384615,-0.6,-0.584615384615384,-0.569230769230769,
-0.553846153846154,-0.538461538461538,-0.523076923076923,-0.507692307692308,
-0.492307692307692,-0.476923076923077,-0.461538461538462,-0.446153846153846,
-0.430769230769231,-0.415384615384615,-0.4,-0.384615384615385,-0.369230769230769,
-0.353846153846154,-0.338461538461538,-0.323076923076923,-0.307692307692308,
-0.292307692307692,-0.276923076923077,-0.261538461538462,-0.246153846153846,
-0.230769230769231,-0.215384615384615,-0.2,-0.184615384615385,-0.169230769230769,
-0.153846153846154,-0.138461538461538,-0.123076923076923,-0.107692307692308,
-0.0923076923076923,-0.0769230769230769,-0.0615384615384615,-0.0461538461538462,
-0.0307692307692308,-0.0153846153846154,-0.00577184337451206),
 .UNSPECIFIED.)
CURVE()
GEOMETRIC_REPRESENTATION_ITEM()
RATIONAL_B_SPLINE_CURVE((1.,1.,1.,1.,1.,1.,1.,1.,1.,1.,1.,1.,1.,1.,1.,1.,
1.,1.,1.,1.,1.,1.,1.,1.,1.,1.,1.,1.,1.,1.,1.,1.,1.,1.,1.,1.,1.,1.,1.,1.,
1.,1.,1.,1.,1.,1.,1.,1.,1.,1.,1.,1.,1.,1.,1.,1.,1.,1.,1.,1.,1.,1.,1.,1.,
1.,1.,1.,1.,1.,1.))
REPRESENTATION_ITEM('')
);
#320=(
BOUNDED_CURVE()
B_SPLINE_CURVE(5,(#42555,#42556,#42557,#42558,#42559,#42560,#42561,#42562,
#42563,#42564,#42565,#42566,#42567,#42568,#42569,#42570,#42571,#42572,#42573,
#42574,#42575,#42576,#42577,#42578,#42579,#42580,#42581,#42582,#42583,#42584,
#42585,#42586,#42587,#42588,#42589,#42590,#42591,#42592,#42593,#42594,#42595,
#42596,#42597,#42598,#42599,#42600,#42601,#42602,#42603,#42604,#42605,#42606,
#42607,#42608,#42609,#42610,#42611,#42612,#42613,#42614,#42615,#42616,#42617,
#42618,#42619,#42620,#42621,#42622,#42623,#42624),.UNSPECIFIED.,.F.,.F.)
B_SPLINE_CURVE_WITH_KNOTS((6,1,1,1,1,1,1,1,1,1,1,1,1,1,1,1,1,1,1,1,1,1,
1,1,1,1,1,1,1,1,1,1,1,1,1,1,1,1,1,1,1,1,1,1,1,1,1,1,1,1,1,1,1,1,1,1,1,1,
1,1,1,1,1,1,1,6),(-0.994228156739717,-0.984615384615383,-0.969230769230768,
-0.953846153846152,-0.938461538461537,-0.923076923076922,-0.907692307692306,
-0.892307692307691,-0.876923076923076,-0.86153846153846,-0.846153846153845,
-0.83076923076923,-0.815384615384614,-0.799999999999999,-0.784615384615384,
-0.769230769230768,-0.753846153846153,-0.738461538461538,-0.723076923076922,
-0.707692307692307,-0.692307692307692,-0.676923076923076,-0.661538461538461,
-0.646153846153846,-0.63076923076923,-0.615384615384615,-0.6,-0.584615384615384,
-0.569230769230769,-0.553846153846154,-0.538461538461538,-0.523076923076923,
-0.507692307692308,-0.492307692307692,-0.476923076923077,-0.461538461538462,
-0.446153846153846,-0.430769230769231,-0.415384615384615,-0.4,-0.384615384615385,
-0.369230769230769,-0.353846153846154,-0.338461538461538,-0.323076923076923,
-0.307692307692308,-0.292307692307692,-0.276923076923077,-0.261538461538462,
-0.246153846153846,-0.230769230769231,-0.215384615384615,-0.2,-0.184615384615385,
-0.169230769230769,-0.153846153846154,-0.138461538461538,-0.123076923076923,
-0.107692307692308,-0.0923076923076923,-0.0769230769230769,-0.0615384615384615,
-0.0461538461538462,-0.0307692307692308,-0.0153846153846154,0.),
 .UNSPECIFIED.)
CURVE()
GEOMETRIC_REPRESENTATION_ITEM()
RATIONAL_B_SPLINE_CURVE((1.,1.,1.,1.,1.,1.,1.,1.,1.,1.,1.,1.,1.,1.,1.,1.,
1.,1.,1.,1.,1.,1.,1.,1.,1.,1.,1.,1.,1.,1.,1.,1.,1.,1.,1.,1.,1.,1.,1.,1.,
1.,1.,1.,1.,1.,1.,1.,1.,1.,1.,1.,1.,1.,1.,1.,1.,1.,1.,1.,1.,1.,1.,1.,1.,
1.,1.,1.,1.,1.,1.))
REPRESENTATION_ITEM('')
);
#321=(
BOUNDED_CURVE()
B_SPLINE_CURVE(5,(#42777,#42778,#42779,#42780,#42781,#42782,#42783,#42784,
#42785,#42786,#42787,#42788,#42789,#42790,#42791,#42792,#42793,#42794,#42795,
#42796,#42797,#42798,#42799,#42800,#42801,#42802,#42803,#42804,#42805,#42806,
#42807,#42808,#42809,#42810,#42811,#42812,#42813,#42814,#42815,#42816,#42817,
#42818,#42819,#42820,#42821,#42822,#42823,#42824,#42825,#42826,#42827,#42828,
#42829,#42830,#42831,#42832,#42833,#42834,#42835,#42836,#42837,#42838,#42839,
#42840,#42841,#42842,#42843,#42844,#42845,#42846),.UNSPECIFIED.,.F.,.F.)
B_SPLINE_CURVE_WITH_KNOTS((6,1,1,1,1,1,1,1,1,1,1,1,1,1,1,1,1,1,1,1,1,1,
1,1,1,1,1,1,1,1,1,1,1,1,1,1,1,1,1,1,1,1,1,1,1,1,1,1,1,1,1,1,1,1,1,1,1,1,
1,1,1,1,1,1,1,6),(-1.,-0.984615384615383,-0.969230769230768,-0.953846153846152,
-0.938461538461537,-0.923076923076922,-0.907692307692306,-0.892307692307691,
-0.876923076923076,-0.86153846153846,-0.846153846153845,-0.83076923076923,
-0.815384615384614,-0.799999999999999,-0.784615384615384,-0.769230769230768,
-0.753846153846153,-0.738461538461538,-0.723076923076922,-0.707692307692307,
-0.692307692307692,-0.676923076923076,-0.661538461538461,-0.646153846153846,
-0.63076923076923,-0.615384615384615,-0.6,-0.584615384615384,-0.569230769230769,
-0.553846153846154,-0.538461538461538,-0.523076923076923,-0.507692307692308,
-0.492307692307692,-0.476923076923077,-0.461538461538462,-0.446153846153846,
-0.430769230769231,-0.415384615384615,-0.4,-0.384615384615385,-0.369230769230769,
-0.353846153846154,-0.338461538461538,-0.323076923076923,-0.307692307692308,
-0.292307692307692,-0.276923076923077,-0.261538461538462,-0.246153846153846,
-0.230769230769231,-0.215384615384615,-0.2,-0.184615384615385,-0.169230769230769,
-0.153846153846154,-0.138461538461538,-0.123076923076923,-0.107692307692308,
-0.0923076923076923,-0.0769230769230769,-0.0615384615384615,-0.0461538461538462,
-0.0307692307692308,-0.0153846153846154,-0.00577184337448646),
 .UNSPECIFIED.)
CURVE()
GEOMETRIC_REPRESENTATION_ITEM()
RATIONAL_B_SPLINE_CURVE((1.,1.,1.,1.,1.,1.,1.,1.,1.,1.,1.,1.,1.,1.,1.,1.,
1.,1.,1.,1.,1.,1.,1.,1.,1.,1.,1.,1.,1.,1.,1.,1.,1.,1.,1.,1.,1.,1.,1.,1.,
1.,1.,1.,1.,1.,1.,1.,1.,1.,1.,1.,1.,1.,1.,1.,1.,1.,1.,1.,1.,1.,1.,1.,1.,
1.,1.,1.,1.,1.,1.))
REPRESENTATION_ITEM('')
);
#322=(
BOUNDED_CURVE()
B_SPLINE_CURVE(5,(#42997,#42998,#42999,#43000,#43001,#43002,#43003,#43004,
#43005,#43006,#43007,#43008,#43009,#43010,#43011,#43012,#43013,#43014,#43015,
#43016,#43017,#43018,#43019,#43020,#43021,#43022,#43023,#43024,#43025,#43026,
#43027,#43028,#43029,#43030,#43031,#43032,#43033,#43034,#43035,#43036,#43037,
#43038,#43039,#43040,#43041,#43042,#43043,#43044,#43045,#43046,#43047,#43048,
#43049,#43050,#43051,#43052,#43053,#43054,#43055,#43056,#43057,#43058,#43059,
#43060,#43061,#43062,#43063,#43064,#43065,#43066),.UNSPECIFIED.,.F.,.F.)
B_SPLINE_CURVE_WITH_KNOTS((6,1,1,1,1,1,1,1,1,1,1,1,1,1,1,1,1,1,1,1,1,1,
1,1,1,1,1,1,1,1,1,1,1,1,1,1,1,1,1,1,1,1,1,1,1,1,1,1,1,1,1,1,1,1,1,1,1,1,
1,1,1,1,1,1,1,6),(-0.994228156739708,-0.984615384615383,-0.969230769230768,
-0.953846153846152,-0.938461538461537,-0.923076923076922,-0.907692307692306,
-0.892307692307691,-0.876923076923076,-0.86153846153846,-0.846153846153845,
-0.83076923076923,-0.815384615384614,-0.799999999999999,-0.784615384615384,
-0.769230769230768,-0.753846153846153,-0.738461538461538,-0.723076923076922,
-0.707692307692307,-0.692307692307692,-0.676923076923076,-0.661538461538461,
-0.646153846153846,-0.63076923076923,-0.615384615384615,-0.6,-0.584615384615384,
-0.569230769230769,-0.553846153846154,-0.538461538461538,-0.523076923076923,
-0.507692307692308,-0.492307692307692,-0.476923076923077,-0.461538461538462,
-0.446153846153846,-0.430769230769231,-0.415384615384615,-0.4,-0.384615384615385,
-0.369230769230769,-0.353846153846154,-0.338461538461538,-0.323076923076923,
-0.307692307692308,-0.292307692307692,-0.276923076923077,-0.261538461538462,
-0.246153846153846,-0.230769230769231,-0.215384615384615,-0.2,-0.184615384615385,
-0.169230769230769,-0.153846153846154,-0.138461538461538,-0.123076923076923,
-0.107692307692308,-0.0923076923076923,-0.0769230769230769,-0.0615384615384615,
-0.0461538461538462,-0.0307692307692308,-0.0153846153846154,0.),
 .UNSPECIFIED.)
CURVE()
GEOMETRIC_REPRESENTATION_ITEM()
RATIONAL_B_SPLINE_CURVE((1.,1.,1.,1.,1.,1.,1.,1.,1.,1.,1.,1.,1.,1.,1.,1.,
1.,1.,1.,1.,1.,1.,1.,1.,1.,1.,1.,1.,1.,1.,1.,1.,1.,1.,1.,1.,1.,1.,1.,1.,
1.,1.,1.,1.,1.,1.,1.,1.,1.,1.,1.,1.,1.,1.,1.,1.,1.,1.,1.,1.,1.,1.,1.,1.,
1.,1.,1.,1.,1.,1.))
REPRESENTATION_ITEM('')
);
#323=(
BOUNDED_CURVE()
B_SPLINE_CURVE(5,(#43219,#43220,#43221,#43222,#43223,#43224,#43225,#43226,
#43227,#43228,#43229,#43230,#43231,#43232,#43233,#43234,#43235,#43236,#43237,
#43238,#43239,#43240,#43241,#43242,#43243,#43244,#43245,#43246,#43247,#43248,
#43249,#43250,#43251,#43252,#43253,#43254,#43255,#43256,#43257,#43258,#43259,
#43260,#43261,#43262,#43263,#43264,#43265,#43266,#43267,#43268,#43269,#43270,
#43271,#43272,#43273,#43274,#43275,#43276,#43277,#43278,#43279,#43280,#43281,
#43282,#43283,#43284,#43285,#43286,#43287,#43288),.UNSPECIFIED.,.F.,.F.)
B_SPLINE_CURVE_WITH_KNOTS((6,1,1,1,1,1,1,1,1,1,1,1,1,1,1,1,1,1,1,1,1,1,
1,1,1,1,1,1,1,1,1,1,1,1,1,1,1,1,1,1,1,1,1,1,1,1,1,1,1,1,1,1,1,1,1,1,1,1,
1,1,1,1,1,1,1,6),(-1.,-0.984615384615383,-0.969230769230768,-0.953846153846152,
-0.938461538461537,-0.923076923076922,-0.907692307692306,-0.892307692307691,
-0.876923076923076,-0.86153846153846,-0.846153846153845,-0.83076923076923,
-0.815384615384614,-0.799999999999999,-0.784615384615384,-0.769230769230768,
-0.753846153846153,-0.738461538461538,-0.723076923076922,-0.707692307692307,
-0.692307692307692,-0.676923076923076,-0.661538461538461,-0.646153846153846,
-0.63076923076923,-0.615384615384615,-0.6,-0.584615384615384,-0.569230769230769,
-0.553846153846154,-0.538461538461538,-0.523076923076923,-0.507692307692308,
-0.492307692307692,-0.476923076923077,-0.461538461538462,-0.446153846153846,
-0.430769230769231,-0.415384615384615,-0.4,-0.384615384615385,-0.369230769230769,
-0.353846153846154,-0.338461538461538,-0.323076923076923,-0.307692307692308,
-0.292307692307692,-0.276923076923077,-0.261538461538462,-0.246153846153846,
-0.230769230769231,-0.215384615384615,-0.2,-0.184615384615385,-0.169230769230769,
-0.153846153846154,-0.138461538461538,-0.123076923076923,-0.107692307692308,
-0.0923076923076923,-0.0769230769230769,-0.0615384615384615,-0.0461538461538462,
-0.0307692307692308,-0.0153846153846154,-0.00577184337451626),
 .UNSPECIFIED.)
CURVE()
GEOMETRIC_REPRESENTATION_ITEM()
RATIONAL_B_SPLINE_CURVE((1.,1.,1.,1.,1.,1.,1.,1.,1.,1.,1.,1.,1.,1.,1.,1.,
1.,1.,1.,1.,1.,1.,1.,1.,1.,1.,1.,1.,1.,1.,1.,1.,1.,1.,1.,1.,1.,1.,1.,1.,
1.,1.,1.,1.,1.,1.,1.,1.,1.,1.,1.,1.,1.,1.,1.,1.,1.,1.,1.,1.,1.,1.,1.,1.,
1.,1.,1.,1.,1.,1.))
REPRESENTATION_ITEM('')
);
#324=(
BOUNDED_CURVE()
B_SPLINE_CURVE(5,(#43439,#43440,#43441,#43442,#43443,#43444,#43445,#43446,
#43447,#43448,#43449,#43450,#43451,#43452,#43453,#43454,#43455,#43456,#43457,
#43458,#43459,#43460,#43461,#43462,#43463,#43464,#43465,#43466,#43467,#43468,
#43469,#43470,#43471,#43472,#43473,#43474,#43475,#43476,#43477,#43478,#43479,
#43480,#43481,#43482,#43483,#43484,#43485,#43486,#43487,#43488,#43489,#43490,
#43491,#43492,#43493,#43494,#43495,#43496,#43497,#43498,#43499,#43500,#43501,
#43502,#43503,#43504,#43505,#43506,#43507,#43508),.UNSPECIFIED.,.F.,.F.)
B_SPLINE_CURVE_WITH_KNOTS((6,1,1,1,1,1,1,1,1,1,1,1,1,1,1,1,1,1,1,1,1,1,
1,1,1,1,1,1,1,1,1,1,1,1,1,1,1,1,1,1,1,1,1,1,1,1,1,1,1,1,1,1,1,1,1,1,1,1,
1,1,1,1,1,1,1,6),(-0.994228156739708,-0.984615384615383,-0.969230769230768,
-0.953846153846152,-0.938461538461537,-0.923076923076922,-0.907692307692306,
-0.892307692307691,-0.876923076923076,-0.86153846153846,-0.846153846153845,
-0.83076923076923,-0.815384615384614,-0.799999999999999,-0.784615384615384,
-0.769230769230768,-0.753846153846153,-0.738461538461538,-0.723076923076922,
-0.707692307692307,-0.692307692307692,-0.676923076923076,-0.661538461538461,
-0.646153846153846,-0.63076923076923,-0.615384615384615,-0.6,-0.584615384615384,
-0.569230769230769,-0.553846153846154,-0.538461538461538,-0.523076923076923,
-0.507692307692308,-0.492307692307692,-0.476923076923077,-0.461538461538462,
-0.446153846153846,-0.430769230769231,-0.415384615384615,-0.4,-0.384615384615385,
-0.369230769230769,-0.353846153846154,-0.338461538461538,-0.323076923076923,
-0.307692307692308,-0.292307692307692,-0.276923076923077,-0.261538461538462,
-0.246153846153846,-0.230769230769231,-0.215384615384615,-0.2,-0.184615384615385,
-0.169230769230769,-0.153846153846154,-0.138461538461538,-0.123076923076923,
-0.107692307692308,-0.0923076923076923,-0.0769230769230769,-0.0615384615384615,
-0.0461538461538462,-0.0307692307692308,-0.0153846153846154,0.),
 .UNSPECIFIED.)
CURVE()
GEOMETRIC_REPRESENTATION_ITEM()
RATIONAL_B_SPLINE_CURVE((1.,1.,1.,1.,1.,1.,1.,1.,1.,1.,1.,1.,1.,1.,1.,1.,
1.,1.,1.,1.,1.,1.,1.,1.,1.,1.,1.,1.,1.,1.,1.,1.,1.,1.,1.,1.,1.,1.,1.,1.,
1.,1.,1.,1.,1.,1.,1.,1.,1.,1.,1.,1.,1.,1.,1.,1.,1.,1.,1.,1.,1.,1.,1.,1.,
1.,1.,1.,1.,1.,1.))
REPRESENTATION_ITEM('')
);
#325=(
BOUNDED_CURVE()
B_SPLINE_CURVE(5,(#43661,#43662,#43663,#43664,#43665,#43666,#43667,#43668,
#43669,#43670,#43671,#43672,#43673,#43674,#43675,#43676,#43677,#43678,#43679,
#43680,#43681,#43682,#43683,#43684,#43685,#43686,#43687,#43688,#43689,#43690,
#43691,#43692,#43693,#43694,#43695,#43696,#43697,#43698,#43699,#43700,#43701,
#43702,#43703,#43704,#43705,#43706,#43707,#43708,#43709,#43710,#43711,#43712,
#43713,#43714,#43715,#43716,#43717,#43718,#43719,#43720,#43721,#43722,#43723,
#43724,#43725,#43726,#43727,#43728,#43729,#43730),.UNSPECIFIED.,.F.,.F.)
B_SPLINE_CURVE_WITH_KNOTS((6,1,1,1,1,1,1,1,1,1,1,1,1,1,1,1,1,1,1,1,1,1,
1,1,1,1,1,1,1,1,1,1,1,1,1,1,1,1,1,1,1,1,1,1,1,1,1,1,1,1,1,1,1,1,1,1,1,1,
1,1,1,1,1,1,1,6),(-1.,-0.984615384615383,-0.969230769230768,-0.953846153846152,
-0.938461538461537,-0.923076923076922,-0.907692307692306,-0.892307692307691,
-0.876923076923076,-0.86153846153846,-0.846153846153845,-0.83076923076923,
-0.815384615384614,-0.799999999999999,-0.784615384615384,-0.769230769230768,
-0.753846153846153,-0.738461538461538,-0.723076923076922,-0.707692307692307,
-0.692307692307692,-0.676923076923076,-0.661538461538461,-0.646153846153846,
-0.63076923076923,-0.615384615384615,-0.6,-0.584615384615384,-0.569230769230769,
-0.553846153846154,-0.538461538461538,-0.523076923076923,-0.507692307692308,
-0.492307692307692,-0.476923076923077,-0.461538461538462,-0.446153846153846,
-0.430769230769231,-0.415384615384615,-0.4,-0.384615384615385,-0.369230769230769,
-0.353846153846154,-0.338461538461538,-0.323076923076923,-0.307692307692308,
-0.292307692307692,-0.276923076923077,-0.261538461538462,-0.246153846153846,
-0.230769230769231,-0.215384615384615,-0.2,-0.184615384615385,-0.169230769230769,
-0.153846153846154,-0.138461538461538,-0.123076923076923,-0.107692307692308,
-0.0923076923076923,-0.0769230769230769,-0.0615384615384615,-0.0461538461538462,
-0.0307692307692308,-0.0153846153846154,-0.00577184337451372),
 .UNSPECIFIED.)
CURVE()
GEOMETRIC_REPRESENTATION_ITEM()
RATIONAL_B_SPLINE_CURVE((1.,1.,1.,1.,1.,1.,1.,1.,1.,1.,1.,1.,1.,1.,1.,1.,
1.,1.,1.,1.,1.,1.,1.,1.,1.,1.,1.,1.,1.,1.,1.,1.,1.,1.,1.,1.,1.,1.,1.,1.,
1.,1.,1.,1.,1.,1.,1.,1.,1.,1.,1.,1.,1.,1.,1.,1.,1.,1.,1.,1.,1.,1.,1.,1.,
1.,1.,1.,1.,1.,1.))
REPRESENTATION_ITEM('')
);
#326=(
BOUNDED_CURVE()
B_SPLINE_CURVE(5,(#43881,#43882,#43883,#43884,#43885,#43886,#43887,#43888,
#43889,#43890,#43891,#43892,#43893,#43894,#43895,#43896,#43897,#43898,#43899,
#43900,#43901,#43902,#43903,#43904,#43905,#43906,#43907,#43908,#43909,#43910,
#43911,#43912,#43913,#43914,#43915,#43916,#43917,#43918,#43919,#43920,#43921,
#43922,#43923,#43924,#43925,#43926,#43927,#43928,#43929,#43930,#43931,#43932,
#43933,#43934,#43935,#43936,#43937,#43938,#43939,#43940,#43941,#43942,#43943,
#43944,#43945,#43946,#43947,#43948,#43949,#43950),.UNSPECIFIED.,.F.,.F.)
B_SPLINE_CURVE_WITH_KNOTS((6,1,1,1,1,1,1,1,1,1,1,1,1,1,1,1,1,1,1,1,1,1,
1,1,1,1,1,1,1,1,1,1,1,1,1,1,1,1,1,1,1,1,1,1,1,1,1,1,1,1,1,1,1,1,1,1,1,1,
1,1,1,1,1,1,1,6),(-0.994228156739703,-0.984615384615383,-0.969230769230768,
-0.953846153846152,-0.938461538461537,-0.923076923076922,-0.907692307692306,
-0.892307692307691,-0.876923076923076,-0.86153846153846,-0.846153846153845,
-0.83076923076923,-0.815384615384614,-0.799999999999999,-0.784615384615384,
-0.769230769230768,-0.753846153846153,-0.738461538461538,-0.723076923076922,
-0.707692307692307,-0.692307692307692,-0.676923076923076,-0.661538461538461,
-0.646153846153846,-0.63076923076923,-0.615384615384615,-0.6,-0.584615384615384,
-0.569230769230769,-0.553846153846154,-0.538461538461538,-0.523076923076923,
-0.507692307692308,-0.492307692307692,-0.476923076923077,-0.461538461538462,
-0.446153846153846,-0.430769230769231,-0.415384615384615,-0.4,-0.384615384615385,
-0.369230769230769,-0.353846153846154,-0.338461538461538,-0.323076923076923,
-0.307692307692308,-0.292307692307692,-0.276923076923077,-0.261538461538462,
-0.246153846153846,-0.230769230769231,-0.215384615384615,-0.2,-0.184615384615385,
-0.169230769230769,-0.153846153846154,-0.138461538461538,-0.123076923076923,
-0.107692307692308,-0.0923076923076923,-0.0769230769230769,-0.0615384615384615,
-0.0461538461538462,-0.0307692307692308,-0.0153846153846154,0.),
 .UNSPECIFIED.)
CURVE()
GEOMETRIC_REPRESENTATION_ITEM()
RATIONAL_B_SPLINE_CURVE((1.,1.,1.,1.,1.,1.,1.,1.,1.,1.,1.,1.,1.,1.,1.,1.,
1.,1.,1.,1.,1.,1.,1.,1.,1.,1.,1.,1.,1.,1.,1.,1.,1.,1.,1.,1.,1.,1.,1.,1.,
1.,1.,1.,1.,1.,1.,1.,1.,1.,1.,1.,1.,1.,1.,1.,1.,1.,1.,1.,1.,1.,1.,1.,1.,
1.,1.,1.,1.,1.,1.))
REPRESENTATION_ITEM('')
);
#327=(
BOUNDED_CURVE()
B_SPLINE_CURVE(5,(#44103,#44104,#44105,#44106,#44107,#44108,#44109,#44110,
#44111,#44112,#44113,#44114,#44115,#44116,#44117,#44118,#44119,#44120,#44121,
#44122,#44123,#44124,#44125,#44126,#44127,#44128,#44129,#44130,#44131,#44132,
#44133,#44134,#44135,#44136,#44137,#44138,#44139,#44140,#44141,#44142,#44143,
#44144,#44145,#44146,#44147,#44148,#44149,#44150,#44151,#44152,#44153,#44154,
#44155,#44156,#44157,#44158,#44159,#44160,#44161,#44162,#44163,#44164,#44165,
#44166,#44167,#44168,#44169,#44170,#44171,#44172),.UNSPECIFIED.,.F.,.F.)
B_SPLINE_CURVE_WITH_KNOTS((6,1,1,1,1,1,1,1,1,1,1,1,1,1,1,1,1,1,1,1,1,1,
1,1,1,1,1,1,1,1,1,1,1,1,1,1,1,1,1,1,1,1,1,1,1,1,1,1,1,1,1,1,1,1,1,1,1,1,
1,1,1,1,1,1,1,6),(-1.,-0.984615384615383,-0.969230769230768,-0.953846153846152,
-0.938461538461537,-0.923076923076922,-0.907692307692306,-0.892307692307691,
-0.876923076923076,-0.86153846153846,-0.846153846153845,-0.83076923076923,
-0.815384615384614,-0.799999999999999,-0.784615384615384,-0.769230769230768,
-0.753846153846153,-0.738461538461538,-0.723076923076922,-0.707692307692307,
-0.692307692307692,-0.676923076923076,-0.661538461538461,-0.646153846153846,
-0.63076923076923,-0.615384615384615,-0.6,-0.584615384615384,-0.569230769230769,
-0.553846153846154,-0.538461538461538,-0.523076923076923,-0.507692307692308,
-0.492307692307692,-0.476923076923077,-0.461538461538462,-0.446153846153846,
-0.430769230769231,-0.415384615384615,-0.4,-0.384615384615385,-0.369230769230769,
-0.353846153846154,-0.338461538461538,-0.323076923076923,-0.307692307692308,
-0.292307692307692,-0.276923076923077,-0.261538461538462,-0.246153846153846,
-0.230769230769231,-0.215384615384615,-0.2,-0.184615384615385,-0.169230769230769,
-0.153846153846154,-0.138461538461538,-0.123076923076923,-0.107692307692308,
-0.0923076923076923,-0.0769230769230769,-0.0615384615384615,-0.0461538461538462,
-0.0307692307692308,-0.0153846153846154,-0.00577184337451698),
 .UNSPECIFIED.)
CURVE()
GEOMETRIC_REPRESENTATION_ITEM()
RATIONAL_B_SPLINE_CURVE((1.,1.,1.,1.,1.,1.,1.,1.,1.,1.,1.,1.,1.,1.,1.,1.,
1.,1.,1.,1.,1.,1.,1.,1.,1.,1.,1.,1.,1.,1.,1.,1.,1.,1.,1.,1.,1.,1.,1.,1.,
1.,1.,1.,1.,1.,1.,1.,1.,1.,1.,1.,1.,1.,1.,1.,1.,1.,1.,1.,1.,1.,1.,1.,1.,
1.,1.,1.,1.,1.,1.))
REPRESENTATION_ITEM('')
);
#328=(
BOUNDED_CURVE()
B_SPLINE_CURVE(5,(#44323,#44324,#44325,#44326,#44327,#44328,#44329,#44330,
#44331,#44332,#44333,#44334,#44335,#44336,#44337,#44338,#44339,#44340,#44341,
#44342,#44343,#44344,#44345,#44346,#44347,#44348,#44349,#44350,#44351,#44352,
#44353,#44354,#44355,#44356,#44357,#44358,#44359,#44360,#44361,#44362,#44363,
#44364,#44365,#44366,#44367,#44368,#44369,#44370,#44371,#44372,#44373,#44374,
#44375,#44376,#44377,#44378,#44379,#44380,#44381,#44382,#44383,#44384,#44385,
#44386,#44387,#44388,#44389,#44390,#44391,#44392),.UNSPECIFIED.,.F.,.F.)
B_SPLINE_CURVE_WITH_KNOTS((6,1,1,1,1,1,1,1,1,1,1,1,1,1,1,1,1,1,1,1,1,1,
1,1,1,1,1,1,1,1,1,1,1,1,1,1,1,1,1,1,1,1,1,1,1,1,1,1,1,1,1,1,1,1,1,1,1,1,
1,1,1,1,1,1,1,6),(-0.994228156739706,-0.984615384615383,-0.969230769230768,
-0.953846153846152,-0.938461538461537,-0.923076923076922,-0.907692307692306,
-0.892307692307691,-0.876923076923076,-0.86153846153846,-0.846153846153845,
-0.83076923076923,-0.815384615384614,-0.799999999999999,-0.784615384615384,
-0.769230769230768,-0.753846153846153,-0.738461538461538,-0.723076923076922,
-0.707692307692307,-0.692307692307692,-0.676923076923076,-0.661538461538461,
-0.646153846153846,-0.63076923076923,-0.615384615384615,-0.6,-0.584615384615384,
-0.569230769230769,-0.553846153846154,-0.538461538461538,-0.523076923076923,
-0.507692307692308,-0.492307692307692,-0.476923076923077,-0.461538461538462,
-0.446153846153846,-0.430769230769231,-0.415384615384615,-0.4,-0.384615384615385,
-0.369230769230769,-0.353846153846154,-0.338461538461538,-0.323076923076923,
-0.307692307692308,-0.292307692307692,-0.276923076923077,-0.261538461538462,
-0.246153846153846,-0.230769230769231,-0.215384615384615,-0.2,-0.184615384615385,
-0.169230769230769,-0.153846153846154,-0.138461538461538,-0.123076923076923,
-0.107692307692308,-0.0923076923076923,-0.0769230769230769,-0.0615384615384615,
-0.0461538461538462,-0.0307692307692308,-0.0153846153846154,0.),
 .UNSPECIFIED.)
CURVE()
GEOMETRIC_REPRESENTATION_ITEM()
RATIONAL_B_SPLINE_CURVE((1.,1.,1.,1.,1.,1.,1.,1.,1.,1.,1.,1.,1.,1.,1.,1.,
1.,1.,1.,1.,1.,1.,1.,1.,1.,1.,1.,1.,1.,1.,1.,1.,1.,1.,1.,1.,1.,1.,1.,1.,
1.,1.,1.,1.,1.,1.,1.,1.,1.,1.,1.,1.,1.,1.,1.,1.,1.,1.,1.,1.,1.,1.,1.,1.,
1.,1.,1.,1.,1.,1.))
REPRESENTATION_ITEM('')
);
#329=(
BOUNDED_CURVE()
B_SPLINE_CURVE(5,(#44545,#44546,#44547,#44548,#44549,#44550,#44551,#44552,
#44553,#44554,#44555,#44556,#44557,#44558,#44559,#44560,#44561,#44562,#44563,
#44564,#44565,#44566,#44567,#44568,#44569,#44570,#44571,#44572,#44573,#44574,
#44575,#44576,#44577,#44578,#44579,#44580,#44581,#44582,#44583,#44584,#44585,
#44586,#44587,#44588,#44589,#44590,#44591,#44592,#44593,#44594,#44595,#44596,
#44597,#44598,#44599,#44600,#44601,#44602,#44603,#44604,#44605,#44606,#44607,
#44608,#44609,#44610,#44611,#44612,#44613,#44614),.UNSPECIFIED.,.F.,.F.)
B_SPLINE_CURVE_WITH_KNOTS((6,1,1,1,1,1,1,1,1,1,1,1,1,1,1,1,1,1,1,1,1,1,
1,1,1,1,1,1,1,1,1,1,1,1,1,1,1,1,1,1,1,1,1,1,1,1,1,1,1,1,1,1,1,1,1,1,1,1,
1,1,1,1,1,1,1,6),(-1.,-0.984615384615383,-0.969230769230768,-0.953846153846152,
-0.938461538461537,-0.923076923076922,-0.907692307692306,-0.892307692307691,
-0.876923076923076,-0.86153846153846,-0.846153846153845,-0.83076923076923,
-0.815384615384614,-0.799999999999999,-0.784615384615384,-0.769230769230768,
-0.753846153846153,-0.738461538461538,-0.723076923076922,-0.707692307692307,
-0.692307692307692,-0.676923076923076,-0.661538461538461,-0.646153846153846,
-0.63076923076923,-0.615384615384615,-0.6,-0.584615384615384,-0.569230769230769,
-0.553846153846154,-0.538461538461538,-0.523076923076923,-0.507692307692308,
-0.492307692307692,-0.476923076923077,-0.461538461538462,-0.446153846153846,
-0.430769230769231,-0.415384615384615,-0.4,-0.384615384615385,-0.369230769230769,
-0.353846153846154,-0.338461538461538,-0.323076923076923,-0.307692307692308,
-0.292307692307692,-0.276923076923077,-0.261538461538462,-0.246153846153846,
-0.230769230769231,-0.215384615384615,-0.2,-0.184615384615385,-0.169230769230769,
-0.153846153846154,-0.138461538461538,-0.123076923076923,-0.107692307692308,
-0.0923076923076923,-0.0769230769230769,-0.0615384615384615,-0.0461538461538462,
-0.0307692307692308,-0.0153846153846154,-0.00577184337452512),
 .UNSPECIFIED.)
CURVE()
GEOMETRIC_REPRESENTATION_ITEM()
RATIONAL_B_SPLINE_CURVE((1.,1.,1.,1.,1.,1.,1.,1.,1.,1.,1.,1.,1.,1.,1.,1.,
1.,1.,1.,1.,1.,1.,1.,1.,1.,1.,1.,1.,1.,1.,1.,1.,1.,1.,1.,1.,1.,1.,1.,1.,
1.,1.,1.,1.,1.,1.,1.,1.,1.,1.,1.,1.,1.,1.,1.,1.,1.,1.,1.,1.,1.,1.,1.,1.,
1.,1.,1.,1.,1.,1.))
REPRESENTATION_ITEM('')
);
#330=(
BOUNDED_CURVE()
B_SPLINE_CURVE(5,(#44765,#44766,#44767,#44768,#44769,#44770,#44771,#44772,
#44773,#44774,#44775,#44776,#44777,#44778,#44779,#44780,#44781,#44782,#44783,
#44784,#44785,#44786,#44787,#44788,#44789,#44790,#44791,#44792,#44793,#44794,
#44795,#44796,#44797,#44798,#44799,#44800,#44801,#44802,#44803,#44804,#44805,
#44806,#44807,#44808,#44809,#44810,#44811,#44812,#44813,#44814,#44815,#44816,
#44817,#44818,#44819,#44820,#44821,#44822,#44823,#44824,#44825,#44826,#44827,
#44828,#44829,#44830,#44831,#44832,#44833,#44834),.UNSPECIFIED.,.F.,.F.)
B_SPLINE_CURVE_WITH_KNOTS((6,1,1,1,1,1,1,1,1,1,1,1,1,1,1,1,1,1,1,1,1,1,
1,1,1,1,1,1,1,1,1,1,1,1,1,1,1,1,1,1,1,1,1,1,1,1,1,1,1,1,1,1,1,1,1,1,1,1,
1,1,1,1,1,1,1,6),(-0.994228156739713,-0.984615384615383,-0.969230769230768,
-0.953846153846152,-0.938461538461537,-0.923076923076922,-0.907692307692306,
-0.892307692307691,-0.876923076923076,-0.86153846153846,-0.846153846153845,
-0.83076923076923,-0.815384615384614,-0.799999999999999,-0.784615384615384,
-0.769230769230768,-0.753846153846153,-0.738461538461538,-0.723076923076922,
-0.707692307692307,-0.692307692307692,-0.676923076923076,-0.661538461538461,
-0.646153846153846,-0.63076923076923,-0.615384615384615,-0.6,-0.584615384615384,
-0.569230769230769,-0.553846153846154,-0.538461538461538,-0.523076923076923,
-0.507692307692308,-0.492307692307692,-0.476923076923077,-0.461538461538462,
-0.446153846153846,-0.430769230769231,-0.415384615384615,-0.4,-0.384615384615385,
-0.369230769230769,-0.353846153846154,-0.338461538461538,-0.323076923076923,
-0.307692307692308,-0.292307692307692,-0.276923076923077,-0.261538461538462,
-0.246153846153846,-0.230769230769231,-0.215384615384615,-0.2,-0.184615384615385,
-0.169230769230769,-0.153846153846154,-0.138461538461538,-0.123076923076923,
-0.107692307692308,-0.0923076923076923,-0.0769230769230769,-0.0615384615384615,
-0.0461538461538462,-0.0307692307692308,-0.0153846153846154,0.),
 .UNSPECIFIED.)
CURVE()
GEOMETRIC_REPRESENTATION_ITEM()
RATIONAL_B_SPLINE_CURVE((1.,1.,1.,1.,1.,1.,1.,1.,1.,1.,1.,1.,1.,1.,1.,1.,
1.,1.,1.,1.,1.,1.,1.,1.,1.,1.,1.,1.,1.,1.,1.,1.,1.,1.,1.,1.,1.,1.,1.,1.,
1.,1.,1.,1.,1.,1.,1.,1.,1.,1.,1.,1.,1.,1.,1.,1.,1.,1.,1.,1.,1.,1.,1.,1.,
1.,1.,1.,1.,1.,1.))
REPRESENTATION_ITEM('')
);
#331=(
BOUNDED_CURVE()
B_SPLINE_CURVE(5,(#44987,#44988,#44989,#44990,#44991,#44992,#44993,#44994,
#44995,#44996,#44997,#44998,#44999,#45000,#45001,#45002,#45003,#45004,#45005,
#45006,#45007,#45008,#45009,#45010,#45011,#45012,#45013,#45014,#45015,#45016,
#45017,#45018,#45019,#45020,#45021,#45022,#45023,#45024,#45025,#45026,#45027,
#45028,#45029,#45030,#45031,#45032,#45033,#45034,#45035,#45036,#45037,#45038,
#45039,#45040,#45041,#45042,#45043,#45044,#45045,#45046,#45047,#45048,#45049,
#45050,#45051,#45052,#45053,#45054,#45055,#45056),.UNSPECIFIED.,.F.,.F.)
B_SPLINE_CURVE_WITH_KNOTS((6,1,1,1,1,1,1,1,1,1,1,1,1,1,1,1,1,1,1,1,1,1,
1,1,1,1,1,1,1,1,1,1,1,1,1,1,1,1,1,1,1,1,1,1,1,1,1,1,1,1,1,1,1,1,1,1,1,1,
1,1,1,1,1,1,1,6),(-1.,-0.984615384615383,-0.969230769230768,-0.953846153846152,
-0.938461538461537,-0.923076923076922,-0.907692307692306,-0.892307692307691,
-0.876923076923076,-0.86153846153846,-0.846153846153845,-0.83076923076923,
-0.815384615384614,-0.799999999999999,-0.784615384615384,-0.769230769230768,
-0.753846153846153,-0.738461538461538,-0.723076923076922,-0.707692307692307,
-0.692307692307692,-0.676923076923076,-0.661538461538461,-0.646153846153846,
-0.63076923076923,-0.615384615384615,-0.6,-0.584615384615384,-0.569230769230769,
-0.553846153846154,-0.538461538461538,-0.523076923076923,-0.507692307692308,
-0.492307692307692,-0.476923076923077,-0.461538461538462,-0.446153846153846,
-0.430769230769231,-0.415384615384615,-0.4,-0.384615384615385,-0.369230769230769,
-0.353846153846154,-0.338461538461538,-0.323076923076923,-0.307692307692308,
-0.292307692307692,-0.276923076923077,-0.261538461538462,-0.246153846153846,
-0.230769230769231,-0.215384615384615,-0.2,-0.184615384615385,-0.169230769230769,
-0.153846153846154,-0.138461538461538,-0.123076923076923,-0.107692307692308,
-0.0923076923076923,-0.0769230769230769,-0.0615384615384615,-0.0461538461538462,
-0.0307692307692308,-0.0153846153846154,-0.00577184337450204),
 .UNSPECIFIED.)
CURVE()
GEOMETRIC_REPRESENTATION_ITEM()
RATIONAL_B_SPLINE_CURVE((1.,1.,1.,1.,1.,1.,1.,1.,1.,1.,1.,1.,1.,1.,1.,1.,
1.,1.,1.,1.,1.,1.,1.,1.,1.,1.,1.,1.,1.,1.,1.,1.,1.,1.,1.,1.,1.,1.,1.,1.,
1.,1.,1.,1.,1.,1.,1.,1.,1.,1.,1.,1.,1.,1.,1.,1.,1.,1.,1.,1.,1.,1.,1.,1.,
1.,1.,1.,1.,1.,1.))
REPRESENTATION_ITEM('')
);
#332=(
BOUNDED_CURVE()
B_SPLINE_CURVE(5,(#45207,#45208,#45209,#45210,#45211,#45212,#45213,#45214,
#45215,#45216,#45217,#45218,#45219,#45220,#45221,#45222,#45223,#45224,#45225,
#45226,#45227,#45228,#45229,#45230,#45231,#45232,#45233,#45234,#45235,#45236,
#45237,#45238,#45239,#45240,#45241,#45242,#45243,#45244,#45245,#45246,#45247,
#45248,#45249,#45250,#45251,#45252,#45253,#45254,#45255,#45256,#45257,#45258,
#45259,#45260,#45261,#45262,#45263,#45264,#45265,#45266,#45267,#45268,#45269,
#45270,#45271,#45272,#45273,#45274,#45275,#45276),.UNSPECIFIED.,.F.,.F.)
B_SPLINE_CURVE_WITH_KNOTS((6,1,1,1,1,1,1,1,1,1,1,1,1,1,1,1,1,1,1,1,1,1,
1,1,1,1,1,1,1,1,1,1,1,1,1,1,1,1,1,1,1,1,1,1,1,1,1,1,1,1,1,1,1,1,1,1,1,1,
1,1,1,1,1,1,1,6),(-0.99422815673972,-0.984615384615383,-0.969230769230768,
-0.953846153846152,-0.938461538461537,-0.923076923076922,-0.907692307692306,
-0.892307692307691,-0.876923076923076,-0.86153846153846,-0.846153846153845,
-0.83076923076923,-0.815384615384614,-0.799999999999999,-0.784615384615384,
-0.769230769230768,-0.753846153846153,-0.738461538461538,-0.723076923076922,
-0.707692307692307,-0.692307692307692,-0.676923076923076,-0.661538461538461,
-0.646153846153846,-0.63076923076923,-0.615384615384615,-0.6,-0.584615384615384,
-0.569230769230769,-0.553846153846154,-0.538461538461538,-0.523076923076923,
-0.507692307692308,-0.492307692307692,-0.476923076923077,-0.461538461538462,
-0.446153846153846,-0.430769230769231,-0.415384615384615,-0.4,-0.384615384615385,
-0.369230769230769,-0.353846153846154,-0.338461538461538,-0.323076923076923,
-0.307692307692308,-0.292307692307692,-0.276923076923077,-0.261538461538462,
-0.246153846153846,-0.230769230769231,-0.215384615384615,-0.2,-0.184615384615385,
-0.169230769230769,-0.153846153846154,-0.138461538461538,-0.123076923076923,
-0.107692307692308,-0.0923076923076923,-0.0769230769230769,-0.0615384615384615,
-0.0461538461538462,-0.0307692307692308,-0.0153846153846154,0.),
 .UNSPECIFIED.)
CURVE()
GEOMETRIC_REPRESENTATION_ITEM()
RATIONAL_B_SPLINE_CURVE((1.,1.,1.,1.,1.,1.,1.,1.,1.,1.,1.,1.,1.,1.,1.,1.,
1.,1.,1.,1.,1.,1.,1.,1.,1.,1.,1.,1.,1.,1.,1.,1.,1.,1.,1.,1.,1.,1.,1.,1.,
1.,1.,1.,1.,1.,1.,1.,1.,1.,1.,1.,1.,1.,1.,1.,1.,1.,1.,1.,1.,1.,1.,1.,1.,
1.,1.,1.,1.,1.,1.))
REPRESENTATION_ITEM('')
);
#333=(
BOUNDED_CURVE()
B_SPLINE_CURVE(5,(#45429,#45430,#45431,#45432,#45433,#45434,#45435,#45436,
#45437,#45438,#45439,#45440,#45441,#45442,#45443,#45444,#45445,#45446,#45447,
#45448,#45449,#45450,#45451,#45452,#45453,#45454,#45455,#45456,#45457,#45458,
#45459,#45460,#45461,#45462,#45463,#45464,#45465,#45466,#45467,#45468,#45469,
#45470,#45471,#45472,#45473,#45474,#45475,#45476,#45477,#45478,#45479,#45480,
#45481,#45482,#45483,#45484,#45485,#45486,#45487,#45488,#45489,#45490,#45491,
#45492,#45493,#45494,#45495,#45496,#45497,#45498),.UNSPECIFIED.,.F.,.F.)
B_SPLINE_CURVE_WITH_KNOTS((6,1,1,1,1,1,1,1,1,1,1,1,1,1,1,1,1,1,1,1,1,1,
1,1,1,1,1,1,1,1,1,1,1,1,1,1,1,1,1,1,1,1,1,1,1,1,1,1,1,1,1,1,1,1,1,1,1,1,
1,1,1,1,1,1,1,6),(-1.,-0.984615384615383,-0.969230769230768,-0.953846153846152,
-0.938461538461537,-0.923076923076922,-0.907692307692306,-0.892307692307691,
-0.876923076923076,-0.86153846153846,-0.846153846153845,-0.83076923076923,
-0.815384615384614,-0.799999999999999,-0.784615384615384,-0.769230769230768,
-0.753846153846153,-0.738461538461538,-0.723076923076922,-0.707692307692307,
-0.692307692307692,-0.676923076923076,-0.661538461538461,-0.646153846153846,
-0.63076923076923,-0.615384615384615,-0.6,-0.584615384615384,-0.569230769230769,
-0.553846153846154,-0.538461538461538,-0.523076923076923,-0.507692307692308,
-0.492307692307692,-0.476923076923077,-0.461538461538462,-0.446153846153846,
-0.430769230769231,-0.415384615384615,-0.4,-0.384615384615385,-0.369230769230769,
-0.353846153846154,-0.338461538461538,-0.323076923076923,-0.307692307692308,
-0.292307692307692,-0.276923076923077,-0.261538461538462,-0.246153846153846,
-0.230769230769231,-0.215384615384615,-0.2,-0.184615384615385,-0.169230769230769,
-0.153846153846154,-0.138461538461538,-0.123076923076923,-0.107692307692308,
-0.0923076923076923,-0.0769230769230769,-0.0615384615384615,-0.0461538461538462,
-0.0307692307692308,-0.0153846153846154,-0.0057718433745107),
 .UNSPECIFIED.)
CURVE()
GEOMETRIC_REPRESENTATION_ITEM()
RATIONAL_B_SPLINE_CURVE((1.,1.,1.,1.,1.,1.,1.,1.,1.,1.,1.,1.,1.,1.,1.,1.,
1.,1.,1.,1.,1.,1.,1.,1.,1.,1.,1.,1.,1.,1.,1.,1.,1.,1.,1.,1.,1.,1.,1.,1.,
1.,1.,1.,1.,1.,1.,1.,1.,1.,1.,1.,1.,1.,1.,1.,1.,1.,1.,1.,1.,1.,1.,1.,1.,
1.,1.,1.,1.,1.,1.))
REPRESENTATION_ITEM('')
);
#334=(
BOUNDED_CURVE()
B_SPLINE_CURVE(5,(#45649,#45650,#45651,#45652,#45653,#45654,#45655,#45656,
#45657,#45658,#45659,#45660,#45661,#45662,#45663,#45664,#45665,#45666,#45667,
#45668,#45669,#45670,#45671,#45672,#45673,#45674,#45675,#45676,#45677,#45678,
#45679,#45680,#45681,#45682,#45683,#45684,#45685,#45686,#45687,#45688,#45689,
#45690,#45691,#45692,#45693,#45694,#45695,#45696,#45697,#45698,#45699,#45700,
#45701,#45702,#45703,#45704,#45705,#45706,#45707,#45708,#45709,#45710,#45711,
#45712,#45713,#45714,#45715,#45716,#45717,#45718),.UNSPECIFIED.,.F.,.F.)
B_SPLINE_CURVE_WITH_KNOTS((6,1,1,1,1,1,1,1,1,1,1,1,1,1,1,1,1,1,1,1,1,1,
1,1,1,1,1,1,1,1,1,1,1,1,1,1,1,1,1,1,1,1,1,1,1,1,1,1,1,1,1,1,1,1,1,1,1,1,
1,1,1,1,1,1,1,6),(-0.994228156739708,-0.984615384615383,-0.969230769230768,
-0.953846153846152,-0.938461538461537,-0.923076923076922,-0.907692307692306,
-0.892307692307691,-0.876923076923076,-0.86153846153846,-0.846153846153845,
-0.83076923076923,-0.815384615384614,-0.799999999999999,-0.784615384615384,
-0.769230769230768,-0.753846153846153,-0.738461538461538,-0.723076923076922,
-0.707692307692307,-0.692307692307692,-0.676923076923076,-0.661538461538461,
-0.646153846153846,-0.63076923076923,-0.615384615384615,-0.6,-0.584615384615384,
-0.569230769230769,-0.553846153846154,-0.538461538461538,-0.523076923076923,
-0.507692307692308,-0.492307692307692,-0.476923076923077,-0.461538461538462,
-0.446153846153846,-0.430769230769231,-0.415384615384615,-0.4,-0.384615384615385,
-0.369230769230769,-0.353846153846154,-0.338461538461538,-0.323076923076923,
-0.307692307692308,-0.292307692307692,-0.276923076923077,-0.261538461538462,
-0.246153846153846,-0.230769230769231,-0.215384615384615,-0.2,-0.184615384615385,
-0.169230769230769,-0.153846153846154,-0.138461538461538,-0.123076923076923,
-0.107692307692308,-0.0923076923076923,-0.0769230769230769,-0.0615384615384615,
-0.0461538461538462,-0.0307692307692308,-0.0153846153846154,0.),
 .UNSPECIFIED.)
CURVE()
GEOMETRIC_REPRESENTATION_ITEM()
RATIONAL_B_SPLINE_CURVE((1.,1.,1.,1.,1.,1.,1.,1.,1.,1.,1.,1.,1.,1.,1.,1.,
1.,1.,1.,1.,1.,1.,1.,1.,1.,1.,1.,1.,1.,1.,1.,1.,1.,1.,1.,1.,1.,1.,1.,1.,
1.,1.,1.,1.,1.,1.,1.,1.,1.,1.,1.,1.,1.,1.,1.,1.,1.,1.,1.,1.,1.,1.,1.,1.,
1.,1.,1.,1.,1.,1.))
REPRESENTATION_ITEM('')
);
#335=(
BOUNDED_CURVE()
B_SPLINE_CURVE(5,(#45871,#45872,#45873,#45874,#45875,#45876,#45877,#45878,
#45879,#45880,#45881,#45882,#45883,#45884,#45885,#45886,#45887,#45888,#45889,
#45890,#45891,#45892,#45893,#45894,#45895,#45896,#45897,#45898,#45899,#45900,
#45901,#45902,#45903,#45904,#45905,#45906,#45907,#45908,#45909,#45910,#45911,
#45912,#45913,#45914,#45915,#45916,#45917,#45918,#45919,#45920,#45921,#45922,
#45923,#45924,#45925,#45926,#45927,#45928,#45929,#45930,#45931,#45932,#45933,
#45934,#45935,#45936,#45937,#45938,#45939,#45940),.UNSPECIFIED.,.F.,.F.)
B_SPLINE_CURVE_WITH_KNOTS((6,1,1,1,1,1,1,1,1,1,1,1,1,1,1,1,1,1,1,1,1,1,
1,1,1,1,1,1,1,1,1,1,1,1,1,1,1,1,1,1,1,1,1,1,1,1,1,1,1,1,1,1,1,1,1,1,1,1,
1,1,1,1,1,1,1,6),(-1.,-0.984615384615383,-0.969230769230768,-0.953846153846152,
-0.938461538461537,-0.923076923076922,-0.907692307692306,-0.892307692307691,
-0.876923076923076,-0.86153846153846,-0.846153846153845,-0.83076923076923,
-0.815384615384614,-0.799999999999999,-0.784615384615384,-0.769230769230768,
-0.753846153846153,-0.738461538461538,-0.723076923076922,-0.707692307692307,
-0.692307692307692,-0.676923076923076,-0.661538461538461,-0.646153846153846,
-0.63076923076923,-0.615384615384615,-0.6,-0.584615384615384,-0.569230769230769,
-0.553846153846154,-0.538461538461538,-0.523076923076923,-0.507692307692308,
-0.492307692307692,-0.476923076923077,-0.461538461538462,-0.446153846153846,
-0.430769230769231,-0.415384615384615,-0.4,-0.384615384615385,-0.369230769230769,
-0.353846153846154,-0.338461538461538,-0.323076923076923,-0.307692307692308,
-0.292307692307692,-0.276923076923077,-0.261538461538462,-0.246153846153846,
-0.230769230769231,-0.215384615384615,-0.2,-0.184615384615385,-0.169230769230769,
-0.153846153846154,-0.138461538461538,-0.123076923076923,-0.107692307692308,
-0.0923076923076923,-0.0769230769230769,-0.0615384615384615,-0.0461538461538462,
-0.0307692307692308,-0.0153846153846154,-0.00577184337451708),
 .UNSPECIFIED.)
CURVE()
GEOMETRIC_REPRESENTATION_ITEM()
RATIONAL_B_SPLINE_CURVE((1.,1.,1.,1.,1.,1.,1.,1.,1.,1.,1.,1.,1.,1.,1.,1.,
1.,1.,1.,1.,1.,1.,1.,1.,1.,1.,1.,1.,1.,1.,1.,1.,1.,1.,1.,1.,1.,1.,1.,1.,
1.,1.,1.,1.,1.,1.,1.,1.,1.,1.,1.,1.,1.,1.,1.,1.,1.,1.,1.,1.,1.,1.,1.,1.,
1.,1.,1.,1.,1.,1.))
REPRESENTATION_ITEM('')
);
#336=(
BOUNDED_CURVE()
B_SPLINE_CURVE(5,(#46091,#46092,#46093,#46094,#46095,#46096,#46097,#46098,
#46099,#46100,#46101,#46102,#46103,#46104,#46105,#46106,#46107,#46108,#46109,
#46110,#46111,#46112,#46113,#46114,#46115,#46116,#46117,#46118,#46119,#46120,
#46121,#46122,#46123,#46124,#46125,#46126,#46127,#46128,#46129,#46130,#46131,
#46132,#46133,#46134,#46135,#46136,#46137,#46138,#46139,#46140,#46141,#46142,
#46143,#46144,#46145,#46146,#46147,#46148,#46149,#46150,#46151,#46152,#46153,
#46154,#46155,#46156,#46157,#46158,#46159,#46160),.UNSPECIFIED.,.F.,.F.)
B_SPLINE_CURVE_WITH_KNOTS((6,1,1,1,1,1,1,1,1,1,1,1,1,1,1,1,1,1,1,1,1,1,
1,1,1,1,1,1,1,1,1,1,1,1,1,1,1,1,1,1,1,1,1,1,1,1,1,1,1,1,1,1,1,1,1,1,1,1,
1,1,1,1,1,1,1,6),(-0.994228156739669,-0.984615384615383,-0.969230769230768,
-0.953846153846152,-0.938461538461537,-0.923076923076922,-0.907692307692306,
-0.892307692307691,-0.876923076923076,-0.86153846153846,-0.846153846153845,
-0.83076923076923,-0.815384615384614,-0.799999999999999,-0.784615384615384,
-0.769230769230768,-0.753846153846153,-0.738461538461538,-0.723076923076922,
-0.707692307692307,-0.692307692307692,-0.676923076923076,-0.661538461538461,
-0.646153846153846,-0.63076923076923,-0.615384615384615,-0.6,-0.584615384615384,
-0.569230769230769,-0.553846153846154,-0.538461538461538,-0.523076923076923,
-0.507692307692308,-0.492307692307692,-0.476923076923077,-0.461538461538462,
-0.446153846153846,-0.430769230769231,-0.415384615384615,-0.4,-0.384615384615385,
-0.369230769230769,-0.353846153846154,-0.338461538461538,-0.323076923076923,
-0.307692307692308,-0.292307692307692,-0.276923076923077,-0.261538461538462,
-0.246153846153846,-0.230769230769231,-0.215384615384615,-0.2,-0.184615384615385,
-0.169230769230769,-0.153846153846154,-0.138461538461538,-0.123076923076923,
-0.107692307692308,-0.0923076923076923,-0.0769230769230769,-0.0615384615384615,
-0.0461538461538462,-0.0307692307692308,-0.0153846153846154,0.),
 .UNSPECIFIED.)
CURVE()
GEOMETRIC_REPRESENTATION_ITEM()
RATIONAL_B_SPLINE_CURVE((1.,1.,1.,1.,1.,1.,1.,1.,1.,1.,1.,1.,1.,1.,1.,1.,
1.,1.,1.,1.,1.,1.,1.,1.,1.,1.,1.,1.,1.,1.,1.,1.,1.,1.,1.,1.,1.,1.,1.,1.,
1.,1.,1.,1.,1.,1.,1.,1.,1.,1.,1.,1.,1.,1.,1.,1.,1.,1.,1.,1.,1.,1.,1.,1.,
1.,1.,1.,1.,1.,1.))
REPRESENTATION_ITEM('')
);
#337=(
BOUNDED_CURVE()
B_SPLINE_CURVE(5,(#46313,#46314,#46315,#46316,#46317,#46318,#46319,#46320,
#46321,#46322,#46323,#46324,#46325,#46326,#46327,#46328,#46329,#46330,#46331,
#46332,#46333,#46334,#46335,#46336,#46337,#46338,#46339,#46340,#46341,#46342,
#46343,#46344,#46345,#46346,#46347,#46348,#46349,#46350,#46351,#46352,#46353,
#46354,#46355,#46356,#46357,#46358,#46359,#46360,#46361,#46362,#46363,#46364,
#46365,#46366,#46367,#46368,#46369,#46370,#46371,#46372,#46373,#46374,#46375,
#46376,#46377,#46378,#46379,#46380,#46381,#46382),.UNSPECIFIED.,.F.,.F.)
B_SPLINE_CURVE_WITH_KNOTS((6,1,1,1,1,1,1,1,1,1,1,1,1,1,1,1,1,1,1,1,1,1,
1,1,1,1,1,1,1,1,1,1,1,1,1,1,1,1,1,1,1,1,1,1,1,1,1,1,1,1,1,1,1,1,1,1,1,1,
1,1,1,1,1,1,1,6),(-1.,-0.984615384615383,-0.969230769230768,-0.953846153846152,
-0.938461538461537,-0.923076923076922,-0.907692307692306,-0.892307692307691,
-0.876923076923076,-0.86153846153846,-0.846153846153845,-0.83076923076923,
-0.815384615384614,-0.799999999999999,-0.784615384615384,-0.769230769230768,
-0.753846153846153,-0.738461538461538,-0.723076923076922,-0.707692307692307,
-0.692307692307692,-0.676923076923076,-0.661538461538461,-0.646153846153846,
-0.63076923076923,-0.615384615384615,-0.6,-0.584615384615384,-0.569230769230769,
-0.553846153846154,-0.538461538461538,-0.523076923076923,-0.507692307692308,
-0.492307692307692,-0.476923076923077,-0.461538461538462,-0.446153846153846,
-0.430769230769231,-0.415384615384615,-0.4,-0.384615384615385,-0.369230769230769,
-0.353846153846154,-0.338461538461538,-0.323076923076923,-0.307692307692308,
-0.292307692307692,-0.276923076923077,-0.261538461538462,-0.246153846153846,
-0.230769230769231,-0.215384615384615,-0.2,-0.184615384615385,-0.169230769230769,
-0.153846153846154,-0.138461538461538,-0.123076923076923,-0.107692307692308,
-0.0923076923076923,-0.0769230769230769,-0.0615384615384615,-0.0461538461538462,
-0.0307692307692308,-0.0153846153846154,-0.0057718433744903),
 .UNSPECIFIED.)
CURVE()
GEOMETRIC_REPRESENTATION_ITEM()
RATIONAL_B_SPLINE_CURVE((1.,1.,1.,1.,1.,1.,1.,1.,1.,1.,1.,1.,1.,1.,1.,1.,
1.,1.,1.,1.,1.,1.,1.,1.,1.,1.,1.,1.,1.,1.,1.,1.,1.,1.,1.,1.,1.,1.,1.,1.,
1.,1.,1.,1.,1.,1.,1.,1.,1.,1.,1.,1.,1.,1.,1.,1.,1.,1.,1.,1.,1.,1.,1.,1.,
1.,1.,1.,1.,1.,1.))
REPRESENTATION_ITEM('')
);
#338=(
BOUNDED_CURVE()
B_SPLINE_CURVE(5,(#46533,#46534,#46535,#46536,#46537,#46538,#46539,#46540,
#46541,#46542,#46543,#46544,#46545,#46546,#46547,#46548,#46549,#46550,#46551,
#46552,#46553,#46554,#46555,#46556,#46557,#46558,#46559,#46560,#46561,#46562,
#46563,#46564,#46565,#46566,#46567,#46568,#46569,#46570,#46571,#46572,#46573,
#46574,#46575,#46576,#46577,#46578,#46579,#46580,#46581,#46582,#46583,#46584,
#46585,#46586,#46587,#46588,#46589,#46590,#46591,#46592,#46593,#46594,#46595,
#46596,#46597,#46598,#46599,#46600,#46601,#46602),.UNSPECIFIED.,.F.,.F.)
B_SPLINE_CURVE_WITH_KNOTS((6,1,1,1,1,1,1,1,1,1,1,1,1,1,1,1,1,1,1,1,1,1,
1,1,1,1,1,1,1,1,1,1,1,1,1,1,1,1,1,1,1,1,1,1,1,1,1,1,1,1,1,1,1,1,1,1,1,1,
1,1,1,1,1,1,1,6),(-0.994228156739712,-0.984615384615383,-0.969230769230768,
-0.953846153846152,-0.938461538461537,-0.923076923076922,-0.907692307692306,
-0.892307692307691,-0.876923076923076,-0.86153846153846,-0.846153846153845,
-0.83076923076923,-0.815384615384614,-0.799999999999999,-0.784615384615384,
-0.769230769230768,-0.753846153846153,-0.738461538461538,-0.723076923076922,
-0.707692307692307,-0.692307692307692,-0.676923076923076,-0.661538461538461,
-0.646153846153846,-0.63076923076923,-0.615384615384615,-0.6,-0.584615384615384,
-0.569230769230769,-0.553846153846154,-0.538461538461538,-0.523076923076923,
-0.507692307692308,-0.492307692307692,-0.476923076923077,-0.461538461538462,
-0.446153846153846,-0.430769230769231,-0.415384615384615,-0.4,-0.384615384615385,
-0.369230769230769,-0.353846153846154,-0.338461538461538,-0.323076923076923,
-0.307692307692308,-0.292307692307692,-0.276923076923077,-0.261538461538462,
-0.246153846153846,-0.230769230769231,-0.215384615384615,-0.2,-0.184615384615385,
-0.169230769230769,-0.153846153846154,-0.138461538461538,-0.123076923076923,
-0.107692307692308,-0.0923076923076923,-0.0769230769230769,-0.0615384615384615,
-0.0461538461538462,-0.0307692307692308,-0.0153846153846154,0.),
 .UNSPECIFIED.)
CURVE()
GEOMETRIC_REPRESENTATION_ITEM()
RATIONAL_B_SPLINE_CURVE((1.,1.,1.,1.,1.,1.,1.,1.,1.,1.,1.,1.,1.,1.,1.,1.,
1.,1.,1.,1.,1.,1.,1.,1.,1.,1.,1.,1.,1.,1.,1.,1.,1.,1.,1.,1.,1.,1.,1.,1.,
1.,1.,1.,1.,1.,1.,1.,1.,1.,1.,1.,1.,1.,1.,1.,1.,1.,1.,1.,1.,1.,1.,1.,1.,
1.,1.,1.,1.,1.,1.))
REPRESENTATION_ITEM('')
);
#339=(
BOUNDED_CURVE()
B_SPLINE_CURVE(5,(#46755,#46756,#46757,#46758,#46759,#46760,#46761,#46762,
#46763,#46764,#46765,#46766,#46767,#46768,#46769,#46770,#46771,#46772,#46773,
#46774,#46775,#46776,#46777,#46778,#46779,#46780,#46781,#46782,#46783,#46784,
#46785,#46786,#46787,#46788,#46789,#46790,#46791,#46792,#46793,#46794,#46795,
#46796,#46797,#46798,#46799,#46800,#46801,#46802,#46803,#46804,#46805,#46806,
#46807,#46808,#46809,#46810,#46811,#46812,#46813,#46814,#46815,#46816,#46817,
#46818,#46819,#46820,#46821,#46822,#46823,#46824),.UNSPECIFIED.,.F.,.F.)
B_SPLINE_CURVE_WITH_KNOTS((6,1,1,1,1,1,1,1,1,1,1,1,1,1,1,1,1,1,1,1,1,1,
1,1,1,1,1,1,1,1,1,1,1,1,1,1,1,1,1,1,1,1,1,1,1,1,1,1,1,1,1,1,1,1,1,1,1,1,
1,1,1,1,1,1,1,6),(-1.,-0.984615384615383,-0.969230769230768,-0.953846153846152,
-0.938461538461537,-0.923076923076922,-0.907692307692306,-0.892307692307691,
-0.876923076923076,-0.86153846153846,-0.846153846153845,-0.83076923076923,
-0.815384615384614,-0.799999999999999,-0.784615384615384,-0.769230769230768,
-0.753846153846153,-0.738461538461538,-0.723076923076922,-0.707692307692307,
-0.692307692307692,-0.676923076923076,-0.661538461538461,-0.646153846153846,
-0.63076923076923,-0.615384615384615,-0.6,-0.584615384615384,-0.569230769230769,
-0.553846153846154,-0.538461538461538,-0.523076923076923,-0.507692307692308,
-0.492307692307692,-0.476923076923077,-0.461538461538462,-0.446153846153846,
-0.430769230769231,-0.415384615384615,-0.4,-0.384615384615385,-0.369230769230769,
-0.353846153846154,-0.338461538461538,-0.323076923076923,-0.307692307692308,
-0.292307692307692,-0.276923076923077,-0.261538461538462,-0.246153846153846,
-0.230769230769231,-0.215384615384615,-0.2,-0.184615384615385,-0.169230769230769,
-0.153846153846154,-0.138461538461538,-0.123076923076923,-0.107692307692308,
-0.0923076923076923,-0.0769230769230769,-0.0615384615384615,-0.0461538461538462,
-0.0307692307692308,-0.0153846153846154,-0.0057718433745291),
 .UNSPECIFIED.)
CURVE()
GEOMETRIC_REPRESENTATION_ITEM()
RATIONAL_B_SPLINE_CURVE((1.,1.,1.,1.,1.,1.,1.,1.,1.,1.,1.,1.,1.,1.,1.,1.,
1.,1.,1.,1.,1.,1.,1.,1.,1.,1.,1.,1.,1.,1.,1.,1.,1.,1.,1.,1.,1.,1.,1.,1.,
1.,1.,1.,1.,1.,1.,1.,1.,1.,1.,1.,1.,1.,1.,1.,1.,1.,1.,1.,1.,1.,1.,1.,1.,
1.,1.,1.,1.,1.,1.))
REPRESENTATION_ITEM('')
);
#340=(
BOUNDED_CURVE()
B_SPLINE_CURVE(5,(#46975,#46976,#46977,#46978,#46979,#46980,#46981,#46982,
#46983,#46984,#46985,#46986,#46987,#46988,#46989,#46990,#46991,#46992,#46993,
#46994,#46995,#46996,#46997,#46998,#46999,#47000,#47001,#47002,#47003,#47004,
#47005,#47006,#47007,#47008,#47009,#47010,#47011,#47012,#47013,#47014,#47015,
#47016,#47017,#47018,#47019,#47020,#47021,#47022,#47023,#47024,#47025,#47026,
#47027,#47028,#47029,#47030,#47031,#47032,#47033,#47034,#47035,#47036,#47037,
#47038,#47039,#47040,#47041,#47042,#47043,#47044),.UNSPECIFIED.,.F.,.F.)
B_SPLINE_CURVE_WITH_KNOTS((6,1,1,1,1,1,1,1,1,1,1,1,1,1,1,1,1,1,1,1,1,1,
1,1,1,1,1,1,1,1,1,1,1,1,1,1,1,1,1,1,1,1,1,1,1,1,1,1,1,1,1,1,1,1,1,1,1,1,
1,1,1,1,1,1,1,6),(-0.994228156739695,-0.984615384615383,-0.969230769230768,
-0.953846153846152,-0.938461538461537,-0.923076923076922,-0.907692307692306,
-0.892307692307691,-0.876923076923076,-0.86153846153846,-0.846153846153845,
-0.83076923076923,-0.815384615384614,-0.799999999999999,-0.784615384615384,
-0.769230769230768,-0.753846153846153,-0.738461538461538,-0.723076923076922,
-0.707692307692307,-0.692307692307692,-0.676923076923076,-0.661538461538461,
-0.646153846153846,-0.63076923076923,-0.615384615384615,-0.6,-0.584615384615384,
-0.569230769230769,-0.553846153846154,-0.538461538461538,-0.523076923076923,
-0.507692307692308,-0.492307692307692,-0.476923076923077,-0.461538461538462,
-0.446153846153846,-0.430769230769231,-0.415384615384615,-0.4,-0.384615384615385,
-0.369230769230769,-0.353846153846154,-0.338461538461538,-0.323076923076923,
-0.307692307692308,-0.292307692307692,-0.276923076923077,-0.261538461538462,
-0.246153846153846,-0.230769230769231,-0.215384615384615,-0.2,-0.184615384615385,
-0.169230769230769,-0.153846153846154,-0.138461538461538,-0.123076923076923,
-0.107692307692308,-0.0923076923076923,-0.0769230769230769,-0.0615384615384615,
-0.0461538461538462,-0.0307692307692308,-0.0153846153846154,0.),
 .UNSPECIFIED.)
CURVE()
GEOMETRIC_REPRESENTATION_ITEM()
RATIONAL_B_SPLINE_CURVE((1.,1.,1.,1.,1.,1.,1.,1.,1.,1.,1.,1.,1.,1.,1.,1.,
1.,1.,1.,1.,1.,1.,1.,1.,1.,1.,1.,1.,1.,1.,1.,1.,1.,1.,1.,1.,1.,1.,1.,1.,
1.,1.,1.,1.,1.,1.,1.,1.,1.,1.,1.,1.,1.,1.,1.,1.,1.,1.,1.,1.,1.,1.,1.,1.,
1.,1.,1.,1.,1.,1.))
REPRESENTATION_ITEM('')
);
#341=(
BOUNDED_CURVE()
B_SPLINE_CURVE(5,(#47197,#47198,#47199,#47200,#47201,#47202,#47203,#47204,
#47205,#47206,#47207,#47208,#47209,#47210,#47211,#47212,#47213,#47214,#47215,
#47216,#47217,#47218,#47219,#47220,#47221,#47222,#47223,#47224,#47225,#47226,
#47227,#47228,#47229,#47230,#47231,#47232,#47233,#47234,#47235,#47236,#47237,
#47238,#47239,#47240,#47241,#47242,#47243,#47244,#47245,#47246,#47247,#47248,
#47249,#47250,#47251,#47252,#47253,#47254,#47255,#47256,#47257,#47258,#47259,
#47260,#47261,#47262,#47263,#47264,#47265,#47266),.UNSPECIFIED.,.F.,.F.)
B_SPLINE_CURVE_WITH_KNOTS((6,1,1,1,1,1,1,1,1,1,1,1,1,1,1,1,1,1,1,1,1,1,
1,1,1,1,1,1,1,1,1,1,1,1,1,1,1,1,1,1,1,1,1,1,1,1,1,1,1,1,1,1,1,1,1,1,1,1,
1,1,1,1,1,1,1,6),(-1.,-0.984615384615383,-0.969230769230768,-0.953846153846152,
-0.938461538461537,-0.923076923076922,-0.907692307692306,-0.892307692307691,
-0.876923076923076,-0.86153846153846,-0.846153846153845,-0.83076923076923,
-0.815384615384614,-0.799999999999999,-0.784615384615384,-0.769230769230768,
-0.753846153846153,-0.738461538461538,-0.723076923076922,-0.707692307692307,
-0.692307692307692,-0.676923076923076,-0.661538461538461,-0.646153846153846,
-0.63076923076923,-0.615384615384615,-0.6,-0.584615384615384,-0.569230769230769,
-0.553846153846154,-0.538461538461538,-0.523076923076923,-0.507692307692308,
-0.492307692307692,-0.476923076923077,-0.461538461538462,-0.446153846153846,
-0.430769230769231,-0.415384615384615,-0.4,-0.384615384615385,-0.369230769230769,
-0.353846153846154,-0.338461538461538,-0.323076923076923,-0.307692307692308,
-0.292307692307692,-0.276923076923077,-0.261538461538462,-0.246153846153846,
-0.230769230769231,-0.215384615384615,-0.2,-0.184615384615385,-0.169230769230769,
-0.153846153846154,-0.138461538461538,-0.123076923076923,-0.107692307692308,
-0.0923076923076923,-0.0769230769230769,-0.0615384615384615,-0.0461538461538462,
-0.0307692307692308,-0.0153846153846154,-0.00577184337450344),
 .UNSPECIFIED.)
CURVE()
GEOMETRIC_REPRESENTATION_ITEM()
RATIONAL_B_SPLINE_CURVE((1.,1.,1.,1.,1.,1.,1.,1.,1.,1.,1.,1.,1.,1.,1.,1.,
1.,1.,1.,1.,1.,1.,1.,1.,1.,1.,1.,1.,1.,1.,1.,1.,1.,1.,1.,1.,1.,1.,1.,1.,
1.,1.,1.,1.,1.,1.,1.,1.,1.,1.,1.,1.,1.,1.,1.,1.,1.,1.,1.,1.,1.,1.,1.,1.,
1.,1.,1.,1.,1.,1.))
REPRESENTATION_ITEM('')
);
#342=(
BOUNDED_CURVE()
B_SPLINE_CURVE(5,(#47417,#47418,#47419,#47420,#47421,#47422,#47423,#47424,
#47425,#47426,#47427,#47428,#47429,#47430,#47431,#47432,#47433,#47434,#47435,
#47436,#47437,#47438,#47439,#47440,#47441,#47442,#47443,#47444,#47445,#47446,
#47447,#47448,#47449,#47450,#47451,#47452,#47453,#47454,#47455,#47456,#47457,
#47458,#47459,#47460,#47461,#47462,#47463,#47464,#47465,#47466,#47467,#47468,
#47469,#47470,#47471,#47472,#47473,#47474,#47475,#47476,#47477,#47478,#47479,
#47480,#47481,#47482,#47483,#47484,#47485,#47486),.UNSPECIFIED.,.F.,.F.)
B_SPLINE_CURVE_WITH_KNOTS((6,1,1,1,1,1,1,1,1,1,1,1,1,1,1,1,1,1,1,1,1,1,
1,1,1,1,1,1,1,1,1,1,1,1,1,1,1,1,1,1,1,1,1,1,1,1,1,1,1,1,1,1,1,1,1,1,1,1,
1,1,1,1,1,1,1,6),(-0.994228156739669,-0.984615384615383,-0.969230769230768,
-0.953846153846152,-0.938461538461537,-0.923076923076922,-0.907692307692306,
-0.892307692307691,-0.876923076923076,-0.86153846153846,-0.846153846153845,
-0.83076923076923,-0.815384615384614,-0.799999999999999,-0.784615384615384,
-0.769230769230768,-0.753846153846153,-0.738461538461538,-0.723076923076922,
-0.707692307692307,-0.692307692307692,-0.676923076923076,-0.661538461538461,
-0.646153846153846,-0.63076923076923,-0.615384615384615,-0.6,-0.584615384615384,
-0.569230769230769,-0.553846153846154,-0.538461538461538,-0.523076923076923,
-0.507692307692308,-0.492307692307692,-0.476923076923077,-0.461538461538462,
-0.446153846153846,-0.430769230769231,-0.415384615384615,-0.4,-0.384615384615385,
-0.369230769230769,-0.353846153846154,-0.338461538461538,-0.323076923076923,
-0.307692307692308,-0.292307692307692,-0.276923076923077,-0.261538461538462,
-0.246153846153846,-0.230769230769231,-0.215384615384615,-0.2,-0.184615384615385,
-0.169230769230769,-0.153846153846154,-0.138461538461538,-0.123076923076923,
-0.107692307692308,-0.0923076923076923,-0.0769230769230769,-0.0615384615384615,
-0.0461538461538462,-0.0307692307692308,-0.0153846153846154,0.),
 .UNSPECIFIED.)
CURVE()
GEOMETRIC_REPRESENTATION_ITEM()
RATIONAL_B_SPLINE_CURVE((1.,1.,1.,1.,1.,1.,1.,1.,1.,1.,1.,1.,1.,1.,1.,1.,
1.,1.,1.,1.,1.,1.,1.,1.,1.,1.,1.,1.,1.,1.,1.,1.,1.,1.,1.,1.,1.,1.,1.,1.,
1.,1.,1.,1.,1.,1.,1.,1.,1.,1.,1.,1.,1.,1.,1.,1.,1.,1.,1.,1.,1.,1.,1.,1.,
1.,1.,1.,1.,1.,1.))
REPRESENTATION_ITEM('')
);
#343=(
BOUNDED_CURVE()
B_SPLINE_CURVE(5,(#47639,#47640,#47641,#47642,#47643,#47644,#47645,#47646,
#47647,#47648,#47649,#47650,#47651,#47652,#47653,#47654,#47655,#47656,#47657,
#47658,#47659,#47660,#47661,#47662,#47663,#47664,#47665,#47666,#47667,#47668,
#47669,#47670,#47671,#47672,#47673,#47674,#47675,#47676,#47677,#47678,#47679,
#47680,#47681,#47682,#47683,#47684,#47685,#47686,#47687,#47688,#47689,#47690,
#47691,#47692,#47693,#47694,#47695,#47696,#47697,#47698,#47699,#47700,#47701,
#47702,#47703,#47704,#47705,#47706,#47707,#47708),.UNSPECIFIED.,.F.,.F.)
B_SPLINE_CURVE_WITH_KNOTS((6,1,1,1,1,1,1,1,1,1,1,1,1,1,1,1,1,1,1,1,1,1,
1,1,1,1,1,1,1,1,1,1,1,1,1,1,1,1,1,1,1,1,1,1,1,1,1,1,1,1,1,1,1,1,1,1,1,1,
1,1,1,1,1,1,1,6),(-1.,-0.984615384615383,-0.969230769230768,-0.953846153846152,
-0.938461538461537,-0.923076923076922,-0.907692307692306,-0.892307692307691,
-0.876923076923076,-0.86153846153846,-0.846153846153845,-0.83076923076923,
-0.815384615384614,-0.799999999999999,-0.784615384615384,-0.769230769230768,
-0.753846153846153,-0.738461538461538,-0.723076923076922,-0.707692307692307,
-0.692307692307692,-0.676923076923076,-0.661538461538461,-0.646153846153846,
-0.63076923076923,-0.615384615384615,-0.6,-0.584615384615384,-0.569230769230769,
-0.553846153846154,-0.538461538461538,-0.523076923076923,-0.507692307692308,
-0.492307692307692,-0.476923076923077,-0.461538461538462,-0.446153846153846,
-0.430769230769231,-0.415384615384615,-0.4,-0.384615384615385,-0.369230769230769,
-0.353846153846154,-0.338461538461538,-0.323076923076923,-0.307692307692308,
-0.292307692307692,-0.276923076923077,-0.261538461538462,-0.246153846153846,
-0.230769230769231,-0.215384615384615,-0.2,-0.184615384615385,-0.169230769230769,
-0.153846153846154,-0.138461538461538,-0.123076923076923,-0.107692307692308,
-0.0923076923076923,-0.0769230769230769,-0.0615384615384615,-0.0461538461538462,
-0.0307692307692308,-0.0153846153846154,-0.00577184337450876),
 .UNSPECIFIED.)
CURVE()
GEOMETRIC_REPRESENTATION_ITEM()
RATIONAL_B_SPLINE_CURVE((1.,1.,1.,1.,1.,1.,1.,1.,1.,1.,1.,1.,1.,1.,1.,1.,
1.,1.,1.,1.,1.,1.,1.,1.,1.,1.,1.,1.,1.,1.,1.,1.,1.,1.,1.,1.,1.,1.,1.,1.,
1.,1.,1.,1.,1.,1.,1.,1.,1.,1.,1.,1.,1.,1.,1.,1.,1.,1.,1.,1.,1.,1.,1.,1.,
1.,1.,1.,1.,1.,1.))
REPRESENTATION_ITEM('')
);
#344=(
BOUNDED_CURVE()
B_SPLINE_CURVE(5,(#47859,#47860,#47861,#47862,#47863,#47864,#47865,#47866,
#47867,#47868,#47869,#47870,#47871,#47872,#47873,#47874,#47875,#47876,#47877,
#47878,#47879,#47880,#47881,#47882,#47883,#47884,#47885,#47886,#47887,#47888,
#47889,#47890,#47891,#47892,#47893,#47894,#47895,#47896,#47897,#47898,#47899,
#47900,#47901,#47902,#47903,#47904,#47905,#47906,#47907,#47908,#47909,#47910,
#47911,#47912,#47913,#47914,#47915,#47916,#47917,#47918,#47919,#47920,#47921,
#47922,#47923,#47924,#47925,#47926,#47927,#47928),.UNSPECIFIED.,.F.,.F.)
B_SPLINE_CURVE_WITH_KNOTS((6,1,1,1,1,1,1,1,1,1,1,1,1,1,1,1,1,1,1,1,1,1,
1,1,1,1,1,1,1,1,1,1,1,1,1,1,1,1,1,1,1,1,1,1,1,1,1,1,1,1,1,1,1,1,1,1,1,1,
1,1,1,1,1,1,1,6),(-0.99422815673966,-0.984615384615383,-0.969230769230768,
-0.953846153846152,-0.938461538461537,-0.923076923076922,-0.907692307692306,
-0.892307692307691,-0.876923076923076,-0.86153846153846,-0.846153846153845,
-0.83076923076923,-0.815384615384614,-0.799999999999999,-0.784615384615384,
-0.769230769230768,-0.753846153846153,-0.738461538461538,-0.723076923076922,
-0.707692307692307,-0.692307692307692,-0.676923076923076,-0.661538461538461,
-0.646153846153846,-0.63076923076923,-0.615384615384615,-0.6,-0.584615384615384,
-0.569230769230769,-0.553846153846154,-0.538461538461538,-0.523076923076923,
-0.507692307692308,-0.492307692307692,-0.476923076923077,-0.461538461538462,
-0.446153846153846,-0.430769230769231,-0.415384615384615,-0.4,-0.384615384615385,
-0.369230769230769,-0.353846153846154,-0.338461538461538,-0.323076923076923,
-0.307692307692308,-0.292307692307692,-0.276923076923077,-0.261538461538462,
-0.246153846153846,-0.230769230769231,-0.215384615384615,-0.2,-0.184615384615385,
-0.169230769230769,-0.153846153846154,-0.138461538461538,-0.123076923076923,
-0.107692307692308,-0.0923076923076923,-0.0769230769230769,-0.0615384615384615,
-0.0461538461538462,-0.0307692307692308,-0.0153846153846154,0.),
 .UNSPECIFIED.)
CURVE()
GEOMETRIC_REPRESENTATION_ITEM()
RATIONAL_B_SPLINE_CURVE((1.,1.,1.,1.,1.,1.,1.,1.,1.,1.,1.,1.,1.,1.,1.,1.,
1.,1.,1.,1.,1.,1.,1.,1.,1.,1.,1.,1.,1.,1.,1.,1.,1.,1.,1.,1.,1.,1.,1.,1.,
1.,1.,1.,1.,1.,1.,1.,1.,1.,1.,1.,1.,1.,1.,1.,1.,1.,1.,1.,1.,1.,1.,1.,1.,
1.,1.,1.,1.,1.,1.))
REPRESENTATION_ITEM('')
);
#345=(
BOUNDED_CURVE()
B_SPLINE_CURVE(5,(#48081,#48082,#48083,#48084,#48085,#48086,#48087,#48088,
#48089,#48090,#48091,#48092,#48093,#48094,#48095,#48096,#48097,#48098,#48099,
#48100,#48101,#48102,#48103,#48104,#48105,#48106,#48107,#48108,#48109,#48110,
#48111,#48112,#48113,#48114,#48115,#48116,#48117,#48118,#48119,#48120,#48121,
#48122,#48123,#48124,#48125,#48126,#48127,#48128,#48129,#48130,#48131,#48132,
#48133,#48134,#48135,#48136,#48137,#48138,#48139,#48140,#48141,#48142,#48143,
#48144,#48145,#48146,#48147,#48148,#48149,#48150),.UNSPECIFIED.,.F.,.F.)
B_SPLINE_CURVE_WITH_KNOTS((6,1,1,1,1,1,1,1,1,1,1,1,1,1,1,1,1,1,1,1,1,1,
1,1,1,1,1,1,1,1,1,1,1,1,1,1,1,1,1,1,1,1,1,1,1,1,1,1,1,1,1,1,1,1,1,1,1,1,
1,1,1,1,1,1,1,6),(-1.,-0.984615384615383,-0.969230769230768,-0.953846153846152,
-0.938461538461537,-0.923076923076922,-0.907692307692306,-0.892307692307691,
-0.876923076923076,-0.86153846153846,-0.846153846153845,-0.83076923076923,
-0.815384615384614,-0.799999999999999,-0.784615384615384,-0.769230769230768,
-0.753846153846153,-0.738461538461538,-0.723076923076922,-0.707692307692307,
-0.692307692307692,-0.676923076923076,-0.661538461538461,-0.646153846153846,
-0.63076923076923,-0.615384615384615,-0.6,-0.584615384615384,-0.569230769230769,
-0.553846153846154,-0.538461538461538,-0.523076923076923,-0.507692307692308,
-0.492307692307692,-0.476923076923077,-0.461538461538462,-0.446153846153846,
-0.430769230769231,-0.415384615384615,-0.4,-0.384615384615385,-0.369230769230769,
-0.353846153846154,-0.338461538461538,-0.323076923076923,-0.307692307692308,
-0.292307692307692,-0.276923076923077,-0.261538461538462,-0.246153846153846,
-0.230769230769231,-0.215384615384615,-0.2,-0.184615384615385,-0.169230769230769,
-0.153846153846154,-0.138461538461538,-0.123076923076923,-0.107692307692308,
-0.0923076923076923,-0.0769230769230769,-0.0615384615384615,-0.0461538461538462,
-0.0307692307692308,-0.0153846153846154,-0.00577184337451051),
 .UNSPECIFIED.)
CURVE()
GEOMETRIC_REPRESENTATION_ITEM()
RATIONAL_B_SPLINE_CURVE((1.,1.,1.,1.,1.,1.,1.,1.,1.,1.,1.,1.,1.,1.,1.,1.,
1.,1.,1.,1.,1.,1.,1.,1.,1.,1.,1.,1.,1.,1.,1.,1.,1.,1.,1.,1.,1.,1.,1.,1.,
1.,1.,1.,1.,1.,1.,1.,1.,1.,1.,1.,1.,1.,1.,1.,1.,1.,1.,1.,1.,1.,1.,1.,1.,
1.,1.,1.,1.,1.,1.))
REPRESENTATION_ITEM('')
);
#346=(
BOUNDED_CURVE()
B_SPLINE_CURVE(5,(#48301,#48302,#48303,#48304,#48305,#48306,#48307,#48308,
#48309,#48310,#48311,#48312,#48313,#48314,#48315,#48316,#48317,#48318,#48319,
#48320,#48321,#48322,#48323,#48324,#48325,#48326,#48327,#48328,#48329,#48330,
#48331,#48332,#48333,#48334,#48335,#48336,#48337,#48338,#48339,#48340,#48341,
#48342,#48343,#48344,#48345,#48346,#48347,#48348,#48349,#48350,#48351,#48352,
#48353,#48354,#48355,#48356,#48357,#48358,#48359,#48360,#48361,#48362,#48363,
#48364,#48365,#48366,#48367,#48368,#48369,#48370),.UNSPECIFIED.,.F.,.F.)
B_SPLINE_CURVE_WITH_KNOTS((6,1,1,1,1,1,1,1,1,1,1,1,1,1,1,1,1,1,1,1,1,1,
1,1,1,1,1,1,1,1,1,1,1,1,1,1,1,1,1,1,1,1,1,1,1,1,1,1,1,1,1,1,1,1,1,1,1,1,
1,1,1,1,1,1,1,6),(-0.994228156739678,-0.984615384615383,-0.969230769230768,
-0.953846153846152,-0.938461538461537,-0.923076923076922,-0.907692307692306,
-0.892307692307691,-0.876923076923076,-0.86153846153846,-0.846153846153845,
-0.83076923076923,-0.815384615384614,-0.799999999999999,-0.784615384615384,
-0.769230769230768,-0.753846153846153,-0.738461538461538,-0.723076923076922,
-0.707692307692307,-0.692307692307692,-0.676923076923076,-0.661538461538461,
-0.646153846153846,-0.63076923076923,-0.615384615384615,-0.6,-0.584615384615384,
-0.569230769230769,-0.553846153846154,-0.538461538461538,-0.523076923076923,
-0.507692307692308,-0.492307692307692,-0.476923076923077,-0.461538461538462,
-0.446153846153846,-0.430769230769231,-0.415384615384615,-0.4,-0.384615384615385,
-0.369230769230769,-0.353846153846154,-0.338461538461538,-0.323076923076923,
-0.307692307692308,-0.292307692307692,-0.276923076923077,-0.261538461538462,
-0.246153846153846,-0.230769230769231,-0.215384615384615,-0.2,-0.184615384615385,
-0.169230769230769,-0.153846153846154,-0.138461538461538,-0.123076923076923,
-0.107692307692308,-0.0923076923076923,-0.0769230769230769,-0.0615384615384615,
-0.0461538461538462,-0.0307692307692308,-0.0153846153846154,0.),
 .UNSPECIFIED.)
CURVE()
GEOMETRIC_REPRESENTATION_ITEM()
RATIONAL_B_SPLINE_CURVE((1.,1.,1.,1.,1.,1.,1.,1.,1.,1.,1.,1.,1.,1.,1.,1.,
1.,1.,1.,1.,1.,1.,1.,1.,1.,1.,1.,1.,1.,1.,1.,1.,1.,1.,1.,1.,1.,1.,1.,1.,
1.,1.,1.,1.,1.,1.,1.,1.,1.,1.,1.,1.,1.,1.,1.,1.,1.,1.,1.,1.,1.,1.,1.,1.,
1.,1.,1.,1.,1.,1.))
REPRESENTATION_ITEM('')
);
#347=(
BOUNDED_CURVE()
B_SPLINE_CURVE(5,(#48523,#48524,#48525,#48526,#48527,#48528,#48529,#48530,
#48531,#48532,#48533,#48534,#48535,#48536,#48537,#48538,#48539,#48540,#48541,
#48542,#48543,#48544,#48545,#48546,#48547,#48548,#48549,#48550,#48551,#48552,
#48553,#48554,#48555,#48556,#48557,#48558,#48559,#48560,#48561,#48562,#48563,
#48564,#48565,#48566,#48567,#48568,#48569,#48570,#48571,#48572,#48573,#48574,
#48575,#48576,#48577,#48578,#48579,#48580,#48581,#48582,#48583,#48584,#48585,
#48586,#48587,#48588,#48589,#48590,#48591,#48592),.UNSPECIFIED.,.F.,.F.)
B_SPLINE_CURVE_WITH_KNOTS((6,1,1,1,1,1,1,1,1,1,1,1,1,1,1,1,1,1,1,1,1,1,
1,1,1,1,1,1,1,1,1,1,1,1,1,1,1,1,1,1,1,1,1,1,1,1,1,1,1,1,1,1,1,1,1,1,1,1,
1,1,1,1,1,1,1,6),(-1.,-0.984615384615383,-0.969230769230768,-0.953846153846152,
-0.938461538461537,-0.923076923076922,-0.907692307692306,-0.892307692307691,
-0.876923076923076,-0.86153846153846,-0.846153846153845,-0.83076923076923,
-0.815384615384614,-0.799999999999999,-0.784615384615384,-0.769230769230768,
-0.753846153846153,-0.738461538461538,-0.723076923076922,-0.707692307692307,
-0.692307692307692,-0.676923076923076,-0.661538461538461,-0.646153846153846,
-0.63076923076923,-0.615384615384615,-0.6,-0.584615384615384,-0.569230769230769,
-0.553846153846154,-0.538461538461538,-0.523076923076923,-0.507692307692308,
-0.492307692307692,-0.476923076923077,-0.461538461538462,-0.446153846153846,
-0.430769230769231,-0.415384615384615,-0.4,-0.384615384615385,-0.369230769230769,
-0.353846153846154,-0.338461538461538,-0.323076923076923,-0.307692307692308,
-0.292307692307692,-0.276923076923077,-0.261538461538462,-0.246153846153846,
-0.230769230769231,-0.215384615384615,-0.2,-0.184615384615385,-0.169230769230769,
-0.153846153846154,-0.138461538461538,-0.123076923076923,-0.107692307692308,
-0.0923076923076923,-0.0769230769230769,-0.0615384615384615,-0.0461538461538462,
-0.0307692307692308,-0.0153846153846154,-0.0057718433745179),
 .UNSPECIFIED.)
CURVE()
GEOMETRIC_REPRESENTATION_ITEM()
RATIONAL_B_SPLINE_CURVE((1.,1.,1.,1.,1.,1.,1.,1.,1.,1.,1.,1.,1.,1.,1.,1.,
1.,1.,1.,1.,1.,1.,1.,1.,1.,1.,1.,1.,1.,1.,1.,1.,1.,1.,1.,1.,1.,1.,1.,1.,
1.,1.,1.,1.,1.,1.,1.,1.,1.,1.,1.,1.,1.,1.,1.,1.,1.,1.,1.,1.,1.,1.,1.,1.,
1.,1.,1.,1.,1.,1.))
REPRESENTATION_ITEM('')
);
#348=(
BOUNDED_CURVE()
B_SPLINE_CURVE(5,(#48743,#48744,#48745,#48746,#48747,#48748,#48749,#48750,
#48751,#48752,#48753,#48754,#48755,#48756,#48757,#48758,#48759,#48760,#48761,
#48762,#48763,#48764,#48765,#48766,#48767,#48768,#48769,#48770,#48771,#48772,
#48773,#48774,#48775,#48776,#48777,#48778,#48779,#48780,#48781,#48782,#48783,
#48784,#48785,#48786,#48787,#48788,#48789,#48790,#48791,#48792,#48793,#48794,
#48795,#48796,#48797,#48798,#48799,#48800,#48801,#48802,#48803,#48804,#48805,
#48806,#48807,#48808,#48809,#48810,#48811,#48812),.UNSPECIFIED.,.F.,.F.)
B_SPLINE_CURVE_WITH_KNOTS((6,1,1,1,1,1,1,1,1,1,1,1,1,1,1,1,1,1,1,1,1,1,
1,1,1,1,1,1,1,1,1,1,1,1,1,1,1,1,1,1,1,1,1,1,1,1,1,1,1,1,1,1,1,1,1,1,1,1,
1,1,1,1,1,1,1,6),(-0.99422815673967,-0.984615384615383,-0.969230769230768,
-0.953846153846152,-0.938461538461537,-0.923076923076922,-0.907692307692306,
-0.892307692307691,-0.876923076923076,-0.86153846153846,-0.846153846153845,
-0.83076923076923,-0.815384615384614,-0.799999999999999,-0.784615384615384,
-0.769230769230768,-0.753846153846153,-0.738461538461538,-0.723076923076922,
-0.707692307692307,-0.692307692307692,-0.676923076923076,-0.661538461538461,
-0.646153846153846,-0.63076923076923,-0.615384615384615,-0.6,-0.584615384615384,
-0.569230769230769,-0.553846153846154,-0.538461538461538,-0.523076923076923,
-0.507692307692308,-0.492307692307692,-0.476923076923077,-0.461538461538462,
-0.446153846153846,-0.430769230769231,-0.415384615384615,-0.4,-0.384615384615385,
-0.369230769230769,-0.353846153846154,-0.338461538461538,-0.323076923076923,
-0.307692307692308,-0.292307692307692,-0.276923076923077,-0.261538461538462,
-0.246153846153846,-0.230769230769231,-0.215384615384615,-0.2,-0.184615384615385,
-0.169230769230769,-0.153846153846154,-0.138461538461538,-0.123076923076923,
-0.107692307692308,-0.0923076923076923,-0.0769230769230769,-0.0615384615384615,
-0.0461538461538462,-0.0307692307692308,-0.0153846153846154,0.),
 .UNSPECIFIED.)
CURVE()
GEOMETRIC_REPRESENTATION_ITEM()
RATIONAL_B_SPLINE_CURVE((1.,1.,1.,1.,1.,1.,1.,1.,1.,1.,1.,1.,1.,1.,1.,1.,
1.,1.,1.,1.,1.,1.,1.,1.,1.,1.,1.,1.,1.,1.,1.,1.,1.,1.,1.,1.,1.,1.,1.,1.,
1.,1.,1.,1.,1.,1.,1.,1.,1.,1.,1.,1.,1.,1.,1.,1.,1.,1.,1.,1.,1.,1.,1.,1.,
1.,1.,1.,1.,1.,1.))
REPRESENTATION_ITEM('')
);
#349=(
BOUNDED_CURVE()
B_SPLINE_CURVE(5,(#48965,#48966,#48967,#48968,#48969,#48970,#48971,#48972,
#48973,#48974,#48975,#48976,#48977,#48978,#48979,#48980,#48981,#48982,#48983,
#48984,#48985,#48986,#48987,#48988,#48989,#48990,#48991,#48992,#48993,#48994,
#48995,#48996,#48997,#48998,#48999,#49000,#49001,#49002,#49003,#49004,#49005,
#49006,#49007,#49008,#49009,#49010,#49011,#49012,#49013,#49014,#49015,#49016,
#49017,#49018,#49019,#49020,#49021,#49022,#49023,#49024,#49025,#49026,#49027,
#49028,#49029,#49030,#49031,#49032,#49033,#49034),.UNSPECIFIED.,.F.,.F.)
B_SPLINE_CURVE_WITH_KNOTS((6,1,1,1,1,1,1,1,1,1,1,1,1,1,1,1,1,1,1,1,1,1,
1,1,1,1,1,1,1,1,1,1,1,1,1,1,1,1,1,1,1,1,1,1,1,1,1,1,1,1,1,1,1,1,1,1,1,1,
1,1,1,1,1,1,1,6),(-1.,-0.984615384615383,-0.969230769230768,-0.953846153846152,
-0.938461538461537,-0.923076923076922,-0.907692307692306,-0.892307692307691,
-0.876923076923076,-0.86153846153846,-0.846153846153845,-0.83076923076923,
-0.815384615384614,-0.799999999999999,-0.784615384615384,-0.769230769230768,
-0.753846153846153,-0.738461538461538,-0.723076923076922,-0.707692307692307,
-0.692307692307692,-0.676923076923076,-0.661538461538461,-0.646153846153846,
-0.63076923076923,-0.615384615384615,-0.6,-0.584615384615384,-0.569230769230769,
-0.553846153846154,-0.538461538461538,-0.523076923076923,-0.507692307692308,
-0.492307692307692,-0.476923076923077,-0.461538461538462,-0.446153846153846,
-0.430769230769231,-0.415384615384615,-0.4,-0.384615384615385,-0.369230769230769,
-0.353846153846154,-0.338461538461538,-0.323076923076923,-0.307692307692308,
-0.292307692307692,-0.276923076923077,-0.261538461538462,-0.246153846153846,
-0.230769230769231,-0.215384615384615,-0.2,-0.184615384615385,-0.169230769230769,
-0.153846153846154,-0.138461538461538,-0.123076923076923,-0.107692307692308,
-0.0923076923076923,-0.0769230769230769,-0.0615384615384615,-0.0461538461538462,
-0.0307692307692308,-0.0153846153846154,-0.00577184337452479),
 .UNSPECIFIED.)
CURVE()
GEOMETRIC_REPRESENTATION_ITEM()
RATIONAL_B_SPLINE_CURVE((1.,1.,1.,1.,1.,1.,1.,1.,1.,1.,1.,1.,1.,1.,1.,1.,
1.,1.,1.,1.,1.,1.,1.,1.,1.,1.,1.,1.,1.,1.,1.,1.,1.,1.,1.,1.,1.,1.,1.,1.,
1.,1.,1.,1.,1.,1.,1.,1.,1.,1.,1.,1.,1.,1.,1.,1.,1.,1.,1.,1.,1.,1.,1.,1.,
1.,1.,1.,1.,1.,1.))
REPRESENTATION_ITEM('')
);
#350=(
BOUNDED_CURVE()
B_SPLINE_CURVE(5,(#49185,#49186,#49187,#49188,#49189,#49190,#49191,#49192,
#49193,#49194,#49195,#49196,#49197,#49198,#49199,#49200,#49201,#49202,#49203,
#49204,#49205,#49206,#49207,#49208,#49209,#49210,#49211,#49212,#49213,#49214,
#49215,#49216,#49217,#49218,#49219,#49220,#49221,#49222,#49223,#49224,#49225,
#49226,#49227,#49228,#49229,#49230,#49231,#49232,#49233,#49234,#49235,#49236,
#49237,#49238,#49239,#49240,#49241,#49242,#49243,#49244,#49245,#49246,#49247,
#49248,#49249,#49250,#49251,#49252,#49253,#49254),.UNSPECIFIED.,.F.,.F.)
B_SPLINE_CURVE_WITH_KNOTS((6,1,1,1,1,1,1,1,1,1,1,1,1,1,1,1,1,1,1,1,1,1,
1,1,1,1,1,1,1,1,1,1,1,1,1,1,1,1,1,1,1,1,1,1,1,1,1,1,1,1,1,1,1,1,1,1,1,1,
1,1,1,1,1,1,1,6),(-0.99422815673967,-0.984615384615383,-0.969230769230768,
-0.953846153846152,-0.938461538461537,-0.923076923076922,-0.907692307692306,
-0.892307692307691,-0.876923076923076,-0.86153846153846,-0.846153846153845,
-0.83076923076923,-0.815384615384614,-0.799999999999999,-0.784615384615384,
-0.769230769230768,-0.753846153846153,-0.738461538461538,-0.723076923076922,
-0.707692307692307,-0.692307692307692,-0.676923076923076,-0.661538461538461,
-0.646153846153846,-0.63076923076923,-0.615384615384615,-0.6,-0.584615384615384,
-0.569230769230769,-0.553846153846154,-0.538461538461538,-0.523076923076923,
-0.507692307692308,-0.492307692307692,-0.476923076923077,-0.461538461538462,
-0.446153846153846,-0.430769230769231,-0.415384615384615,-0.4,-0.384615384615385,
-0.369230769230769,-0.353846153846154,-0.338461538461538,-0.323076923076923,
-0.307692307692308,-0.292307692307692,-0.276923076923077,-0.261538461538462,
-0.246153846153846,-0.230769230769231,-0.215384615384615,-0.2,-0.184615384615385,
-0.169230769230769,-0.153846153846154,-0.138461538461538,-0.123076923076923,
-0.107692307692308,-0.0923076923076923,-0.0769230769230769,-0.0615384615384615,
-0.0461538461538462,-0.0307692307692308,-0.0153846153846154,0.),
 .UNSPECIFIED.)
CURVE()
GEOMETRIC_REPRESENTATION_ITEM()
RATIONAL_B_SPLINE_CURVE((1.,1.,1.,1.,1.,1.,1.,1.,1.,1.,1.,1.,1.,1.,1.,1.,
1.,1.,1.,1.,1.,1.,1.,1.,1.,1.,1.,1.,1.,1.,1.,1.,1.,1.,1.,1.,1.,1.,1.,1.,
1.,1.,1.,1.,1.,1.,1.,1.,1.,1.,1.,1.,1.,1.,1.,1.,1.,1.,1.,1.,1.,1.,1.,1.,
1.,1.,1.,1.,1.,1.))
REPRESENTATION_ITEM('')
);
#351=(
BOUNDED_CURVE()
B_SPLINE_CURVE(5,(#49407,#49408,#49409,#49410,#49411,#49412,#49413,#49414,
#49415,#49416,#49417,#49418,#49419,#49420,#49421,#49422,#49423,#49424,#49425,
#49426,#49427,#49428,#49429,#49430,#49431,#49432,#49433,#49434,#49435,#49436,
#49437,#49438,#49439,#49440,#49441,#49442,#49443,#49444,#49445,#49446,#49447,
#49448,#49449,#49450,#49451,#49452,#49453,#49454,#49455,#49456,#49457,#49458,
#49459,#49460,#49461,#49462,#49463,#49464,#49465,#49466,#49467,#49468,#49469,
#49470,#49471,#49472,#49473,#49474,#49475,#49476),.UNSPECIFIED.,.F.,.F.)
B_SPLINE_CURVE_WITH_KNOTS((6,1,1,1,1,1,1,1,1,1,1,1,1,1,1,1,1,1,1,1,1,1,
1,1,1,1,1,1,1,1,1,1,1,1,1,1,1,1,1,1,1,1,1,1,1,1,1,1,1,1,1,1,1,1,1,1,1,1,
1,1,1,1,1,1,1,6),(-1.,-0.984615384615383,-0.969230769230768,-0.953846153846152,
-0.938461538461537,-0.923076923076922,-0.907692307692306,-0.892307692307691,
-0.876923076923076,-0.86153846153846,-0.846153846153845,-0.83076923076923,
-0.815384615384614,-0.799999999999999,-0.784615384615384,-0.769230769230768,
-0.753846153846153,-0.738461538461538,-0.723076923076922,-0.707692307692307,
-0.692307692307692,-0.676923076923076,-0.661538461538461,-0.646153846153846,
-0.63076923076923,-0.615384615384615,-0.6,-0.584615384615384,-0.569230769230769,
-0.553846153846154,-0.538461538461538,-0.523076923076923,-0.507692307692308,
-0.492307692307692,-0.476923076923077,-0.461538461538462,-0.446153846153846,
-0.430769230769231,-0.415384615384615,-0.4,-0.384615384615385,-0.369230769230769,
-0.353846153846154,-0.338461538461538,-0.323076923076923,-0.307692307692308,
-0.292307692307692,-0.276923076923077,-0.261538461538462,-0.246153846153846,
-0.230769230769231,-0.215384615384615,-0.2,-0.184615384615385,-0.169230769230769,
-0.153846153846154,-0.138461538461538,-0.123076923076923,-0.107692307692308,
-0.0923076923076923,-0.0769230769230769,-0.0615384615384615,-0.0461538461538462,
-0.0307692307692308,-0.0153846153846154,-0.0057718433745009),
 .UNSPECIFIED.)
CURVE()
GEOMETRIC_REPRESENTATION_ITEM()
RATIONAL_B_SPLINE_CURVE((1.,1.,1.,1.,1.,1.,1.,1.,1.,1.,1.,1.,1.,1.,1.,1.,
1.,1.,1.,1.,1.,1.,1.,1.,1.,1.,1.,1.,1.,1.,1.,1.,1.,1.,1.,1.,1.,1.,1.,1.,
1.,1.,1.,1.,1.,1.,1.,1.,1.,1.,1.,1.,1.,1.,1.,1.,1.,1.,1.,1.,1.,1.,1.,1.,
1.,1.,1.,1.,1.,1.))
REPRESENTATION_ITEM('')
);
#352=(
BOUNDED_CURVE()
B_SPLINE_CURVE(5,(#49627,#49628,#49629,#49630,#49631,#49632,#49633,#49634,
#49635,#49636,#49637,#49638,#49639,#49640,#49641,#49642,#49643,#49644,#49645,
#49646,#49647,#49648,#49649,#49650,#49651,#49652,#49653,#49654,#49655,#49656,
#49657,#49658,#49659,#49660,#49661,#49662,#49663,#49664,#49665,#49666,#49667,
#49668,#49669,#49670,#49671,#49672,#49673,#49674,#49675,#49676,#49677,#49678,
#49679,#49680,#49681,#49682,#49683,#49684,#49685,#49686,#49687,#49688,#49689,
#49690,#49691,#49692,#49693,#49694,#49695,#49696),.UNSPECIFIED.,.F.,.F.)
B_SPLINE_CURVE_WITH_KNOTS((6,1,1,1,1,1,1,1,1,1,1,1,1,1,1,1,1,1,1,1,1,1,
1,1,1,1,1,1,1,1,1,1,1,1,1,1,1,1,1,1,1,1,1,1,1,1,1,1,1,1,1,1,1,1,1,1,1,1,
1,1,1,1,1,1,1,6),(-0.99422815673967,-0.984615384615383,-0.969230769230768,
-0.953846153846152,-0.938461538461537,-0.923076923076922,-0.907692307692306,
-0.892307692307691,-0.876923076923076,-0.86153846153846,-0.846153846153845,
-0.83076923076923,-0.815384615384614,-0.799999999999999,-0.784615384615384,
-0.769230769230768,-0.753846153846153,-0.738461538461538,-0.723076923076922,
-0.707692307692307,-0.692307692307692,-0.676923076923076,-0.661538461538461,
-0.646153846153846,-0.63076923076923,-0.615384615384615,-0.6,-0.584615384615384,
-0.569230769230769,-0.553846153846154,-0.538461538461538,-0.523076923076923,
-0.507692307692308,-0.492307692307692,-0.476923076923077,-0.461538461538462,
-0.446153846153846,-0.430769230769231,-0.415384615384615,-0.4,-0.384615384615385,
-0.369230769230769,-0.353846153846154,-0.338461538461538,-0.323076923076923,
-0.307692307692308,-0.292307692307692,-0.276923076923077,-0.261538461538462,
-0.246153846153846,-0.230769230769231,-0.215384615384615,-0.2,-0.184615384615385,
-0.169230769230769,-0.153846153846154,-0.138461538461538,-0.123076923076923,
-0.107692307692308,-0.0923076923076923,-0.0769230769230769,-0.0615384615384615,
-0.0461538461538462,-0.0307692307692308,-0.0153846153846154,0.),
 .UNSPECIFIED.)
CURVE()
GEOMETRIC_REPRESENTATION_ITEM()
RATIONAL_B_SPLINE_CURVE((1.,1.,1.,1.,1.,1.,1.,1.,1.,1.,1.,1.,1.,1.,1.,1.,
1.,1.,1.,1.,1.,1.,1.,1.,1.,1.,1.,1.,1.,1.,1.,1.,1.,1.,1.,1.,1.,1.,1.,1.,
1.,1.,1.,1.,1.,1.,1.,1.,1.,1.,1.,1.,1.,1.,1.,1.,1.,1.,1.,1.,1.,1.,1.,1.,
1.,1.,1.,1.,1.,1.))
REPRESENTATION_ITEM('')
);
#353=(
BOUNDED_CURVE()
B_SPLINE_CURVE(5,(#49849,#49850,#49851,#49852,#49853,#49854,#49855,#49856,
#49857,#49858,#49859,#49860,#49861,#49862,#49863,#49864,#49865,#49866,#49867,
#49868,#49869,#49870,#49871,#49872,#49873,#49874,#49875,#49876,#49877,#49878,
#49879,#49880,#49881,#49882,#49883,#49884,#49885,#49886,#49887,#49888,#49889,
#49890,#49891,#49892,#49893,#49894,#49895,#49896,#49897,#49898,#49899,#49900,
#49901,#49902,#49903,#49904,#49905,#49906,#49907,#49908,#49909,#49910,#49911,
#49912,#49913,#49914,#49915,#49916,#49917,#49918),.UNSPECIFIED.,.F.,.F.)
B_SPLINE_CURVE_WITH_KNOTS((6,1,1,1,1,1,1,1,1,1,1,1,1,1,1,1,1,1,1,1,1,1,
1,1,1,1,1,1,1,1,1,1,1,1,1,1,1,1,1,1,1,1,1,1,1,1,1,1,1,1,1,1,1,1,1,1,1,1,
1,1,1,1,1,1,1,6),(-1.,-0.984615384615383,-0.969230769230768,-0.953846153846152,
-0.938461538461537,-0.923076923076922,-0.907692307692306,-0.892307692307691,
-0.876923076923076,-0.86153846153846,-0.846153846153845,-0.83076923076923,
-0.815384615384614,-0.799999999999999,-0.784615384615384,-0.769230769230768,
-0.753846153846153,-0.738461538461538,-0.723076923076922,-0.707692307692307,
-0.692307692307692,-0.676923076923076,-0.661538461538461,-0.646153846153846,
-0.63076923076923,-0.615384615384615,-0.6,-0.584615384615384,-0.569230769230769,
-0.553846153846154,-0.538461538461538,-0.523076923076923,-0.507692307692308,
-0.492307692307692,-0.476923076923077,-0.461538461538462,-0.446153846153846,
-0.430769230769231,-0.415384615384615,-0.4,-0.384615384615385,-0.369230769230769,
-0.353846153846154,-0.338461538461538,-0.323076923076923,-0.307692307692308,
-0.292307692307692,-0.276923076923077,-0.261538461538462,-0.246153846153846,
-0.230769230769231,-0.215384615384615,-0.2,-0.184615384615385,-0.169230769230769,
-0.153846153846154,-0.138461538461538,-0.123076923076923,-0.107692307692308,
-0.0923076923076923,-0.0769230769230769,-0.0615384615384615,-0.0461538461538462,
-0.0307692307692308,-0.0153846153846154,-0.00577184337450701),
 .UNSPECIFIED.)
CURVE()
GEOMETRIC_REPRESENTATION_ITEM()
RATIONAL_B_SPLINE_CURVE((1.,1.,1.,1.,1.,1.,1.,1.,1.,1.,1.,1.,1.,1.,1.,1.,
1.,1.,1.,1.,1.,1.,1.,1.,1.,1.,1.,1.,1.,1.,1.,1.,1.,1.,1.,1.,1.,1.,1.,1.,
1.,1.,1.,1.,1.,1.,1.,1.,1.,1.,1.,1.,1.,1.,1.,1.,1.,1.,1.,1.,1.,1.,1.,1.,
1.,1.,1.,1.,1.,1.))
REPRESENTATION_ITEM('')
);
#354=(
BOUNDED_CURVE()
B_SPLINE_CURVE(5,(#50069,#50070,#50071,#50072,#50073,#50074,#50075,#50076,
#50077,#50078,#50079,#50080,#50081,#50082,#50083,#50084,#50085,#50086,#50087,
#50088,#50089,#50090,#50091,#50092,#50093,#50094,#50095,#50096,#50097,#50098,
#50099,#50100,#50101,#50102,#50103,#50104,#50105,#50106,#50107,#50108,#50109,
#50110,#50111,#50112,#50113,#50114,#50115,#50116,#50117,#50118,#50119,#50120,
#50121,#50122,#50123,#50124,#50125,#50126,#50127,#50128,#50129,#50130,#50131,
#50132,#50133,#50134,#50135,#50136,#50137,#50138),.UNSPECIFIED.,.F.,.F.)
B_SPLINE_CURVE_WITH_KNOTS((6,1,1,1,1,1,1,1,1,1,1,1,1,1,1,1,1,1,1,1,1,1,
1,1,1,1,1,1,1,1,1,1,1,1,1,1,1,1,1,1,1,1,1,1,1,1,1,1,1,1,1,1,1,1,1,1,1,1,
1,1,1,1,1,1,1,6),(-0.994228156739689,-0.984615384615383,-0.969230769230768,
-0.953846153846152,-0.938461538461537,-0.923076923076922,-0.907692307692306,
-0.892307692307691,-0.876923076923076,-0.86153846153846,-0.846153846153845,
-0.83076923076923,-0.815384615384614,-0.799999999999999,-0.784615384615384,
-0.769230769230768,-0.753846153846153,-0.738461538461538,-0.723076923076922,
-0.707692307692307,-0.692307692307692,-0.676923076923076,-0.661538461538461,
-0.646153846153846,-0.63076923076923,-0.615384615384615,-0.6,-0.584615384615384,
-0.569230769230769,-0.553846153846154,-0.538461538461538,-0.523076923076923,
-0.507692307692308,-0.492307692307692,-0.476923076923077,-0.461538461538462,
-0.446153846153846,-0.430769230769231,-0.415384615384615,-0.4,-0.384615384615385,
-0.369230769230769,-0.353846153846154,-0.338461538461538,-0.323076923076923,
-0.307692307692308,-0.292307692307692,-0.276923076923077,-0.261538461538462,
-0.246153846153846,-0.230769230769231,-0.215384615384615,-0.2,-0.184615384615385,
-0.169230769230769,-0.153846153846154,-0.138461538461538,-0.123076923076923,
-0.107692307692308,-0.0923076923076923,-0.0769230769230769,-0.0615384615384615,
-0.0461538461538462,-0.0307692307692308,-0.0153846153846154,0.),
 .UNSPECIFIED.)
CURVE()
GEOMETRIC_REPRESENTATION_ITEM()
RATIONAL_B_SPLINE_CURVE((1.,1.,1.,1.,1.,1.,1.,1.,1.,1.,1.,1.,1.,1.,1.,1.,
1.,1.,1.,1.,1.,1.,1.,1.,1.,1.,1.,1.,1.,1.,1.,1.,1.,1.,1.,1.,1.,1.,1.,1.,
1.,1.,1.,1.,1.,1.,1.,1.,1.,1.,1.,1.,1.,1.,1.,1.,1.,1.,1.,1.,1.,1.,1.,1.,
1.,1.,1.,1.,1.,1.))
REPRESENTATION_ITEM('')
);
#355=(
BOUNDED_CURVE()
B_SPLINE_CURVE(5,(#50291,#50292,#50293,#50294,#50295,#50296,#50297,#50298,
#50299,#50300,#50301,#50302,#50303,#50304,#50305,#50306,#50307,#50308,#50309,
#50310,#50311,#50312,#50313,#50314,#50315,#50316,#50317,#50318,#50319,#50320,
#50321,#50322,#50323,#50324,#50325,#50326,#50327,#50328,#50329,#50330,#50331,
#50332,#50333,#50334,#50335,#50336,#50337,#50338,#50339,#50340,#50341,#50342,
#50343,#50344,#50345,#50346,#50347,#50348,#50349,#50350,#50351,#50352,#50353,
#50354,#50355,#50356,#50357,#50358,#50359,#50360),.UNSPECIFIED.,.F.,.F.)
B_SPLINE_CURVE_WITH_KNOTS((6,1,1,1,1,1,1,1,1,1,1,1,1,1,1,1,1,1,1,1,1,1,
1,1,1,1,1,1,1,1,1,1,1,1,1,1,1,1,1,1,1,1,1,1,1,1,1,1,1,1,1,1,1,1,1,1,1,1,
1,1,1,1,1,1,1,6),(-1.,-0.984615384615383,-0.969230769230768,-0.953846153846152,
-0.938461538461537,-0.923076923076922,-0.907692307692306,-0.892307692307691,
-0.876923076923076,-0.86153846153846,-0.846153846153845,-0.83076923076923,
-0.815384615384614,-0.799999999999999,-0.784615384615384,-0.769230769230768,
-0.753846153846153,-0.738461538461538,-0.723076923076922,-0.707692307692307,
-0.692307692307692,-0.676923076923076,-0.661538461538461,-0.646153846153846,
-0.63076923076923,-0.615384615384615,-0.6,-0.584615384615384,-0.569230769230769,
-0.553846153846154,-0.538461538461538,-0.523076923076923,-0.507692307692308,
-0.492307692307692,-0.476923076923077,-0.461538461538462,-0.446153846153846,
-0.430769230769231,-0.415384615384615,-0.4,-0.384615384615385,-0.369230769230769,
-0.353846153846154,-0.338461538461538,-0.323076923076923,-0.307692307692308,
-0.292307692307692,-0.276923076923077,-0.261538461538462,-0.246153846153846,
-0.230769230769231,-0.215384615384615,-0.2,-0.184615384615385,-0.169230769230769,
-0.153846153846154,-0.138461538461538,-0.123076923076923,-0.107692307692308,
-0.0923076923076923,-0.0769230769230769,-0.0615384615384615,-0.0461538461538462,
-0.0307692307692308,-0.0153846153846154,-0.00577184337452382),
 .UNSPECIFIED.)
CURVE()
GEOMETRIC_REPRESENTATION_ITEM()
RATIONAL_B_SPLINE_CURVE((1.,1.,1.,1.,1.,1.,1.,1.,1.,1.,1.,1.,1.,1.,1.,1.,
1.,1.,1.,1.,1.,1.,1.,1.,1.,1.,1.,1.,1.,1.,1.,1.,1.,1.,1.,1.,1.,1.,1.,1.,
1.,1.,1.,1.,1.,1.,1.,1.,1.,1.,1.,1.,1.,1.,1.,1.,1.,1.,1.,1.,1.,1.,1.,1.,
1.,1.,1.,1.,1.,1.))
REPRESENTATION_ITEM('')
);
#356=(
BOUNDED_CURVE()
B_SPLINE_CURVE(5,(#50511,#50512,#50513,#50514,#50515,#50516,#50517,#50518,
#50519,#50520,#50521,#50522,#50523,#50524,#50525,#50526,#50527,#50528,#50529,
#50530,#50531,#50532,#50533,#50534,#50535,#50536,#50537,#50538,#50539,#50540,
#50541,#50542,#50543,#50544,#50545,#50546,#50547,#50548,#50549,#50550,#50551,
#50552,#50553,#50554,#50555,#50556,#50557,#50558,#50559,#50560,#50561,#50562,
#50563,#50564,#50565,#50566,#50567,#50568,#50569,#50570,#50571,#50572,#50573,
#50574,#50575,#50576,#50577,#50578,#50579,#50580),.UNSPECIFIED.,.F.,.F.)
B_SPLINE_CURVE_WITH_KNOTS((6,1,1,1,1,1,1,1,1,1,1,1,1,1,1,1,1,1,1,1,1,1,
1,1,1,1,1,1,1,1,1,1,1,1,1,1,1,1,1,1,1,1,1,1,1,1,1,1,1,1,1,1,1,1,1,1,1,1,
1,1,1,1,1,1,1,6),(-0.994228156739677,-0.984615384615383,-0.969230769230768,
-0.953846153846152,-0.938461538461537,-0.923076923076922,-0.907692307692306,
-0.892307692307691,-0.876923076923076,-0.86153846153846,-0.846153846153845,
-0.83076923076923,-0.815384615384614,-0.799999999999999,-0.784615384615384,
-0.769230769230768,-0.753846153846153,-0.738461538461538,-0.723076923076922,
-0.707692307692307,-0.692307692307692,-0.676923076923076,-0.661538461538461,
-0.646153846153846,-0.63076923076923,-0.615384615384615,-0.6,-0.584615384615384,
-0.569230769230769,-0.553846153846154,-0.538461538461538,-0.523076923076923,
-0.507692307692308,-0.492307692307692,-0.476923076923077,-0.461538461538462,
-0.446153846153846,-0.430769230769231,-0.415384615384615,-0.4,-0.384615384615385,
-0.369230769230769,-0.353846153846154,-0.338461538461538,-0.323076923076923,
-0.307692307692308,-0.292307692307692,-0.276923076923077,-0.261538461538462,
-0.246153846153846,-0.230769230769231,-0.215384615384615,-0.2,-0.184615384615385,
-0.169230769230769,-0.153846153846154,-0.138461538461538,-0.123076923076923,
-0.107692307692308,-0.0923076923076923,-0.0769230769230769,-0.0615384615384615,
-0.0461538461538462,-0.0307692307692308,-0.0153846153846154,0.),
 .UNSPECIFIED.)
CURVE()
GEOMETRIC_REPRESENTATION_ITEM()
RATIONAL_B_SPLINE_CURVE((1.,1.,1.,1.,1.,1.,1.,1.,1.,1.,1.,1.,1.,1.,1.,1.,
1.,1.,1.,1.,1.,1.,1.,1.,1.,1.,1.,1.,1.,1.,1.,1.,1.,1.,1.,1.,1.,1.,1.,1.,
1.,1.,1.,1.,1.,1.,1.,1.,1.,1.,1.,1.,1.,1.,1.,1.,1.,1.,1.,1.,1.,1.,1.,1.,
1.,1.,1.,1.,1.,1.))
REPRESENTATION_ITEM('')
);
#357=(
BOUNDED_CURVE()
B_SPLINE_CURVE(5,(#50733,#50734,#50735,#50736,#50737,#50738,#50739,#50740,
#50741,#50742,#50743,#50744,#50745,#50746,#50747,#50748,#50749,#50750,#50751,
#50752,#50753,#50754,#50755,#50756,#50757,#50758,#50759,#50760,#50761,#50762,
#50763,#50764,#50765,#50766,#50767,#50768,#50769,#50770,#50771,#50772,#50773,
#50774,#50775,#50776,#50777,#50778,#50779,#50780,#50781,#50782,#50783,#50784,
#50785,#50786,#50787,#50788,#50789,#50790,#50791,#50792,#50793,#50794,#50795,
#50796,#50797,#50798,#50799,#50800,#50801,#50802),.UNSPECIFIED.,.F.,.F.)
B_SPLINE_CURVE_WITH_KNOTS((6,1,1,1,1,1,1,1,1,1,1,1,1,1,1,1,1,1,1,1,1,1,
1,1,1,1,1,1,1,1,1,1,1,1,1,1,1,1,1,1,1,1,1,1,1,1,1,1,1,1,1,1,1,1,1,1,1,1,
1,1,1,1,1,1,1,6),(-1.,-0.984615384615383,-0.969230769230768,-0.953846153846152,
-0.938461538461537,-0.923076923076922,-0.907692307692306,-0.892307692307691,
-0.876923076923076,-0.86153846153846,-0.846153846153845,-0.83076923076923,
-0.815384615384614,-0.799999999999999,-0.784615384615384,-0.769230769230768,
-0.753846153846153,-0.738461538461538,-0.723076923076922,-0.707692307692307,
-0.692307692307692,-0.676923076923076,-0.661538461538461,-0.646153846153846,
-0.63076923076923,-0.615384615384615,-0.6,-0.584615384615384,-0.569230769230769,
-0.553846153846154,-0.538461538461538,-0.523076923076923,-0.507692307692308,
-0.492307692307692,-0.476923076923077,-0.461538461538462,-0.446153846153846,
-0.430769230769231,-0.415384615384615,-0.4,-0.384615384615385,-0.369230769230769,
-0.353846153846154,-0.338461538461538,-0.323076923076923,-0.307692307692308,
-0.292307692307692,-0.276923076923077,-0.261538461538462,-0.246153846153846,
-0.230769230769231,-0.215384615384615,-0.2,-0.184615384615385,-0.169230769230769,
-0.153846153846154,-0.138461538461538,-0.123076923076923,-0.107692307692308,
-0.0923076923076923,-0.0769230769230769,-0.0615384615384615,-0.0461538461538462,
-0.0307692307692308,-0.0153846153846154,-0.0057718433744938),
 .UNSPECIFIED.)
CURVE()
GEOMETRIC_REPRESENTATION_ITEM()
RATIONAL_B_SPLINE_CURVE((1.,1.,1.,1.,1.,1.,1.,1.,1.,1.,1.,1.,1.,1.,1.,1.,
1.,1.,1.,1.,1.,1.,1.,1.,1.,1.,1.,1.,1.,1.,1.,1.,1.,1.,1.,1.,1.,1.,1.,1.,
1.,1.,1.,1.,1.,1.,1.,1.,1.,1.,1.,1.,1.,1.,1.,1.,1.,1.,1.,1.,1.,1.,1.,1.,
1.,1.,1.,1.,1.,1.))
REPRESENTATION_ITEM('')
);
#358=(
BOUNDED_CURVE()
B_SPLINE_CURVE(5,(#50953,#50954,#50955,#50956,#50957,#50958,#50959,#50960,
#50961,#50962,#50963,#50964,#50965,#50966,#50967,#50968,#50969,#50970,#50971,
#50972,#50973,#50974,#50975,#50976,#50977,#50978,#50979,#50980,#50981,#50982,
#50983,#50984,#50985,#50986,#50987,#50988,#50989,#50990,#50991,#50992,#50993,
#50994,#50995,#50996,#50997,#50998,#50999,#51000,#51001,#51002,#51003,#51004,
#51005,#51006,#51007,#51008,#51009,#51010,#51011,#51012,#51013,#51014,#51015,
#51016,#51017,#51018,#51019,#51020,#51021,#51022),.UNSPECIFIED.,.F.,.F.)
B_SPLINE_CURVE_WITH_KNOTS((6,1,1,1,1,1,1,1,1,1,1,1,1,1,1,1,1,1,1,1,1,1,
1,1,1,1,1,1,1,1,1,1,1,1,1,1,1,1,1,1,1,1,1,1,1,1,1,1,1,1,1,1,1,1,1,1,1,1,
1,1,1,1,1,1,1,6),(-0.994228156739743,-0.984615384615383,-0.969230769230768,
-0.953846153846152,-0.938461538461537,-0.923076923076922,-0.907692307692306,
-0.892307692307691,-0.876923076923076,-0.86153846153846,-0.846153846153845,
-0.83076923076923,-0.815384615384614,-0.799999999999999,-0.784615384615384,
-0.769230769230768,-0.753846153846153,-0.738461538461538,-0.723076923076922,
-0.707692307692307,-0.692307692307692,-0.676923076923076,-0.661538461538461,
-0.646153846153846,-0.63076923076923,-0.615384615384615,-0.6,-0.584615384615384,
-0.569230769230769,-0.553846153846154,-0.538461538461538,-0.523076923076923,
-0.507692307692308,-0.492307692307692,-0.476923076923077,-0.461538461538462,
-0.446153846153846,-0.430769230769231,-0.415384615384615,-0.4,-0.384615384615385,
-0.369230769230769,-0.353846153846154,-0.338461538461538,-0.323076923076923,
-0.307692307692308,-0.292307692307692,-0.276923076923077,-0.261538461538462,
-0.246153846153846,-0.230769230769231,-0.215384615384615,-0.2,-0.184615384615385,
-0.169230769230769,-0.153846153846154,-0.138461538461538,-0.123076923076923,
-0.107692307692308,-0.0923076923076923,-0.0769230769230769,-0.0615384615384615,
-0.0461538461538462,-0.0307692307692308,-0.0153846153846154,0.),
 .UNSPECIFIED.)
CURVE()
GEOMETRIC_REPRESENTATION_ITEM()
RATIONAL_B_SPLINE_CURVE((1.,1.,1.,1.,1.,1.,1.,1.,1.,1.,1.,1.,1.,1.,1.,1.,
1.,1.,1.,1.,1.,1.,1.,1.,1.,1.,1.,1.,1.,1.,1.,1.,1.,1.,1.,1.,1.,1.,1.,1.,
1.,1.,1.,1.,1.,1.,1.,1.,1.,1.,1.,1.,1.,1.,1.,1.,1.,1.,1.,1.,1.,1.,1.,1.,
1.,1.,1.,1.,1.,1.))
REPRESENTATION_ITEM('')
);
#359=(
BOUNDED_CURVE()
B_SPLINE_CURVE(5,(#51175,#51176,#51177,#51178,#51179,#51180,#51181,#51182,
#51183,#51184,#51185,#51186,#51187,#51188,#51189,#51190,#51191,#51192,#51193,
#51194,#51195,#51196,#51197,#51198,#51199,#51200,#51201,#51202,#51203,#51204,
#51205,#51206,#51207,#51208,#51209,#51210,#51211,#51212,#51213,#51214,#51215,
#51216,#51217,#51218,#51219,#51220,#51221,#51222,#51223,#51224,#51225,#51226,
#51227,#51228,#51229,#51230,#51231,#51232,#51233,#51234,#51235,#51236,#51237,
#51238,#51239,#51240,#51241,#51242,#51243,#51244),.UNSPECIFIED.,.F.,.F.)
B_SPLINE_CURVE_WITH_KNOTS((6,1,1,1,1,1,1,1,1,1,1,1,1,1,1,1,1,1,1,1,1,1,
1,1,1,1,1,1,1,1,1,1,1,1,1,1,1,1,1,1,1,1,1,1,1,1,1,1,1,1,1,1,1,1,1,1,1,1,
1,1,1,1,1,1,1,6),(-1.,-0.984615384615383,-0.969230769230768,-0.953846153846152,
-0.938461538461537,-0.923076923076922,-0.907692307692306,-0.892307692307691,
-0.876923076923076,-0.86153846153846,-0.846153846153845,-0.83076923076923,
-0.815384615384614,-0.799999999999999,-0.784615384615384,-0.769230769230768,
-0.753846153846153,-0.738461538461538,-0.723076923076922,-0.707692307692307,
-0.692307692307692,-0.676923076923076,-0.661538461538461,-0.646153846153846,
-0.63076923076923,-0.615384615384615,-0.6,-0.584615384615384,-0.569230769230769,
-0.553846153846154,-0.538461538461538,-0.523076923076923,-0.507692307692308,
-0.492307692307692,-0.476923076923077,-0.461538461538462,-0.446153846153846,
-0.430769230769231,-0.415384615384615,-0.4,-0.384615384615385,-0.369230769230769,
-0.353846153846154,-0.338461538461538,-0.323076923076923,-0.307692307692308,
-0.292307692307692,-0.276923076923077,-0.261538461538462,-0.246153846153846,
-0.230769230769231,-0.215384615384615,-0.2,-0.184615384615385,-0.169230769230769,
-0.153846153846154,-0.138461538461538,-0.123076923076923,-0.107692307692308,
-0.0923076923076923,-0.0769230769230769,-0.0615384615384615,-0.0461538461538462,
-0.0307692307692308,-0.0153846153846154,-0.0057718433745291),
 .UNSPECIFIED.)
CURVE()
GEOMETRIC_REPRESENTATION_ITEM()
RATIONAL_B_SPLINE_CURVE((1.,1.,1.,1.,1.,1.,1.,1.,1.,1.,1.,1.,1.,1.,1.,1.,
1.,1.,1.,1.,1.,1.,1.,1.,1.,1.,1.,1.,1.,1.,1.,1.,1.,1.,1.,1.,1.,1.,1.,1.,
1.,1.,1.,1.,1.,1.,1.,1.,1.,1.,1.,1.,1.,1.,1.,1.,1.,1.,1.,1.,1.,1.,1.,1.,
1.,1.,1.,1.,1.,1.))
REPRESENTATION_ITEM('')
);
#360=(
BOUNDED_CURVE()
B_SPLINE_CURVE(5,(#51395,#51396,#51397,#51398,#51399,#51400,#51401,#51402,
#51403,#51404,#51405,#51406,#51407,#51408,#51409,#51410,#51411,#51412,#51413,
#51414,#51415,#51416,#51417,#51418,#51419,#51420,#51421,#51422,#51423,#51424,
#51425,#51426,#51427,#51428,#51429,#51430,#51431,#51432,#51433,#51434,#51435,
#51436,#51437,#51438,#51439,#51440,#51441,#51442,#51443,#51444,#51445,#51446,
#51447,#51448,#51449,#51450,#51451,#51452,#51453,#51454,#51455,#51456,#51457,
#51458,#51459,#51460,#51461,#51462,#51463,#51464),.UNSPECIFIED.,.F.,.F.)
B_SPLINE_CURVE_WITH_KNOTS((6,1,1,1,1,1,1,1,1,1,1,1,1,1,1,1,1,1,1,1,1,1,
1,1,1,1,1,1,1,1,1,1,1,1,1,1,1,1,1,1,1,1,1,1,1,1,1,1,1,1,1,1,1,1,1,1,1,1,
1,1,1,1,1,1,1,6),(-0.994228156739665,-0.984615384615383,-0.969230769230768,
-0.953846153846152,-0.938461538461537,-0.923076923076922,-0.907692307692306,
-0.892307692307691,-0.876923076923076,-0.86153846153846,-0.846153846153845,
-0.83076923076923,-0.815384615384614,-0.799999999999999,-0.784615384615384,
-0.769230769230768,-0.753846153846153,-0.738461538461538,-0.723076923076922,
-0.707692307692307,-0.692307692307692,-0.676923076923076,-0.661538461538461,
-0.646153846153846,-0.63076923076923,-0.615384615384615,-0.6,-0.584615384615384,
-0.569230769230769,-0.553846153846154,-0.538461538461538,-0.523076923076923,
-0.507692307692308,-0.492307692307692,-0.476923076923077,-0.461538461538462,
-0.446153846153846,-0.430769230769231,-0.415384615384615,-0.4,-0.384615384615385,
-0.369230769230769,-0.353846153846154,-0.338461538461538,-0.323076923076923,
-0.307692307692308,-0.292307692307692,-0.276923076923077,-0.261538461538462,
-0.246153846153846,-0.230769230769231,-0.215384615384615,-0.2,-0.184615384615385,
-0.169230769230769,-0.153846153846154,-0.138461538461538,-0.123076923076923,
-0.107692307692308,-0.0923076923076923,-0.0769230769230769,-0.0615384615384615,
-0.0461538461538462,-0.0307692307692308,-0.0153846153846154,0.),
 .UNSPECIFIED.)
CURVE()
GEOMETRIC_REPRESENTATION_ITEM()
RATIONAL_B_SPLINE_CURVE((1.,1.,1.,1.,1.,1.,1.,1.,1.,1.,1.,1.,1.,1.,1.,1.,
1.,1.,1.,1.,1.,1.,1.,1.,1.,1.,1.,1.,1.,1.,1.,1.,1.,1.,1.,1.,1.,1.,1.,1.,
1.,1.,1.,1.,1.,1.,1.,1.,1.,1.,1.,1.,1.,1.,1.,1.,1.,1.,1.,1.,1.,1.,1.,1.,
1.,1.,1.,1.,1.,1.))
REPRESENTATION_ITEM('')
);
#361=(
BOUNDED_CURVE()
B_SPLINE_CURVE(5,(#51617,#51618,#51619,#51620,#51621,#51622,#51623,#51624,
#51625,#51626,#51627,#51628,#51629,#51630,#51631,#51632,#51633,#51634,#51635,
#51636,#51637,#51638,#51639,#51640,#51641,#51642,#51643,#51644,#51645,#51646,
#51647,#51648,#51649,#51650,#51651,#51652,#51653,#51654,#51655,#51656,#51657,
#51658,#51659,#51660,#51661,#51662,#51663,#51664,#51665,#51666,#51667,#51668,
#51669,#51670,#51671,#51672,#51673,#51674,#51675,#51676,#51677,#51678,#51679,
#51680,#51681,#51682,#51683,#51684,#51685,#51686),.UNSPECIFIED.,.F.,.F.)
B_SPLINE_CURVE_WITH_KNOTS((6,1,1,1,1,1,1,1,1,1,1,1,1,1,1,1,1,1,1,1,1,1,
1,1,1,1,1,1,1,1,1,1,1,1,1,1,1,1,1,1,1,1,1,1,1,1,1,1,1,1,1,1,1,1,1,1,1,1,
1,1,1,1,1,1,1,6),(-1.,-0.984615384615383,-0.969230769230768,-0.953846153846152,
-0.938461538461537,-0.923076923076922,-0.907692307692306,-0.892307692307691,
-0.876923076923076,-0.86153846153846,-0.846153846153845,-0.83076923076923,
-0.815384615384614,-0.799999999999999,-0.784615384615384,-0.769230769230768,
-0.753846153846153,-0.738461538461538,-0.723076923076922,-0.707692307692307,
-0.692307692307692,-0.676923076923076,-0.661538461538461,-0.646153846153846,
-0.63076923076923,-0.615384615384615,-0.6,-0.584615384615384,-0.569230769230769,
-0.553846153846154,-0.538461538461538,-0.523076923076923,-0.507692307692308,
-0.492307692307692,-0.476923076923077,-0.461538461538462,-0.446153846153846,
-0.430769230769231,-0.415384615384615,-0.4,-0.384615384615385,-0.369230769230769,
-0.353846153846154,-0.338461538461538,-0.323076923076923,-0.307692307692308,
-0.292307692307692,-0.276923076923077,-0.261538461538462,-0.246153846153846,
-0.230769230769231,-0.215384615384615,-0.2,-0.184615384615385,-0.169230769230769,
-0.153846153846154,-0.138461538461538,-0.123076923076923,-0.107692307692308,
-0.0923076923076923,-0.0769230769230769,-0.0615384615384615,-0.0461538461538462,
-0.0307692307692308,-0.0153846153846154,-0.00577184337450666),
 .UNSPECIFIED.)
CURVE()
GEOMETRIC_REPRESENTATION_ITEM()
RATIONAL_B_SPLINE_CURVE((1.,1.,1.,1.,1.,1.,1.,1.,1.,1.,1.,1.,1.,1.,1.,1.,
1.,1.,1.,1.,1.,1.,1.,1.,1.,1.,1.,1.,1.,1.,1.,1.,1.,1.,1.,1.,1.,1.,1.,1.,
1.,1.,1.,1.,1.,1.,1.,1.,1.,1.,1.,1.,1.,1.,1.,1.,1.,1.,1.,1.,1.,1.,1.,1.,
1.,1.,1.,1.,1.,1.))
REPRESENTATION_ITEM('')
);
#362=(
BOUNDED_CURVE()
B_SPLINE_CURVE(5,(#51837,#51838,#51839,#51840,#51841,#51842,#51843,#51844,
#51845,#51846,#51847,#51848,#51849,#51850,#51851,#51852,#51853,#51854,#51855,
#51856,#51857,#51858,#51859,#51860,#51861,#51862,#51863,#51864,#51865,#51866,
#51867,#51868,#51869,#51870,#51871,#51872,#51873,#51874,#51875,#51876,#51877,
#51878,#51879,#51880,#51881,#51882,#51883,#51884,#51885,#51886,#51887,#51888,
#51889,#51890,#51891,#51892,#51893,#51894,#51895,#51896,#51897,#51898,#51899,
#51900,#51901,#51902,#51903,#51904,#51905,#51906),.UNSPECIFIED.,.F.,.F.)
B_SPLINE_CURVE_WITH_KNOTS((6,1,1,1,1,1,1,1,1,1,1,1,1,1,1,1,1,1,1,1,1,1,
1,1,1,1,1,1,1,1,1,1,1,1,1,1,1,1,1,1,1,1,1,1,1,1,1,1,1,1,1,1,1,1,1,1,1,1,
1,1,1,1,1,1,1,6),(-0.994228156739758,-0.984615384615383,-0.969230769230768,
-0.953846153846152,-0.938461538461537,-0.923076923076922,-0.907692307692306,
-0.892307692307691,-0.876923076923076,-0.86153846153846,-0.846153846153845,
-0.83076923076923,-0.815384615384614,-0.799999999999999,-0.784615384615384,
-0.769230769230768,-0.753846153846153,-0.738461538461538,-0.723076923076922,
-0.707692307692307,-0.692307692307692,-0.676923076923076,-0.661538461538461,
-0.646153846153846,-0.63076923076923,-0.615384615384615,-0.6,-0.584615384615384,
-0.569230769230769,-0.553846153846154,-0.538461538461538,-0.523076923076923,
-0.507692307692308,-0.492307692307692,-0.476923076923077,-0.461538461538462,
-0.446153846153846,-0.430769230769231,-0.415384615384615,-0.4,-0.384615384615385,
-0.369230769230769,-0.353846153846154,-0.338461538461538,-0.323076923076923,
-0.307692307692308,-0.292307692307692,-0.276923076923077,-0.261538461538462,
-0.246153846153846,-0.230769230769231,-0.215384615384615,-0.2,-0.184615384615385,
-0.169230769230769,-0.153846153846154,-0.138461538461538,-0.123076923076923,
-0.107692307692308,-0.0923076923076923,-0.0769230769230769,-0.0615384615384615,
-0.0461538461538462,-0.0307692307692308,-0.0153846153846154,0.),
 .UNSPECIFIED.)
CURVE()
GEOMETRIC_REPRESENTATION_ITEM()
RATIONAL_B_SPLINE_CURVE((1.,1.,1.,1.,1.,1.,1.,1.,1.,1.,1.,1.,1.,1.,1.,1.,
1.,1.,1.,1.,1.,1.,1.,1.,1.,1.,1.,1.,1.,1.,1.,1.,1.,1.,1.,1.,1.,1.,1.,1.,
1.,1.,1.,1.,1.,1.,1.,1.,1.,1.,1.,1.,1.,1.,1.,1.,1.,1.,1.,1.,1.,1.,1.,1.,
1.,1.,1.,1.,1.,1.))
REPRESENTATION_ITEM('')
);
#363=(
BOUNDED_CURVE()
B_SPLINE_CURVE(5,(#52059,#52060,#52061,#52062,#52063,#52064,#52065,#52066,
#52067,#52068,#52069,#52070,#52071,#52072,#52073,#52074,#52075,#52076,#52077,
#52078,#52079,#52080,#52081,#52082,#52083,#52084,#52085,#52086,#52087,#52088,
#52089,#52090,#52091,#52092,#52093,#52094,#52095,#52096,#52097,#52098,#52099,
#52100,#52101,#52102,#52103,#52104,#52105,#52106,#52107,#52108,#52109,#52110,
#52111,#52112,#52113,#52114,#52115,#52116,#52117,#52118,#52119,#52120,#52121,
#52122,#52123,#52124,#52125,#52126,#52127,#52128),.UNSPECIFIED.,.F.,.F.)
B_SPLINE_CURVE_WITH_KNOTS((6,1,1,1,1,1,1,1,1,1,1,1,1,1,1,1,1,1,1,1,1,1,
1,1,1,1,1,1,1,1,1,1,1,1,1,1,1,1,1,1,1,1,1,1,1,1,1,1,1,1,1,1,1,1,1,1,1,1,
1,1,1,1,1,1,1,6),(-1.,-0.984615384615383,-0.969230769230768,-0.953846153846152,
-0.938461538461537,-0.923076923076922,-0.907692307692306,-0.892307692307691,
-0.876923076923076,-0.86153846153846,-0.846153846153845,-0.83076923076923,
-0.815384615384614,-0.799999999999999,-0.784615384615384,-0.769230769230768,
-0.753846153846153,-0.738461538461538,-0.723076923076922,-0.707692307692307,
-0.692307692307692,-0.676923076923076,-0.661538461538461,-0.646153846153846,
-0.63076923076923,-0.615384615384615,-0.6,-0.584615384615384,-0.569230769230769,
-0.553846153846154,-0.538461538461538,-0.523076923076923,-0.507692307692308,
-0.492307692307692,-0.476923076923077,-0.461538461538462,-0.446153846153846,
-0.430769230769231,-0.415384615384615,-0.4,-0.384615384615385,-0.369230769230769,
-0.353846153846154,-0.338461538461538,-0.323076923076923,-0.307692307692308,
-0.292307692307692,-0.276923076923077,-0.261538461538462,-0.246153846153846,
-0.230769230769231,-0.215384615384615,-0.2,-0.184615384615385,-0.169230769230769,
-0.153846153846154,-0.138461538461538,-0.123076923076923,-0.107692307692308,
-0.0923076923076923,-0.0769230769230769,-0.0615384615384615,-0.0461538461538462,
-0.0307692307692308,-0.0153846153846154,-0.00577184337451981),
 .UNSPECIFIED.)
CURVE()
GEOMETRIC_REPRESENTATION_ITEM()
RATIONAL_B_SPLINE_CURVE((1.,1.,1.,1.,1.,1.,1.,1.,1.,1.,1.,1.,1.,1.,1.,1.,
1.,1.,1.,1.,1.,1.,1.,1.,1.,1.,1.,1.,1.,1.,1.,1.,1.,1.,1.,1.,1.,1.,1.,1.,
1.,1.,1.,1.,1.,1.,1.,1.,1.,1.,1.,1.,1.,1.,1.,1.,1.,1.,1.,1.,1.,1.,1.,1.,
1.,1.,1.,1.,1.,1.))
REPRESENTATION_ITEM('')
);
#364=(
BOUNDED_CURVE()
B_SPLINE_CURVE(5,(#52279,#52280,#52281,#52282,#52283,#52284,#52285,#52286,
#52287,#52288,#52289,#52290,#52291,#52292,#52293,#52294,#52295,#52296,#52297,
#52298,#52299,#52300,#52301,#52302,#52303,#52304,#52305,#52306,#52307,#52308,
#52309,#52310,#52311,#52312,#52313,#52314,#52315,#52316,#52317,#52318,#52319,
#52320,#52321,#52322,#52323,#52324,#52325,#52326,#52327,#52328,#52329,#52330,
#52331,#52332,#52333,#52334,#52335,#52336,#52337,#52338,#52339,#52340,#52341,
#52342,#52343,#52344,#52345,#52346,#52347,#52348),.UNSPECIFIED.,.F.,.F.)
B_SPLINE_CURVE_WITH_KNOTS((6,1,1,1,1,1,1,1,1,1,1,1,1,1,1,1,1,1,1,1,1,1,
1,1,1,1,1,1,1,1,1,1,1,1,1,1,1,1,1,1,1,1,1,1,1,1,1,1,1,1,1,1,1,1,1,1,1,1,
1,1,1,1,1,1,1,6),(-0.994228156739659,-0.984615384615383,-0.969230769230768,
-0.953846153846152,-0.938461538461537,-0.923076923076922,-0.907692307692306,
-0.892307692307691,-0.876923076923076,-0.86153846153846,-0.846153846153845,
-0.83076923076923,-0.815384615384614,-0.799999999999999,-0.784615384615384,
-0.769230769230768,-0.753846153846153,-0.738461538461538,-0.723076923076922,
-0.707692307692307,-0.692307692307692,-0.676923076923076,-0.661538461538461,
-0.646153846153846,-0.63076923076923,-0.615384615384615,-0.6,-0.584615384615384,
-0.569230769230769,-0.553846153846154,-0.538461538461538,-0.523076923076923,
-0.507692307692308,-0.492307692307692,-0.476923076923077,-0.461538461538462,
-0.446153846153846,-0.430769230769231,-0.415384615384615,-0.4,-0.384615384615385,
-0.369230769230769,-0.353846153846154,-0.338461538461538,-0.323076923076923,
-0.307692307692308,-0.292307692307692,-0.276923076923077,-0.261538461538462,
-0.246153846153846,-0.230769230769231,-0.215384615384615,-0.2,-0.184615384615385,
-0.169230769230769,-0.153846153846154,-0.138461538461538,-0.123076923076923,
-0.107692307692308,-0.0923076923076923,-0.0769230769230769,-0.0615384615384615,
-0.0461538461538462,-0.0307692307692308,-0.0153846153846154,0.),
 .UNSPECIFIED.)
CURVE()
GEOMETRIC_REPRESENTATION_ITEM()
RATIONAL_B_SPLINE_CURVE((1.,1.,1.,1.,1.,1.,1.,1.,1.,1.,1.,1.,1.,1.,1.,1.,
1.,1.,1.,1.,1.,1.,1.,1.,1.,1.,1.,1.,1.,1.,1.,1.,1.,1.,1.,1.,1.,1.,1.,1.,
1.,1.,1.,1.,1.,1.,1.,1.,1.,1.,1.,1.,1.,1.,1.,1.,1.,1.,1.,1.,1.,1.,1.,1.,
1.,1.,1.,1.,1.,1.))
REPRESENTATION_ITEM('')
);
#365=(
BOUNDED_CURVE()
B_SPLINE_CURVE(5,(#52501,#52502,#52503,#52504,#52505,#52506,#52507,#52508,
#52509,#52510,#52511,#52512,#52513,#52514,#52515,#52516,#52517,#52518,#52519,
#52520,#52521,#52522,#52523,#52524,#52525,#52526,#52527,#52528,#52529,#52530,
#52531,#52532,#52533,#52534,#52535,#52536,#52537,#52538,#52539,#52540,#52541,
#52542,#52543,#52544,#52545,#52546,#52547,#52548,#52549,#52550,#52551,#52552,
#52553,#52554,#52555,#52556,#52557,#52558,#52559,#52560,#52561,#52562,#52563,
#52564,#52565,#52566,#52567,#52568,#52569,#52570),.UNSPECIFIED.,.F.,.F.)
B_SPLINE_CURVE_WITH_KNOTS((6,1,1,1,1,1,1,1,1,1,1,1,1,1,1,1,1,1,1,1,1,1,
1,1,1,1,1,1,1,1,1,1,1,1,1,1,1,1,1,1,1,1,1,1,1,1,1,1,1,1,1,1,1,1,1,1,1,1,
1,1,1,1,1,1,1,6),(-1.,-0.984615384615383,-0.969230769230768,-0.953846153846152,
-0.938461538461537,-0.923076923076922,-0.907692307692306,-0.892307692307691,
-0.876923076923076,-0.86153846153846,-0.846153846153845,-0.83076923076923,
-0.815384615384614,-0.799999999999999,-0.784615384615384,-0.769230769230768,
-0.753846153846153,-0.738461538461538,-0.723076923076922,-0.707692307692307,
-0.692307692307692,-0.676923076923076,-0.661538461538461,-0.646153846153846,
-0.63076923076923,-0.615384615384615,-0.6,-0.584615384615384,-0.569230769230769,
-0.553846153846154,-0.538461538461538,-0.523076923076923,-0.507692307692308,
-0.492307692307692,-0.476923076923077,-0.461538461538462,-0.446153846153846,
-0.430769230769231,-0.415384615384615,-0.4,-0.384615384615385,-0.369230769230769,
-0.353846153846154,-0.338461538461538,-0.323076923076923,-0.307692307692308,
-0.292307692307692,-0.276923076923077,-0.261538461538462,-0.246153846153846,
-0.230769230769231,-0.215384615384615,-0.2,-0.184615384615385,-0.169230769230769,
-0.153846153846154,-0.138461538461538,-0.123076923076923,-0.107692307692308,
-0.0923076923076923,-0.0769230769230769,-0.0615384615384615,-0.0461538461538462,
-0.0307692307692308,-0.0153846153846154,-0.00577184337450306),
 .UNSPECIFIED.)
CURVE()
GEOMETRIC_REPRESENTATION_ITEM()
RATIONAL_B_SPLINE_CURVE((1.,1.,1.,1.,1.,1.,1.,1.,1.,1.,1.,1.,1.,1.,1.,1.,
1.,1.,1.,1.,1.,1.,1.,1.,1.,1.,1.,1.,1.,1.,1.,1.,1.,1.,1.,1.,1.,1.,1.,1.,
1.,1.,1.,1.,1.,1.,1.,1.,1.,1.,1.,1.,1.,1.,1.,1.,1.,1.,1.,1.,1.,1.,1.,1.,
1.,1.,1.,1.,1.,1.))
REPRESENTATION_ITEM('')
);
#366=(
BOUNDED_CURVE()
B_SPLINE_CURVE(5,(#52721,#52722,#52723,#52724,#52725,#52726,#52727,#52728,
#52729,#52730,#52731,#52732,#52733,#52734,#52735,#52736,#52737,#52738,#52739,
#52740,#52741,#52742,#52743,#52744,#52745,#52746,#52747,#52748,#52749,#52750,
#52751,#52752,#52753,#52754,#52755,#52756,#52757,#52758,#52759,#52760,#52761,
#52762,#52763,#52764,#52765,#52766,#52767,#52768,#52769,#52770,#52771,#52772,
#52773,#52774,#52775,#52776,#52777,#52778,#52779,#52780,#52781,#52782,#52783,
#52784,#52785,#52786,#52787,#52788,#52789,#52790),.UNSPECIFIED.,.F.,.F.)
B_SPLINE_CURVE_WITH_KNOTS((6,1,1,1,1,1,1,1,1,1,1,1,1,1,1,1,1,1,1,1,1,1,
1,1,1,1,1,1,1,1,1,1,1,1,1,1,1,1,1,1,1,1,1,1,1,1,1,1,1,1,1,1,1,1,1,1,1,1,
1,1,1,1,1,1,1,6),(-0.994228156739675,-0.984615384615383,-0.969230769230768,
-0.953846153846152,-0.938461538461537,-0.923076923076922,-0.907692307692306,
-0.892307692307691,-0.876923076923076,-0.86153846153846,-0.846153846153845,
-0.83076923076923,-0.815384615384614,-0.799999999999999,-0.784615384615384,
-0.769230769230768,-0.753846153846153,-0.738461538461538,-0.723076923076922,
-0.707692307692307,-0.692307692307692,-0.676923076923076,-0.661538461538461,
-0.646153846153846,-0.63076923076923,-0.615384615384615,-0.6,-0.584615384615384,
-0.569230769230769,-0.553846153846154,-0.538461538461538,-0.523076923076923,
-0.507692307692308,-0.492307692307692,-0.476923076923077,-0.461538461538462,
-0.446153846153846,-0.430769230769231,-0.415384615384615,-0.4,-0.384615384615385,
-0.369230769230769,-0.353846153846154,-0.338461538461538,-0.323076923076923,
-0.307692307692308,-0.292307692307692,-0.276923076923077,-0.261538461538462,
-0.246153846153846,-0.230769230769231,-0.215384615384615,-0.2,-0.184615384615385,
-0.169230769230769,-0.153846153846154,-0.138461538461538,-0.123076923076923,
-0.107692307692308,-0.0923076923076923,-0.0769230769230769,-0.0615384615384615,
-0.0461538461538462,-0.0307692307692308,-0.0153846153846154,0.),
 .UNSPECIFIED.)
CURVE()
GEOMETRIC_REPRESENTATION_ITEM()
RATIONAL_B_SPLINE_CURVE((1.,1.,1.,1.,1.,1.,1.,1.,1.,1.,1.,1.,1.,1.,1.,1.,
1.,1.,1.,1.,1.,1.,1.,1.,1.,1.,1.,1.,1.,1.,1.,1.,1.,1.,1.,1.,1.,1.,1.,1.,
1.,1.,1.,1.,1.,1.,1.,1.,1.,1.,1.,1.,1.,1.,1.,1.,1.,1.,1.,1.,1.,1.,1.,1.,
1.,1.,1.,1.,1.,1.))
REPRESENTATION_ITEM('')
);
#367=(
BOUNDED_CURVE()
B_SPLINE_CURVE(5,(#52943,#52944,#52945,#52946,#52947,#52948,#52949,#52950,
#52951,#52952,#52953,#52954,#52955,#52956,#52957,#52958,#52959,#52960,#52961,
#52962,#52963,#52964,#52965,#52966,#52967,#52968,#52969,#52970,#52971,#52972,
#52973,#52974,#52975,#52976,#52977,#52978,#52979,#52980,#52981,#52982,#52983,
#52984,#52985,#52986,#52987,#52988,#52989,#52990,#52991,#52992,#52993,#52994,
#52995,#52996,#52997,#52998,#52999,#53000,#53001,#53002,#53003,#53004,#53005,
#53006,#53007,#53008,#53009,#53010,#53011,#53012),.UNSPECIFIED.,.F.,.F.)
B_SPLINE_CURVE_WITH_KNOTS((6,1,1,1,1,1,1,1,1,1,1,1,1,1,1,1,1,1,1,1,1,1,
1,1,1,1,1,1,1,1,1,1,1,1,1,1,1,1,1,1,1,1,1,1,1,1,1,1,1,1,1,1,1,1,1,1,1,1,
1,1,1,1,1,1,1,6),(-1.,-0.984615384615383,-0.969230769230768,-0.953846153846152,
-0.938461538461537,-0.923076923076922,-0.907692307692306,-0.892307692307691,
-0.876923076923076,-0.86153846153846,-0.846153846153845,-0.83076923076923,
-0.815384615384614,-0.799999999999999,-0.784615384615384,-0.769230769230768,
-0.753846153846153,-0.738461538461538,-0.723076923076922,-0.707692307692307,
-0.692307692307692,-0.676923076923076,-0.661538461538461,-0.646153846153846,
-0.63076923076923,-0.615384615384615,-0.6,-0.584615384615384,-0.569230769230769,
-0.553846153846154,-0.538461538461538,-0.523076923076923,-0.507692307692308,
-0.492307692307692,-0.476923076923077,-0.461538461538462,-0.446153846153846,
-0.430769230769231,-0.415384615384615,-0.4,-0.384615384615385,-0.369230769230769,
-0.353846153846154,-0.338461538461538,-0.323076923076923,-0.307692307692308,
-0.292307692307692,-0.276923076923077,-0.261538461538462,-0.246153846153846,
-0.230769230769231,-0.215384615384615,-0.2,-0.184615384615385,-0.169230769230769,
-0.153846153846154,-0.138461538461538,-0.123076923076923,-0.107692307692308,
-0.0923076923076923,-0.0769230769230769,-0.0615384615384615,-0.0461538461538462,
-0.0307692307692308,-0.0153846153846154,-0.00577184337450328),
 .UNSPECIFIED.)
CURVE()
GEOMETRIC_REPRESENTATION_ITEM()
RATIONAL_B_SPLINE_CURVE((1.,1.,1.,1.,1.,1.,1.,1.,1.,1.,1.,1.,1.,1.,1.,1.,
1.,1.,1.,1.,1.,1.,1.,1.,1.,1.,1.,1.,1.,1.,1.,1.,1.,1.,1.,1.,1.,1.,1.,1.,
1.,1.,1.,1.,1.,1.,1.,1.,1.,1.,1.,1.,1.,1.,1.,1.,1.,1.,1.,1.,1.,1.,1.,1.,
1.,1.,1.,1.,1.,1.))
REPRESENTATION_ITEM('')
);
#368=(
BOUNDED_CURVE()
B_SPLINE_CURVE(5,(#53165,#53166,#53167,#53168,#53169,#53170,#53171,#53172,
#53173,#53174,#53175,#53176,#53177,#53178,#53179,#53180,#53181,#53182,#53183,
#53184,#53185,#53186,#53187,#53188,#53189,#53190,#53191,#53192,#53193,#53194,
#53195,#53196,#53197,#53198,#53199,#53200,#53201,#53202,#53203,#53204,#53205,
#53206,#53207,#53208,#53209,#53210,#53211,#53212,#53213,#53214,#53215,#53216,
#53217,#53218,#53219,#53220,#53221,#53222,#53223,#53224,#53225,#53226,#53227,
#53228,#53229,#53230,#53231,#53232,#53233,#53234),.UNSPECIFIED.,.F.,.F.)
B_SPLINE_CURVE_WITH_KNOTS((6,1,1,1,1,1,1,1,1,1,1,1,1,1,1,1,1,1,1,1,1,1,
1,1,1,1,1,1,1,1,1,1,1,1,1,1,1,1,1,1,1,1,1,1,1,1,1,1,1,1,1,1,1,1,1,1,1,1,
1,1,1,1,1,1,1,6),(-0.994228156739672,-0.984615384615383,-0.969230769230768,
-0.953846153846152,-0.938461538461537,-0.923076923076922,-0.907692307692306,
-0.892307692307691,-0.876923076923076,-0.86153846153846,-0.846153846153845,
-0.83076923076923,-0.815384615384614,-0.799999999999999,-0.784615384615384,
-0.769230769230768,-0.753846153846153,-0.738461538461538,-0.723076923076922,
-0.707692307692307,-0.692307692307692,-0.676923076923076,-0.661538461538461,
-0.646153846153846,-0.63076923076923,-0.615384615384615,-0.6,-0.584615384615384,
-0.569230769230769,-0.553846153846154,-0.538461538461538,-0.523076923076923,
-0.507692307692308,-0.492307692307692,-0.476923076923077,-0.461538461538462,
-0.446153846153846,-0.430769230769231,-0.415384615384615,-0.4,-0.384615384615385,
-0.369230769230769,-0.353846153846154,-0.338461538461538,-0.323076923076923,
-0.307692307692308,-0.292307692307692,-0.276923076923077,-0.261538461538462,
-0.246153846153846,-0.230769230769231,-0.215384615384615,-0.2,-0.184615384615385,
-0.169230769230769,-0.153846153846154,-0.138461538461538,-0.123076923076923,
-0.107692307692308,-0.0923076923076923,-0.0769230769230769,-0.0615384615384615,
-0.0461538461538462,-0.0307692307692308,-0.0153846153846154,0.),
 .UNSPECIFIED.)
CURVE()
GEOMETRIC_REPRESENTATION_ITEM()
RATIONAL_B_SPLINE_CURVE((1.,1.,1.,1.,1.,1.,1.,1.,1.,1.,1.,1.,1.,1.,1.,1.,
1.,1.,1.,1.,1.,1.,1.,1.,1.,1.,1.,1.,1.,1.,1.,1.,1.,1.,1.,1.,1.,1.,1.,1.,
1.,1.,1.,1.,1.,1.,1.,1.,1.,1.,1.,1.,1.,1.,1.,1.,1.,1.,1.,1.,1.,1.,1.,1.,
1.,1.,1.,1.,1.,1.))
REPRESENTATION_ITEM('')
);
#369=(
BOUNDED_CURVE()
B_SPLINE_CURVE(5,(#53393,#53394,#53395,#53396,#53397,#53398,#53399,#53400,
#53401,#53402,#53403,#53404,#53405,#53406,#53407,#53408,#53409,#53410,#53411,
#53412,#53413,#53414,#53415,#53416,#53417,#53418,#53419,#53420,#53421,#53422,
#53423,#53424,#53425,#53426,#53427,#53428,#53429,#53430,#53431,#53432,#53433,
#53434,#53435,#53436,#53437,#53438,#53439,#53440,#53441,#53442,#53443,#53444,
#53445,#53446,#53447,#53448,#53449,#53450,#53451,#53452,#53453,#53454,#53455,
#53456,#53457,#53458,#53459,#53460,#53461,#53462),.UNSPECIFIED.,.F.,.F.)
B_SPLINE_CURVE_WITH_KNOTS((6,1,1,1,1,1,1,1,1,1,1,1,1,1,1,1,1,1,1,1,1,1,
1,1,1,1,1,1,1,1,1,1,1,1,1,1,1,1,1,1,1,1,1,1,1,1,1,1,1,1,1,1,1,1,1,1,1,1,
1,1,1,1,1,1,1,6),(-0.994228156739704,-0.984615384615383,-0.969230769230768,
-0.953846153846152,-0.938461538461537,-0.923076923076922,-0.907692307692306,
-0.892307692307691,-0.876923076923076,-0.86153846153846,-0.846153846153845,
-0.83076923076923,-0.815384615384614,-0.799999999999999,-0.784615384615384,
-0.769230769230768,-0.753846153846153,-0.738461538461538,-0.723076923076922,
-0.707692307692307,-0.692307692307692,-0.676923076923076,-0.661538461538461,
-0.646153846153846,-0.63076923076923,-0.615384615384615,-0.6,-0.584615384615384,
-0.569230769230769,-0.553846153846154,-0.538461538461538,-0.523076923076923,
-0.507692307692308,-0.492307692307692,-0.476923076923077,-0.461538461538462,
-0.446153846153846,-0.430769230769231,-0.415384615384615,-0.4,-0.384615384615385,
-0.369230769230769,-0.353846153846154,-0.338461538461538,-0.323076923076923,
-0.307692307692308,-0.292307692307692,-0.276923076923077,-0.261538461538462,
-0.246153846153846,-0.230769230769231,-0.215384615384615,-0.2,-0.184615384615385,
-0.169230769230769,-0.153846153846154,-0.138461538461538,-0.123076923076923,
-0.107692307692308,-0.0923076923076923,-0.0769230769230769,-0.0615384615384615,
-0.0461538461538462,-0.0307692307692308,-0.0153846153846154,0.),
 .UNSPECIFIED.)
CURVE()
GEOMETRIC_REPRESENTATION_ITEM()
RATIONAL_B_SPLINE_CURVE((1.,1.,1.,1.,1.,1.,1.,1.,1.,1.,1.,1.,1.,1.,1.,1.,
1.,1.,1.,1.,1.,1.,1.,1.,1.,1.,1.,1.,1.,1.,1.,1.,1.,1.,1.,1.,1.,1.,1.,1.,
1.,1.,1.,1.,1.,1.,1.,1.,1.,1.,1.,1.,1.,1.,1.,1.,1.,1.,1.,1.,1.,1.,1.,1.,
1.,1.,1.,1.,1.,1.))
REPRESENTATION_ITEM('')
);
#370=(
BOUNDED_CURVE()
B_SPLINE_CURVE(5,(#53604,#53605,#53606,#53607,#53608,#53609,#53610,#53611,
#53612,#53613,#53614,#53615,#53616,#53617,#53618,#53619,#53620,#53621,#53622,
#53623,#53624,#53625,#53626,#53627,#53628,#53629,#53630,#53631,#53632,#53633,
#53634,#53635,#53636,#53637,#53638,#53639,#53640,#53641,#53642,#53643,#53644,
#53645,#53646,#53647,#53648,#53649,#53650,#53651,#53652,#53653,#53654,#53655,
#53656,#53657,#53658,#53659,#53660,#53661,#53662,#53663,#53664,#53665,#53666,
#53667,#53668,#53669,#53670,#53671,#53672,#53673),.UNSPECIFIED.,.F.,.F.)
B_SPLINE_CURVE_WITH_KNOTS((6,1,1,1,1,1,1,1,1,1,1,1,1,1,1,1,1,1,1,1,1,1,
1,1,1,1,1,1,1,1,1,1,1,1,1,1,1,1,1,1,1,1,1,1,1,1,1,1,1,1,1,1,1,1,1,1,1,1,
1,1,1,1,1,1,1,6),(-1.,-0.984615384615383,-0.969230769230768,-0.953846153846152,
-0.938461538461537,-0.923076923076922,-0.907692307692306,-0.892307692307691,
-0.876923076923076,-0.86153846153846,-0.846153846153845,-0.83076923076923,
-0.815384615384614,-0.799999999999999,-0.784615384615384,-0.769230769230768,
-0.753846153846153,-0.738461538461538,-0.723076923076922,-0.707692307692307,
-0.692307692307692,-0.676923076923076,-0.661538461538461,-0.646153846153846,
-0.63076923076923,-0.615384615384615,-0.6,-0.584615384615384,-0.569230769230769,
-0.553846153846154,-0.538461538461538,-0.523076923076923,-0.507692307692308,
-0.492307692307692,-0.476923076923077,-0.461538461538462,-0.446153846153846,
-0.430769230769231,-0.415384615384615,-0.4,-0.384615384615385,-0.369230769230769,
-0.353846153846154,-0.338461538461538,-0.323076923076923,-0.307692307692308,
-0.292307692307692,-0.276923076923077,-0.261538461538462,-0.246153846153846,
-0.230769230769231,-0.215384615384615,-0.2,-0.184615384615385,-0.169230769230769,
-0.153846153846154,-0.138461538461538,-0.123076923076923,-0.107692307692308,
-0.0923076923076923,-0.0769230769230769,-0.0615384615384615,-0.0461538461538462,
-0.0307692307692308,-0.0153846153846154,-0.00577184337451611),
 .UNSPECIFIED.)
CURVE()
GEOMETRIC_REPRESENTATION_ITEM()
RATIONAL_B_SPLINE_CURVE((1.,1.,1.,1.,1.,1.,1.,1.,1.,1.,1.,1.,1.,1.,1.,1.,
1.,1.,1.,1.,1.,1.,1.,1.,1.,1.,1.,1.,1.,1.,1.,1.,1.,1.,1.,1.,1.,1.,1.,1.,
1.,1.,1.,1.,1.,1.,1.,1.,1.,1.,1.,1.,1.,1.,1.,1.,1.,1.,1.,1.,1.,1.,1.,1.,
1.,1.,1.,1.,1.,1.))
REPRESENTATION_ITEM('')
);
#715=B_SPLINE_CURVE_WITH_KNOTS('',3,(#36140,#36141,#36142,#36143,#36144,
#36145),.UNSPECIFIED.,.F.,.F.,(4,2,4),(0.,1.,2.),.UNSPECIFIED.);
#716=B_SPLINE_CURVE_WITH_KNOTS('',3,(#36359,#36360,#36361,#36362,#36363,
#36364),.UNSPECIFIED.,.F.,.F.,(4,2,4),(0.,1.,2.),.UNSPECIFIED.);
#717=B_SPLINE_CURVE_WITH_KNOTS('',3,(#36442,#36443,#36444,#36445,#36446,
#36447),.UNSPECIFIED.,.F.,.F.,(4,2,4),(0.,1.,2.),.UNSPECIFIED.);
#718=B_SPLINE_CURVE_WITH_KNOTS('',3,(#36801,#36802,#36803,#36804,#36805,
#36806),.UNSPECIFIED.,.F.,.F.,(4,2,4),(0.,1.,2.),.UNSPECIFIED.);
#719=B_SPLINE_CURVE_WITH_KNOTS('',3,(#36884,#36885,#36886,#36887,#36888,
#36889),.UNSPECIFIED.,.F.,.F.,(4,2,4),(0.,1.,2.),.UNSPECIFIED.);
#720=B_SPLINE_CURVE_WITH_KNOTS('',3,(#37243,#37244,#37245,#37246,#37247,
#37248),.UNSPECIFIED.,.F.,.F.,(4,2,4),(0.,1.,2.),.UNSPECIFIED.);
#721=B_SPLINE_CURVE_WITH_KNOTS('',3,(#37326,#37327,#37328,#37329,#37330,
#37331),.UNSPECIFIED.,.F.,.F.,(4,2,4),(0.,1.,2.),.UNSPECIFIED.);
#722=B_SPLINE_CURVE_WITH_KNOTS('',3,(#37685,#37686,#37687,#37688,#37689,
#37690),.UNSPECIFIED.,.F.,.F.,(4,2,4),(0.,1.,2.),.UNSPECIFIED.);
#723=B_SPLINE_CURVE_WITH_KNOTS('',3,(#37768,#37769,#37770,#37771,#37772,
#37773),.UNSPECIFIED.,.F.,.F.,(4,2,4),(0.,1.,2.),.UNSPECIFIED.);
#724=B_SPLINE_CURVE_WITH_KNOTS('',3,(#38127,#38128,#38129,#38130,#38131,
#38132),.UNSPECIFIED.,.F.,.F.,(4,2,4),(0.,1.,2.),.UNSPECIFIED.);
#725=B_SPLINE_CURVE_WITH_KNOTS('',3,(#38210,#38211,#38212,#38213,#38214,
#38215),.UNSPECIFIED.,.F.,.F.,(4,2,4),(0.,1.,2.),.UNSPECIFIED.);
#726=B_SPLINE_CURVE_WITH_KNOTS('',3,(#38569,#38570,#38571,#38572,#38573,
#38574),.UNSPECIFIED.,.F.,.F.,(4,2,4),(0.,1.,2.),.UNSPECIFIED.);
#727=B_SPLINE_CURVE_WITH_KNOTS('',3,(#38652,#38653,#38654,#38655,#38656,
#38657),.UNSPECIFIED.,.F.,.F.,(4,2,4),(0.,1.,2.),.UNSPECIFIED.);
#728=B_SPLINE_CURVE_WITH_KNOTS('',3,(#39011,#39012,#39013,#39014,#39015,
#39016),.UNSPECIFIED.,.F.,.F.,(4,2,4),(0.,1.,2.),.UNSPECIFIED.);
#729=B_SPLINE_CURVE_WITH_KNOTS('',3,(#39094,#39095,#39096,#39097,#39098,
#39099),.UNSPECIFIED.,.F.,.F.,(4,2,4),(0.,1.,2.),.UNSPECIFIED.);
#730=B_SPLINE_CURVE_WITH_KNOTS('',3,(#39453,#39454,#39455,#39456,#39457,
#39458),.UNSPECIFIED.,.F.,.F.,(4,2,4),(0.,1.,2.),.UNSPECIFIED.);
#731=B_SPLINE_CURVE_WITH_KNOTS('',3,(#39536,#39537,#39538,#39539,#39540,
#39541),.UNSPECIFIED.,.F.,.F.,(4,2,4),(0.,1.,2.),.UNSPECIFIED.);
#732=B_SPLINE_CURVE_WITH_KNOTS('',3,(#39895,#39896,#39897,#39898,#39899,
#39900),.UNSPECIFIED.,.F.,.F.,(4,2,4),(0.,1.,2.),.UNSPECIFIED.);
#733=B_SPLINE_CURVE_WITH_KNOTS('',3,(#39978,#39979,#39980,#39981,#39982,
#39983),.UNSPECIFIED.,.F.,.F.,(4,2,4),(0.,1.,2.),.UNSPECIFIED.);
#734=B_SPLINE_CURVE_WITH_KNOTS('',3,(#40337,#40338,#40339,#40340,#40341,
#40342),.UNSPECIFIED.,.F.,.F.,(4,2,4),(0.,1.,2.),.UNSPECIFIED.);
#735=B_SPLINE_CURVE_WITH_KNOTS('',3,(#40420,#40421,#40422,#40423,#40424,
#40425),.UNSPECIFIED.,.F.,.F.,(4,2,4),(0.,1.,2.),.UNSPECIFIED.);
#736=B_SPLINE_CURVE_WITH_KNOTS('',3,(#40779,#40780,#40781,#40782,#40783,
#40784),.UNSPECIFIED.,.F.,.F.,(4,2,4),(0.,1.,2.),.UNSPECIFIED.);
#737=B_SPLINE_CURVE_WITH_KNOTS('',3,(#40862,#40863,#40864,#40865,#40866,
#40867),.UNSPECIFIED.,.F.,.F.,(4,2,4),(0.,1.,2.),.UNSPECIFIED.);
#738=B_SPLINE_CURVE_WITH_KNOTS('',3,(#41221,#41222,#41223,#41224,#41225,
#41226),.UNSPECIFIED.,.F.,.F.,(4,2,4),(0.,1.,2.),.UNSPECIFIED.);
#739=B_SPLINE_CURVE_WITH_KNOTS('',3,(#41304,#41305,#41306,#41307,#41308,
#41309),.UNSPECIFIED.,.F.,.F.,(4,2,4),(0.,1.,2.),.UNSPECIFIED.);
#740=B_SPLINE_CURVE_WITH_KNOTS('',3,(#41663,#41664,#41665,#41666,#41667,
#41668),.UNSPECIFIED.,.F.,.F.,(4,2,4),(0.,1.,2.),.UNSPECIFIED.);
#741=B_SPLINE_CURVE_WITH_KNOTS('',3,(#41746,#41747,#41748,#41749,#41750,
#41751),.UNSPECIFIED.,.F.,.F.,(4,2,4),(0.,1.,2.),.UNSPECIFIED.);
#742=B_SPLINE_CURVE_WITH_KNOTS('',3,(#42105,#42106,#42107,#42108,#42109,
#42110),.UNSPECIFIED.,.F.,.F.,(4,2,4),(0.,1.,2.),.UNSPECIFIED.);
#743=B_SPLINE_CURVE_WITH_KNOTS('',3,(#42188,#42189,#42190,#42191,#42192,
#42193),.UNSPECIFIED.,.F.,.F.,(4,2,4),(0.,1.,2.),.UNSPECIFIED.);
#744=B_SPLINE_CURVE_WITH_KNOTS('',3,(#42547,#42548,#42549,#42550,#42551,
#42552),.UNSPECIFIED.,.F.,.F.,(4,2,4),(0.,1.,2.),.UNSPECIFIED.);
#745=B_SPLINE_CURVE_WITH_KNOTS('',3,(#42630,#42631,#42632,#42633,#42634,
#42635),.UNSPECIFIED.,.F.,.F.,(4,2,4),(0.,1.,2.),.UNSPECIFIED.);
#746=B_SPLINE_CURVE_WITH_KNOTS('',3,(#42989,#42990,#42991,#42992,#42993,
#42994),.UNSPECIFIED.,.F.,.F.,(4,2,4),(0.,1.,2.),.UNSPECIFIED.);
#747=B_SPLINE_CURVE_WITH_KNOTS('',3,(#43072,#43073,#43074,#43075,#43076,
#43077),.UNSPECIFIED.,.F.,.F.,(4,2,4),(0.,1.,2.),.UNSPECIFIED.);
#748=B_SPLINE_CURVE_WITH_KNOTS('',3,(#43431,#43432,#43433,#43434,#43435,
#43436),.UNSPECIFIED.,.F.,.F.,(4,2,4),(0.,1.,2.),.UNSPECIFIED.);
#749=B_SPLINE_CURVE_WITH_KNOTS('',3,(#43514,#43515,#43516,#43517,#43518,
#43519),.UNSPECIFIED.,.F.,.F.,(4,2,4),(0.,1.,2.),.UNSPECIFIED.);
#750=B_SPLINE_CURVE_WITH_KNOTS('',3,(#43873,#43874,#43875,#43876,#43877,
#43878),.UNSPECIFIED.,.F.,.F.,(4,2,4),(0.,1.,2.),.UNSPECIFIED.);
#751=B_SPLINE_CURVE_WITH_KNOTS('',3,(#43956,#43957,#43958,#43959,#43960,
#43961),.UNSPECIFIED.,.F.,.F.,(4,2,4),(0.,1.,2.),.UNSPECIFIED.);
#752=B_SPLINE_CURVE_WITH_KNOTS('',3,(#44315,#44316,#44317,#44318,#44319,
#44320),.UNSPECIFIED.,.F.,.F.,(4,2,4),(0.,1.,2.),.UNSPECIFIED.);
#753=B_SPLINE_CURVE_WITH_KNOTS('',3,(#44398,#44399,#44400,#44401,#44402,
#44403),.UNSPECIFIED.,.F.,.F.,(4,2,4),(0.,1.,2.),.UNSPECIFIED.);
#754=B_SPLINE_CURVE_WITH_KNOTS('',3,(#44757,#44758,#44759,#44760,#44761,
#44762),.UNSPECIFIED.,.F.,.F.,(4,2,4),(0.,1.,2.),.UNSPECIFIED.);
#755=B_SPLINE_CURVE_WITH_KNOTS('',3,(#44840,#44841,#44842,#44843,#44844,
#44845),.UNSPECIFIED.,.F.,.F.,(4,2,4),(0.,1.,2.),.UNSPECIFIED.);
#756=B_SPLINE_CURVE_WITH_KNOTS('',3,(#45199,#45200,#45201,#45202,#45203,
#45204),.UNSPECIFIED.,.F.,.F.,(4,2,4),(0.,1.,2.),.UNSPECIFIED.);
#757=B_SPLINE_CURVE_WITH_KNOTS('',3,(#45282,#45283,#45284,#45285,#45286,
#45287),.UNSPECIFIED.,.F.,.F.,(4,2,4),(0.,1.,2.),.UNSPECIFIED.);
#758=B_SPLINE_CURVE_WITH_KNOTS('',3,(#45641,#45642,#45643,#45644,#45645,
#45646),.UNSPECIFIED.,.F.,.F.,(4,2,4),(0.,1.,2.),.UNSPECIFIED.);
#759=B_SPLINE_CURVE_WITH_KNOTS('',3,(#45724,#45725,#45726,#45727,#45728,
#45729),.UNSPECIFIED.,.F.,.F.,(4,2,4),(0.,1.,2.),.UNSPECIFIED.);
#760=B_SPLINE_CURVE_WITH_KNOTS('',3,(#46083,#46084,#46085,#46086,#46087,
#46088),.UNSPECIFIED.,.F.,.F.,(4,2,4),(0.,1.,2.),.UNSPECIFIED.);
#761=B_SPLINE_CURVE_WITH_KNOTS('',3,(#46166,#46167,#46168,#46169,#46170,
#46171),.UNSPECIFIED.,.F.,.F.,(4,2,4),(0.,1.,2.),.UNSPECIFIED.);
#762=B_SPLINE_CURVE_WITH_KNOTS('',3,(#46525,#46526,#46527,#46528,#46529,
#46530),.UNSPECIFIED.,.F.,.F.,(4,2,4),(0.,1.,2.),.UNSPECIFIED.);
#763=B_SPLINE_CURVE_WITH_KNOTS('',3,(#46608,#46609,#46610,#46611,#46612,
#46613),.UNSPECIFIED.,.F.,.F.,(4,2,4),(0.,1.,2.),.UNSPECIFIED.);
#764=B_SPLINE_CURVE_WITH_KNOTS('',3,(#46967,#46968,#46969,#46970,#46971,
#46972),.UNSPECIFIED.,.F.,.F.,(4,2,4),(0.,1.,2.),.UNSPECIFIED.);
#765=B_SPLINE_CURVE_WITH_KNOTS('',3,(#47050,#47051,#47052,#47053,#47054,
#47055),.UNSPECIFIED.,.F.,.F.,(4,2,4),(0.,1.,2.),.UNSPECIFIED.);
#766=B_SPLINE_CURVE_WITH_KNOTS('',3,(#47409,#47410,#47411,#47412,#47413,
#47414),.UNSPECIFIED.,.F.,.F.,(4,2,4),(0.,1.,2.),.UNSPECIFIED.);
#767=B_SPLINE_CURVE_WITH_KNOTS('',3,(#47492,#47493,#47494,#47495,#47496,
#47497),.UNSPECIFIED.,.F.,.F.,(4,2,4),(0.,1.,2.),.UNSPECIFIED.);
#768=B_SPLINE_CURVE_WITH_KNOTS('',3,(#47851,#47852,#47853,#47854,#47855,
#47856),.UNSPECIFIED.,.F.,.F.,(4,2,4),(0.,1.,2.),.UNSPECIFIED.);
#769=B_SPLINE_CURVE_WITH_KNOTS('',3,(#47934,#47935,#47936,#47937,#47938,
#47939),.UNSPECIFIED.,.F.,.F.,(4,2,4),(0.,1.,2.),.UNSPECIFIED.);
#770=B_SPLINE_CURVE_WITH_KNOTS('',3,(#48293,#48294,#48295,#48296,#48297,
#48298),.UNSPECIFIED.,.F.,.F.,(4,2,4),(0.,1.,2.),.UNSPECIFIED.);
#771=B_SPLINE_CURVE_WITH_KNOTS('',3,(#48376,#48377,#48378,#48379,#48380,
#48381),.UNSPECIFIED.,.F.,.F.,(4,2,4),(0.,1.,2.),.UNSPECIFIED.);
#772=B_SPLINE_CURVE_WITH_KNOTS('',3,(#48735,#48736,#48737,#48738,#48739,
#48740),.UNSPECIFIED.,.F.,.F.,(4,2,4),(0.,1.,2.),.UNSPECIFIED.);
#773=B_SPLINE_CURVE_WITH_KNOTS('',3,(#48818,#48819,#48820,#48821,#48822,
#48823),.UNSPECIFIED.,.F.,.F.,(4,2,4),(0.,1.,2.),.UNSPECIFIED.);
#774=B_SPLINE_CURVE_WITH_KNOTS('',3,(#49177,#49178,#49179,#49180,#49181,
#49182),.UNSPECIFIED.,.F.,.F.,(4,2,4),(0.,1.,2.),.UNSPECIFIED.);
#775=B_SPLINE_CURVE_WITH_KNOTS('',3,(#49260,#49261,#49262,#49263,#49264,
#49265),.UNSPECIFIED.,.F.,.F.,(4,2,4),(0.,1.,2.),.UNSPECIFIED.);
#776=B_SPLINE_CURVE_WITH_KNOTS('',3,(#49619,#49620,#49621,#49622,#49623,
#49624),.UNSPECIFIED.,.F.,.F.,(4,2,4),(0.,1.,2.),.UNSPECIFIED.);
#777=B_SPLINE_CURVE_WITH_KNOTS('',3,(#49702,#49703,#49704,#49705,#49706,
#49707),.UNSPECIFIED.,.F.,.F.,(4,2,4),(0.,1.,2.),.UNSPECIFIED.);
#778=B_SPLINE_CURVE_WITH_KNOTS('',3,(#50061,#50062,#50063,#50064,#50065,
#50066),.UNSPECIFIED.,.F.,.F.,(4,2,4),(0.,1.,2.),.UNSPECIFIED.);
#779=B_SPLINE_CURVE_WITH_KNOTS('',3,(#50144,#50145,#50146,#50147,#50148,
#50149),.UNSPECIFIED.,.F.,.F.,(4,2,4),(0.,1.,2.),.UNSPECIFIED.);
#780=B_SPLINE_CURVE_WITH_KNOTS('',3,(#50503,#50504,#50505,#50506,#50507,
#50508),.UNSPECIFIED.,.F.,.F.,(4,2,4),(0.,1.,2.),.UNSPECIFIED.);
#781=B_SPLINE_CURVE_WITH_KNOTS('',3,(#50586,#50587,#50588,#50589,#50590,
#50591),.UNSPECIFIED.,.F.,.F.,(4,2,4),(0.,1.,2.),.UNSPECIFIED.);
#782=B_SPLINE_CURVE_WITH_KNOTS('',3,(#50945,#50946,#50947,#50948,#50949,
#50950),.UNSPECIFIED.,.F.,.F.,(4,2,4),(0.,1.,2.),.UNSPECIFIED.);
#783=B_SPLINE_CURVE_WITH_KNOTS('',3,(#51028,#51029,#51030,#51031,#51032,
#51033),.UNSPECIFIED.,.F.,.F.,(4,2,4),(0.,1.,2.),.UNSPECIFIED.);
#784=B_SPLINE_CURVE_WITH_KNOTS('',3,(#51387,#51388,#51389,#51390,#51391,
#51392),.UNSPECIFIED.,.F.,.F.,(4,2,4),(0.,1.,2.),.UNSPECIFIED.);
#785=B_SPLINE_CURVE_WITH_KNOTS('',3,(#51470,#51471,#51472,#51473,#51474,
#51475),.UNSPECIFIED.,.F.,.F.,(4,2,4),(0.,1.,2.),.UNSPECIFIED.);
#786=B_SPLINE_CURVE_WITH_KNOTS('',3,(#51829,#51830,#51831,#51832,#51833,
#51834),.UNSPECIFIED.,.F.,.F.,(4,2,4),(0.,1.,2.),.UNSPECIFIED.);
#787=B_SPLINE_CURVE_WITH_KNOTS('',3,(#51912,#51913,#51914,#51915,#51916,
#51917),.UNSPECIFIED.,.F.,.F.,(4,2,4),(0.,1.,2.),.UNSPECIFIED.);
#788=B_SPLINE_CURVE_WITH_KNOTS('',3,(#52271,#52272,#52273,#52274,#52275,
#52276),.UNSPECIFIED.,.F.,.F.,(4,2,4),(0.,1.,2.),.UNSPECIFIED.);
#789=B_SPLINE_CURVE_WITH_KNOTS('',3,(#52354,#52355,#52356,#52357,#52358,
#52359),.UNSPECIFIED.,.F.,.F.,(4,2,4),(0.,1.,2.),.UNSPECIFIED.);
#790=B_SPLINE_CURVE_WITH_KNOTS('',3,(#52713,#52714,#52715,#52716,#52717,
#52718),.UNSPECIFIED.,.F.,.F.,(4,2,4),(0.,1.,2.),.UNSPECIFIED.);
#791=B_SPLINE_CURVE_WITH_KNOTS('',3,(#52796,#52797,#52798,#52799,#52800,
#52801),.UNSPECIFIED.,.F.,.F.,(4,2,4),(0.,1.,2.),.UNSPECIFIED.);
#792=B_SPLINE_CURVE_WITH_KNOTS('',3,(#53159,#53160,#53161,#53162,#53163,
#53164),.UNSPECIFIED.,.F.,.F.,(4,2,4),(0.,1.,2.),.UNSPECIFIED.);
#793=B_SPLINE_CURVE_WITH_KNOTS('',3,(#53238,#53239,#53240,#53241,#53242,
#53243),.UNSPECIFIED.,.F.,.F.,(4,2,4),(0.,1.,2.),.UNSPECIFIED.);
#794=B_SPLINE_CURVE_WITH_KNOTS('',3,(#53385,#53386,#53387,#53388,#53389,
#53390),.UNSPECIFIED.,.F.,.F.,(4,2,4),(0.,1.,2.),.UNSPECIFIED.);
#901=SHAPE_REPRESENTATION_RELATIONSHIP('SRR','None',#54132,#944);
#944=ADVANCED_BREP_SHAPE_REPRESENTATION('',(#1057),#53906);
#1002=STYLED_ITEM('',(#54390),#1057);
#1057=MANIFOLD_SOLID_BREP('Body1',#11329);
#1234=FACE_BOUND('',#2787,.T.);
#1235=FACE_BOUND('',#2791,.T.);
#1236=FACE_BOUND('',#2952,.T.);
#1438=PLANE('',#12757);
#1439=PLANE('',#12758);
#1440=PLANE('',#12759);
#1441=PLANE('',#12760);
#1442=PLANE('',#12807);
#1443=PLANE('',#12808);
#1444=PLANE('',#12811);
#1445=PLANE('',#12814);
#1446=PLANE('',#12817);
#1447=PLANE('',#12820);
#1448=PLANE('',#12823);
#1449=PLANE('',#12826);
#1450=PLANE('',#12829);
#1451=PLANE('',#12832);
#1452=PLANE('',#12835);
#1453=PLANE('',#12838);
#1454=PLANE('',#12841);
#1455=PLANE('',#12844);
#1456=PLANE('',#12847);
#1457=PLANE('',#12850);
#1458=PLANE('',#12853);
#1459=PLANE('',#12856);
#1460=PLANE('',#12859);
#1461=PLANE('',#12862);
#1462=PLANE('',#12865);
#1463=PLANE('',#12868);
#1464=PLANE('',#12871);
#1465=PLANE('',#12874);
#1466=PLANE('',#12877);
#1467=PLANE('',#12880);
#1468=PLANE('',#12883);
#1469=PLANE('',#12886);
#1470=PLANE('',#12889);
#1471=PLANE('',#12892);
#1472=PLANE('',#12895);
#1473=PLANE('',#12898);
#1474=PLANE('',#12901);
#1475=PLANE('',#12904);
#1476=PLANE('',#12907);
#1477=PLANE('',#12910);
#1478=PLANE('',#12913);
#1479=PLANE('',#12916);
#1480=PLANE('',#12919);
#1481=PLANE('',#12922);
#1482=PLANE('',#12925);
#1483=PLANE('',#12926);
#1961=FACE_OUTER_BOUND('',#2783,.T.);
#1962=FACE_OUTER_BOUND('',#2784,.T.);
#1963=FACE_OUTER_BOUND('',#2785,.T.);
#1964=FACE_OUTER_BOUND('',#2786,.T.);
#1965=FACE_OUTER_BOUND('',#2788,.T.);
#1966=FACE_OUTER_BOUND('',#2789,.T.);
#1967=FACE_OUTER_BOUND('',#2790,.T.);
#1968=FACE_OUTER_BOUND('',#2792,.T.);
#1969=FACE_OUTER_BOUND('',#2793,.T.);
#1970=FACE_OUTER_BOUND('',#2794,.T.);
#1971=FACE_OUTER_BOUND('',#2795,.T.);
#1972=FACE_OUTER_BOUND('',#2796,.T.);
#1973=FACE_OUTER_BOUND('',#2797,.T.);
#1974=FACE_OUTER_BOUND('',#2798,.T.);
#1975=FACE_OUTER_BOUND('',#2799,.T.);
#1976=FACE_OUTER_BOUND('',#2800,.T.);
#1977=FACE_OUTER_BOUND('',#2801,.T.);
#1978=FACE_OUTER_BOUND('',#2802,.T.);
#1979=FACE_OUTER_BOUND('',#2803,.T.);
#1980=FACE_OUTER_BOUND('',#2804,.T.);
#1981=FACE_OUTER_BOUND('',#2805,.T.);
#1982=FACE_OUTER_BOUND('',#2806,.T.);
#1983=FACE_OUTER_BOUND('',#2807,.T.);
#1984=FACE_OUTER_BOUND('',#2808,.T.);
#1985=FACE_OUTER_BOUND('',#2809,.T.);
#1986=FACE_OUTER_BOUND('',#2810,.T.);
#1987=FACE_OUTER_BOUND('',#2811,.T.);
#1988=FACE_OUTER_BOUND('',#2812,.T.);
#1989=FACE_OUTER_BOUND('',#2813,.T.);
#1990=FACE_OUTER_BOUND('',#2814,.T.);
#1991=FACE_OUTER_BOUND('',#2815,.T.);
#1992=FACE_OUTER_BOUND('',#2816,.T.);
#1993=FACE_OUTER_BOUND('',#2817,.T.);
#1994=FACE_OUTER_BOUND('',#2818,.T.);
#1995=FACE_OUTER_BOUND('',#2819,.T.);
#1996=FACE_OUTER_BOUND('',#2820,.T.);
#1997=FACE_OUTER_BOUND('',#2821,.T.);
#1998=FACE_OUTER_BOUND('',#2822,.T.);
#1999=FACE_OUTER_BOUND('',#2823,.T.);
#2000=FACE_OUTER_BOUND('',#2824,.T.);
#2001=FACE_OUTER_BOUND('',#2825,.T.);
#2002=FACE_OUTER_BOUND('',#2826,.T.);
#2003=FACE_OUTER_BOUND('',#2827,.T.);
#2004=FACE_OUTER_BOUND('',#2828,.T.);
#2005=FACE_OUTER_BOUND('',#2829,.T.);
#2006=FACE_OUTER_BOUND('',#2830,.T.);
#2007=FACE_OUTER_BOUND('',#2831,.T.);
#2008=FACE_OUTER_BOUND('',#2832,.T.);
#2009=FACE_OUTER_BOUND('',#2833,.T.);
#2010=FACE_OUTER_BOUND('',#2834,.T.);
#2011=FACE_OUTER_BOUND('',#2835,.T.);
#2012=FACE_OUTER_BOUND('',#2836,.T.);
#2013=FACE_OUTER_BOUND('',#2837,.T.);
#2014=FACE_OUTER_BOUND('',#2838,.T.);
#2015=FACE_OUTER_BOUND('',#2839,.T.);
#2016=FACE_OUTER_BOUND('',#2840,.T.);
#2017=FACE_OUTER_BOUND('',#2841,.T.);
#2018=FACE_OUTER_BOUND('',#2842,.T.);
#2019=FACE_OUTER_BOUND('',#2843,.T.);
#2020=FACE_OUTER_BOUND('',#2844,.T.);
#2021=FACE_OUTER_BOUND('',#2845,.T.);
#2022=FACE_OUTER_BOUND('',#2846,.T.);
#2023=FACE_OUTER_BOUND('',#2847,.T.);
#2024=FACE_OUTER_BOUND('',#2848,.T.);
#2025=FACE_OUTER_BOUND('',#2849,.T.);
#2026=FACE_OUTER_BOUND('',#2850,.T.);
#2027=FACE_OUTER_BOUND('',#2851,.T.);
#2028=FACE_OUTER_BOUND('',#2852,.T.);
#2029=FACE_OUTER_BOUND('',#2853,.T.);
#2030=FACE_OUTER_BOUND('',#2854,.T.);
#2031=FACE_OUTER_BOUND('',#2855,.T.);
#2032=FACE_OUTER_BOUND('',#2856,.T.);
#2033=FACE_OUTER_BOUND('',#2857,.T.);
#2034=FACE_OUTER_BOUND('',#2858,.T.);
#2035=FACE_OUTER_BOUND('',#2859,.T.);
#2036=FACE_OUTER_BOUND('',#2860,.T.);
#2037=FACE_OUTER_BOUND('',#2861,.T.);
#2038=FACE_OUTER_BOUND('',#2862,.T.);
#2039=FACE_OUTER_BOUND('',#2863,.T.);
#2040=FACE_OUTER_BOUND('',#2864,.T.);
#2041=FACE_OUTER_BOUND('',#2865,.T.);
#2042=FACE_OUTER_BOUND('',#2866,.T.);
#2043=FACE_OUTER_BOUND('',#2867,.T.);
#2044=FACE_OUTER_BOUND('',#2868,.T.);
#2045=FACE_OUTER_BOUND('',#2869,.T.);
#2046=FACE_OUTER_BOUND('',#2870,.T.);
#2047=FACE_OUTER_BOUND('',#2871,.T.);
#2048=FACE_OUTER_BOUND('',#2872,.T.);
#2049=FACE_OUTER_BOUND('',#2873,.T.);
#2050=FACE_OUTER_BOUND('',#2874,.T.);
#2051=FACE_OUTER_BOUND('',#2875,.T.);
#2052=FACE_OUTER_BOUND('',#2876,.T.);
#2053=FACE_OUTER_BOUND('',#2877,.T.);
#2054=FACE_OUTER_BOUND('',#2878,.T.);
#2055=FACE_OUTER_BOUND('',#2879,.T.);
#2056=FACE_OUTER_BOUND('',#2880,.T.);
#2057=FACE_OUTER_BOUND('',#2881,.T.);
#2058=FACE_OUTER_BOUND('',#2882,.T.);
#2059=FACE_OUTER_BOUND('',#2883,.T.);
#2060=FACE_OUTER_BOUND('',#2884,.T.);
#2061=FACE_OUTER_BOUND('',#2885,.T.);
#2062=FACE_OUTER_BOUND('',#2886,.T.);
#2063=FACE_OUTER_BOUND('',#2887,.T.);
#2064=FACE_OUTER_BOUND('',#2888,.T.);
#2065=FACE_OUTER_BOUND('',#2889,.T.);
#2066=FACE_OUTER_BOUND('',#2890,.T.);
#2067=FACE_OUTER_BOUND('',#2891,.T.);
#2068=FACE_OUTER_BOUND('',#2892,.T.);
#2069=FACE_OUTER_BOUND('',#2893,.T.);
#2070=FACE_OUTER_BOUND('',#2894,.T.);
#2071=FACE_OUTER_BOUND('',#2895,.T.);
#2072=FACE_OUTER_BOUND('',#2896,.T.);
#2073=FACE_OUTER_BOUND('',#2897,.T.);
#2074=FACE_OUTER_BOUND('',#2898,.T.);
#2075=FACE_OUTER_BOUND('',#2899,.T.);
#2076=FACE_OUTER_BOUND('',#2900,.T.);
#2077=FACE_OUTER_BOUND('',#2901,.T.);
#2078=FACE_OUTER_BOUND('',#2902,.T.);
#2079=FACE_OUTER_BOUND('',#2903,.T.);
#2080=FACE_OUTER_BOUND('',#2904,.T.);
#2081=FACE_OUTER_BOUND('',#2905,.T.);
#2082=FACE_OUTER_BOUND('',#2906,.T.);
#2083=FACE_OUTER_BOUND('',#2907,.T.);
#2084=FACE_OUTER_BOUND('',#2908,.T.);
#2085=FACE_OUTER_BOUND('',#2909,.T.);
#2086=FACE_OUTER_BOUND('',#2910,.T.);
#2087=FACE_OUTER_BOUND('',#2911,.T.);
#2088=FACE_OUTER_BOUND('',#2912,.T.);
#2089=FACE_OUTER_BOUND('',#2913,.T.);
#2090=FACE_OUTER_BOUND('',#2914,.T.);
#2091=FACE_OUTER_BOUND('',#2915,.T.);
#2092=FACE_OUTER_BOUND('',#2916,.T.);
#2093=FACE_OUTER_BOUND('',#2917,.T.);
#2094=FACE_OUTER_BOUND('',#2918,.T.);
#2095=FACE_OUTER_BOUND('',#2919,.T.);
#2096=FACE_OUTER_BOUND('',#2920,.T.);
#2097=FACE_OUTER_BOUND('',#2921,.T.);
#2098=FACE_OUTER_BOUND('',#2922,.T.);
#2099=FACE_OUTER_BOUND('',#2923,.T.);
#2100=FACE_OUTER_BOUND('',#2924,.T.);
#2101=FACE_OUTER_BOUND('',#2925,.T.);
#2102=FACE_OUTER_BOUND('',#2926,.T.);
#2103=FACE_OUTER_BOUND('',#2927,.T.);
#2104=FACE_OUTER_BOUND('',#2928,.T.);
#2105=FACE_OUTER_BOUND('',#2929,.T.);
#2106=FACE_OUTER_BOUND('',#2930,.T.);
#2107=FACE_OUTER_BOUND('',#2931,.T.);
#2108=FACE_OUTER_BOUND('',#2932,.T.);
#2109=FACE_OUTER_BOUND('',#2933,.T.);
#2110=FACE_OUTER_BOUND('',#2934,.T.);
#2111=FACE_OUTER_BOUND('',#2935,.T.);
#2112=FACE_OUTER_BOUND('',#2936,.T.);
#2113=FACE_OUTER_BOUND('',#2937,.T.);
#2114=FACE_OUTER_BOUND('',#2938,.T.);
#2115=FACE_OUTER_BOUND('',#2939,.T.);
#2116=FACE_OUTER_BOUND('',#2940,.T.);
#2117=FACE_OUTER_BOUND('',#2941,.T.);
#2118=FACE_OUTER_BOUND('',#2942,.T.);
#2119=FACE_OUTER_BOUND('',#2943,.T.);
#2120=FACE_OUTER_BOUND('',#2944,.T.);
#2121=FACE_OUTER_BOUND('',#2945,.T.);
#2122=FACE_OUTER_BOUND('',#2946,.T.);
#2123=FACE_OUTER_BOUND('',#2947,.T.);
#2124=FACE_OUTER_BOUND('',#2948,.T.);
#2125=FACE_OUTER_BOUND('',#2949,.T.);
#2126=FACE_OUTER_BOUND('',#2950,.T.);
#2127=FACE_OUTER_BOUND('',#2951,.T.);
#2128=FACE_OUTER_BOUND('',#2953,.T.);
#2783=EDGE_LOOP('',(#9332,#9333,#9334,#9335));
#2784=EDGE_LOOP('',(#9336,#9337,#9338,#9339));
#2785=EDGE_LOOP('',(#9340,#9341,#9342,#9343));
#2786=EDGE_LOOP('',(#9344,#9345,#9346,#9347,#9348,#9349,#9350,#9351,#9352,
#9353,#9354,#9355,#9356,#9357,#9358,#9359,#9360,#9361,#9362,#9363,#9364,
#9365,#9366,#9367,#9368,#9369,#9370,#9371,#9372,#9373,#9374,#9375,#9376,
#9377,#9378,#9379,#9380,#9381,#9382,#9383,#9384,#9385,#9386,#9387,#9388,
#9389,#9390,#9391,#9392,#9393,#9394,#9395,#9396,#9397,#9398,#9399,#9400,
#9401,#9402,#9403,#9404,#9405,#9406,#9407,#9408,#9409,#9410,#9411,#9412,
#9413,#9414,#9415,#9416,#9417,#9418,#9419,#9420,#9421,#9422,#9423,#9424,
#9425,#9426,#9427,#9428,#9429,#9430,#9431,#9432,#9433,#9434,#9435,#9436,
#9437,#9438,#9439,#9440,#9441,#9442,#9443,#9444,#9445,#9446,#9447,#9448,
#9449,#9450,#9451,#9452,#9453,#9454,#9455,#9456,#9457,#9458,#9459,#9460,
#9461,#9462,#9463,#9464,#9465,#9466,#9467,#9468,#9469,#9470,#9471,#9472,
#9473,#9474,#9475,#9476,#9477,#9478,#9479,#9480,#9481,#9482,#9483,#9484,
#9485,#9486,#9487,#9488,#9489,#9490,#9491,#9492,#9493,#9494,#9495,#9496,
#9497,#9498,#9499,#9500,#9501,#9502,#9503));
#2787=EDGE_LOOP('',(#9504,#9505,#9506,#9507));
#2788=EDGE_LOOP('',(#9508,#9509,#9510,#9511));
#2789=EDGE_LOOP('',(#9512,#9513,#9514,#9515));
#2790=EDGE_LOOP('',(#9516));
#2791=EDGE_LOOP('',(#9517,#9518,#9519,#9520));
#2792=EDGE_LOOP('',(#9521,#9522,#9523,#9524));
#2793=EDGE_LOOP('',(#9525,#9526,#9527,#9528));
#2794=EDGE_LOOP('',(#9529,#9530,#9531,#9532));
#2795=EDGE_LOOP('',(#9533,#9534,#9535,#9536));
#2796=EDGE_LOOP('',(#9537,#9538,#9539,#9540));
#2797=EDGE_LOOP('',(#9541,#9542,#9543,#9544));
#2798=EDGE_LOOP('',(#9545,#9546,#9547,#9548));
#2799=EDGE_LOOP('',(#9549,#9550,#9551,#9552));
#2800=EDGE_LOOP('',(#9553,#9554,#9555,#9556));
#2801=EDGE_LOOP('',(#9557,#9558,#9559,#9560));
#2802=EDGE_LOOP('',(#9561,#9562,#9563,#9564));
#2803=EDGE_LOOP('',(#9565,#9566,#9567,#9568));
#2804=EDGE_LOOP('',(#9569,#9570,#9571,#9572));
#2805=EDGE_LOOP('',(#9573,#9574,#9575,#9576));
#2806=EDGE_LOOP('',(#9577,#9578,#9579,#9580));
#2807=EDGE_LOOP('',(#9581,#9582,#9583,#9584));
#2808=EDGE_LOOP('',(#9585,#9586,#9587,#9588));
#2809=EDGE_LOOP('',(#9589,#9590,#9591,#9592));
#2810=EDGE_LOOP('',(#9593,#9594,#9595,#9596));
#2811=EDGE_LOOP('',(#9597,#9598,#9599,#9600));
#2812=EDGE_LOOP('',(#9601,#9602,#9603,#9604));
#2813=EDGE_LOOP('',(#9605,#9606,#9607,#9608));
#2814=EDGE_LOOP('',(#9609,#9610,#9611,#9612));
#2815=EDGE_LOOP('',(#9613,#9614,#9615,#9616));
#2816=EDGE_LOOP('',(#9617,#9618,#9619,#9620));
#2817=EDGE_LOOP('',(#9621,#9622,#9623,#9624));
#2818=EDGE_LOOP('',(#9625,#9626,#9627,#9628));
#2819=EDGE_LOOP('',(#9629,#9630,#9631,#9632));
#2820=EDGE_LOOP('',(#9633,#9634,#9635,#9636));
#2821=EDGE_LOOP('',(#9637,#9638,#9639,#9640));
#2822=EDGE_LOOP('',(#9641,#9642,#9643,#9644));
#2823=EDGE_LOOP('',(#9645,#9646,#9647,#9648));
#2824=EDGE_LOOP('',(#9649,#9650,#9651,#9652));
#2825=EDGE_LOOP('',(#9653,#9654,#9655,#9656));
#2826=EDGE_LOOP('',(#9657,#9658,#9659,#9660));
#2827=EDGE_LOOP('',(#9661,#9662,#9663,#9664));
#2828=EDGE_LOOP('',(#9665,#9666,#9667,#9668));
#2829=EDGE_LOOP('',(#9669,#9670,#9671,#9672));
#2830=EDGE_LOOP('',(#9673,#9674,#9675,#9676));
#2831=EDGE_LOOP('',(#9677,#9678,#9679,#9680));
#2832=EDGE_LOOP('',(#9681,#9682,#9683,#9684));
#2833=EDGE_LOOP('',(#9685,#9686,#9687,#9688));
#2834=EDGE_LOOP('',(#9689,#9690,#9691,#9692));
#2835=EDGE_LOOP('',(#9693,#9694,#9695,#9696));
#2836=EDGE_LOOP('',(#9697,#9698,#9699,#9700));
#2837=EDGE_LOOP('',(#9701,#9702,#9703,#9704));
#2838=EDGE_LOOP('',(#9705,#9706,#9707,#9708));
#2839=EDGE_LOOP('',(#9709,#9710,#9711,#9712));
#2840=EDGE_LOOP('',(#9713,#9714,#9715,#9716));
#2841=EDGE_LOOP('',(#9717,#9718,#9719,#9720));
#2842=EDGE_LOOP('',(#9721,#9722,#9723,#9724));
#2843=EDGE_LOOP('',(#9725,#9726,#9727,#9728));
#2844=EDGE_LOOP('',(#9729,#9730,#9731,#9732));
#2845=EDGE_LOOP('',(#9733,#9734,#9735,#9736));
#2846=EDGE_LOOP('',(#9737,#9738,#9739,#9740));
#2847=EDGE_LOOP('',(#9741,#9742,#9743,#9744));
#2848=EDGE_LOOP('',(#9745,#9746,#9747,#9748));
#2849=EDGE_LOOP('',(#9749,#9750,#9751,#9752));
#2850=EDGE_LOOP('',(#9753,#9754,#9755,#9756));
#2851=EDGE_LOOP('',(#9757,#9758,#9759,#9760));
#2852=EDGE_LOOP('',(#9761,#9762,#9763,#9764));
#2853=EDGE_LOOP('',(#9765,#9766,#9767,#9768));
#2854=EDGE_LOOP('',(#9769,#9770,#9771,#9772));
#2855=EDGE_LOOP('',(#9773,#9774,#9775,#9776));
#2856=EDGE_LOOP('',(#9777,#9778,#9779,#9780));
#2857=EDGE_LOOP('',(#9781,#9782,#9783,#9784));
#2858=EDGE_LOOP('',(#9785,#9786,#9787,#9788));
#2859=EDGE_LOOP('',(#9789,#9790,#9791,#9792));
#2860=EDGE_LOOP('',(#9793,#9794,#9795,#9796));
#2861=EDGE_LOOP('',(#9797,#9798,#9799,#9800));
#2862=EDGE_LOOP('',(#9801,#9802,#9803,#9804));
#2863=EDGE_LOOP('',(#9805,#9806,#9807,#9808));
#2864=EDGE_LOOP('',(#9809,#9810,#9811,#9812));
#2865=EDGE_LOOP('',(#9813,#9814,#9815,#9816));
#2866=EDGE_LOOP('',(#9817,#9818,#9819,#9820));
#2867=EDGE_LOOP('',(#9821,#9822,#9823,#9824));
#2868=EDGE_LOOP('',(#9825,#9826,#9827,#9828));
#2869=EDGE_LOOP('',(#9829,#9830,#9831,#9832));
#2870=EDGE_LOOP('',(#9833,#9834,#9835,#9836));
#2871=EDGE_LOOP('',(#9837,#9838,#9839,#9840));
#2872=EDGE_LOOP('',(#9841,#9842,#9843,#9844));
#2873=EDGE_LOOP('',(#9845,#9846,#9847,#9848));
#2874=EDGE_LOOP('',(#9849,#9850,#9851,#9852));
#2875=EDGE_LOOP('',(#9853,#9854,#9855,#9856));
#2876=EDGE_LOOP('',(#9857,#9858,#9859,#9860));
#2877=EDGE_LOOP('',(#9861,#9862,#9863,#9864));
#2878=EDGE_LOOP('',(#9865,#9866,#9867,#9868));
#2879=EDGE_LOOP('',(#9869,#9870,#9871,#9872));
#2880=EDGE_LOOP('',(#9873,#9874,#9875,#9876));
#2881=EDGE_LOOP('',(#9877,#9878,#9879,#9880));
#2882=EDGE_LOOP('',(#9881,#9882,#9883,#9884));
#2883=EDGE_LOOP('',(#9885,#9886,#9887,#9888));
#2884=EDGE_LOOP('',(#9889,#9890,#9891,#9892));
#2885=EDGE_LOOP('',(#9893,#9894,#9895,#9896));
#2886=EDGE_LOOP('',(#9897,#9898,#9899,#9900));
#2887=EDGE_LOOP('',(#9901,#9902,#9903,#9904));
#2888=EDGE_LOOP('',(#9905,#9906,#9907,#9908));
#2889=EDGE_LOOP('',(#9909,#9910,#9911,#9912));
#2890=EDGE_LOOP('',(#9913,#9914,#9915,#9916));
#2891=EDGE_LOOP('',(#9917,#9918,#9919,#9920));
#2892=EDGE_LOOP('',(#9921,#9922,#9923,#9924));
#2893=EDGE_LOOP('',(#9925,#9926,#9927,#9928));
#2894=EDGE_LOOP('',(#9929,#9930,#9931,#9932));
#2895=EDGE_LOOP('',(#9933,#9934,#9935,#9936));
#2896=EDGE_LOOP('',(#9937,#9938,#9939,#9940));
#2897=EDGE_LOOP('',(#9941,#9942,#9943,#9944));
#2898=EDGE_LOOP('',(#9945,#9946,#9947,#9948));
#2899=EDGE_LOOP('',(#9949,#9950,#9951,#9952));
#2900=EDGE_LOOP('',(#9953,#9954,#9955,#9956));
#2901=EDGE_LOOP('',(#9957,#9958,#9959,#9960));
#2902=EDGE_LOOP('',(#9961,#9962,#9963,#9964));
#2903=EDGE_LOOP('',(#9965,#9966,#9967,#9968));
#2904=EDGE_LOOP('',(#9969,#9970,#9971,#9972));
#2905=EDGE_LOOP('',(#9973,#9974,#9975,#9976));
#2906=EDGE_LOOP('',(#9977,#9978,#9979,#9980));
#2907=EDGE_LOOP('',(#9981,#9982,#9983,#9984));
#2908=EDGE_LOOP('',(#9985,#9986,#9987,#9988));
#2909=EDGE_LOOP('',(#9989,#9990,#9991,#9992));
#2910=EDGE_LOOP('',(#9993,#9994,#9995,#9996));
#2911=EDGE_LOOP('',(#9997,#9998,#9999,#10000));
#2912=EDGE_LOOP('',(#10001,#10002,#10003,#10004));
#2913=EDGE_LOOP('',(#10005,#10006,#10007,#10008));
#2914=EDGE_LOOP('',(#10009,#10010,#10011,#10012));
#2915=EDGE_LOOP('',(#10013,#10014,#10015,#10016));
#2916=EDGE_LOOP('',(#10017,#10018,#10019,#10020));
#2917=EDGE_LOOP('',(#10021,#10022,#10023,#10024));
#2918=EDGE_LOOP('',(#10025,#10026,#10027,#10028));
#2919=EDGE_LOOP('',(#10029,#10030,#10031,#10032));
#2920=EDGE_LOOP('',(#10033,#10034,#10035,#10036));
#2921=EDGE_LOOP('',(#10037,#10038,#10039,#10040));
#2922=EDGE_LOOP('',(#10041,#10042,#10043,#10044));
#2923=EDGE_LOOP('',(#10045,#10046,#10047,#10048));
#2924=EDGE_LOOP('',(#10049,#10050,#10051,#10052));
#2925=EDGE_LOOP('',(#10053,#10054,#10055,#10056));
#2926=EDGE_LOOP('',(#10057,#10058,#10059,#10060));
#2927=EDGE_LOOP('',(#10061,#10062,#10063,#10064));
#2928=EDGE_LOOP('',(#10065,#10066,#10067,#10068));
#2929=EDGE_LOOP('',(#10069,#10070,#10071,#10072));
#2930=EDGE_LOOP('',(#10073,#10074,#10075,#10076));
#2931=EDGE_LOOP('',(#10077,#10078,#10079,#10080));
#2932=EDGE_LOOP('',(#10081,#10082,#10083,#10084));
#2933=EDGE_LOOP('',(#10085,#10086,#10087,#10088));
#2934=EDGE_LOOP('',(#10089,#10090,#10091,#10092));
#2935=EDGE_LOOP('',(#10093,#10094,#10095,#10096));
#2936=EDGE_LOOP('',(#10097,#10098,#10099,#10100));
#2937=EDGE_LOOP('',(#10101,#10102,#10103,#10104));
#2938=EDGE_LOOP('',(#10105,#10106,#10107,#10108));
#2939=EDGE_LOOP('',(#10109,#10110,#10111,#10112));
#2940=EDGE_LOOP('',(#10113,#10114,#10115,#10116));
#2941=EDGE_LOOP('',(#10117,#10118,#10119,#10120));
#2942=EDGE_LOOP('',(#10121,#10122,#10123,#10124));
#2943=EDGE_LOOP('',(#10125,#10126,#10127,#10128));
#2944=EDGE_LOOP('',(#10129,#10130,#10131,#10132));
#2945=EDGE_LOOP('',(#10133,#10134,#10135,#10136));
#2946=EDGE_LOOP('',(#10137,#10138,#10139,#10140));
#2947=EDGE_LOOP('',(#10141,#10142,#10143,#10144));
#2948=EDGE_LOOP('',(#10145,#10146,#10147,#10148));
#2949=EDGE_LOOP('',(#10149,#10150,#10151,#10152));
#2950=EDGE_LOOP('',(#10153,#10154,#10155,#10156));
#2951=EDGE_LOOP('',(#10157,#10158,#10159,#10160,#10161,#10162,#10163,#10164,
#10165,#10166,#10167,#10168,#10169,#10170,#10171,#10172,#10173,#10174,#10175,
#10176,#10177,#10178,#10179,#10180,#10181,#10182,#10183,#10184,#10185,#10186,
#10187,#10188,#10189,#10190,#10191,#10192,#10193,#10194,#10195,#10196,#10197,
#10198,#10199,#10200,#10201,#10202,#10203,#10204,#10205,#10206,#10207,#10208,
#10209,#10210,#10211,#10212,#10213,#10214,#10215,#10216,#10217,#10218,#10219,
#10220,#10221,#10222,#10223,#10224,#10225,#10226,#10227,#10228,#10229,#10230,
#10231,#10232,#10233,#10234,#10235,#10236,#10237,#10238,#10239,#10240,#10241,
#10242,#10243,#10244,#10245,#10246,#10247,#10248,#10249,#10250,#10251,#10252,
#10253,#10254,#10255,#10256,#10257,#10258,#10259,#10260,#10261,#10262,#10263,
#10264,#10265,#10266,#10267,#10268,#10269,#10270,#10271,#10272,#10273,#10274,
#10275,#10276,#10277,#10278,#10279,#10280,#10281,#10282,#10283,#10284,#10285,
#10286,#10287,#10288,#10289,#10290,#10291,#10292,#10293,#10294,#10295,#10296,
#10297,#10298,#10299,#10300,#10301,#10302,#10303,#10304,#10305,#10306,#10307,
#10308,#10309,#10310,#10311,#10312,#10313,#10314,#10315,#10316));
#2952=EDGE_LOOP('',(#10317));
#2953=EDGE_LOOP('',(#10318,#10319,#10320,#10321));
#3402=LINE('',#30130,#4043);
#3403=LINE('',#30132,#4044);
#3404=LINE('',#30134,#4045);
#3405=LINE('',#30135,#4046);
#3406=LINE('',#30138,#4047);
#3407=LINE('',#30140,#4048);
#3408=LINE('',#30141,#4049);
#3409=LINE('',#30144,#4050);
#3410=LINE('',#30146,#4051);
#3411=LINE('',#30147,#4052);
#3412=LINE('',#30224,#4053);
#3413=LINE('',#30370,#4054);
#3414=LINE('',#30516,#4055);
#3415=LINE('',#30662,#4056);
#3416=LINE('',#30808,#4057);
#3417=LINE('',#30954,#4058);
#3418=LINE('',#31100,#4059);
#3419=LINE('',#31246,#4060);
#3420=LINE('',#31392,#4061);
#3421=LINE('',#31538,#4062);
#3422=LINE('',#31684,#4063);
#3423=LINE('',#31830,#4064);
#3424=LINE('',#31976,#4065);
#3425=LINE('',#32122,#4066);
#3426=LINE('',#32268,#4067);
#3427=LINE('',#32414,#4068);
#3428=LINE('',#32560,#4069);
#3429=LINE('',#32706,#4070);
#3430=LINE('',#32852,#4071);
#3431=LINE('',#32998,#4072);
#3432=LINE('',#33144,#4073);
#3433=LINE('',#33290,#4074);
#3434=LINE('',#33436,#4075);
#3435=LINE('',#33582,#4076);
#3436=LINE('',#33728,#4077);
#3437=LINE('',#33874,#4078);
#3438=LINE('',#34020,#4079);
#3439=LINE('',#34166,#4080);
#3440=LINE('',#34312,#4081);
#3441=LINE('',#34458,#4082);
#3442=LINE('',#34604,#4083);
#3443=LINE('',#34750,#4084);
#3444=LINE('',#34896,#4085);
#3445=LINE('',#35042,#4086);
#3446=LINE('',#35188,#4087);
#3447=LINE('',#35334,#4088);
#3448=LINE('',#35480,#4089);
#3449=LINE('',#35626,#4090);
#3450=LINE('',#35772,#4091);
#3451=LINE('',#35918,#4092);
#3452=LINE('',#35996,#4093);
#3453=LINE('',#36217,#4094);
#3454=LINE('',#36366,#4095);
#3455=LINE('',#36438,#4096);
#3456=LINE('',#36659,#4097);
#3457=LINE('',#36808,#4098);
#3458=LINE('',#36880,#4099);
#3459=LINE('',#37101,#4100);
#3460=LINE('',#37250,#4101);
#3461=LINE('',#37322,#4102);
#3462=LINE('',#37543,#4103);
#3463=LINE('',#37692,#4104);
#3464=LINE('',#37764,#4105);
#3465=LINE('',#37985,#4106);
#3466=LINE('',#38134,#4107);
#3467=LINE('',#38206,#4108);
#3468=LINE('',#38427,#4109);
#3469=LINE('',#38576,#4110);
#3470=LINE('',#38648,#4111);
#3471=LINE('',#38869,#4112);
#3472=LINE('',#39018,#4113);
#3473=LINE('',#39090,#4114);
#3474=LINE('',#39311,#4115);
#3475=LINE('',#39460,#4116);
#3476=LINE('',#39532,#4117);
#3477=LINE('',#39753,#4118);
#3478=LINE('',#39902,#4119);
#3479=LINE('',#39974,#4120);
#3480=LINE('',#40195,#4121);
#3481=LINE('',#40344,#4122);
#3482=LINE('',#40416,#4123);
#3483=LINE('',#40637,#4124);
#3484=LINE('',#40786,#4125);
#3485=LINE('',#40858,#4126);
#3486=LINE('',#41079,#4127);
#3487=LINE('',#41228,#4128);
#3488=LINE('',#41300,#4129);
#3489=LINE('',#41521,#4130);
#3490=LINE('',#41670,#4131);
#3491=LINE('',#41742,#4132);
#3492=LINE('',#41963,#4133);
#3493=LINE('',#42112,#4134);
#3494=LINE('',#42184,#4135);
#3495=LINE('',#42405,#4136);
#3496=LINE('',#42554,#4137);
#3497=LINE('',#42626,#4138);
#3498=LINE('',#42847,#4139);
#3499=LINE('',#42996,#4140);
#3500=LINE('',#43068,#4141);
#3501=LINE('',#43289,#4142);
#3502=LINE('',#43438,#4143);
#3503=LINE('',#43510,#4144);
#3504=LINE('',#43731,#4145);
#3505=LINE('',#43880,#4146);
#3506=LINE('',#43952,#4147);
#3507=LINE('',#44173,#4148);
#3508=LINE('',#44322,#4149);
#3509=LINE('',#44394,#4150);
#3510=LINE('',#44615,#4151);
#3511=LINE('',#44764,#4152);
#3512=LINE('',#44836,#4153);
#3513=LINE('',#45057,#4154);
#3514=LINE('',#45206,#4155);
#3515=LINE('',#45278,#4156);
#3516=LINE('',#45499,#4157);
#3517=LINE('',#45648,#4158);
#3518=LINE('',#45720,#4159);
#3519=LINE('',#45941,#4160);
#3520=LINE('',#46090,#4161);
#3521=LINE('',#46162,#4162);
#3522=LINE('',#46383,#4163);
#3523=LINE('',#46532,#4164);
#3524=LINE('',#46604,#4165);
#3525=LINE('',#46825,#4166);
#3526=LINE('',#46974,#4167);
#3527=LINE('',#47046,#4168);
#3528=LINE('',#47267,#4169);
#3529=LINE('',#47416,#4170);
#3530=LINE('',#47488,#4171);
#3531=LINE('',#47709,#4172);
#3532=LINE('',#47858,#4173);
#3533=LINE('',#47930,#4174);
#3534=LINE('',#48151,#4175);
#3535=LINE('',#48300,#4176);
#3536=LINE('',#48372,#4177);
#3537=LINE('',#48593,#4178);
#3538=LINE('',#48742,#4179);
#3539=LINE('',#48814,#4180);
#3540=LINE('',#49035,#4181);
#3541=LINE('',#49184,#4182);
#3542=LINE('',#49256,#4183);
#3543=LINE('',#49477,#4184);
#3544=LINE('',#49626,#4185);
#3545=LINE('',#49698,#4186);
#3546=LINE('',#49919,#4187);
#3547=LINE('',#50068,#4188);
#3548=LINE('',#50140,#4189);
#3549=LINE('',#50361,#4190);
#3550=LINE('',#50510,#4191);
#3551=LINE('',#50582,#4192);
#3552=LINE('',#50803,#4193);
#3553=LINE('',#50952,#4194);
#3554=LINE('',#51024,#4195);
#3555=LINE('',#51245,#4196);
#3556=LINE('',#51394,#4197);
#3557=LINE('',#51466,#4198);
#3558=LINE('',#51687,#4199);
#3559=LINE('',#51836,#4200);
#3560=LINE('',#51908,#4201);
#3561=LINE('',#52129,#4202);
#3562=LINE('',#52278,#4203);
#3563=LINE('',#52350,#4204);
#3564=LINE('',#52571,#4205);
#3565=LINE('',#52720,#4206);
#3566=LINE('',#52792,#4207);
#3567=LINE('',#53013,#4208);
#3568=LINE('',#53016,#4209);
#3569=LINE('',#53017,#4210);
#3570=LINE('',#53392,#4211);
#3571=LINE('',#53674,#4212);
#3572=LINE('',#53676,#4213);
#4043=VECTOR('',#15311,1.);
#4044=VECTOR('',#15312,1.);
#4045=VECTOR('',#15313,1.);
#4046=VECTOR('',#15314,1.);
#4047=VECTOR('',#15317,1.);
#4048=VECTOR('',#15318,1.);
#4049=VECTOR('',#15319,1.);
#4050=VECTOR('',#15322,1.);
#4051=VECTOR('',#15323,1.);
#4052=VECTOR('',#15324,1.);
#4053=VECTOR('',#15329,1.);
#4054=VECTOR('',#15332,1.);
#4055=VECTOR('',#15335,1.);
#4056=VECTOR('',#15338,1.);
#4057=VECTOR('',#15341,1.);
#4058=VECTOR('',#15344,1.);
#4059=VECTOR('',#15347,1.);
#4060=VECTOR('',#15350,1.);
#4061=VECTOR('',#15353,1.);
#4062=VECTOR('',#15356,1.);
#4063=VECTOR('',#15359,1.);
#4064=VECTOR('',#15362,1.);
#4065=VECTOR('',#15365,1.);
#4066=VECTOR('',#15368,1.);
#4067=VECTOR('',#15371,1.);
#4068=VECTOR('',#15374,1.);
#4069=VECTOR('',#15377,1.);
#4070=VECTOR('',#15380,1.);
#4071=VECTOR('',#15383,1.);
#4072=VECTOR('',#15386,1.);
#4073=VECTOR('',#15389,1.);
#4074=VECTOR('',#15392,1.);
#4075=VECTOR('',#15395,1.);
#4076=VECTOR('',#15398,1.);
#4077=VECTOR('',#15401,1.);
#4078=VECTOR('',#15404,1.);
#4079=VECTOR('',#15407,1.);
#4080=VECTOR('',#15410,1.);
#4081=VECTOR('',#15413,1.);
#4082=VECTOR('',#15416,1.);
#4083=VECTOR('',#15419,1.);
#4084=VECTOR('',#15422,1.);
#4085=VECTOR('',#15425,1.);
#4086=VECTOR('',#15428,1.);
#4087=VECTOR('',#15431,1.);
#4088=VECTOR('',#15434,1.);
#4089=VECTOR('',#15437,1.);
#4090=VECTOR('',#15440,1.);
#4091=VECTOR('',#15443,1.);
#4092=VECTOR('',#15446,1.);
#4093=VECTOR('',#15457,2.);
#4094=VECTOR('',#15462,1.);
#4095=VECTOR('',#15463,1.);
#4096=VECTOR('',#15466,1.);
#4097=VECTOR('',#15471,1.);
#4098=VECTOR('',#15472,1.);
#4099=VECTOR('',#15475,1.);
#4100=VECTOR('',#15480,1.);
#4101=VECTOR('',#15481,1.);
#4102=VECTOR('',#15484,1.);
#4103=VECTOR('',#15489,1.);
#4104=VECTOR('',#15490,1.);
#4105=VECTOR('',#15493,1.);
#4106=VECTOR('',#15498,1.);
#4107=VECTOR('',#15499,1.);
#4108=VECTOR('',#15502,1.);
#4109=VECTOR('',#15507,1.);
#4110=VECTOR('',#15508,1.);
#4111=VECTOR('',#15511,1.);
#4112=VECTOR('',#15516,1.);
#4113=VECTOR('',#15517,1.);
#4114=VECTOR('',#15520,1.);
#4115=VECTOR('',#15525,1.);
#4116=VECTOR('',#15526,1.);
#4117=VECTOR('',#15529,1.);
#4118=VECTOR('',#15534,1.);
#4119=VECTOR('',#15535,1.);
#4120=VECTOR('',#15538,1.);
#4121=VECTOR('',#15543,1.);
#4122=VECTOR('',#15544,1.);
#4123=VECTOR('',#15547,1.);
#4124=VECTOR('',#15552,1.);
#4125=VECTOR('',#15553,1.);
#4126=VECTOR('',#15556,1.);
#4127=VECTOR('',#15561,1.);
#4128=VECTOR('',#15562,1.);
#4129=VECTOR('',#15565,1.);
#4130=VECTOR('',#15570,1.);
#4131=VECTOR('',#15571,1.);
#4132=VECTOR('',#15574,1.);
#4133=VECTOR('',#15579,1.);
#4134=VECTOR('',#15580,1.);
#4135=VECTOR('',#15583,1.);
#4136=VECTOR('',#15588,1.);
#4137=VECTOR('',#15589,1.);
#4138=VECTOR('',#15592,1.);
#4139=VECTOR('',#15597,1.);
#4140=VECTOR('',#15598,1.);
#4141=VECTOR('',#15601,1.);
#4142=VECTOR('',#15606,1.);
#4143=VECTOR('',#15607,1.);
#4144=VECTOR('',#15610,1.);
#4145=VECTOR('',#15615,1.);
#4146=VECTOR('',#15616,1.);
#4147=VECTOR('',#15619,1.);
#4148=VECTOR('',#15624,1.);
#4149=VECTOR('',#15625,1.);
#4150=VECTOR('',#15628,1.);
#4151=VECTOR('',#15633,1.);
#4152=VECTOR('',#15634,1.);
#4153=VECTOR('',#15637,1.);
#4154=VECTOR('',#15642,1.);
#4155=VECTOR('',#15643,1.);
#4156=VECTOR('',#15646,1.);
#4157=VECTOR('',#15651,1.);
#4158=VECTOR('',#15652,1.);
#4159=VECTOR('',#15655,1.);
#4160=VECTOR('',#15660,1.);
#4161=VECTOR('',#15661,1.);
#4162=VECTOR('',#15664,1.);
#4163=VECTOR('',#15669,1.);
#4164=VECTOR('',#15670,1.);
#4165=VECTOR('',#15673,1.);
#4166=VECTOR('',#15678,1.);
#4167=VECTOR('',#15679,1.);
#4168=VECTOR('',#15682,1.);
#4169=VECTOR('',#15687,1.);
#4170=VECTOR('',#15688,1.);
#4171=VECTOR('',#15691,1.);
#4172=VECTOR('',#15696,1.);
#4173=VECTOR('',#15697,1.);
#4174=VECTOR('',#15700,1.);
#4175=VECTOR('',#15705,1.);
#4176=VECTOR('',#15706,1.);
#4177=VECTOR('',#15709,1.);
#4178=VECTOR('',#15714,1.);
#4179=VECTOR('',#15715,1.);
#4180=VECTOR('',#15718,1.);
#4181=VECTOR('',#15723,1.);
#4182=VECTOR('',#15724,1.);
#4183=VECTOR('',#15727,1.);
#4184=VECTOR('',#15732,1.);
#4185=VECTOR('',#15733,1.);
#4186=VECTOR('',#15736,1.);
#4187=VECTOR('',#15741,1.);
#4188=VECTOR('',#15742,1.);
#4189=VECTOR('',#15745,1.);
#4190=VECTOR('',#15750,1.);
#4191=VECTOR('',#15751,1.);
#4192=VECTOR('',#15754,1.);
#4193=VECTOR('',#15759,1.);
#4194=VECTOR('',#15760,1.);
#4195=VECTOR('',#15763,1.);
#4196=VECTOR('',#15768,1.);
#4197=VECTOR('',#15769,1.);
#4198=VECTOR('',#15772,1.);
#4199=VECTOR('',#15777,1.);
#4200=VECTOR('',#15778,1.);
#4201=VECTOR('',#15781,1.);
#4202=VECTOR('',#15786,1.);
#4203=VECTOR('',#15787,1.);
#4204=VECTOR('',#15790,1.);
#4205=VECTOR('',#15795,1.);
#4206=VECTOR('',#15796,1.);
#4207=VECTOR('',#15799,1.);
#4208=VECTOR('',#15804,1.);
#4209=VECTOR('',#15807,1.);
#4210=VECTOR('',#15808,1.);
#4211=VECTOR('',#15813,1.);
#4212=VECTOR('',#15814,1.);
#4213=VECTOR('',#15817,1.);
#4696=CIRCLE('',#12761,3.75);
#4697=CIRCLE('',#12762,3.75);
#4698=CIRCLE('',#12763,3.75);
#4699=CIRCLE('',#12764,3.75);
#4700=CIRCLE('',#12765,3.75);
#4701=CIRCLE('',#12766,3.75);
#4702=CIRCLE('',#12767,3.75);
#4703=CIRCLE('',#12768,3.75);
#4704=CIRCLE('',#12769,3.75);
#4705=CIRCLE('',#12770,3.75);
#4706=CIRCLE('',#12771,3.75);
#4707=CIRCLE('',#12772,3.75);
#4708=CIRCLE('',#12773,3.75);
#4709=CIRCLE('',#12774,3.75);
#4710=CIRCLE('',#12775,3.75);
#4711=CIRCLE('',#12776,3.75);
#4712=CIRCLE('',#12777,3.75);
#4713=CIRCLE('',#12778,3.75);
#4714=CIRCLE('',#12779,3.75);
#4715=CIRCLE('',#12780,3.75);
#4716=CIRCLE('',#12781,3.75);
#4717=CIRCLE('',#12782,3.75);
#4718=CIRCLE('',#12783,3.75);
#4719=CIRCLE('',#12784,3.75);
#4720=CIRCLE('',#12785,3.75);
#4721=CIRCLE('',#12786,3.75);
#4722=CIRCLE('',#12787,3.75);
#4723=CIRCLE('',#12788,3.75);
#4724=CIRCLE('',#12789,3.75);
#4725=CIRCLE('',#12790,3.75);
#4726=CIRCLE('',#12791,3.75);
#4727=CIRCLE('',#12792,3.75);
#4728=CIRCLE('',#12793,3.75);
#4729=CIRCLE('',#12794,3.75);
#4730=CIRCLE('',#12795,3.75);
#4731=CIRCLE('',#12796,3.75);
#4732=CIRCLE('',#12797,3.75);
#4733=CIRCLE('',#12798,3.75);
#4734=CIRCLE('',#12799,3.75);
#4735=CIRCLE('',#12800,3.75);
#4736=CIRCLE('',#12801,1.);
#4737=CIRCLE('',#12803,1.);
#4738=CIRCLE('',#12805,2.);
#4739=CIRCLE('',#12806,2.);
#4740=CIRCLE('',#12810,3.75);
#4741=CIRCLE('',#12813,3.75);
#4742=CIRCLE('',#12816,3.75);
#4743=CIRCLE('',#12819,3.75);
#4744=CIRCLE('',#12822,3.75);
#4745=CIRCLE('',#12825,3.75);
#4746=CIRCLE('',#12828,3.75);
#4747=CIRCLE('',#12831,3.75);
#4748=CIRCLE('',#12834,3.75);
#4749=CIRCLE('',#12837,3.75);
#4750=CIRCLE('',#12840,3.75);
#4751=CIRCLE('',#12843,3.75);
#4752=CIRCLE('',#12846,3.75);
#4753=CIRCLE('',#12849,3.75);
#4754=CIRCLE('',#12852,3.75);
#4755=CIRCLE('',#12855,3.75);
#4756=CIRCLE('',#12858,3.75);
#4757=CIRCLE('',#12861,3.75);
#4758=CIRCLE('',#12864,3.75);
#4759=CIRCLE('',#12867,3.75);
#4760=CIRCLE('',#12870,3.75);
#4761=CIRCLE('',#12873,3.75);
#4762=CIRCLE('',#12876,3.75);
#4763=CIRCLE('',#12879,3.75);
#4764=CIRCLE('',#12882,3.75);
#4765=CIRCLE('',#12885,3.75);
#4766=CIRCLE('',#12888,3.75);
#4767=CIRCLE('',#12891,3.75);
#4768=CIRCLE('',#12894,3.75);
#4769=CIRCLE('',#12897,3.75);
#4770=CIRCLE('',#12900,3.75);
#4771=CIRCLE('',#12903,3.75);
#4772=CIRCLE('',#12906,3.75);
#4773=CIRCLE('',#12909,3.75);
#4774=CIRCLE('',#12912,3.75);
#4775=CIRCLE('',#12915,3.75);
#4776=CIRCLE('',#12918,3.75);
#4777=CIRCLE('',#12921,3.75);
#4778=CIRCLE('',#12924,3.75);
#4779=CIRCLE('',#12927,3.75);
#5456=VERTEX_POINT('',#30128);
#5457=VERTEX_POINT('',#30129);
#5458=VERTEX_POINT('',#30131);
#5459=VERTEX_POINT('',#30133);
#5460=VERTEX_POINT('',#30137);
#5461=VERTEX_POINT('',#30139);
#5462=VERTEX_POINT('',#30143);
#5463=VERTEX_POINT('',#30145);
#5464=VERTEX_POINT('',#30149);
#5465=VERTEX_POINT('',#30150);
#5466=VERTEX_POINT('',#30152);
#5467=VERTEX_POINT('',#30223);
#5468=VERTEX_POINT('',#30225);
#5469=VERTEX_POINT('',#30296);
#5470=VERTEX_POINT('',#30298);
#5471=VERTEX_POINT('',#30369);
#5472=VERTEX_POINT('',#30371);
#5473=VERTEX_POINT('',#30442);
#5474=VERTEX_POINT('',#30444);
#5475=VERTEX_POINT('',#30515);
#5476=VERTEX_POINT('',#30517);
#5477=VERTEX_POINT('',#30588);
#5478=VERTEX_POINT('',#30590);
#5479=VERTEX_POINT('',#30661);
#5480=VERTEX_POINT('',#30663);
#5481=VERTEX_POINT('',#30734);
#5482=VERTEX_POINT('',#30736);
#5483=VERTEX_POINT('',#30807);
#5484=VERTEX_POINT('',#30809);
#5485=VERTEX_POINT('',#30880);
#5486=VERTEX_POINT('',#30882);
#5487=VERTEX_POINT('',#30953);
#5488=VERTEX_POINT('',#30955);
#5489=VERTEX_POINT('',#31026);
#5490=VERTEX_POINT('',#31028);
#5491=VERTEX_POINT('',#31099);
#5492=VERTEX_POINT('',#31101);
#5493=VERTEX_POINT('',#31172);
#5494=VERTEX_POINT('',#31174);
#5495=VERTEX_POINT('',#31245);
#5496=VERTEX_POINT('',#31247);
#5497=VERTEX_POINT('',#31318);
#5498=VERTEX_POINT('',#31320);
#5499=VERTEX_POINT('',#31391);
#5500=VERTEX_POINT('',#31393);
#5501=VERTEX_POINT('',#31464);
#5502=VERTEX_POINT('',#31466);
#5503=VERTEX_POINT('',#31537);
#5504=VERTEX_POINT('',#31539);
#5505=VERTEX_POINT('',#31610);
#5506=VERTEX_POINT('',#31612);
#5507=VERTEX_POINT('',#31683);
#5508=VERTEX_POINT('',#31685);
#5509=VERTEX_POINT('',#31756);
#5510=VERTEX_POINT('',#31758);
#5511=VERTEX_POINT('',#31829);
#5512=VERTEX_POINT('',#31831);
#5513=VERTEX_POINT('',#31902);
#5514=VERTEX_POINT('',#31904);
#5515=VERTEX_POINT('',#31975);
#5516=VERTEX_POINT('',#31977);
#5517=VERTEX_POINT('',#32048);
#5518=VERTEX_POINT('',#32050);
#5519=VERTEX_POINT('',#32121);
#5520=VERTEX_POINT('',#32123);
#5521=VERTEX_POINT('',#32194);
#5522=VERTEX_POINT('',#32196);
#5523=VERTEX_POINT('',#32267);
#5524=VERTEX_POINT('',#32269);
#5525=VERTEX_POINT('',#32340);
#5526=VERTEX_POINT('',#32342);
#5527=VERTEX_POINT('',#32413);
#5528=VERTEX_POINT('',#32415);
#5529=VERTEX_POINT('',#32486);
#5530=VERTEX_POINT('',#32488);
#5531=VERTEX_POINT('',#32559);
#5532=VERTEX_POINT('',#32561);
#5533=VERTEX_POINT('',#32632);
#5534=VERTEX_POINT('',#32634);
#5535=VERTEX_POINT('',#32705);
#5536=VERTEX_POINT('',#32707);
#5537=VERTEX_POINT('',#32778);
#5538=VERTEX_POINT('',#32780);
#5539=VERTEX_POINT('',#32851);
#5540=VERTEX_POINT('',#32853);
#5541=VERTEX_POINT('',#32924);
#5542=VERTEX_POINT('',#32926);
#5543=VERTEX_POINT('',#32997);
#5544=VERTEX_POINT('',#32999);
#5545=VERTEX_POINT('',#33070);
#5546=VERTEX_POINT('',#33072);
#5547=VERTEX_POINT('',#33143);
#5548=VERTEX_POINT('',#33145);
#5549=VERTEX_POINT('',#33216);
#5550=VERTEX_POINT('',#33218);
#5551=VERTEX_POINT('',#33289);
#5552=VERTEX_POINT('',#33291);
#5553=VERTEX_POINT('',#33362);
#5554=VERTEX_POINT('',#33364);
#5555=VERTEX_POINT('',#33435);
#5556=VERTEX_POINT('',#33437);
#5557=VERTEX_POINT('',#33508);
#5558=VERTEX_POINT('',#33510);
#5559=VERTEX_POINT('',#33581);
#5560=VERTEX_POINT('',#33583);
#5561=VERTEX_POINT('',#33654);
#5562=VERTEX_POINT('',#33656);
#5563=VERTEX_POINT('',#33727);
#5564=VERTEX_POINT('',#33729);
#5565=VERTEX_POINT('',#33800);
#5566=VERTEX_POINT('',#33802);
#5567=VERTEX_POINT('',#33873);
#5568=VERTEX_POINT('',#33875);
#5569=VERTEX_POINT('',#33946);
#5570=VERTEX_POINT('',#33948);
#5571=VERTEX_POINT('',#34019);
#5572=VERTEX_POINT('',#34021);
#5573=VERTEX_POINT('',#34092);
#5574=VERTEX_POINT('',#34094);
#5575=VERTEX_POINT('',#34165);
#5576=VERTEX_POINT('',#34167);
#5577=VERTEX_POINT('',#34238);
#5578=VERTEX_POINT('',#34240);
#5579=VERTEX_POINT('',#34311);
#5580=VERTEX_POINT('',#34313);
#5581=VERTEX_POINT('',#34384);
#5582=VERTEX_POINT('',#34386);
#5583=VERTEX_POINT('',#34457);
#5584=VERTEX_POINT('',#34459);
#5585=VERTEX_POINT('',#34530);
#5586=VERTEX_POINT('',#34532);
#5587=VERTEX_POINT('',#34603);
#5588=VERTEX_POINT('',#34605);
#5589=VERTEX_POINT('',#34676);
#5590=VERTEX_POINT('',#34678);
#5591=VERTEX_POINT('',#34749);
#5592=VERTEX_POINT('',#34751);
#5593=VERTEX_POINT('',#34822);
#5594=VERTEX_POINT('',#34824);
#5595=VERTEX_POINT('',#34895);
#5596=VERTEX_POINT('',#34897);
#5597=VERTEX_POINT('',#34968);
#5598=VERTEX_POINT('',#34970);
#5599=VERTEX_POINT('',#35041);
#5600=VERTEX_POINT('',#35043);
#5601=VERTEX_POINT('',#35114);
#5602=VERTEX_POINT('',#35116);
#5603=VERTEX_POINT('',#35187);
#5604=VERTEX_POINT('',#35189);
#5605=VERTEX_POINT('',#35260);
#5606=VERTEX_POINT('',#35262);
#5607=VERTEX_POINT('',#35333);
#5608=VERTEX_POINT('',#35335);
#5609=VERTEX_POINT('',#35406);
#5610=VERTEX_POINT('',#35408);
#5611=VERTEX_POINT('',#35479);
#5612=VERTEX_POINT('',#35481);
#5613=VERTEX_POINT('',#35552);
#5614=VERTEX_POINT('',#35554);
#5615=VERTEX_POINT('',#35625);
#5616=VERTEX_POINT('',#35627);
#5617=VERTEX_POINT('',#35698);
#5618=VERTEX_POINT('',#35700);
#5619=VERTEX_POINT('',#35771);
#5620=VERTEX_POINT('',#35773);
#5621=VERTEX_POINT('',#35844);
#5622=VERTEX_POINT('',#35846);
#5623=VERTEX_POINT('',#35917);
#5624=VERTEX_POINT('',#35993);
#5625=VERTEX_POINT('',#35995);
#5626=VERTEX_POINT('',#36139);
#5627=VERTEX_POINT('',#36146);
#5628=VERTEX_POINT('',#36358);
#5629=VERTEX_POINT('',#36365);
#5630=VERTEX_POINT('',#36440);
#5631=VERTEX_POINT('',#36588);
#5632=VERTEX_POINT('',#36800);
#5633=VERTEX_POINT('',#36807);
#5634=VERTEX_POINT('',#36882);
#5635=VERTEX_POINT('',#37030);
#5636=VERTEX_POINT('',#37242);
#5637=VERTEX_POINT('',#37249);
#5638=VERTEX_POINT('',#37324);
#5639=VERTEX_POINT('',#37472);
#5640=VERTEX_POINT('',#37684);
#5641=VERTEX_POINT('',#37691);
#5642=VERTEX_POINT('',#37766);
#5643=VERTEX_POINT('',#37914);
#5644=VERTEX_POINT('',#38126);
#5645=VERTEX_POINT('',#38133);
#5646=VERTEX_POINT('',#38208);
#5647=VERTEX_POINT('',#38356);
#5648=VERTEX_POINT('',#38568);
#5649=VERTEX_POINT('',#38575);
#5650=VERTEX_POINT('',#38650);
#5651=VERTEX_POINT('',#38798);
#5652=VERTEX_POINT('',#39010);
#5653=VERTEX_POINT('',#39017);
#5654=VERTEX_POINT('',#39092);
#5655=VERTEX_POINT('',#39240);
#5656=VERTEX_POINT('',#39452);
#5657=VERTEX_POINT('',#39459);
#5658=VERTEX_POINT('',#39534);
#5659=VERTEX_POINT('',#39682);
#5660=VERTEX_POINT('',#39894);
#5661=VERTEX_POINT('',#39901);
#5662=VERTEX_POINT('',#39976);
#5663=VERTEX_POINT('',#40124);
#5664=VERTEX_POINT('',#40336);
#5665=VERTEX_POINT('',#40343);
#5666=VERTEX_POINT('',#40418);
#5667=VERTEX_POINT('',#40566);
#5668=VERTEX_POINT('',#40778);
#5669=VERTEX_POINT('',#40785);
#5670=VERTEX_POINT('',#40860);
#5671=VERTEX_POINT('',#41008);
#5672=VERTEX_POINT('',#41220);
#5673=VERTEX_POINT('',#41227);
#5674=VERTEX_POINT('',#41302);
#5675=VERTEX_POINT('',#41450);
#5676=VERTEX_POINT('',#41662);
#5677=VERTEX_POINT('',#41669);
#5678=VERTEX_POINT('',#41744);
#5679=VERTEX_POINT('',#41892);
#5680=VERTEX_POINT('',#42104);
#5681=VERTEX_POINT('',#42111);
#5682=VERTEX_POINT('',#42186);
#5683=VERTEX_POINT('',#42334);
#5684=VERTEX_POINT('',#42546);
#5685=VERTEX_POINT('',#42553);
#5686=VERTEX_POINT('',#42628);
#5687=VERTEX_POINT('',#42776);
#5688=VERTEX_POINT('',#42988);
#5689=VERTEX_POINT('',#42995);
#5690=VERTEX_POINT('',#43070);
#5691=VERTEX_POINT('',#43218);
#5692=VERTEX_POINT('',#43430);
#5693=VERTEX_POINT('',#43437);
#5694=VERTEX_POINT('',#43512);
#5695=VERTEX_POINT('',#43660);
#5696=VERTEX_POINT('',#43872);
#5697=VERTEX_POINT('',#43879);
#5698=VERTEX_POINT('',#43954);
#5699=VERTEX_POINT('',#44102);
#5700=VERTEX_POINT('',#44314);
#5701=VERTEX_POINT('',#44321);
#5702=VERTEX_POINT('',#44396);
#5703=VERTEX_POINT('',#44544);
#5704=VERTEX_POINT('',#44756);
#5705=VERTEX_POINT('',#44763);
#5706=VERTEX_POINT('',#44838);
#5707=VERTEX_POINT('',#44986);
#5708=VERTEX_POINT('',#45198);
#5709=VERTEX_POINT('',#45205);
#5710=VERTEX_POINT('',#45280);
#5711=VERTEX_POINT('',#45428);
#5712=VERTEX_POINT('',#45640);
#5713=VERTEX_POINT('',#45647);
#5714=VERTEX_POINT('',#45722);
#5715=VERTEX_POINT('',#45870);
#5716=VERTEX_POINT('',#46082);
#5717=VERTEX_POINT('',#46089);
#5718=VERTEX_POINT('',#46164);
#5719=VERTEX_POINT('',#46312);
#5720=VERTEX_POINT('',#46524);
#5721=VERTEX_POINT('',#46531);
#5722=VERTEX_POINT('',#46606);
#5723=VERTEX_POINT('',#46754);
#5724=VERTEX_POINT('',#46966);
#5725=VERTEX_POINT('',#46973);
#5726=VERTEX_POINT('',#47048);
#5727=VERTEX_POINT('',#47196);
#5728=VERTEX_POINT('',#47408);
#5729=VERTEX_POINT('',#47415);
#5730=VERTEX_POINT('',#47490);
#5731=VERTEX_POINT('',#47638);
#5732=VERTEX_POINT('',#47850);
#5733=VERTEX_POINT('',#47857);
#5734=VERTEX_POINT('',#47932);
#5735=VERTEX_POINT('',#48080);
#5736=VERTEX_POINT('',#48292);
#5737=VERTEX_POINT('',#48299);
#5738=VERTEX_POINT('',#48374);
#5739=VERTEX_POINT('',#48522);
#5740=VERTEX_POINT('',#48734);
#5741=VERTEX_POINT('',#48741);
#5742=VERTEX_POINT('',#48816);
#5743=VERTEX_POINT('',#48964);
#5744=VERTEX_POINT('',#49176);
#5745=VERTEX_POINT('',#49183);
#5746=VERTEX_POINT('',#49258);
#5747=VERTEX_POINT('',#49406);
#5748=VERTEX_POINT('',#49618);
#5749=VERTEX_POINT('',#49625);
#5750=VERTEX_POINT('',#49700);
#5751=VERTEX_POINT('',#49848);
#5752=VERTEX_POINT('',#50060);
#5753=VERTEX_POINT('',#50067);
#5754=VERTEX_POINT('',#50142);
#5755=VERTEX_POINT('',#50290);
#5756=VERTEX_POINT('',#50502);
#5757=VERTEX_POINT('',#50509);
#5758=VERTEX_POINT('',#50584);
#5759=VERTEX_POINT('',#50732);
#5760=VERTEX_POINT('',#50944);
#5761=VERTEX_POINT('',#50951);
#5762=VERTEX_POINT('',#51026);
#5763=VERTEX_POINT('',#51174);
#5764=VERTEX_POINT('',#51386);
#5765=VERTEX_POINT('',#51393);
#5766=VERTEX_POINT('',#51468);
#5767=VERTEX_POINT('',#51616);
#5768=VERTEX_POINT('',#51828);
#5769=VERTEX_POINT('',#51835);
#5770=VERTEX_POINT('',#51910);
#5771=VERTEX_POINT('',#52058);
#5772=VERTEX_POINT('',#52270);
#5773=VERTEX_POINT('',#52277);
#5774=VERTEX_POINT('',#52352);
#5775=VERTEX_POINT('',#52500);
#5776=VERTEX_POINT('',#52712);
#5777=VERTEX_POINT('',#52719);
#5778=VERTEX_POINT('',#52794);
#5779=VERTEX_POINT('',#52942);
#5780=VERTEX_POINT('',#53015);
#5781=VERTEX_POINT('',#53158);
#5782=VERTEX_POINT('',#53236);
#5783=VERTEX_POINT('',#53384);
#5784=VERTEX_POINT('',#53391);
#5785=VERTEX_POINT('',#53603);
#6808=EDGE_CURVE('',#5456,#5457,#3402,.T.);
#6809=EDGE_CURVE('',#5458,#5456,#3403,.T.);
#6810=EDGE_CURVE('',#5459,#5458,#3404,.T.);
#6811=EDGE_CURVE('',#5457,#5459,#3405,.T.);
#6812=EDGE_CURVE('',#5460,#5456,#3406,.T.);
#6813=EDGE_CURVE('',#5460,#5461,#3407,.T.);
#6814=EDGE_CURVE('',#5458,#5461,#3408,.T.);
#6815=EDGE_CURVE('',#5462,#5460,#3409,.T.);
#6816=EDGE_CURVE('',#5463,#5462,#3410,.T.);
#6817=EDGE_CURVE('',#5461,#5463,#3411,.T.);
#6818=EDGE_CURVE('',#5464,#5465,#4696,.T.);
#6819=EDGE_CURVE('',#5465,#5466,#211,.T.);
#6820=EDGE_CURVE('',#5466,#5467,#3412,.T.);
#6821=EDGE_CURVE('',#5467,#5468,#212,.T.);
#6822=EDGE_CURVE('',#5468,#5469,#4697,.T.);
#6823=EDGE_CURVE('',#5469,#5470,#213,.T.);
#6824=EDGE_CURVE('',#5470,#5471,#3413,.T.);
#6825=EDGE_CURVE('',#5471,#5472,#214,.T.);
#6826=EDGE_CURVE('',#5472,#5473,#4698,.T.);
#6827=EDGE_CURVE('',#5473,#5474,#215,.T.);
#6828=EDGE_CURVE('',#5474,#5475,#3414,.T.);
#6829=EDGE_CURVE('',#5475,#5476,#216,.T.);
#6830=EDGE_CURVE('',#5476,#5477,#4699,.T.);
#6831=EDGE_CURVE('',#5477,#5478,#217,.T.);
#6832=EDGE_CURVE('',#5478,#5479,#3415,.T.);
#6833=EDGE_CURVE('',#5479,#5480,#218,.T.);
#6834=EDGE_CURVE('',#5480,#5481,#4700,.T.);
#6835=EDGE_CURVE('',#5481,#5482,#219,.T.);
#6836=EDGE_CURVE('',#5482,#5483,#3416,.T.);
#6837=EDGE_CURVE('',#5483,#5484,#220,.T.);
#6838=EDGE_CURVE('',#5484,#5485,#4701,.T.);
#6839=EDGE_CURVE('',#5485,#5486,#221,.T.);
#6840=EDGE_CURVE('',#5486,#5487,#3417,.T.);
#6841=EDGE_CURVE('',#5487,#5488,#222,.T.);
#6842=EDGE_CURVE('',#5488,#5489,#4702,.T.);
#6843=EDGE_CURVE('',#5489,#5490,#223,.T.);
#6844=EDGE_CURVE('',#5490,#5491,#3418,.T.);
#6845=EDGE_CURVE('',#5491,#5492,#224,.T.);
#6846=EDGE_CURVE('',#5492,#5493,#4703,.T.);
#6847=EDGE_CURVE('',#5493,#5494,#225,.T.);
#6848=EDGE_CURVE('',#5494,#5495,#3419,.T.);
#6849=EDGE_CURVE('',#5495,#5496,#226,.T.);
#6850=EDGE_CURVE('',#5496,#5497,#4704,.T.);
#6851=EDGE_CURVE('',#5497,#5498,#227,.T.);
#6852=EDGE_CURVE('',#5498,#5499,#3420,.T.);
#6853=EDGE_CURVE('',#5499,#5500,#228,.T.);
#6854=EDGE_CURVE('',#5500,#5501,#4705,.T.);
#6855=EDGE_CURVE('',#5501,#5502,#229,.T.);
#6856=EDGE_CURVE('',#5502,#5503,#3421,.T.);
#6857=EDGE_CURVE('',#5503,#5504,#230,.T.);
#6858=EDGE_CURVE('',#5504,#5505,#4706,.T.);
#6859=EDGE_CURVE('',#5505,#5506,#231,.T.);
#6860=EDGE_CURVE('',#5506,#5507,#3422,.T.);
#6861=EDGE_CURVE('',#5507,#5508,#232,.T.);
#6862=EDGE_CURVE('',#5508,#5509,#4707,.T.);
#6863=EDGE_CURVE('',#5509,#5510,#233,.T.);
#6864=EDGE_CURVE('',#5510,#5511,#3423,.T.);
#6865=EDGE_CURVE('',#5511,#5512,#234,.T.);
#6866=EDGE_CURVE('',#5512,#5513,#4708,.T.);
#6867=EDGE_CURVE('',#5513,#5514,#235,.T.);
#6868=EDGE_CURVE('',#5514,#5515,#3424,.T.);
#6869=EDGE_CURVE('',#5515,#5516,#236,.T.);
#6870=EDGE_CURVE('',#5516,#5517,#4709,.T.);
#6871=EDGE_CURVE('',#5517,#5518,#237,.T.);
#6872=EDGE_CURVE('',#5518,#5519,#3425,.T.);
#6873=EDGE_CURVE('',#5519,#5520,#238,.T.);
#6874=EDGE_CURVE('',#5520,#5521,#4710,.T.);
#6875=EDGE_CURVE('',#5521,#5522,#239,.T.);
#6876=EDGE_CURVE('',#5522,#5523,#3426,.T.);
#6877=EDGE_CURVE('',#5523,#5524,#240,.T.);
#6878=EDGE_CURVE('',#5524,#5525,#4711,.T.);
#6879=EDGE_CURVE('',#5525,#5526,#241,.T.);
#6880=EDGE_CURVE('',#5526,#5527,#3427,.T.);
#6881=EDGE_CURVE('',#5527,#5528,#242,.T.);
#6882=EDGE_CURVE('',#5528,#5529,#4712,.T.);
#6883=EDGE_CURVE('',#5529,#5530,#243,.T.);
#6884=EDGE_CURVE('',#5530,#5531,#3428,.T.);
#6885=EDGE_CURVE('',#5531,#5532,#244,.T.);
#6886=EDGE_CURVE('',#5532,#5533,#4713,.T.);
#6887=EDGE_CURVE('',#5533,#5534,#245,.T.);
#6888=EDGE_CURVE('',#5534,#5535,#3429,.T.);
#6889=EDGE_CURVE('',#5535,#5536,#246,.T.);
#6890=EDGE_CURVE('',#5536,#5537,#4714,.T.);
#6891=EDGE_CURVE('',#5537,#5538,#247,.T.);
#6892=EDGE_CURVE('',#5538,#5539,#3430,.T.);
#6893=EDGE_CURVE('',#5539,#5540,#248,.T.);
#6894=EDGE_CURVE('',#5540,#5541,#4715,.T.);
#6895=EDGE_CURVE('',#5541,#5542,#249,.T.);
#6896=EDGE_CURVE('',#5542,#5543,#3431,.T.);
#6897=EDGE_CURVE('',#5543,#5544,#250,.T.);
#6898=EDGE_CURVE('',#5544,#5545,#4716,.T.);
#6899=EDGE_CURVE('',#5545,#5546,#251,.T.);
#6900=EDGE_CURVE('',#5546,#5547,#3432,.T.);
#6901=EDGE_CURVE('',#5547,#5548,#252,.T.);
#6902=EDGE_CURVE('',#5548,#5549,#4717,.T.);
#6903=EDGE_CURVE('',#5549,#5550,#253,.T.);
#6904=EDGE_CURVE('',#5550,#5551,#3433,.T.);
#6905=EDGE_CURVE('',#5551,#5552,#254,.T.);
#6906=EDGE_CURVE('',#5552,#5553,#4718,.T.);
#6907=EDGE_CURVE('',#5553,#5554,#255,.T.);
#6908=EDGE_CURVE('',#5554,#5555,#3434,.T.);
#6909=EDGE_CURVE('',#5555,#5556,#256,.T.);
#6910=EDGE_CURVE('',#5556,#5557,#4719,.T.);
#6911=EDGE_CURVE('',#5557,#5558,#257,.T.);
#6912=EDGE_CURVE('',#5558,#5559,#3435,.T.);
#6913=EDGE_CURVE('',#5559,#5560,#258,.T.);
#6914=EDGE_CURVE('',#5560,#5561,#4720,.T.);
#6915=EDGE_CURVE('',#5561,#5562,#259,.T.);
#6916=EDGE_CURVE('',#5562,#5563,#3436,.T.);
#6917=EDGE_CURVE('',#5563,#5564,#260,.T.);
#6918=EDGE_CURVE('',#5564,#5565,#4721,.T.);
#6919=EDGE_CURVE('',#5565,#5566,#261,.T.);
#6920=EDGE_CURVE('',#5566,#5567,#3437,.T.);
#6921=EDGE_CURVE('',#5567,#5568,#262,.T.);
#6922=EDGE_CURVE('',#5568,#5569,#4722,.T.);
#6923=EDGE_CURVE('',#5569,#5570,#263,.T.);
#6924=EDGE_CURVE('',#5570,#5571,#3438,.T.);
#6925=EDGE_CURVE('',#5571,#5572,#264,.T.);
#6926=EDGE_CURVE('',#5572,#5573,#4723,.T.);
#6927=EDGE_CURVE('',#5573,#5574,#265,.T.);
#6928=EDGE_CURVE('',#5574,#5575,#3439,.T.);
#6929=EDGE_CURVE('',#5575,#5576,#266,.T.);
#6930=EDGE_CURVE('',#5576,#5577,#4724,.T.);
#6931=EDGE_CURVE('',#5577,#5578,#267,.T.);
#6932=EDGE_CURVE('',#5578,#5579,#3440,.T.);
#6933=EDGE_CURVE('',#5579,#5580,#268,.T.);
#6934=EDGE_CURVE('',#5580,#5581,#4725,.T.);
#6935=EDGE_CURVE('',#5581,#5582,#269,.T.);
#6936=EDGE_CURVE('',#5582,#5583,#3441,.T.);
#6937=EDGE_CURVE('',#5583,#5584,#270,.T.);
#6938=EDGE_CURVE('',#5584,#5585,#4726,.T.);
#6939=EDGE_CURVE('',#5585,#5586,#271,.T.);
#6940=EDGE_CURVE('',#5586,#5587,#3442,.T.);
#6941=EDGE_CURVE('',#5587,#5588,#272,.T.);
#6942=EDGE_CURVE('',#5588,#5589,#4727,.T.);
#6943=EDGE_CURVE('',#5589,#5590,#273,.T.);
#6944=EDGE_CURVE('',#5590,#5591,#3443,.T.);
#6945=EDGE_CURVE('',#5591,#5592,#274,.T.);
#6946=EDGE_CURVE('',#5592,#5593,#4728,.T.);
#6947=EDGE_CURVE('',#5593,#5594,#275,.T.);
#6948=EDGE_CURVE('',#5594,#5595,#3444,.T.);
#6949=EDGE_CURVE('',#5595,#5596,#276,.T.);
#6950=EDGE_CURVE('',#5596,#5597,#4729,.T.);
#6951=EDGE_CURVE('',#5597,#5598,#277,.T.);
#6952=EDGE_CURVE('',#5598,#5599,#3445,.T.);
#6953=EDGE_CURVE('',#5599,#5600,#278,.T.);
#6954=EDGE_CURVE('',#5600,#5601,#4730,.T.);
#6955=EDGE_CURVE('',#5601,#5602,#279,.T.);
#6956=EDGE_CURVE('',#5602,#5603,#3446,.T.);
#6957=EDGE_CURVE('',#5603,#5604,#280,.T.);
#6958=EDGE_CURVE('',#5604,#5605,#4731,.T.);
#6959=EDGE_CURVE('',#5605,#5606,#281,.T.);
#6960=EDGE_CURVE('',#5606,#5607,#3447,.T.);
#6961=EDGE_CURVE('',#5607,#5608,#282,.T.);
#6962=EDGE_CURVE('',#5608,#5609,#4732,.T.);
#6963=EDGE_CURVE('',#5609,#5610,#283,.T.);
#6964=EDGE_CURVE('',#5610,#5611,#3448,.T.);
#6965=EDGE_CURVE('',#5611,#5612,#284,.T.);
#6966=EDGE_CURVE('',#5612,#5613,#4733,.T.);
#6967=EDGE_CURVE('',#5613,#5614,#285,.T.);
#6968=EDGE_CURVE('',#5614,#5615,#3449,.T.);
#6969=EDGE_CURVE('',#5615,#5616,#286,.T.);
#6970=EDGE_CURVE('',#5616,#5617,#4734,.T.);
#6971=EDGE_CURVE('',#5617,#5618,#287,.T.);
#6972=EDGE_CURVE('',#5618,#5619,#3450,.T.);
#6973=EDGE_CURVE('',#5619,#5620,#288,.T.);
#6974=EDGE_CURVE('',#5620,#5621,#4735,.T.);
#6975=EDGE_CURVE('',#5621,#5622,#289,.T.);
#6976=EDGE_CURVE('',#5622,#5623,#3451,.T.);
#6977=EDGE_CURVE('',#5623,#5464,#290,.T.);
#6978=EDGE_CURVE('',#5463,#5459,#4736,.T.);
#6979=EDGE_CURVE('',#5457,#5462,#4737,.T.);
#6980=EDGE_CURVE('',#5624,#5624,#4738,.T.);
#6981=EDGE_CURVE('',#5624,#5625,#3452,.T.);
#6982=EDGE_CURVE('',#5625,#5625,#4739,.T.);
#6983=EDGE_CURVE('',#5626,#5621,#715,.T.);
#6984=EDGE_CURVE('',#5627,#5626,#291,.T.);
#6985=EDGE_CURVE('',#5622,#5627,#3453,.T.);
#6986=EDGE_CURVE('',#5464,#5628,#716,.T.);
#6987=EDGE_CURVE('',#5623,#5629,#3454,.T.);
#6988=EDGE_CURVE('',#5628,#5629,#292,.T.);
#6989=EDGE_CURVE('',#5629,#5627,#3455,.T.);
#6990=EDGE_CURVE('',#5630,#5628,#4740,.T.);
#6991=EDGE_CURVE('',#5630,#5465,#717,.T.);
#6992=EDGE_CURVE('',#5631,#5630,#293,.T.);
#6993=EDGE_CURVE('',#5466,#5631,#3456,.T.);
#6994=EDGE_CURVE('',#5468,#5632,#718,.T.);
#6995=EDGE_CURVE('',#5467,#5633,#3457,.T.);
#6996=EDGE_CURVE('',#5632,#5633,#294,.T.);
#6997=EDGE_CURVE('',#5633,#5631,#3458,.T.);
#6998=EDGE_CURVE('',#5634,#5632,#4741,.T.);
#6999=EDGE_CURVE('',#5634,#5469,#719,.T.);
#7000=EDGE_CURVE('',#5635,#5634,#295,.T.);
#7001=EDGE_CURVE('',#5470,#5635,#3459,.T.);
#7002=EDGE_CURVE('',#5472,#5636,#720,.T.);
#7003=EDGE_CURVE('',#5471,#5637,#3460,.T.);
#7004=EDGE_CURVE('',#5636,#5637,#296,.T.);
#7005=EDGE_CURVE('',#5637,#5635,#3461,.T.);
#7006=EDGE_CURVE('',#5638,#5636,#4742,.T.);
#7007=EDGE_CURVE('',#5638,#5473,#721,.T.);
#7008=EDGE_CURVE('',#5639,#5638,#297,.T.);
#7009=EDGE_CURVE('',#5474,#5639,#3462,.T.);
#7010=EDGE_CURVE('',#5476,#5640,#722,.T.);
#7011=EDGE_CURVE('',#5475,#5641,#3463,.T.);
#7012=EDGE_CURVE('',#5640,#5641,#298,.T.);
#7013=EDGE_CURVE('',#5641,#5639,#3464,.T.);
#7014=EDGE_CURVE('',#5642,#5640,#4743,.T.);
#7015=EDGE_CURVE('',#5642,#5477,#723,.T.);
#7016=EDGE_CURVE('',#5643,#5642,#299,.T.);
#7017=EDGE_CURVE('',#5478,#5643,#3465,.T.);
#7018=EDGE_CURVE('',#5480,#5644,#724,.T.);
#7019=EDGE_CURVE('',#5479,#5645,#3466,.T.);
#7020=EDGE_CURVE('',#5644,#5645,#300,.T.);
#7021=EDGE_CURVE('',#5645,#5643,#3467,.T.);
#7022=EDGE_CURVE('',#5646,#5644,#4744,.T.);
#7023=EDGE_CURVE('',#5646,#5481,#725,.T.);
#7024=EDGE_CURVE('',#5647,#5646,#301,.T.);
#7025=EDGE_CURVE('',#5482,#5647,#3468,.T.);
#7026=EDGE_CURVE('',#5484,#5648,#726,.T.);
#7027=EDGE_CURVE('',#5483,#5649,#3469,.T.);
#7028=EDGE_CURVE('',#5648,#5649,#302,.T.);
#7029=EDGE_CURVE('',#5649,#5647,#3470,.T.);
#7030=EDGE_CURVE('',#5650,#5648,#4745,.T.);
#7031=EDGE_CURVE('',#5650,#5485,#727,.T.);
#7032=EDGE_CURVE('',#5651,#5650,#303,.T.);
#7033=EDGE_CURVE('',#5486,#5651,#3471,.T.);
#7034=EDGE_CURVE('',#5488,#5652,#728,.T.);
#7035=EDGE_CURVE('',#5487,#5653,#3472,.T.);
#7036=EDGE_CURVE('',#5652,#5653,#304,.T.);
#7037=EDGE_CURVE('',#5653,#5651,#3473,.T.);
#7038=EDGE_CURVE('',#5654,#5652,#4746,.T.);
#7039=EDGE_CURVE('',#5654,#5489,#729,.T.);
#7040=EDGE_CURVE('',#5655,#5654,#305,.T.);
#7041=EDGE_CURVE('',#5490,#5655,#3474,.T.);
#7042=EDGE_CURVE('',#5492,#5656,#730,.T.);
#7043=EDGE_CURVE('',#5491,#5657,#3475,.T.);
#7044=EDGE_CURVE('',#5656,#5657,#306,.T.);
#7045=EDGE_CURVE('',#5657,#5655,#3476,.T.);
#7046=EDGE_CURVE('',#5658,#5656,#4747,.T.);
#7047=EDGE_CURVE('',#5658,#5493,#731,.T.);
#7048=EDGE_CURVE('',#5659,#5658,#307,.T.);
#7049=EDGE_CURVE('',#5494,#5659,#3477,.T.);
#7050=EDGE_CURVE('',#5496,#5660,#732,.T.);
#7051=EDGE_CURVE('',#5495,#5661,#3478,.T.);
#7052=EDGE_CURVE('',#5660,#5661,#308,.T.);
#7053=EDGE_CURVE('',#5661,#5659,#3479,.T.);
#7054=EDGE_CURVE('',#5662,#5660,#4748,.T.);
#7055=EDGE_CURVE('',#5662,#5497,#733,.T.);
#7056=EDGE_CURVE('',#5663,#5662,#309,.T.);
#7057=EDGE_CURVE('',#5498,#5663,#3480,.T.);
#7058=EDGE_CURVE('',#5500,#5664,#734,.T.);
#7059=EDGE_CURVE('',#5499,#5665,#3481,.T.);
#7060=EDGE_CURVE('',#5664,#5665,#310,.T.);
#7061=EDGE_CURVE('',#5665,#5663,#3482,.T.);
#7062=EDGE_CURVE('',#5666,#5664,#4749,.T.);
#7063=EDGE_CURVE('',#5666,#5501,#735,.T.);
#7064=EDGE_CURVE('',#5667,#5666,#311,.T.);
#7065=EDGE_CURVE('',#5502,#5667,#3483,.T.);
#7066=EDGE_CURVE('',#5504,#5668,#736,.T.);
#7067=EDGE_CURVE('',#5503,#5669,#3484,.T.);
#7068=EDGE_CURVE('',#5668,#5669,#312,.T.);
#7069=EDGE_CURVE('',#5669,#5667,#3485,.T.);
#7070=EDGE_CURVE('',#5670,#5668,#4750,.T.);
#7071=EDGE_CURVE('',#5670,#5505,#737,.T.);
#7072=EDGE_CURVE('',#5671,#5670,#313,.T.);
#7073=EDGE_CURVE('',#5506,#5671,#3486,.T.);
#7074=EDGE_CURVE('',#5508,#5672,#738,.T.);
#7075=EDGE_CURVE('',#5507,#5673,#3487,.T.);
#7076=EDGE_CURVE('',#5672,#5673,#314,.T.);
#7077=EDGE_CURVE('',#5673,#5671,#3488,.T.);
#7078=EDGE_CURVE('',#5674,#5672,#4751,.T.);
#7079=EDGE_CURVE('',#5674,#5509,#739,.T.);
#7080=EDGE_CURVE('',#5675,#5674,#315,.T.);
#7081=EDGE_CURVE('',#5510,#5675,#3489,.T.);
#7082=EDGE_CURVE('',#5512,#5676,#740,.T.);
#7083=EDGE_CURVE('',#5511,#5677,#3490,.T.);
#7084=EDGE_CURVE('',#5676,#5677,#316,.T.);
#7085=EDGE_CURVE('',#5677,#5675,#3491,.T.);
#7086=EDGE_CURVE('',#5678,#5676,#4752,.T.);
#7087=EDGE_CURVE('',#5678,#5513,#741,.T.);
#7088=EDGE_CURVE('',#5679,#5678,#317,.T.);
#7089=EDGE_CURVE('',#5514,#5679,#3492,.T.);
#7090=EDGE_CURVE('',#5516,#5680,#742,.T.);
#7091=EDGE_CURVE('',#5515,#5681,#3493,.T.);
#7092=EDGE_CURVE('',#5680,#5681,#318,.T.);
#7093=EDGE_CURVE('',#5681,#5679,#3494,.T.);
#7094=EDGE_CURVE('',#5682,#5680,#4753,.T.);
#7095=EDGE_CURVE('',#5682,#5517,#743,.T.);
#7096=EDGE_CURVE('',#5683,#5682,#319,.T.);
#7097=EDGE_CURVE('',#5518,#5683,#3495,.T.);
#7098=EDGE_CURVE('',#5520,#5684,#744,.T.);
#7099=EDGE_CURVE('',#5519,#5685,#3496,.T.);
#7100=EDGE_CURVE('',#5684,#5685,#320,.T.);
#7101=EDGE_CURVE('',#5685,#5683,#3497,.T.);
#7102=EDGE_CURVE('',#5686,#5684,#4754,.T.);
#7103=EDGE_CURVE('',#5686,#5521,#745,.T.);
#7104=EDGE_CURVE('',#5687,#5686,#321,.T.);
#7105=EDGE_CURVE('',#5522,#5687,#3498,.T.);
#7106=EDGE_CURVE('',#5524,#5688,#746,.T.);
#7107=EDGE_CURVE('',#5523,#5689,#3499,.T.);
#7108=EDGE_CURVE('',#5688,#5689,#322,.T.);
#7109=EDGE_CURVE('',#5689,#5687,#3500,.T.);
#7110=EDGE_CURVE('',#5690,#5688,#4755,.T.);
#7111=EDGE_CURVE('',#5690,#5525,#747,.T.);
#7112=EDGE_CURVE('',#5691,#5690,#323,.T.);
#7113=EDGE_CURVE('',#5526,#5691,#3501,.T.);
#7114=EDGE_CURVE('',#5528,#5692,#748,.T.);
#7115=EDGE_CURVE('',#5527,#5693,#3502,.T.);
#7116=EDGE_CURVE('',#5692,#5693,#324,.T.);
#7117=EDGE_CURVE('',#5693,#5691,#3503,.T.);
#7118=EDGE_CURVE('',#5694,#5692,#4756,.T.);
#7119=EDGE_CURVE('',#5694,#5529,#749,.T.);
#7120=EDGE_CURVE('',#5695,#5694,#325,.T.);
#7121=EDGE_CURVE('',#5530,#5695,#3504,.T.);
#7122=EDGE_CURVE('',#5532,#5696,#750,.T.);
#7123=EDGE_CURVE('',#5531,#5697,#3505,.T.);
#7124=EDGE_CURVE('',#5696,#5697,#326,.T.);
#7125=EDGE_CURVE('',#5697,#5695,#3506,.T.);
#7126=EDGE_CURVE('',#5698,#5696,#4757,.T.);
#7127=EDGE_CURVE('',#5698,#5533,#751,.T.);
#7128=EDGE_CURVE('',#5699,#5698,#327,.T.);
#7129=EDGE_CURVE('',#5534,#5699,#3507,.T.);
#7130=EDGE_CURVE('',#5536,#5700,#752,.T.);
#7131=EDGE_CURVE('',#5535,#5701,#3508,.T.);
#7132=EDGE_CURVE('',#5700,#5701,#328,.T.);
#7133=EDGE_CURVE('',#5701,#5699,#3509,.T.);
#7134=EDGE_CURVE('',#5702,#5700,#4758,.T.);
#7135=EDGE_CURVE('',#5702,#5537,#753,.T.);
#7136=EDGE_CURVE('',#5703,#5702,#329,.T.);
#7137=EDGE_CURVE('',#5538,#5703,#3510,.T.);
#7138=EDGE_CURVE('',#5540,#5704,#754,.T.);
#7139=EDGE_CURVE('',#5539,#5705,#3511,.T.);
#7140=EDGE_CURVE('',#5704,#5705,#330,.T.);
#7141=EDGE_CURVE('',#5705,#5703,#3512,.T.);
#7142=EDGE_CURVE('',#5706,#5704,#4759,.T.);
#7143=EDGE_CURVE('',#5706,#5541,#755,.T.);
#7144=EDGE_CURVE('',#5707,#5706,#331,.T.);
#7145=EDGE_CURVE('',#5542,#5707,#3513,.T.);
#7146=EDGE_CURVE('',#5544,#5708,#756,.T.);
#7147=EDGE_CURVE('',#5543,#5709,#3514,.T.);
#7148=EDGE_CURVE('',#5708,#5709,#332,.T.);
#7149=EDGE_CURVE('',#5709,#5707,#3515,.T.);
#7150=EDGE_CURVE('',#5710,#5708,#4760,.T.);
#7151=EDGE_CURVE('',#5710,#5545,#757,.T.);
#7152=EDGE_CURVE('',#5711,#5710,#333,.T.);
#7153=EDGE_CURVE('',#5546,#5711,#3516,.T.);
#7154=EDGE_CURVE('',#5548,#5712,#758,.T.);
#7155=EDGE_CURVE('',#5547,#5713,#3517,.T.);
#7156=EDGE_CURVE('',#5712,#5713,#334,.T.);
#7157=EDGE_CURVE('',#5713,#5711,#3518,.T.);
#7158=EDGE_CURVE('',#5714,#5712,#4761,.T.);
#7159=EDGE_CURVE('',#5714,#5549,#759,.T.);
#7160=EDGE_CURVE('',#5715,#5714,#335,.T.);
#7161=EDGE_CURVE('',#5550,#5715,#3519,.T.);
#7162=EDGE_CURVE('',#5552,#5716,#760,.T.);
#7163=EDGE_CURVE('',#5551,#5717,#3520,.T.);
#7164=EDGE_CURVE('',#5716,#5717,#336,.T.);
#7165=EDGE_CURVE('',#5717,#5715,#3521,.T.);
#7166=EDGE_CURVE('',#5718,#5716,#4762,.T.);
#7167=EDGE_CURVE('',#5718,#5553,#761,.T.);
#7168=EDGE_CURVE('',#5719,#5718,#337,.T.);
#7169=EDGE_CURVE('',#5554,#5719,#3522,.T.);
#7170=EDGE_CURVE('',#5556,#5720,#762,.T.);
#7171=EDGE_CURVE('',#5555,#5721,#3523,.T.);
#7172=EDGE_CURVE('',#5720,#5721,#338,.T.);
#7173=EDGE_CURVE('',#5721,#5719,#3524,.T.);
#7174=EDGE_CURVE('',#5722,#5720,#4763,.T.);
#7175=EDGE_CURVE('',#5722,#5557,#763,.T.);
#7176=EDGE_CURVE('',#5723,#5722,#339,.T.);
#7177=EDGE_CURVE('',#5558,#5723,#3525,.T.);
#7178=EDGE_CURVE('',#5560,#5724,#764,.T.);
#7179=EDGE_CURVE('',#5559,#5725,#3526,.T.);
#7180=EDGE_CURVE('',#5724,#5725,#340,.T.);
#7181=EDGE_CURVE('',#5725,#5723,#3527,.T.);
#7182=EDGE_CURVE('',#5726,#5724,#4764,.T.);
#7183=EDGE_CURVE('',#5726,#5561,#765,.T.);
#7184=EDGE_CURVE('',#5727,#5726,#341,.T.);
#7185=EDGE_CURVE('',#5562,#5727,#3528,.T.);
#7186=EDGE_CURVE('',#5564,#5728,#766,.T.);
#7187=EDGE_CURVE('',#5563,#5729,#3529,.T.);
#7188=EDGE_CURVE('',#5728,#5729,#342,.T.);
#7189=EDGE_CURVE('',#5729,#5727,#3530,.T.);
#7190=EDGE_CURVE('',#5730,#5728,#4765,.T.);
#7191=EDGE_CURVE('',#5730,#5565,#767,.T.);
#7192=EDGE_CURVE('',#5731,#5730,#343,.T.);
#7193=EDGE_CURVE('',#5566,#5731,#3531,.T.);
#7194=EDGE_CURVE('',#5568,#5732,#768,.T.);
#7195=EDGE_CURVE('',#5567,#5733,#3532,.T.);
#7196=EDGE_CURVE('',#5732,#5733,#344,.T.);
#7197=EDGE_CURVE('',#5733,#5731,#3533,.T.);
#7198=EDGE_CURVE('',#5734,#5732,#4766,.T.);
#7199=EDGE_CURVE('',#5734,#5569,#769,.T.);
#7200=EDGE_CURVE('',#5735,#5734,#345,.T.);
#7201=EDGE_CURVE('',#5570,#5735,#3534,.T.);
#7202=EDGE_CURVE('',#5572,#5736,#770,.T.);
#7203=EDGE_CURVE('',#5571,#5737,#3535,.T.);
#7204=EDGE_CURVE('',#5736,#5737,#346,.T.);
#7205=EDGE_CURVE('',#5737,#5735,#3536,.T.);
#7206=EDGE_CURVE('',#5738,#5736,#4767,.T.);
#7207=EDGE_CURVE('',#5738,#5573,#771,.T.);
#7208=EDGE_CURVE('',#5739,#5738,#347,.T.);
#7209=EDGE_CURVE('',#5574,#5739,#3537,.T.);
#7210=EDGE_CURVE('',#5576,#5740,#772,.T.);
#7211=EDGE_CURVE('',#5575,#5741,#3538,.T.);
#7212=EDGE_CURVE('',#5740,#5741,#348,.T.);
#7213=EDGE_CURVE('',#5741,#5739,#3539,.T.);
#7214=EDGE_CURVE('',#5742,#5740,#4768,.T.);
#7215=EDGE_CURVE('',#5742,#5577,#773,.T.);
#7216=EDGE_CURVE('',#5743,#5742,#349,.T.);
#7217=EDGE_CURVE('',#5578,#5743,#3540,.T.);
#7218=EDGE_CURVE('',#5580,#5744,#774,.T.);
#7219=EDGE_CURVE('',#5579,#5745,#3541,.T.);
#7220=EDGE_CURVE('',#5744,#5745,#350,.T.);
#7221=EDGE_CURVE('',#5745,#5743,#3542,.T.);
#7222=EDGE_CURVE('',#5746,#5744,#4769,.T.);
#7223=EDGE_CURVE('',#5746,#5581,#775,.T.);
#7224=EDGE_CURVE('',#5747,#5746,#351,.T.);
#7225=EDGE_CURVE('',#5582,#5747,#3543,.T.);
#7226=EDGE_CURVE('',#5584,#5748,#776,.T.);
#7227=EDGE_CURVE('',#5583,#5749,#3544,.T.);
#7228=EDGE_CURVE('',#5748,#5749,#352,.T.);
#7229=EDGE_CURVE('',#5749,#5747,#3545,.T.);
#7230=EDGE_CURVE('',#5750,#5748,#4770,.T.);
#7231=EDGE_CURVE('',#5750,#5585,#777,.T.);
#7232=EDGE_CURVE('',#5751,#5750,#353,.T.);
#7233=EDGE_CURVE('',#5586,#5751,#3546,.T.);
#7234=EDGE_CURVE('',#5588,#5752,#778,.T.);
#7235=EDGE_CURVE('',#5587,#5753,#3547,.T.);
#7236=EDGE_CURVE('',#5752,#5753,#354,.T.);
#7237=EDGE_CURVE('',#5753,#5751,#3548,.T.);
#7238=EDGE_CURVE('',#5754,#5752,#4771,.T.);
#7239=EDGE_CURVE('',#5754,#5589,#779,.T.);
#7240=EDGE_CURVE('',#5755,#5754,#355,.T.);
#7241=EDGE_CURVE('',#5590,#5755,#3549,.T.);
#7242=EDGE_CURVE('',#5592,#5756,#780,.T.);
#7243=EDGE_CURVE('',#5591,#5757,#3550,.T.);
#7244=EDGE_CURVE('',#5756,#5757,#356,.T.);
#7245=EDGE_CURVE('',#5757,#5755,#3551,.T.);
#7246=EDGE_CURVE('',#5758,#5756,#4772,.T.);
#7247=EDGE_CURVE('',#5758,#5593,#781,.T.);
#7248=EDGE_CURVE('',#5759,#5758,#357,.T.);
#7249=EDGE_CURVE('',#5594,#5759,#3552,.T.);
#7250=EDGE_CURVE('',#5596,#5760,#782,.T.);
#7251=EDGE_CURVE('',#5595,#5761,#3553,.T.);
#7252=EDGE_CURVE('',#5760,#5761,#358,.T.);
#7253=EDGE_CURVE('',#5761,#5759,#3554,.T.);
#7254=EDGE_CURVE('',#5762,#5760,#4773,.T.);
#7255=EDGE_CURVE('',#5762,#5597,#783,.T.);
#7256=EDGE_CURVE('',#5763,#5762,#359,.T.);
#7257=EDGE_CURVE('',#5598,#5763,#3555,.T.);
#7258=EDGE_CURVE('',#5600,#5764,#784,.T.);
#7259=EDGE_CURVE('',#5599,#5765,#3556,.T.);
#7260=EDGE_CURVE('',#5764,#5765,#360,.T.);
#7261=EDGE_CURVE('',#5765,#5763,#3557,.T.);
#7262=EDGE_CURVE('',#5766,#5764,#4774,.T.);
#7263=EDGE_CURVE('',#5766,#5601,#785,.T.);
#7264=EDGE_CURVE('',#5767,#5766,#361,.T.);
#7265=EDGE_CURVE('',#5602,#5767,#3558,.T.);
#7266=EDGE_CURVE('',#5604,#5768,#786,.T.);
#7267=EDGE_CURVE('',#5603,#5769,#3559,.T.);
#7268=EDGE_CURVE('',#5768,#5769,#362,.T.);
#7269=EDGE_CURVE('',#5769,#5767,#3560,.T.);
#7270=EDGE_CURVE('',#5770,#5768,#4775,.T.);
#7271=EDGE_CURVE('',#5770,#5605,#787,.T.);
#7272=EDGE_CURVE('',#5771,#5770,#363,.T.);
#7273=EDGE_CURVE('',#5606,#5771,#3561,.T.);
#7274=EDGE_CURVE('',#5608,#5772,#788,.T.);
#7275=EDGE_CURVE('',#5607,#5773,#3562,.T.);
#7276=EDGE_CURVE('',#5772,#5773,#364,.T.);
#7277=EDGE_CURVE('',#5773,#5771,#3563,.T.);
#7278=EDGE_CURVE('',#5774,#5772,#4776,.T.);
#7279=EDGE_CURVE('',#5774,#5609,#789,.T.);
#7280=EDGE_CURVE('',#5775,#5774,#365,.T.);
#7281=EDGE_CURVE('',#5610,#5775,#3564,.T.);
#7282=EDGE_CURVE('',#5612,#5776,#790,.T.);
#7283=EDGE_CURVE('',#5611,#5777,#3565,.T.);
#7284=EDGE_CURVE('',#5776,#5777,#366,.T.);
#7285=EDGE_CURVE('',#5777,#5775,#3566,.T.);
#7286=EDGE_CURVE('',#5778,#5776,#4777,.T.);
#7287=EDGE_CURVE('',#5778,#5613,#791,.T.);
#7288=EDGE_CURVE('',#5779,#5778,#367,.T.);
#7289=EDGE_CURVE('',#5614,#5779,#3567,.T.);
#7290=EDGE_CURVE('',#5780,#5779,#3568,.T.);
#7291=EDGE_CURVE('',#5615,#5780,#3569,.T.);
#7292=EDGE_CURVE('',#5616,#5781,#792,.T.);
#7293=EDGE_CURVE('',#5781,#5780,#368,.T.);
#7294=EDGE_CURVE('',#5782,#5781,#4778,.T.);
#7295=EDGE_CURVE('',#5782,#5617,#793,.T.);
#7296=EDGE_CURVE('',#5620,#5783,#794,.T.);
#7297=EDGE_CURVE('',#5619,#5784,#3570,.T.);
#7298=EDGE_CURVE('',#5783,#5784,#369,.T.);
#7299=EDGE_CURVE('',#5785,#5782,#370,.T.);
#7300=EDGE_CURVE('',#5618,#5785,#3571,.T.);
#7301=EDGE_CURVE('',#5784,#5785,#3572,.T.);
#7302=EDGE_CURVE('',#5626,#5783,#4779,.T.);
#9332=ORIENTED_EDGE('',*,*,#6808,.F.);
#9333=ORIENTED_EDGE('',*,*,#6809,.F.);
#9334=ORIENTED_EDGE('',*,*,#6810,.F.);
#9335=ORIENTED_EDGE('',*,*,#6811,.F.);
#9336=ORIENTED_EDGE('',*,*,#6812,.F.);
#9337=ORIENTED_EDGE('',*,*,#6813,.T.);
#9338=ORIENTED_EDGE('',*,*,#6814,.F.);
#9339=ORIENTED_EDGE('',*,*,#6809,.T.);
#9340=ORIENTED_EDGE('',*,*,#6815,.F.);
#9341=ORIENTED_EDGE('',*,*,#6816,.F.);
#9342=ORIENTED_EDGE('',*,*,#6817,.F.);
#9343=ORIENTED_EDGE('',*,*,#6813,.F.);
#9344=ORIENTED_EDGE('',*,*,#6818,.T.);
#9345=ORIENTED_EDGE('',*,*,#6819,.T.);
#9346=ORIENTED_EDGE('',*,*,#6820,.T.);
#9347=ORIENTED_EDGE('',*,*,#6821,.T.);
#9348=ORIENTED_EDGE('',*,*,#6822,.T.);
#9349=ORIENTED_EDGE('',*,*,#6823,.T.);
#9350=ORIENTED_EDGE('',*,*,#6824,.T.);
#9351=ORIENTED_EDGE('',*,*,#6825,.T.);
#9352=ORIENTED_EDGE('',*,*,#6826,.T.);
#9353=ORIENTED_EDGE('',*,*,#6827,.T.);
#9354=ORIENTED_EDGE('',*,*,#6828,.T.);
#9355=ORIENTED_EDGE('',*,*,#6829,.T.);
#9356=ORIENTED_EDGE('',*,*,#6830,.T.);
#9357=ORIENTED_EDGE('',*,*,#6831,.T.);
#9358=ORIENTED_EDGE('',*,*,#6832,.T.);
#9359=ORIENTED_EDGE('',*,*,#6833,.T.);
#9360=ORIENTED_EDGE('',*,*,#6834,.T.);
#9361=ORIENTED_EDGE('',*,*,#6835,.T.);
#9362=ORIENTED_EDGE('',*,*,#6836,.T.);
#9363=ORIENTED_EDGE('',*,*,#6837,.T.);
#9364=ORIENTED_EDGE('',*,*,#6838,.T.);
#9365=ORIENTED_EDGE('',*,*,#6839,.T.);
#9366=ORIENTED_EDGE('',*,*,#6840,.T.);
#9367=ORIENTED_EDGE('',*,*,#6841,.T.);
#9368=ORIENTED_EDGE('',*,*,#6842,.T.);
#9369=ORIENTED_EDGE('',*,*,#6843,.T.);
#9370=ORIENTED_EDGE('',*,*,#6844,.T.);
#9371=ORIENTED_EDGE('',*,*,#6845,.T.);
#9372=ORIENTED_EDGE('',*,*,#6846,.T.);
#9373=ORIENTED_EDGE('',*,*,#6847,.T.);
#9374=ORIENTED_EDGE('',*,*,#6848,.T.);
#9375=ORIENTED_EDGE('',*,*,#6849,.T.);
#9376=ORIENTED_EDGE('',*,*,#6850,.T.);
#9377=ORIENTED_EDGE('',*,*,#6851,.T.);
#9378=ORIENTED_EDGE('',*,*,#6852,.T.);
#9379=ORIENTED_EDGE('',*,*,#6853,.T.);
#9380=ORIENTED_EDGE('',*,*,#6854,.T.);
#9381=ORIENTED_EDGE('',*,*,#6855,.T.);
#9382=ORIENTED_EDGE('',*,*,#6856,.T.);
#9383=ORIENTED_EDGE('',*,*,#6857,.T.);
#9384=ORIENTED_EDGE('',*,*,#6858,.T.);
#9385=ORIENTED_EDGE('',*,*,#6859,.T.);
#9386=ORIENTED_EDGE('',*,*,#6860,.T.);
#9387=ORIENTED_EDGE('',*,*,#6861,.T.);
#9388=ORIENTED_EDGE('',*,*,#6862,.T.);
#9389=ORIENTED_EDGE('',*,*,#6863,.T.);
#9390=ORIENTED_EDGE('',*,*,#6864,.T.);
#9391=ORIENTED_EDGE('',*,*,#6865,.T.);
#9392=ORIENTED_EDGE('',*,*,#6866,.T.);
#9393=ORIENTED_EDGE('',*,*,#6867,.T.);
#9394=ORIENTED_EDGE('',*,*,#6868,.T.);
#9395=ORIENTED_EDGE('',*,*,#6869,.T.);
#9396=ORIENTED_EDGE('',*,*,#6870,.T.);
#9397=ORIENTED_EDGE('',*,*,#6871,.T.);
#9398=ORIENTED_EDGE('',*,*,#6872,.T.);
#9399=ORIENTED_EDGE('',*,*,#6873,.T.);
#9400=ORIENTED_EDGE('',*,*,#6874,.T.);
#9401=ORIENTED_EDGE('',*,*,#6875,.T.);
#9402=ORIENTED_EDGE('',*,*,#6876,.T.);
#9403=ORIENTED_EDGE('',*,*,#6877,.T.);
#9404=ORIENTED_EDGE('',*,*,#6878,.T.);
#9405=ORIENTED_EDGE('',*,*,#6879,.T.);
#9406=ORIENTED_EDGE('',*,*,#6880,.T.);
#9407=ORIENTED_EDGE('',*,*,#6881,.T.);
#9408=ORIENTED_EDGE('',*,*,#6882,.T.);
#9409=ORIENTED_EDGE('',*,*,#6883,.T.);
#9410=ORIENTED_EDGE('',*,*,#6884,.T.);
#9411=ORIENTED_EDGE('',*,*,#6885,.T.);
#9412=ORIENTED_EDGE('',*,*,#6886,.T.);
#9413=ORIENTED_EDGE('',*,*,#6887,.T.);
#9414=ORIENTED_EDGE('',*,*,#6888,.T.);
#9415=ORIENTED_EDGE('',*,*,#6889,.T.);
#9416=ORIENTED_EDGE('',*,*,#6890,.T.);
#9417=ORIENTED_EDGE('',*,*,#6891,.T.);
#9418=ORIENTED_EDGE('',*,*,#6892,.T.);
#9419=ORIENTED_EDGE('',*,*,#6893,.T.);
#9420=ORIENTED_EDGE('',*,*,#6894,.T.);
#9421=ORIENTED_EDGE('',*,*,#6895,.T.);
#9422=ORIENTED_EDGE('',*,*,#6896,.T.);
#9423=ORIENTED_EDGE('',*,*,#6897,.T.);
#9424=ORIENTED_EDGE('',*,*,#6898,.T.);
#9425=ORIENTED_EDGE('',*,*,#6899,.T.);
#9426=ORIENTED_EDGE('',*,*,#6900,.T.);
#9427=ORIENTED_EDGE('',*,*,#6901,.T.);
#9428=ORIENTED_EDGE('',*,*,#6902,.T.);
#9429=ORIENTED_EDGE('',*,*,#6903,.T.);
#9430=ORIENTED_EDGE('',*,*,#6904,.T.);
#9431=ORIENTED_EDGE('',*,*,#6905,.T.);
#9432=ORIENTED_EDGE('',*,*,#6906,.T.);
#9433=ORIENTED_EDGE('',*,*,#6907,.T.);
#9434=ORIENTED_EDGE('',*,*,#6908,.T.);
#9435=ORIENTED_EDGE('',*,*,#6909,.T.);
#9436=ORIENTED_EDGE('',*,*,#6910,.T.);
#9437=ORIENTED_EDGE('',*,*,#6911,.T.);
#9438=ORIENTED_EDGE('',*,*,#6912,.T.);
#9439=ORIENTED_EDGE('',*,*,#6913,.T.);
#9440=ORIENTED_EDGE('',*,*,#6914,.T.);
#9441=ORIENTED_EDGE('',*,*,#6915,.T.);
#9442=ORIENTED_EDGE('',*,*,#6916,.T.);
#9443=ORIENTED_EDGE('',*,*,#6917,.T.);
#9444=ORIENTED_EDGE('',*,*,#6918,.T.);
#9445=ORIENTED_EDGE('',*,*,#6919,.T.);
#9446=ORIENTED_EDGE('',*,*,#6920,.T.);
#9447=ORIENTED_EDGE('',*,*,#6921,.T.);
#9448=ORIENTED_EDGE('',*,*,#6922,.T.);
#9449=ORIENTED_EDGE('',*,*,#6923,.T.);
#9450=ORIENTED_EDGE('',*,*,#6924,.T.);
#9451=ORIENTED_EDGE('',*,*,#6925,.T.);
#9452=ORIENTED_EDGE('',*,*,#6926,.T.);
#9453=ORIENTED_EDGE('',*,*,#6927,.T.);
#9454=ORIENTED_EDGE('',*,*,#6928,.T.);
#9455=ORIENTED_EDGE('',*,*,#6929,.T.);
#9456=ORIENTED_EDGE('',*,*,#6930,.T.);
#9457=ORIENTED_EDGE('',*,*,#6931,.T.);
#9458=ORIENTED_EDGE('',*,*,#6932,.T.);
#9459=ORIENTED_EDGE('',*,*,#6933,.T.);
#9460=ORIENTED_EDGE('',*,*,#6934,.T.);
#9461=ORIENTED_EDGE('',*,*,#6935,.T.);
#9462=ORIENTED_EDGE('',*,*,#6936,.T.);
#9463=ORIENTED_EDGE('',*,*,#6937,.T.);
#9464=ORIENTED_EDGE('',*,*,#6938,.T.);
#9465=ORIENTED_EDGE('',*,*,#6939,.T.);
#9466=ORIENTED_EDGE('',*,*,#6940,.T.);
#9467=ORIENTED_EDGE('',*,*,#6941,.T.);
#9468=ORIENTED_EDGE('',*,*,#6942,.T.);
#9469=ORIENTED_EDGE('',*,*,#6943,.T.);
#9470=ORIENTED_EDGE('',*,*,#6944,.T.);
#9471=ORIENTED_EDGE('',*,*,#6945,.T.);
#9472=ORIENTED_EDGE('',*,*,#6946,.T.);
#9473=ORIENTED_EDGE('',*,*,#6947,.T.);
#9474=ORIENTED_EDGE('',*,*,#6948,.T.);
#9475=ORIENTED_EDGE('',*,*,#6949,.T.);
#9476=ORIENTED_EDGE('',*,*,#6950,.T.);
#9477=ORIENTED_EDGE('',*,*,#6951,.T.);
#9478=ORIENTED_EDGE('',*,*,#6952,.T.);
#9479=ORIENTED_EDGE('',*,*,#6953,.T.);
#9480=ORIENTED_EDGE('',*,*,#6954,.T.);
#9481=ORIENTED_EDGE('',*,*,#6955,.T.);
#9482=ORIENTED_EDGE('',*,*,#6956,.T.);
#9483=ORIENTED_EDGE('',*,*,#6957,.T.);
#9484=ORIENTED_EDGE('',*,*,#6958,.T.);
#9485=ORIENTED_EDGE('',*,*,#6959,.T.);
#9486=ORIENTED_EDGE('',*,*,#6960,.T.);
#9487=ORIENTED_EDGE('',*,*,#6961,.T.);
#9488=ORIENTED_EDGE('',*,*,#6962,.T.);
#9489=ORIENTED_EDGE('',*,*,#6963,.T.);
#9490=ORIENTED_EDGE('',*,*,#6964,.T.);
#9491=ORIENTED_EDGE('',*,*,#6965,.T.);
#9492=ORIENTED_EDGE('',*,*,#6966,.T.);
#9493=ORIENTED_EDGE('',*,*,#6967,.T.);
#9494=ORIENTED_EDGE('',*,*,#6968,.T.);
#9495=ORIENTED_EDGE('',*,*,#6969,.T.);
#9496=ORIENTED_EDGE('',*,*,#6970,.T.);
#9497=ORIENTED_EDGE('',*,*,#6971,.T.);
#9498=ORIENTED_EDGE('',*,*,#6972,.T.);
#9499=ORIENTED_EDGE('',*,*,#6973,.T.);
#9500=ORIENTED_EDGE('',*,*,#6974,.T.);
#9501=ORIENTED_EDGE('',*,*,#6975,.T.);
#9502=ORIENTED_EDGE('',*,*,#6976,.T.);
#9503=ORIENTED_EDGE('',*,*,#6977,.T.);
#9504=ORIENTED_EDGE('',*,*,#6810,.T.);
#9505=ORIENTED_EDGE('',*,*,#6814,.T.);
#9506=ORIENTED_EDGE('',*,*,#6817,.T.);
#9507=ORIENTED_EDGE('',*,*,#6978,.T.);
#9508=ORIENTED_EDGE('',*,*,#6811,.T.);
#9509=ORIENTED_EDGE('',*,*,#6978,.F.);
#9510=ORIENTED_EDGE('',*,*,#6816,.T.);
#9511=ORIENTED_EDGE('',*,*,#6979,.F.);
#9512=ORIENTED_EDGE('',*,*,#6980,.F.);
#9513=ORIENTED_EDGE('',*,*,#6981,.T.);
#9514=ORIENTED_EDGE('',*,*,#6982,.F.);
#9515=ORIENTED_EDGE('',*,*,#6981,.F.);
#9516=ORIENTED_EDGE('',*,*,#6980,.T.);
#9517=ORIENTED_EDGE('',*,*,#6808,.T.);
#9518=ORIENTED_EDGE('',*,*,#6979,.T.);
#9519=ORIENTED_EDGE('',*,*,#6815,.T.);
#9520=ORIENTED_EDGE('',*,*,#6812,.T.);
#9521=ORIENTED_EDGE('',*,*,#6983,.F.);
#9522=ORIENTED_EDGE('',*,*,#6984,.F.);
#9523=ORIENTED_EDGE('',*,*,#6985,.F.);
#9524=ORIENTED_EDGE('',*,*,#6975,.F.);
#9525=ORIENTED_EDGE('',*,*,#6986,.F.);
#9526=ORIENTED_EDGE('',*,*,#6977,.F.);
#9527=ORIENTED_EDGE('',*,*,#6987,.T.);
#9528=ORIENTED_EDGE('',*,*,#6988,.F.);
#9529=ORIENTED_EDGE('',*,*,#6985,.T.);
#9530=ORIENTED_EDGE('',*,*,#6989,.F.);
#9531=ORIENTED_EDGE('',*,*,#6987,.F.);
#9532=ORIENTED_EDGE('',*,*,#6976,.F.);
#9533=ORIENTED_EDGE('',*,*,#6986,.T.);
#9534=ORIENTED_EDGE('',*,*,#6990,.F.);
#9535=ORIENTED_EDGE('',*,*,#6991,.T.);
#9536=ORIENTED_EDGE('',*,*,#6818,.F.);
#9537=ORIENTED_EDGE('',*,*,#6991,.F.);
#9538=ORIENTED_EDGE('',*,*,#6992,.F.);
#9539=ORIENTED_EDGE('',*,*,#6993,.F.);
#9540=ORIENTED_EDGE('',*,*,#6819,.F.);
#9541=ORIENTED_EDGE('',*,*,#6994,.F.);
#9542=ORIENTED_EDGE('',*,*,#6821,.F.);
#9543=ORIENTED_EDGE('',*,*,#6995,.T.);
#9544=ORIENTED_EDGE('',*,*,#6996,.F.);
#9545=ORIENTED_EDGE('',*,*,#6993,.T.);
#9546=ORIENTED_EDGE('',*,*,#6997,.F.);
#9547=ORIENTED_EDGE('',*,*,#6995,.F.);
#9548=ORIENTED_EDGE('',*,*,#6820,.F.);
#9549=ORIENTED_EDGE('',*,*,#6994,.T.);
#9550=ORIENTED_EDGE('',*,*,#6998,.F.);
#9551=ORIENTED_EDGE('',*,*,#6999,.T.);
#9552=ORIENTED_EDGE('',*,*,#6822,.F.);
#9553=ORIENTED_EDGE('',*,*,#6999,.F.);
#9554=ORIENTED_EDGE('',*,*,#7000,.F.);
#9555=ORIENTED_EDGE('',*,*,#7001,.F.);
#9556=ORIENTED_EDGE('',*,*,#6823,.F.);
#9557=ORIENTED_EDGE('',*,*,#7002,.F.);
#9558=ORIENTED_EDGE('',*,*,#6825,.F.);
#9559=ORIENTED_EDGE('',*,*,#7003,.T.);
#9560=ORIENTED_EDGE('',*,*,#7004,.F.);
#9561=ORIENTED_EDGE('',*,*,#7001,.T.);
#9562=ORIENTED_EDGE('',*,*,#7005,.F.);
#9563=ORIENTED_EDGE('',*,*,#7003,.F.);
#9564=ORIENTED_EDGE('',*,*,#6824,.F.);
#9565=ORIENTED_EDGE('',*,*,#7002,.T.);
#9566=ORIENTED_EDGE('',*,*,#7006,.F.);
#9567=ORIENTED_EDGE('',*,*,#7007,.T.);
#9568=ORIENTED_EDGE('',*,*,#6826,.F.);
#9569=ORIENTED_EDGE('',*,*,#7007,.F.);
#9570=ORIENTED_EDGE('',*,*,#7008,.F.);
#9571=ORIENTED_EDGE('',*,*,#7009,.F.);
#9572=ORIENTED_EDGE('',*,*,#6827,.F.);
#9573=ORIENTED_EDGE('',*,*,#7010,.F.);
#9574=ORIENTED_EDGE('',*,*,#6829,.F.);
#9575=ORIENTED_EDGE('',*,*,#7011,.T.);
#9576=ORIENTED_EDGE('',*,*,#7012,.F.);
#9577=ORIENTED_EDGE('',*,*,#7009,.T.);
#9578=ORIENTED_EDGE('',*,*,#7013,.F.);
#9579=ORIENTED_EDGE('',*,*,#7011,.F.);
#9580=ORIENTED_EDGE('',*,*,#6828,.F.);
#9581=ORIENTED_EDGE('',*,*,#7010,.T.);
#9582=ORIENTED_EDGE('',*,*,#7014,.F.);
#9583=ORIENTED_EDGE('',*,*,#7015,.T.);
#9584=ORIENTED_EDGE('',*,*,#6830,.F.);
#9585=ORIENTED_EDGE('',*,*,#7015,.F.);
#9586=ORIENTED_EDGE('',*,*,#7016,.F.);
#9587=ORIENTED_EDGE('',*,*,#7017,.F.);
#9588=ORIENTED_EDGE('',*,*,#6831,.F.);
#9589=ORIENTED_EDGE('',*,*,#7018,.F.);
#9590=ORIENTED_EDGE('',*,*,#6833,.F.);
#9591=ORIENTED_EDGE('',*,*,#7019,.T.);
#9592=ORIENTED_EDGE('',*,*,#7020,.F.);
#9593=ORIENTED_EDGE('',*,*,#7017,.T.);
#9594=ORIENTED_EDGE('',*,*,#7021,.F.);
#9595=ORIENTED_EDGE('',*,*,#7019,.F.);
#9596=ORIENTED_EDGE('',*,*,#6832,.F.);
#9597=ORIENTED_EDGE('',*,*,#7018,.T.);
#9598=ORIENTED_EDGE('',*,*,#7022,.F.);
#9599=ORIENTED_EDGE('',*,*,#7023,.T.);
#9600=ORIENTED_EDGE('',*,*,#6834,.F.);
#9601=ORIENTED_EDGE('',*,*,#7023,.F.);
#9602=ORIENTED_EDGE('',*,*,#7024,.F.);
#9603=ORIENTED_EDGE('',*,*,#7025,.F.);
#9604=ORIENTED_EDGE('',*,*,#6835,.F.);
#9605=ORIENTED_EDGE('',*,*,#7026,.F.);
#9606=ORIENTED_EDGE('',*,*,#6837,.F.);
#9607=ORIENTED_EDGE('',*,*,#7027,.T.);
#9608=ORIENTED_EDGE('',*,*,#7028,.F.);
#9609=ORIENTED_EDGE('',*,*,#7025,.T.);
#9610=ORIENTED_EDGE('',*,*,#7029,.F.);
#9611=ORIENTED_EDGE('',*,*,#7027,.F.);
#9612=ORIENTED_EDGE('',*,*,#6836,.F.);
#9613=ORIENTED_EDGE('',*,*,#7026,.T.);
#9614=ORIENTED_EDGE('',*,*,#7030,.F.);
#9615=ORIENTED_EDGE('',*,*,#7031,.T.);
#9616=ORIENTED_EDGE('',*,*,#6838,.F.);
#9617=ORIENTED_EDGE('',*,*,#7031,.F.);
#9618=ORIENTED_EDGE('',*,*,#7032,.F.);
#9619=ORIENTED_EDGE('',*,*,#7033,.F.);
#9620=ORIENTED_EDGE('',*,*,#6839,.F.);
#9621=ORIENTED_EDGE('',*,*,#7034,.F.);
#9622=ORIENTED_EDGE('',*,*,#6841,.F.);
#9623=ORIENTED_EDGE('',*,*,#7035,.T.);
#9624=ORIENTED_EDGE('',*,*,#7036,.F.);
#9625=ORIENTED_EDGE('',*,*,#7033,.T.);
#9626=ORIENTED_EDGE('',*,*,#7037,.F.);
#9627=ORIENTED_EDGE('',*,*,#7035,.F.);
#9628=ORIENTED_EDGE('',*,*,#6840,.F.);
#9629=ORIENTED_EDGE('',*,*,#7034,.T.);
#9630=ORIENTED_EDGE('',*,*,#7038,.F.);
#9631=ORIENTED_EDGE('',*,*,#7039,.T.);
#9632=ORIENTED_EDGE('',*,*,#6842,.F.);
#9633=ORIENTED_EDGE('',*,*,#7039,.F.);
#9634=ORIENTED_EDGE('',*,*,#7040,.F.);
#9635=ORIENTED_EDGE('',*,*,#7041,.F.);
#9636=ORIENTED_EDGE('',*,*,#6843,.F.);
#9637=ORIENTED_EDGE('',*,*,#7042,.F.);
#9638=ORIENTED_EDGE('',*,*,#6845,.F.);
#9639=ORIENTED_EDGE('',*,*,#7043,.T.);
#9640=ORIENTED_EDGE('',*,*,#7044,.F.);
#9641=ORIENTED_EDGE('',*,*,#7041,.T.);
#9642=ORIENTED_EDGE('',*,*,#7045,.F.);
#9643=ORIENTED_EDGE('',*,*,#7043,.F.);
#9644=ORIENTED_EDGE('',*,*,#6844,.F.);
#9645=ORIENTED_EDGE('',*,*,#7042,.T.);
#9646=ORIENTED_EDGE('',*,*,#7046,.F.);
#9647=ORIENTED_EDGE('',*,*,#7047,.T.);
#9648=ORIENTED_EDGE('',*,*,#6846,.F.);
#9649=ORIENTED_EDGE('',*,*,#7047,.F.);
#9650=ORIENTED_EDGE('',*,*,#7048,.F.);
#9651=ORIENTED_EDGE('',*,*,#7049,.F.);
#9652=ORIENTED_EDGE('',*,*,#6847,.F.);
#9653=ORIENTED_EDGE('',*,*,#7050,.F.);
#9654=ORIENTED_EDGE('',*,*,#6849,.F.);
#9655=ORIENTED_EDGE('',*,*,#7051,.T.);
#9656=ORIENTED_EDGE('',*,*,#7052,.F.);
#9657=ORIENTED_EDGE('',*,*,#7049,.T.);
#9658=ORIENTED_EDGE('',*,*,#7053,.F.);
#9659=ORIENTED_EDGE('',*,*,#7051,.F.);
#9660=ORIENTED_EDGE('',*,*,#6848,.F.);
#9661=ORIENTED_EDGE('',*,*,#7050,.T.);
#9662=ORIENTED_EDGE('',*,*,#7054,.F.);
#9663=ORIENTED_EDGE('',*,*,#7055,.T.);
#9664=ORIENTED_EDGE('',*,*,#6850,.F.);
#9665=ORIENTED_EDGE('',*,*,#7055,.F.);
#9666=ORIENTED_EDGE('',*,*,#7056,.F.);
#9667=ORIENTED_EDGE('',*,*,#7057,.F.);
#9668=ORIENTED_EDGE('',*,*,#6851,.F.);
#9669=ORIENTED_EDGE('',*,*,#7058,.F.);
#9670=ORIENTED_EDGE('',*,*,#6853,.F.);
#9671=ORIENTED_EDGE('',*,*,#7059,.T.);
#9672=ORIENTED_EDGE('',*,*,#7060,.F.);
#9673=ORIENTED_EDGE('',*,*,#7057,.T.);
#9674=ORIENTED_EDGE('',*,*,#7061,.F.);
#9675=ORIENTED_EDGE('',*,*,#7059,.F.);
#9676=ORIENTED_EDGE('',*,*,#6852,.F.);
#9677=ORIENTED_EDGE('',*,*,#7058,.T.);
#9678=ORIENTED_EDGE('',*,*,#7062,.F.);
#9679=ORIENTED_EDGE('',*,*,#7063,.T.);
#9680=ORIENTED_EDGE('',*,*,#6854,.F.);
#9681=ORIENTED_EDGE('',*,*,#7063,.F.);
#9682=ORIENTED_EDGE('',*,*,#7064,.F.);
#9683=ORIENTED_EDGE('',*,*,#7065,.F.);
#9684=ORIENTED_EDGE('',*,*,#6855,.F.);
#9685=ORIENTED_EDGE('',*,*,#7066,.F.);
#9686=ORIENTED_EDGE('',*,*,#6857,.F.);
#9687=ORIENTED_EDGE('',*,*,#7067,.T.);
#9688=ORIENTED_EDGE('',*,*,#7068,.F.);
#9689=ORIENTED_EDGE('',*,*,#7065,.T.);
#9690=ORIENTED_EDGE('',*,*,#7069,.F.);
#9691=ORIENTED_EDGE('',*,*,#7067,.F.);
#9692=ORIENTED_EDGE('',*,*,#6856,.F.);
#9693=ORIENTED_EDGE('',*,*,#7066,.T.);
#9694=ORIENTED_EDGE('',*,*,#7070,.F.);
#9695=ORIENTED_EDGE('',*,*,#7071,.T.);
#9696=ORIENTED_EDGE('',*,*,#6858,.F.);
#9697=ORIENTED_EDGE('',*,*,#7071,.F.);
#9698=ORIENTED_EDGE('',*,*,#7072,.F.);
#9699=ORIENTED_EDGE('',*,*,#7073,.F.);
#9700=ORIENTED_EDGE('',*,*,#6859,.F.);
#9701=ORIENTED_EDGE('',*,*,#7074,.F.);
#9702=ORIENTED_EDGE('',*,*,#6861,.F.);
#9703=ORIENTED_EDGE('',*,*,#7075,.T.);
#9704=ORIENTED_EDGE('',*,*,#7076,.F.);
#9705=ORIENTED_EDGE('',*,*,#7073,.T.);
#9706=ORIENTED_EDGE('',*,*,#7077,.F.);
#9707=ORIENTED_EDGE('',*,*,#7075,.F.);
#9708=ORIENTED_EDGE('',*,*,#6860,.F.);
#9709=ORIENTED_EDGE('',*,*,#7074,.T.);
#9710=ORIENTED_EDGE('',*,*,#7078,.F.);
#9711=ORIENTED_EDGE('',*,*,#7079,.T.);
#9712=ORIENTED_EDGE('',*,*,#6862,.F.);
#9713=ORIENTED_EDGE('',*,*,#7079,.F.);
#9714=ORIENTED_EDGE('',*,*,#7080,.F.);
#9715=ORIENTED_EDGE('',*,*,#7081,.F.);
#9716=ORIENTED_EDGE('',*,*,#6863,.F.);
#9717=ORIENTED_EDGE('',*,*,#7082,.F.);
#9718=ORIENTED_EDGE('',*,*,#6865,.F.);
#9719=ORIENTED_EDGE('',*,*,#7083,.T.);
#9720=ORIENTED_EDGE('',*,*,#7084,.F.);
#9721=ORIENTED_EDGE('',*,*,#7081,.T.);
#9722=ORIENTED_EDGE('',*,*,#7085,.F.);
#9723=ORIENTED_EDGE('',*,*,#7083,.F.);
#9724=ORIENTED_EDGE('',*,*,#6864,.F.);
#9725=ORIENTED_EDGE('',*,*,#7082,.T.);
#9726=ORIENTED_EDGE('',*,*,#7086,.F.);
#9727=ORIENTED_EDGE('',*,*,#7087,.T.);
#9728=ORIENTED_EDGE('',*,*,#6866,.F.);
#9729=ORIENTED_EDGE('',*,*,#7087,.F.);
#9730=ORIENTED_EDGE('',*,*,#7088,.F.);
#9731=ORIENTED_EDGE('',*,*,#7089,.F.);
#9732=ORIENTED_EDGE('',*,*,#6867,.F.);
#9733=ORIENTED_EDGE('',*,*,#7090,.F.);
#9734=ORIENTED_EDGE('',*,*,#6869,.F.);
#9735=ORIENTED_EDGE('',*,*,#7091,.T.);
#9736=ORIENTED_EDGE('',*,*,#7092,.F.);
#9737=ORIENTED_EDGE('',*,*,#7089,.T.);
#9738=ORIENTED_EDGE('',*,*,#7093,.F.);
#9739=ORIENTED_EDGE('',*,*,#7091,.F.);
#9740=ORIENTED_EDGE('',*,*,#6868,.F.);
#9741=ORIENTED_EDGE('',*,*,#7090,.T.);
#9742=ORIENTED_EDGE('',*,*,#7094,.F.);
#9743=ORIENTED_EDGE('',*,*,#7095,.T.);
#9744=ORIENTED_EDGE('',*,*,#6870,.F.);
#9745=ORIENTED_EDGE('',*,*,#7095,.F.);
#9746=ORIENTED_EDGE('',*,*,#7096,.F.);
#9747=ORIENTED_EDGE('',*,*,#7097,.F.);
#9748=ORIENTED_EDGE('',*,*,#6871,.F.);
#9749=ORIENTED_EDGE('',*,*,#7098,.F.);
#9750=ORIENTED_EDGE('',*,*,#6873,.F.);
#9751=ORIENTED_EDGE('',*,*,#7099,.T.);
#9752=ORIENTED_EDGE('',*,*,#7100,.F.);
#9753=ORIENTED_EDGE('',*,*,#7097,.T.);
#9754=ORIENTED_EDGE('',*,*,#7101,.F.);
#9755=ORIENTED_EDGE('',*,*,#7099,.F.);
#9756=ORIENTED_EDGE('',*,*,#6872,.F.);
#9757=ORIENTED_EDGE('',*,*,#7098,.T.);
#9758=ORIENTED_EDGE('',*,*,#7102,.F.);
#9759=ORIENTED_EDGE('',*,*,#7103,.T.);
#9760=ORIENTED_EDGE('',*,*,#6874,.F.);
#9761=ORIENTED_EDGE('',*,*,#7103,.F.);
#9762=ORIENTED_EDGE('',*,*,#7104,.F.);
#9763=ORIENTED_EDGE('',*,*,#7105,.F.);
#9764=ORIENTED_EDGE('',*,*,#6875,.F.);
#9765=ORIENTED_EDGE('',*,*,#7106,.F.);
#9766=ORIENTED_EDGE('',*,*,#6877,.F.);
#9767=ORIENTED_EDGE('',*,*,#7107,.T.);
#9768=ORIENTED_EDGE('',*,*,#7108,.F.);
#9769=ORIENTED_EDGE('',*,*,#7105,.T.);
#9770=ORIENTED_EDGE('',*,*,#7109,.F.);
#9771=ORIENTED_EDGE('',*,*,#7107,.F.);
#9772=ORIENTED_EDGE('',*,*,#6876,.F.);
#9773=ORIENTED_EDGE('',*,*,#7106,.T.);
#9774=ORIENTED_EDGE('',*,*,#7110,.F.);
#9775=ORIENTED_EDGE('',*,*,#7111,.T.);
#9776=ORIENTED_EDGE('',*,*,#6878,.F.);
#9777=ORIENTED_EDGE('',*,*,#7111,.F.);
#9778=ORIENTED_EDGE('',*,*,#7112,.F.);
#9779=ORIENTED_EDGE('',*,*,#7113,.F.);
#9780=ORIENTED_EDGE('',*,*,#6879,.F.);
#9781=ORIENTED_EDGE('',*,*,#7114,.F.);
#9782=ORIENTED_EDGE('',*,*,#6881,.F.);
#9783=ORIENTED_EDGE('',*,*,#7115,.T.);
#9784=ORIENTED_EDGE('',*,*,#7116,.F.);
#9785=ORIENTED_EDGE('',*,*,#7113,.T.);
#9786=ORIENTED_EDGE('',*,*,#7117,.F.);
#9787=ORIENTED_EDGE('',*,*,#7115,.F.);
#9788=ORIENTED_EDGE('',*,*,#6880,.F.);
#9789=ORIENTED_EDGE('',*,*,#7114,.T.);
#9790=ORIENTED_EDGE('',*,*,#7118,.F.);
#9791=ORIENTED_EDGE('',*,*,#7119,.T.);
#9792=ORIENTED_EDGE('',*,*,#6882,.F.);
#9793=ORIENTED_EDGE('',*,*,#7119,.F.);
#9794=ORIENTED_EDGE('',*,*,#7120,.F.);
#9795=ORIENTED_EDGE('',*,*,#7121,.F.);
#9796=ORIENTED_EDGE('',*,*,#6883,.F.);
#9797=ORIENTED_EDGE('',*,*,#7122,.F.);
#9798=ORIENTED_EDGE('',*,*,#6885,.F.);
#9799=ORIENTED_EDGE('',*,*,#7123,.T.);
#9800=ORIENTED_EDGE('',*,*,#7124,.F.);
#9801=ORIENTED_EDGE('',*,*,#7121,.T.);
#9802=ORIENTED_EDGE('',*,*,#7125,.F.);
#9803=ORIENTED_EDGE('',*,*,#7123,.F.);
#9804=ORIENTED_EDGE('',*,*,#6884,.F.);
#9805=ORIENTED_EDGE('',*,*,#7122,.T.);
#9806=ORIENTED_EDGE('',*,*,#7126,.F.);
#9807=ORIENTED_EDGE('',*,*,#7127,.T.);
#9808=ORIENTED_EDGE('',*,*,#6886,.F.);
#9809=ORIENTED_EDGE('',*,*,#7127,.F.);
#9810=ORIENTED_EDGE('',*,*,#7128,.F.);
#9811=ORIENTED_EDGE('',*,*,#7129,.F.);
#9812=ORIENTED_EDGE('',*,*,#6887,.F.);
#9813=ORIENTED_EDGE('',*,*,#7130,.F.);
#9814=ORIENTED_EDGE('',*,*,#6889,.F.);
#9815=ORIENTED_EDGE('',*,*,#7131,.T.);
#9816=ORIENTED_EDGE('',*,*,#7132,.F.);
#9817=ORIENTED_EDGE('',*,*,#7129,.T.);
#9818=ORIENTED_EDGE('',*,*,#7133,.F.);
#9819=ORIENTED_EDGE('',*,*,#7131,.F.);
#9820=ORIENTED_EDGE('',*,*,#6888,.F.);
#9821=ORIENTED_EDGE('',*,*,#7130,.T.);
#9822=ORIENTED_EDGE('',*,*,#7134,.F.);
#9823=ORIENTED_EDGE('',*,*,#7135,.T.);
#9824=ORIENTED_EDGE('',*,*,#6890,.F.);
#9825=ORIENTED_EDGE('',*,*,#7135,.F.);
#9826=ORIENTED_EDGE('',*,*,#7136,.F.);
#9827=ORIENTED_EDGE('',*,*,#7137,.F.);
#9828=ORIENTED_EDGE('',*,*,#6891,.F.);
#9829=ORIENTED_EDGE('',*,*,#7138,.F.);
#9830=ORIENTED_EDGE('',*,*,#6893,.F.);
#9831=ORIENTED_EDGE('',*,*,#7139,.T.);
#9832=ORIENTED_EDGE('',*,*,#7140,.F.);
#9833=ORIENTED_EDGE('',*,*,#7137,.T.);
#9834=ORIENTED_EDGE('',*,*,#7141,.F.);
#9835=ORIENTED_EDGE('',*,*,#7139,.F.);
#9836=ORIENTED_EDGE('',*,*,#6892,.F.);
#9837=ORIENTED_EDGE('',*,*,#7138,.T.);
#9838=ORIENTED_EDGE('',*,*,#7142,.F.);
#9839=ORIENTED_EDGE('',*,*,#7143,.T.);
#9840=ORIENTED_EDGE('',*,*,#6894,.F.);
#9841=ORIENTED_EDGE('',*,*,#7143,.F.);
#9842=ORIENTED_EDGE('',*,*,#7144,.F.);
#9843=ORIENTED_EDGE('',*,*,#7145,.F.);
#9844=ORIENTED_EDGE('',*,*,#6895,.F.);
#9845=ORIENTED_EDGE('',*,*,#7146,.F.);
#9846=ORIENTED_EDGE('',*,*,#6897,.F.);
#9847=ORIENTED_EDGE('',*,*,#7147,.T.);
#9848=ORIENTED_EDGE('',*,*,#7148,.F.);
#9849=ORIENTED_EDGE('',*,*,#7145,.T.);
#9850=ORIENTED_EDGE('',*,*,#7149,.F.);
#9851=ORIENTED_EDGE('',*,*,#7147,.F.);
#9852=ORIENTED_EDGE('',*,*,#6896,.F.);
#9853=ORIENTED_EDGE('',*,*,#7146,.T.);
#9854=ORIENTED_EDGE('',*,*,#7150,.F.);
#9855=ORIENTED_EDGE('',*,*,#7151,.T.);
#9856=ORIENTED_EDGE('',*,*,#6898,.F.);
#9857=ORIENTED_EDGE('',*,*,#7151,.F.);
#9858=ORIENTED_EDGE('',*,*,#7152,.F.);
#9859=ORIENTED_EDGE('',*,*,#7153,.F.);
#9860=ORIENTED_EDGE('',*,*,#6899,.F.);
#9861=ORIENTED_EDGE('',*,*,#7154,.F.);
#9862=ORIENTED_EDGE('',*,*,#6901,.F.);
#9863=ORIENTED_EDGE('',*,*,#7155,.T.);
#9864=ORIENTED_EDGE('',*,*,#7156,.F.);
#9865=ORIENTED_EDGE('',*,*,#7153,.T.);
#9866=ORIENTED_EDGE('',*,*,#7157,.F.);
#9867=ORIENTED_EDGE('',*,*,#7155,.F.);
#9868=ORIENTED_EDGE('',*,*,#6900,.F.);
#9869=ORIENTED_EDGE('',*,*,#7154,.T.);
#9870=ORIENTED_EDGE('',*,*,#7158,.F.);
#9871=ORIENTED_EDGE('',*,*,#7159,.T.);
#9872=ORIENTED_EDGE('',*,*,#6902,.F.);
#9873=ORIENTED_EDGE('',*,*,#7159,.F.);
#9874=ORIENTED_EDGE('',*,*,#7160,.F.);
#9875=ORIENTED_EDGE('',*,*,#7161,.F.);
#9876=ORIENTED_EDGE('',*,*,#6903,.F.);
#9877=ORIENTED_EDGE('',*,*,#7162,.F.);
#9878=ORIENTED_EDGE('',*,*,#6905,.F.);
#9879=ORIENTED_EDGE('',*,*,#7163,.T.);
#9880=ORIENTED_EDGE('',*,*,#7164,.F.);
#9881=ORIENTED_EDGE('',*,*,#7161,.T.);
#9882=ORIENTED_EDGE('',*,*,#7165,.F.);
#9883=ORIENTED_EDGE('',*,*,#7163,.F.);
#9884=ORIENTED_EDGE('',*,*,#6904,.F.);
#9885=ORIENTED_EDGE('',*,*,#7162,.T.);
#9886=ORIENTED_EDGE('',*,*,#7166,.F.);
#9887=ORIENTED_EDGE('',*,*,#7167,.T.);
#9888=ORIENTED_EDGE('',*,*,#6906,.F.);
#9889=ORIENTED_EDGE('',*,*,#7167,.F.);
#9890=ORIENTED_EDGE('',*,*,#7168,.F.);
#9891=ORIENTED_EDGE('',*,*,#7169,.F.);
#9892=ORIENTED_EDGE('',*,*,#6907,.F.);
#9893=ORIENTED_EDGE('',*,*,#7170,.F.);
#9894=ORIENTED_EDGE('',*,*,#6909,.F.);
#9895=ORIENTED_EDGE('',*,*,#7171,.T.);
#9896=ORIENTED_EDGE('',*,*,#7172,.F.);
#9897=ORIENTED_EDGE('',*,*,#7169,.T.);
#9898=ORIENTED_EDGE('',*,*,#7173,.F.);
#9899=ORIENTED_EDGE('',*,*,#7171,.F.);
#9900=ORIENTED_EDGE('',*,*,#6908,.F.);
#9901=ORIENTED_EDGE('',*,*,#7170,.T.);
#9902=ORIENTED_EDGE('',*,*,#7174,.F.);
#9903=ORIENTED_EDGE('',*,*,#7175,.T.);
#9904=ORIENTED_EDGE('',*,*,#6910,.F.);
#9905=ORIENTED_EDGE('',*,*,#7175,.F.);
#9906=ORIENTED_EDGE('',*,*,#7176,.F.);
#9907=ORIENTED_EDGE('',*,*,#7177,.F.);
#9908=ORIENTED_EDGE('',*,*,#6911,.F.);
#9909=ORIENTED_EDGE('',*,*,#7178,.F.);
#9910=ORIENTED_EDGE('',*,*,#6913,.F.);
#9911=ORIENTED_EDGE('',*,*,#7179,.T.);
#9912=ORIENTED_EDGE('',*,*,#7180,.F.);
#9913=ORIENTED_EDGE('',*,*,#7177,.T.);
#9914=ORIENTED_EDGE('',*,*,#7181,.F.);
#9915=ORIENTED_EDGE('',*,*,#7179,.F.);
#9916=ORIENTED_EDGE('',*,*,#6912,.F.);
#9917=ORIENTED_EDGE('',*,*,#7178,.T.);
#9918=ORIENTED_EDGE('',*,*,#7182,.F.);
#9919=ORIENTED_EDGE('',*,*,#7183,.T.);
#9920=ORIENTED_EDGE('',*,*,#6914,.F.);
#9921=ORIENTED_EDGE('',*,*,#7183,.F.);
#9922=ORIENTED_EDGE('',*,*,#7184,.F.);
#9923=ORIENTED_EDGE('',*,*,#7185,.F.);
#9924=ORIENTED_EDGE('',*,*,#6915,.F.);
#9925=ORIENTED_EDGE('',*,*,#7186,.F.);
#9926=ORIENTED_EDGE('',*,*,#6917,.F.);
#9927=ORIENTED_EDGE('',*,*,#7187,.T.);
#9928=ORIENTED_EDGE('',*,*,#7188,.F.);
#9929=ORIENTED_EDGE('',*,*,#7185,.T.);
#9930=ORIENTED_EDGE('',*,*,#7189,.F.);
#9931=ORIENTED_EDGE('',*,*,#7187,.F.);
#9932=ORIENTED_EDGE('',*,*,#6916,.F.);
#9933=ORIENTED_EDGE('',*,*,#7186,.T.);
#9934=ORIENTED_EDGE('',*,*,#7190,.F.);
#9935=ORIENTED_EDGE('',*,*,#7191,.T.);
#9936=ORIENTED_EDGE('',*,*,#6918,.F.);
#9937=ORIENTED_EDGE('',*,*,#7191,.F.);
#9938=ORIENTED_EDGE('',*,*,#7192,.F.);
#9939=ORIENTED_EDGE('',*,*,#7193,.F.);
#9940=ORIENTED_EDGE('',*,*,#6919,.F.);
#9941=ORIENTED_EDGE('',*,*,#7194,.F.);
#9942=ORIENTED_EDGE('',*,*,#6921,.F.);
#9943=ORIENTED_EDGE('',*,*,#7195,.T.);
#9944=ORIENTED_EDGE('',*,*,#7196,.F.);
#9945=ORIENTED_EDGE('',*,*,#7193,.T.);
#9946=ORIENTED_EDGE('',*,*,#7197,.F.);
#9947=ORIENTED_EDGE('',*,*,#7195,.F.);
#9948=ORIENTED_EDGE('',*,*,#6920,.F.);
#9949=ORIENTED_EDGE('',*,*,#7194,.T.);
#9950=ORIENTED_EDGE('',*,*,#7198,.F.);
#9951=ORIENTED_EDGE('',*,*,#7199,.T.);
#9952=ORIENTED_EDGE('',*,*,#6922,.F.);
#9953=ORIENTED_EDGE('',*,*,#7199,.F.);
#9954=ORIENTED_EDGE('',*,*,#7200,.F.);
#9955=ORIENTED_EDGE('',*,*,#7201,.F.);
#9956=ORIENTED_EDGE('',*,*,#6923,.F.);
#9957=ORIENTED_EDGE('',*,*,#7202,.F.);
#9958=ORIENTED_EDGE('',*,*,#6925,.F.);
#9959=ORIENTED_EDGE('',*,*,#7203,.T.);
#9960=ORIENTED_EDGE('',*,*,#7204,.F.);
#9961=ORIENTED_EDGE('',*,*,#7201,.T.);
#9962=ORIENTED_EDGE('',*,*,#7205,.F.);
#9963=ORIENTED_EDGE('',*,*,#7203,.F.);
#9964=ORIENTED_EDGE('',*,*,#6924,.F.);
#9965=ORIENTED_EDGE('',*,*,#7202,.T.);
#9966=ORIENTED_EDGE('',*,*,#7206,.F.);
#9967=ORIENTED_EDGE('',*,*,#7207,.T.);
#9968=ORIENTED_EDGE('',*,*,#6926,.F.);
#9969=ORIENTED_EDGE('',*,*,#7207,.F.);
#9970=ORIENTED_EDGE('',*,*,#7208,.F.);
#9971=ORIENTED_EDGE('',*,*,#7209,.F.);
#9972=ORIENTED_EDGE('',*,*,#6927,.F.);
#9973=ORIENTED_EDGE('',*,*,#7210,.F.);
#9974=ORIENTED_EDGE('',*,*,#6929,.F.);
#9975=ORIENTED_EDGE('',*,*,#7211,.T.);
#9976=ORIENTED_EDGE('',*,*,#7212,.F.);
#9977=ORIENTED_EDGE('',*,*,#7209,.T.);
#9978=ORIENTED_EDGE('',*,*,#7213,.F.);
#9979=ORIENTED_EDGE('',*,*,#7211,.F.);
#9980=ORIENTED_EDGE('',*,*,#6928,.F.);
#9981=ORIENTED_EDGE('',*,*,#7210,.T.);
#9982=ORIENTED_EDGE('',*,*,#7214,.F.);
#9983=ORIENTED_EDGE('',*,*,#7215,.T.);
#9984=ORIENTED_EDGE('',*,*,#6930,.F.);
#9985=ORIENTED_EDGE('',*,*,#7215,.F.);
#9986=ORIENTED_EDGE('',*,*,#7216,.F.);
#9987=ORIENTED_EDGE('',*,*,#7217,.F.);
#9988=ORIENTED_EDGE('',*,*,#6931,.F.);
#9989=ORIENTED_EDGE('',*,*,#7218,.F.);
#9990=ORIENTED_EDGE('',*,*,#6933,.F.);
#9991=ORIENTED_EDGE('',*,*,#7219,.T.);
#9992=ORIENTED_EDGE('',*,*,#7220,.F.);
#9993=ORIENTED_EDGE('',*,*,#7217,.T.);
#9994=ORIENTED_EDGE('',*,*,#7221,.F.);
#9995=ORIENTED_EDGE('',*,*,#7219,.F.);
#9996=ORIENTED_EDGE('',*,*,#6932,.F.);
#9997=ORIENTED_EDGE('',*,*,#7218,.T.);
#9998=ORIENTED_EDGE('',*,*,#7222,.F.);
#9999=ORIENTED_EDGE('',*,*,#7223,.T.);
#10000=ORIENTED_EDGE('',*,*,#6934,.F.);
#10001=ORIENTED_EDGE('',*,*,#7223,.F.);
#10002=ORIENTED_EDGE('',*,*,#7224,.F.);
#10003=ORIENTED_EDGE('',*,*,#7225,.F.);
#10004=ORIENTED_EDGE('',*,*,#6935,.F.);
#10005=ORIENTED_EDGE('',*,*,#7226,.F.);
#10006=ORIENTED_EDGE('',*,*,#6937,.F.);
#10007=ORIENTED_EDGE('',*,*,#7227,.T.);
#10008=ORIENTED_EDGE('',*,*,#7228,.F.);
#10009=ORIENTED_EDGE('',*,*,#7225,.T.);
#10010=ORIENTED_EDGE('',*,*,#7229,.F.);
#10011=ORIENTED_EDGE('',*,*,#7227,.F.);
#10012=ORIENTED_EDGE('',*,*,#6936,.F.);
#10013=ORIENTED_EDGE('',*,*,#7226,.T.);
#10014=ORIENTED_EDGE('',*,*,#7230,.F.);
#10015=ORIENTED_EDGE('',*,*,#7231,.T.);
#10016=ORIENTED_EDGE('',*,*,#6938,.F.);
#10017=ORIENTED_EDGE('',*,*,#7231,.F.);
#10018=ORIENTED_EDGE('',*,*,#7232,.F.);
#10019=ORIENTED_EDGE('',*,*,#7233,.F.);
#10020=ORIENTED_EDGE('',*,*,#6939,.F.);
#10021=ORIENTED_EDGE('',*,*,#7234,.F.);
#10022=ORIENTED_EDGE('',*,*,#6941,.F.);
#10023=ORIENTED_EDGE('',*,*,#7235,.T.);
#10024=ORIENTED_EDGE('',*,*,#7236,.F.);
#10025=ORIENTED_EDGE('',*,*,#7233,.T.);
#10026=ORIENTED_EDGE('',*,*,#7237,.F.);
#10027=ORIENTED_EDGE('',*,*,#7235,.F.);
#10028=ORIENTED_EDGE('',*,*,#6940,.F.);
#10029=ORIENTED_EDGE('',*,*,#7234,.T.);
#10030=ORIENTED_EDGE('',*,*,#7238,.F.);
#10031=ORIENTED_EDGE('',*,*,#7239,.T.);
#10032=ORIENTED_EDGE('',*,*,#6942,.F.);
#10033=ORIENTED_EDGE('',*,*,#7239,.F.);
#10034=ORIENTED_EDGE('',*,*,#7240,.F.);
#10035=ORIENTED_EDGE('',*,*,#7241,.F.);
#10036=ORIENTED_EDGE('',*,*,#6943,.F.);
#10037=ORIENTED_EDGE('',*,*,#7242,.F.);
#10038=ORIENTED_EDGE('',*,*,#6945,.F.);
#10039=ORIENTED_EDGE('',*,*,#7243,.T.);
#10040=ORIENTED_EDGE('',*,*,#7244,.F.);
#10041=ORIENTED_EDGE('',*,*,#7241,.T.);
#10042=ORIENTED_EDGE('',*,*,#7245,.F.);
#10043=ORIENTED_EDGE('',*,*,#7243,.F.);
#10044=ORIENTED_EDGE('',*,*,#6944,.F.);
#10045=ORIENTED_EDGE('',*,*,#7242,.T.);
#10046=ORIENTED_EDGE('',*,*,#7246,.F.);
#10047=ORIENTED_EDGE('',*,*,#7247,.T.);
#10048=ORIENTED_EDGE('',*,*,#6946,.F.);
#10049=ORIENTED_EDGE('',*,*,#7247,.F.);
#10050=ORIENTED_EDGE('',*,*,#7248,.F.);
#10051=ORIENTED_EDGE('',*,*,#7249,.F.);
#10052=ORIENTED_EDGE('',*,*,#6947,.F.);
#10053=ORIENTED_EDGE('',*,*,#7250,.F.);
#10054=ORIENTED_EDGE('',*,*,#6949,.F.);
#10055=ORIENTED_EDGE('',*,*,#7251,.T.);
#10056=ORIENTED_EDGE('',*,*,#7252,.F.);
#10057=ORIENTED_EDGE('',*,*,#7249,.T.);
#10058=ORIENTED_EDGE('',*,*,#7253,.F.);
#10059=ORIENTED_EDGE('',*,*,#7251,.F.);
#10060=ORIENTED_EDGE('',*,*,#6948,.F.);
#10061=ORIENTED_EDGE('',*,*,#7250,.T.);
#10062=ORIENTED_EDGE('',*,*,#7254,.F.);
#10063=ORIENTED_EDGE('',*,*,#7255,.T.);
#10064=ORIENTED_EDGE('',*,*,#6950,.F.);
#10065=ORIENTED_EDGE('',*,*,#7255,.F.);
#10066=ORIENTED_EDGE('',*,*,#7256,.F.);
#10067=ORIENTED_EDGE('',*,*,#7257,.F.);
#10068=ORIENTED_EDGE('',*,*,#6951,.F.);
#10069=ORIENTED_EDGE('',*,*,#7258,.F.);
#10070=ORIENTED_EDGE('',*,*,#6953,.F.);
#10071=ORIENTED_EDGE('',*,*,#7259,.T.);
#10072=ORIENTED_EDGE('',*,*,#7260,.F.);
#10073=ORIENTED_EDGE('',*,*,#7257,.T.);
#10074=ORIENTED_EDGE('',*,*,#7261,.F.);
#10075=ORIENTED_EDGE('',*,*,#7259,.F.);
#10076=ORIENTED_EDGE('',*,*,#6952,.F.);
#10077=ORIENTED_EDGE('',*,*,#7258,.T.);
#10078=ORIENTED_EDGE('',*,*,#7262,.F.);
#10079=ORIENTED_EDGE('',*,*,#7263,.T.);
#10080=ORIENTED_EDGE('',*,*,#6954,.F.);
#10081=ORIENTED_EDGE('',*,*,#7263,.F.);
#10082=ORIENTED_EDGE('',*,*,#7264,.F.);
#10083=ORIENTED_EDGE('',*,*,#7265,.F.);
#10084=ORIENTED_EDGE('',*,*,#6955,.F.);
#10085=ORIENTED_EDGE('',*,*,#7266,.F.);
#10086=ORIENTED_EDGE('',*,*,#6957,.F.);
#10087=ORIENTED_EDGE('',*,*,#7267,.T.);
#10088=ORIENTED_EDGE('',*,*,#7268,.F.);
#10089=ORIENTED_EDGE('',*,*,#7265,.T.);
#10090=ORIENTED_EDGE('',*,*,#7269,.F.);
#10091=ORIENTED_EDGE('',*,*,#7267,.F.);
#10092=ORIENTED_EDGE('',*,*,#6956,.F.);
#10093=ORIENTED_EDGE('',*,*,#7266,.T.);
#10094=ORIENTED_EDGE('',*,*,#7270,.F.);
#10095=ORIENTED_EDGE('',*,*,#7271,.T.);
#10096=ORIENTED_EDGE('',*,*,#6958,.F.);
#10097=ORIENTED_EDGE('',*,*,#7271,.F.);
#10098=ORIENTED_EDGE('',*,*,#7272,.F.);
#10099=ORIENTED_EDGE('',*,*,#7273,.F.);
#10100=ORIENTED_EDGE('',*,*,#6959,.F.);
#10101=ORIENTED_EDGE('',*,*,#7274,.F.);
#10102=ORIENTED_EDGE('',*,*,#6961,.F.);
#10103=ORIENTED_EDGE('',*,*,#7275,.T.);
#10104=ORIENTED_EDGE('',*,*,#7276,.F.);
#10105=ORIENTED_EDGE('',*,*,#7273,.T.);
#10106=ORIENTED_EDGE('',*,*,#7277,.F.);
#10107=ORIENTED_EDGE('',*,*,#7275,.F.);
#10108=ORIENTED_EDGE('',*,*,#6960,.F.);
#10109=ORIENTED_EDGE('',*,*,#7274,.T.);
#10110=ORIENTED_EDGE('',*,*,#7278,.F.);
#10111=ORIENTED_EDGE('',*,*,#7279,.T.);
#10112=ORIENTED_EDGE('',*,*,#6962,.F.);
#10113=ORIENTED_EDGE('',*,*,#7279,.F.);
#10114=ORIENTED_EDGE('',*,*,#7280,.F.);
#10115=ORIENTED_EDGE('',*,*,#7281,.F.);
#10116=ORIENTED_EDGE('',*,*,#6963,.F.);
#10117=ORIENTED_EDGE('',*,*,#7282,.F.);
#10118=ORIENTED_EDGE('',*,*,#6965,.F.);
#10119=ORIENTED_EDGE('',*,*,#7283,.T.);
#10120=ORIENTED_EDGE('',*,*,#7284,.F.);
#10121=ORIENTED_EDGE('',*,*,#7281,.T.);
#10122=ORIENTED_EDGE('',*,*,#7285,.F.);
#10123=ORIENTED_EDGE('',*,*,#7283,.F.);
#10124=ORIENTED_EDGE('',*,*,#6964,.F.);
#10125=ORIENTED_EDGE('',*,*,#7282,.T.);
#10126=ORIENTED_EDGE('',*,*,#7286,.F.);
#10127=ORIENTED_EDGE('',*,*,#7287,.T.);
#10128=ORIENTED_EDGE('',*,*,#6966,.F.);
#10129=ORIENTED_EDGE('',*,*,#7287,.F.);
#10130=ORIENTED_EDGE('',*,*,#7288,.F.);
#10131=ORIENTED_EDGE('',*,*,#7289,.F.);
#10132=ORIENTED_EDGE('',*,*,#6967,.F.);
#10133=ORIENTED_EDGE('',*,*,#7289,.T.);
#10134=ORIENTED_EDGE('',*,*,#7290,.F.);
#10135=ORIENTED_EDGE('',*,*,#7291,.F.);
#10136=ORIENTED_EDGE('',*,*,#6968,.F.);
#10137=ORIENTED_EDGE('',*,*,#7292,.F.);
#10138=ORIENTED_EDGE('',*,*,#6969,.F.);
#10139=ORIENTED_EDGE('',*,*,#7291,.T.);
#10140=ORIENTED_EDGE('',*,*,#7293,.F.);
#10141=ORIENTED_EDGE('',*,*,#7292,.T.);
#10142=ORIENTED_EDGE('',*,*,#7294,.F.);
#10143=ORIENTED_EDGE('',*,*,#7295,.T.);
#10144=ORIENTED_EDGE('',*,*,#6970,.F.);
#10145=ORIENTED_EDGE('',*,*,#7296,.F.);
#10146=ORIENTED_EDGE('',*,*,#6973,.F.);
#10147=ORIENTED_EDGE('',*,*,#7297,.T.);
#10148=ORIENTED_EDGE('',*,*,#7298,.F.);
#10149=ORIENTED_EDGE('',*,*,#7295,.F.);
#10150=ORIENTED_EDGE('',*,*,#7299,.F.);
#10151=ORIENTED_EDGE('',*,*,#7300,.F.);
#10152=ORIENTED_EDGE('',*,*,#6971,.F.);
#10153=ORIENTED_EDGE('',*,*,#7300,.T.);
#10154=ORIENTED_EDGE('',*,*,#7301,.F.);
#10155=ORIENTED_EDGE('',*,*,#7297,.F.);
#10156=ORIENTED_EDGE('',*,*,#6972,.F.);
#10157=ORIENTED_EDGE('',*,*,#6988,.T.);
#10158=ORIENTED_EDGE('',*,*,#6989,.T.);
#10159=ORIENTED_EDGE('',*,*,#6984,.T.);
#10160=ORIENTED_EDGE('',*,*,#7302,.T.);
#10161=ORIENTED_EDGE('',*,*,#7298,.T.);
#10162=ORIENTED_EDGE('',*,*,#7301,.T.);
#10163=ORIENTED_EDGE('',*,*,#7299,.T.);
#10164=ORIENTED_EDGE('',*,*,#7294,.T.);
#10165=ORIENTED_EDGE('',*,*,#7293,.T.);
#10166=ORIENTED_EDGE('',*,*,#7290,.T.);
#10167=ORIENTED_EDGE('',*,*,#7288,.T.);
#10168=ORIENTED_EDGE('',*,*,#7286,.T.);
#10169=ORIENTED_EDGE('',*,*,#7284,.T.);
#10170=ORIENTED_EDGE('',*,*,#7285,.T.);
#10171=ORIENTED_EDGE('',*,*,#7280,.T.);
#10172=ORIENTED_EDGE('',*,*,#7278,.T.);
#10173=ORIENTED_EDGE('',*,*,#7276,.T.);
#10174=ORIENTED_EDGE('',*,*,#7277,.T.);
#10175=ORIENTED_EDGE('',*,*,#7272,.T.);
#10176=ORIENTED_EDGE('',*,*,#7270,.T.);
#10177=ORIENTED_EDGE('',*,*,#7268,.T.);
#10178=ORIENTED_EDGE('',*,*,#7269,.T.);
#10179=ORIENTED_EDGE('',*,*,#7264,.T.);
#10180=ORIENTED_EDGE('',*,*,#7262,.T.);
#10181=ORIENTED_EDGE('',*,*,#7260,.T.);
#10182=ORIENTED_EDGE('',*,*,#7261,.T.);
#10183=ORIENTED_EDGE('',*,*,#7256,.T.);
#10184=ORIENTED_EDGE('',*,*,#7254,.T.);
#10185=ORIENTED_EDGE('',*,*,#7252,.T.);
#10186=ORIENTED_EDGE('',*,*,#7253,.T.);
#10187=ORIENTED_EDGE('',*,*,#7248,.T.);
#10188=ORIENTED_EDGE('',*,*,#7246,.T.);
#10189=ORIENTED_EDGE('',*,*,#7244,.T.);
#10190=ORIENTED_EDGE('',*,*,#7245,.T.);
#10191=ORIENTED_EDGE('',*,*,#7240,.T.);
#10192=ORIENTED_EDGE('',*,*,#7238,.T.);
#10193=ORIENTED_EDGE('',*,*,#7236,.T.);
#10194=ORIENTED_EDGE('',*,*,#7237,.T.);
#10195=ORIENTED_EDGE('',*,*,#7232,.T.);
#10196=ORIENTED_EDGE('',*,*,#7230,.T.);
#10197=ORIENTED_EDGE('',*,*,#7228,.T.);
#10198=ORIENTED_EDGE('',*,*,#7229,.T.);
#10199=ORIENTED_EDGE('',*,*,#7224,.T.);
#10200=ORIENTED_EDGE('',*,*,#7222,.T.);
#10201=ORIENTED_EDGE('',*,*,#7220,.T.);
#10202=ORIENTED_EDGE('',*,*,#7221,.T.);
#10203=ORIENTED_EDGE('',*,*,#7216,.T.);
#10204=ORIENTED_EDGE('',*,*,#7214,.T.);
#10205=ORIENTED_EDGE('',*,*,#7212,.T.);
#10206=ORIENTED_EDGE('',*,*,#7213,.T.);
#10207=ORIENTED_EDGE('',*,*,#7208,.T.);
#10208=ORIENTED_EDGE('',*,*,#7206,.T.);
#10209=ORIENTED_EDGE('',*,*,#7204,.T.);
#10210=ORIENTED_EDGE('',*,*,#7205,.T.);
#10211=ORIENTED_EDGE('',*,*,#7200,.T.);
#10212=ORIENTED_EDGE('',*,*,#7198,.T.);
#10213=ORIENTED_EDGE('',*,*,#7196,.T.);
#10214=ORIENTED_EDGE('',*,*,#7197,.T.);
#10215=ORIENTED_EDGE('',*,*,#7192,.T.);
#10216=ORIENTED_EDGE('',*,*,#7190,.T.);
#10217=ORIENTED_EDGE('',*,*,#7188,.T.);
#10218=ORIENTED_EDGE('',*,*,#7189,.T.);
#10219=ORIENTED_EDGE('',*,*,#7184,.T.);
#10220=ORIENTED_EDGE('',*,*,#7182,.T.);
#10221=ORIENTED_EDGE('',*,*,#7180,.T.);
#10222=ORIENTED_EDGE('',*,*,#7181,.T.);
#10223=ORIENTED_EDGE('',*,*,#7176,.T.);
#10224=ORIENTED_EDGE('',*,*,#7174,.T.);
#10225=ORIENTED_EDGE('',*,*,#7172,.T.);
#10226=ORIENTED_EDGE('',*,*,#7173,.T.);
#10227=ORIENTED_EDGE('',*,*,#7168,.T.);
#10228=ORIENTED_EDGE('',*,*,#7166,.T.);
#10229=ORIENTED_EDGE('',*,*,#7164,.T.);
#10230=ORIENTED_EDGE('',*,*,#7165,.T.);
#10231=ORIENTED_EDGE('',*,*,#7160,.T.);
#10232=ORIENTED_EDGE('',*,*,#7158,.T.);
#10233=ORIENTED_EDGE('',*,*,#7156,.T.);
#10234=ORIENTED_EDGE('',*,*,#7157,.T.);
#10235=ORIENTED_EDGE('',*,*,#7152,.T.);
#10236=ORIENTED_EDGE('',*,*,#7150,.T.);
#10237=ORIENTED_EDGE('',*,*,#7148,.T.);
#10238=ORIENTED_EDGE('',*,*,#7149,.T.);
#10239=ORIENTED_EDGE('',*,*,#7144,.T.);
#10240=ORIENTED_EDGE('',*,*,#7142,.T.);
#10241=ORIENTED_EDGE('',*,*,#7140,.T.);
#10242=ORIENTED_EDGE('',*,*,#7141,.T.);
#10243=ORIENTED_EDGE('',*,*,#7136,.T.);
#10244=ORIENTED_EDGE('',*,*,#7134,.T.);
#10245=ORIENTED_EDGE('',*,*,#7132,.T.);
#10246=ORIENTED_EDGE('',*,*,#7133,.T.);
#10247=ORIENTED_EDGE('',*,*,#7128,.T.);
#10248=ORIENTED_EDGE('',*,*,#7126,.T.);
#10249=ORIENTED_EDGE('',*,*,#7124,.T.);
#10250=ORIENTED_EDGE('',*,*,#7125,.T.);
#10251=ORIENTED_EDGE('',*,*,#7120,.T.);
#10252=ORIENTED_EDGE('',*,*,#7118,.T.);
#10253=ORIENTED_EDGE('',*,*,#7116,.T.);
#10254=ORIENTED_EDGE('',*,*,#7117,.T.);
#10255=ORIENTED_EDGE('',*,*,#7112,.T.);
#10256=ORIENTED_EDGE('',*,*,#7110,.T.);
#10257=ORIENTED_EDGE('',*,*,#7108,.T.);
#10258=ORIENTED_EDGE('',*,*,#7109,.T.);
#10259=ORIENTED_EDGE('',*,*,#7104,.T.);
#10260=ORIENTED_EDGE('',*,*,#7102,.T.);
#10261=ORIENTED_EDGE('',*,*,#7100,.T.);
#10262=ORIENTED_EDGE('',*,*,#7101,.T.);
#10263=ORIENTED_EDGE('',*,*,#7096,.T.);
#10264=ORIENTED_EDGE('',*,*,#7094,.T.);
#10265=ORIENTED_EDGE('',*,*,#7092,.T.);
#10266=ORIENTED_EDGE('',*,*,#7093,.T.);
#10267=ORIENTED_EDGE('',*,*,#7088,.T.);
#10268=ORIENTED_EDGE('',*,*,#7086,.T.);
#10269=ORIENTED_EDGE('',*,*,#7084,.T.);
#10270=ORIENTED_EDGE('',*,*,#7085,.T.);
#10271=ORIENTED_EDGE('',*,*,#7080,.T.);
#10272=ORIENTED_EDGE('',*,*,#7078,.T.);
#10273=ORIENTED_EDGE('',*,*,#7076,.T.);
#10274=ORIENTED_EDGE('',*,*,#7077,.T.);
#10275=ORIENTED_EDGE('',*,*,#7072,.T.);
#10276=ORIENTED_EDGE('',*,*,#7070,.T.);
#10277=ORIENTED_EDGE('',*,*,#7068,.T.);
#10278=ORIENTED_EDGE('',*,*,#7069,.T.);
#10279=ORIENTED_EDGE('',*,*,#7064,.T.);
#10280=ORIENTED_EDGE('',*,*,#7062,.T.);
#10281=ORIENTED_EDGE('',*,*,#7060,.T.);
#10282=ORIENTED_EDGE('',*,*,#7061,.T.);
#10283=ORIENTED_EDGE('',*,*,#7056,.T.);
#10284=ORIENTED_EDGE('',*,*,#7054,.T.);
#10285=ORIENTED_EDGE('',*,*,#7052,.T.);
#10286=ORIENTED_EDGE('',*,*,#7053,.T.);
#10287=ORIENTED_EDGE('',*,*,#7048,.T.);
#10288=ORIENTED_EDGE('',*,*,#7046,.T.);
#10289=ORIENTED_EDGE('',*,*,#7044,.T.);
#10290=ORIENTED_EDGE('',*,*,#7045,.T.);
#10291=ORIENTED_EDGE('',*,*,#7040,.T.);
#10292=ORIENTED_EDGE('',*,*,#7038,.T.);
#10293=ORIENTED_EDGE('',*,*,#7036,.T.);
#10294=ORIENTED_EDGE('',*,*,#7037,.T.);
#10295=ORIENTED_EDGE('',*,*,#7032,.T.);
#10296=ORIENTED_EDGE('',*,*,#7030,.T.);
#10297=ORIENTED_EDGE('',*,*,#7028,.T.);
#10298=ORIENTED_EDGE('',*,*,#7029,.T.);
#10299=ORIENTED_EDGE('',*,*,#7024,.T.);
#10300=ORIENTED_EDGE('',*,*,#7022,.T.);
#10301=ORIENTED_EDGE('',*,*,#7020,.T.);
#10302=ORIENTED_EDGE('',*,*,#7021,.T.);
#10303=ORIENTED_EDGE('',*,*,#7016,.T.);
#10304=ORIENTED_EDGE('',*,*,#7014,.T.);
#10305=ORIENTED_EDGE('',*,*,#7012,.T.);
#10306=ORIENTED_EDGE('',*,*,#7013,.T.);
#10307=ORIENTED_EDGE('',*,*,#7008,.T.);
#10308=ORIENTED_EDGE('',*,*,#7006,.T.);
#10309=ORIENTED_EDGE('',*,*,#7004,.T.);
#10310=ORIENTED_EDGE('',*,*,#7005,.T.);
#10311=ORIENTED_EDGE('',*,*,#7000,.T.);
#10312=ORIENTED_EDGE('',*,*,#6998,.T.);
#10313=ORIENTED_EDGE('',*,*,#6996,.T.);
#10314=ORIENTED_EDGE('',*,*,#6997,.T.);
#10315=ORIENTED_EDGE('',*,*,#6992,.T.);
#10316=ORIENTED_EDGE('',*,*,#6990,.T.);
#10317=ORIENTED_EDGE('',*,*,#6982,.T.);
#10318=ORIENTED_EDGE('',*,*,#6983,.T.);
#10319=ORIENTED_EDGE('',*,*,#6974,.F.);
#10320=ORIENTED_EDGE('',*,*,#7296,.T.);
#10321=ORIENTED_EDGE('',*,*,#7302,.F.);
#10580=CYLINDRICAL_SURFACE('',#12802,1.);
#10581=CYLINDRICAL_SURFACE('',#12804,2.);
#10582=CYLINDRICAL_SURFACE('',#12809,3.75);
#10583=CYLINDRICAL_SURFACE('',#12812,3.75);
#10584=CYLINDRICAL_SURFACE('',#12815,3.75);
#10585=CYLINDRICAL_SURFACE('',#12818,3.75);
#10586=CYLINDRICAL_SURFACE('',#12821,3.75);
#10587=CYLINDRICAL_SURFACE('',#12824,3.75);
#10588=CYLINDRICAL_SURFACE('',#12827,3.75);
#10589=CYLINDRICAL_SURFACE('',#12830,3.75);
#10590=CYLINDRICAL_SURFACE('',#12833,3.75);
#10591=CYLINDRICAL_SURFACE('',#12836,3.75);
#10592=CYLINDRICAL_SURFACE('',#12839,3.75);
#10593=CYLINDRICAL_SURFACE('',#12842,3.75);
#10594=CYLINDRICAL_SURFACE('',#12845,3.75);
#10595=CYLINDRICAL_SURFACE('',#12848,3.75);
#10596=CYLINDRICAL_SURFACE('',#12851,3.75);
#10597=CYLINDRICAL_SURFACE('',#12854,3.75);
#10598=CYLINDRICAL_SURFACE('',#12857,3.75);
#10599=CYLINDRICAL_SURFACE('',#12860,3.75);
#10600=CYLINDRICAL_SURFACE('',#12863,3.75);
#10601=CYLINDRICAL_SURFACE('',#12866,3.75);
#10602=CYLINDRICAL_SURFACE('',#12869,3.75);
#10603=CYLINDRICAL_SURFACE('',#12872,3.75);
#10604=CYLINDRICAL_SURFACE('',#12875,3.75);
#10605=CYLINDRICAL_SURFACE('',#12878,3.75);
#10606=CYLINDRICAL_SURFACE('',#12881,3.75);
#10607=CYLINDRICAL_SURFACE('',#12884,3.75);
#10608=CYLINDRICAL_SURFACE('',#12887,3.75);
#10609=CYLINDRICAL_SURFACE('',#12890,3.75);
#10610=CYLINDRICAL_SURFACE('',#12893,3.75);
#10611=CYLINDRICAL_SURFACE('',#12896,3.75);
#10612=CYLINDRICAL_SURFACE('',#12899,3.75);
#10613=CYLINDRICAL_SURFACE('',#12902,3.75);
#10614=CYLINDRICAL_SURFACE('',#12905,3.75);
#10615=CYLINDRICAL_SURFACE('',#12908,3.75);
#10616=CYLINDRICAL_SURFACE('',#12911,3.75);
#10617=CYLINDRICAL_SURFACE('',#12914,3.75);
#10618=CYLINDRICAL_SURFACE('',#12917,3.75);
#10619=CYLINDRICAL_SURFACE('',#12920,3.75);
#10620=CYLINDRICAL_SURFACE('',#12923,3.75);
#10621=CYLINDRICAL_SURFACE('',#12928,3.75);
#11081=ADVANCED_FACE('',(#1961),#1438,.F.);
#11082=ADVANCED_FACE('',(#1962),#1439,.F.);
#11083=ADVANCED_FACE('',(#1963),#1440,.F.);
#11084=ADVANCED_FACE('',(#1964,#1234),#1441,.F.);
#11085=ADVANCED_FACE('',(#1965),#10580,.F.);
#11086=ADVANCED_FACE('',(#1966),#10581,.T.);
#11087=ADVANCED_FACE('',(#1967,#1235),#1442,.T.);
#11088=ADVANCED_FACE('',(#1968),#51,.T.);
#11089=ADVANCED_FACE('',(#1969),#52,.T.);
#11090=ADVANCED_FACE('',(#1970),#1443,.T.);
#11091=ADVANCED_FACE('',(#1971),#10582,.T.);
#11092=ADVANCED_FACE('',(#1972),#53,.T.);
#11093=ADVANCED_FACE('',(#1973),#54,.T.);
#11094=ADVANCED_FACE('',(#1974),#1444,.T.);
#11095=ADVANCED_FACE('',(#1975),#10583,.T.);
#11096=ADVANCED_FACE('',(#1976),#55,.T.);
#11097=ADVANCED_FACE('',(#1977),#56,.T.);
#11098=ADVANCED_FACE('',(#1978),#1445,.T.);
#11099=ADVANCED_FACE('',(#1979),#10584,.T.);
#11100=ADVANCED_FACE('',(#1980),#57,.T.);
#11101=ADVANCED_FACE('',(#1981),#58,.T.);
#11102=ADVANCED_FACE('',(#1982),#1446,.T.);
#11103=ADVANCED_FACE('',(#1983),#10585,.T.);
#11104=ADVANCED_FACE('',(#1984),#59,.T.);
#11105=ADVANCED_FACE('',(#1985),#60,.T.);
#11106=ADVANCED_FACE('',(#1986),#1447,.T.);
#11107=ADVANCED_FACE('',(#1987),#10586,.T.);
#11108=ADVANCED_FACE('',(#1988),#61,.T.);
#11109=ADVANCED_FACE('',(#1989),#62,.T.);
#11110=ADVANCED_FACE('',(#1990),#1448,.T.);
#11111=ADVANCED_FACE('',(#1991),#10587,.T.);
#11112=ADVANCED_FACE('',(#1992),#63,.T.);
#11113=ADVANCED_FACE('',(#1993),#64,.T.);
#11114=ADVANCED_FACE('',(#1994),#1449,.T.);
#11115=ADVANCED_FACE('',(#1995),#10588,.T.);
#11116=ADVANCED_FACE('',(#1996),#65,.T.);
#11117=ADVANCED_FACE('',(#1997),#66,.T.);
#11118=ADVANCED_FACE('',(#1998),#1450,.T.);
#11119=ADVANCED_FACE('',(#1999),#10589,.T.);
#11120=ADVANCED_FACE('',(#2000),#67,.T.);
#11121=ADVANCED_FACE('',(#2001),#68,.T.);
#11122=ADVANCED_FACE('',(#2002),#1451,.T.);
#11123=ADVANCED_FACE('',(#2003),#10590,.T.);
#11124=ADVANCED_FACE('',(#2004),#69,.T.);
#11125=ADVANCED_FACE('',(#2005),#70,.T.);
#11126=ADVANCED_FACE('',(#2006),#1452,.T.);
#11127=ADVANCED_FACE('',(#2007),#10591,.T.);
#11128=ADVANCED_FACE('',(#2008),#71,.T.);
#11129=ADVANCED_FACE('',(#2009),#72,.T.);
#11130=ADVANCED_FACE('',(#2010),#1453,.T.);
#11131=ADVANCED_FACE('',(#2011),#10592,.T.);
#11132=ADVANCED_FACE('',(#2012),#73,.T.);
#11133=ADVANCED_FACE('',(#2013),#74,.T.);
#11134=ADVANCED_FACE('',(#2014),#1454,.T.);
#11135=ADVANCED_FACE('',(#2015),#10593,.T.);
#11136=ADVANCED_FACE('',(#2016),#75,.T.);
#11137=ADVANCED_FACE('',(#2017),#76,.T.);
#11138=ADVANCED_FACE('',(#2018),#1455,.T.);
#11139=ADVANCED_FACE('',(#2019),#10594,.T.);
#11140=ADVANCED_FACE('',(#2020),#77,.T.);
#11141=ADVANCED_FACE('',(#2021),#78,.T.);
#11142=ADVANCED_FACE('',(#2022),#1456,.T.);
#11143=ADVANCED_FACE('',(#2023),#10595,.T.);
#11144=ADVANCED_FACE('',(#2024),#79,.T.);
#11145=ADVANCED_FACE('',(#2025),#80,.T.);
#11146=ADVANCED_FACE('',(#2026),#1457,.T.);
#11147=ADVANCED_FACE('',(#2027),#10596,.T.);
#11148=ADVANCED_FACE('',(#2028),#81,.T.);
#11149=ADVANCED_FACE('',(#2029),#82,.T.);
#11150=ADVANCED_FACE('',(#2030),#1458,.T.);
#11151=ADVANCED_FACE('',(#2031),#10597,.T.);
#11152=ADVANCED_FACE('',(#2032),#83,.T.);
#11153=ADVANCED_FACE('',(#2033),#84,.T.);
#11154=ADVANCED_FACE('',(#2034),#1459,.T.);
#11155=ADVANCED_FACE('',(#2035),#10598,.T.);
#11156=ADVANCED_FACE('',(#2036),#85,.T.);
#11157=ADVANCED_FACE('',(#2037),#86,.T.);
#11158=ADVANCED_FACE('',(#2038),#1460,.T.);
#11159=ADVANCED_FACE('',(#2039),#10599,.T.);
#11160=ADVANCED_FACE('',(#2040),#87,.T.);
#11161=ADVANCED_FACE('',(#2041),#88,.T.);
#11162=ADVANCED_FACE('',(#2042),#1461,.T.);
#11163=ADVANCED_FACE('',(#2043),#10600,.T.);
#11164=ADVANCED_FACE('',(#2044),#89,.T.);
#11165=ADVANCED_FACE('',(#2045),#90,.T.);
#11166=ADVANCED_FACE('',(#2046),#1462,.T.);
#11167=ADVANCED_FACE('',(#2047),#10601,.T.);
#11168=ADVANCED_FACE('',(#2048),#91,.T.);
#11169=ADVANCED_FACE('',(#2049),#92,.T.);
#11170=ADVANCED_FACE('',(#2050),#1463,.T.);
#11171=ADVANCED_FACE('',(#2051),#10602,.T.);
#11172=ADVANCED_FACE('',(#2052),#93,.T.);
#11173=ADVANCED_FACE('',(#2053),#94,.T.);
#11174=ADVANCED_FACE('',(#2054),#1464,.T.);
#11175=ADVANCED_FACE('',(#2055),#10603,.T.);
#11176=ADVANCED_FACE('',(#2056),#95,.T.);
#11177=ADVANCED_FACE('',(#2057),#96,.T.);
#11178=ADVANCED_FACE('',(#2058),#1465,.T.);
#11179=ADVANCED_FACE('',(#2059),#10604,.T.);
#11180=ADVANCED_FACE('',(#2060),#97,.T.);
#11181=ADVANCED_FACE('',(#2061),#98,.T.);
#11182=ADVANCED_FACE('',(#2062),#1466,.T.);
#11183=ADVANCED_FACE('',(#2063),#10605,.T.);
#11184=ADVANCED_FACE('',(#2064),#99,.T.);
#11185=ADVANCED_FACE('',(#2065),#100,.T.);
#11186=ADVANCED_FACE('',(#2066),#1467,.T.);
#11187=ADVANCED_FACE('',(#2067),#10606,.T.);
#11188=ADVANCED_FACE('',(#2068),#101,.T.);
#11189=ADVANCED_FACE('',(#2069),#102,.T.);
#11190=ADVANCED_FACE('',(#2070),#1468,.T.);
#11191=ADVANCED_FACE('',(#2071),#10607,.T.);
#11192=ADVANCED_FACE('',(#2072),#103,.T.);
#11193=ADVANCED_FACE('',(#2073),#104,.T.);
#11194=ADVANCED_FACE('',(#2074),#1469,.T.);
#11195=ADVANCED_FACE('',(#2075),#10608,.T.);
#11196=ADVANCED_FACE('',(#2076),#105,.T.);
#11197=ADVANCED_FACE('',(#2077),#106,.T.);
#11198=ADVANCED_FACE('',(#2078),#1470,.T.);
#11199=ADVANCED_FACE('',(#2079),#10609,.T.);
#11200=ADVANCED_FACE('',(#2080),#107,.T.);
#11201=ADVANCED_FACE('',(#2081),#108,.T.);
#11202=ADVANCED_FACE('',(#2082),#1471,.T.);
#11203=ADVANCED_FACE('',(#2083),#10610,.T.);
#11204=ADVANCED_FACE('',(#2084),#109,.T.);
#11205=ADVANCED_FACE('',(#2085),#110,.T.);
#11206=ADVANCED_FACE('',(#2086),#1472,.T.);
#11207=ADVANCED_FACE('',(#2087),#10611,.T.);
#11208=ADVANCED_FACE('',(#2088),#111,.T.);
#11209=ADVANCED_FACE('',(#2089),#112,.T.);
#11210=ADVANCED_FACE('',(#2090),#1473,.T.);
#11211=ADVANCED_FACE('',(#2091),#10612,.T.);
#11212=ADVANCED_FACE('',(#2092),#113,.T.);
#11213=ADVANCED_FACE('',(#2093),#114,.T.);
#11214=ADVANCED_FACE('',(#2094),#1474,.T.);
#11215=ADVANCED_FACE('',(#2095),#10613,.T.);
#11216=ADVANCED_FACE('',(#2096),#115,.T.);
#11217=ADVANCED_FACE('',(#2097),#116,.T.);
#11218=ADVANCED_FACE('',(#2098),#1475,.T.);
#11219=ADVANCED_FACE('',(#2099),#10614,.T.);
#11220=ADVANCED_FACE('',(#2100),#117,.T.);
#11221=ADVANCED_FACE('',(#2101),#118,.T.);
#11222=ADVANCED_FACE('',(#2102),#1476,.T.);
#11223=ADVANCED_FACE('',(#2103),#10615,.T.);
#11224=ADVANCED_FACE('',(#2104),#119,.T.);
#11225=ADVANCED_FACE('',(#2105),#120,.T.);
#11226=ADVANCED_FACE('',(#2106),#1477,.T.);
#11227=ADVANCED_FACE('',(#2107),#10616,.T.);
#11228=ADVANCED_FACE('',(#2108),#121,.T.);
#11229=ADVANCED_FACE('',(#2109),#122,.T.);
#11230=ADVANCED_FACE('',(#2110),#1478,.T.);
#11231=ADVANCED_FACE('',(#2111),#10617,.T.);
#11232=ADVANCED_FACE('',(#2112),#123,.T.);
#11233=ADVANCED_FACE('',(#2113),#124,.T.);
#11234=ADVANCED_FACE('',(#2114),#1479,.T.);
#11235=ADVANCED_FACE('',(#2115),#10618,.T.);
#11236=ADVANCED_FACE('',(#2116),#125,.T.);
#11237=ADVANCED_FACE('',(#2117),#126,.T.);
#11238=ADVANCED_FACE('',(#2118),#1480,.T.);
#11239=ADVANCED_FACE('',(#2119),#10619,.T.);
#11240=ADVANCED_FACE('',(#2120),#127,.T.);
#11241=ADVANCED_FACE('',(#2121),#1481,.T.);
#11242=ADVANCED_FACE('',(#2122),#128,.T.);
#11243=ADVANCED_FACE('',(#2123),#10620,.T.);
#11244=ADVANCED_FACE('',(#2124),#129,.T.);
#11245=ADVANCED_FACE('',(#2125),#130,.T.);
#11246=ADVANCED_FACE('',(#2126),#1482,.T.);
#11247=ADVANCED_FACE('',(#2127,#1236),#1483,.T.);
#11248=ADVANCED_FACE('',(#2128),#10621,.T.);
#11329=CLOSED_SHELL('',(#11081,#11082,#11083,#11084,#11085,#11086,#11087,
#11088,#11089,#11090,#11091,#11092,#11093,#11094,#11095,#11096,#11097,#11098,
#11099,#11100,#11101,#11102,#11103,#11104,#11105,#11106,#11107,#11108,#11109,
#11110,#11111,#11112,#11113,#11114,#11115,#11116,#11117,#11118,#11119,#11120,
#11121,#11122,#11123,#11124,#11125,#11126,#11127,#11128,#11129,#11130,#11131,
#11132,#11133,#11134,#11135,#11136,#11137,#11138,#11139,#11140,#11141,#11142,
#11143,#11144,#11145,#11146,#11147,#11148,#11149,#11150,#11151,#11152,#11153,
#11154,#11155,#11156,#11157,#11158,#11159,#11160,#11161,#11162,#11163,#11164,
#11165,#11166,#11167,#11168,#11169,#11170,#11171,#11172,#11173,#11174,#11175,
#11176,#11177,#11178,#11179,#11180,#11181,#11182,#11183,#11184,#11185,#11186,
#11187,#11188,#11189,#11190,#11191,#11192,#11193,#11194,#11195,#11196,#11197,
#11198,#11199,#11200,#11201,#11202,#11203,#11204,#11205,#11206,#11207,#11208,
#11209,#11210,#11211,#11212,#11213,#11214,#11215,#11216,#11217,#11218,#11219,
#11220,#11221,#11222,#11223,#11224,#11225,#11226,#11227,#11228,#11229,#11230,
#11231,#11232,#11233,#11234,#11235,#11236,#11237,#11238,#11239,#11240,#11241,
#11242,#11243,#11244,#11245,#11246,#11247,#11248));
#12756=AXIS2_PLACEMENT_3D('',#30126,#15307,#15308);
#12757=AXIS2_PLACEMENT_3D('',#30127,#15309,#15310);
#12758=AXIS2_PLACEMENT_3D('',#30136,#15315,#15316);
#12759=AXIS2_PLACEMENT_3D('',#30142,#15320,#15321);
#12760=AXIS2_PLACEMENT_3D('',#30148,#15325,#15326);
#12761=AXIS2_PLACEMENT_3D('',#30151,#15327,#15328);
#12762=AXIS2_PLACEMENT_3D('',#30297,#15330,#15331);
#12763=AXIS2_PLACEMENT_3D('',#30443,#15333,#15334);
#12764=AXIS2_PLACEMENT_3D('',#30589,#15336,#15337);
#12765=AXIS2_PLACEMENT_3D('',#30735,#15339,#15340);
#12766=AXIS2_PLACEMENT_3D('',#30881,#15342,#15343);
#12767=AXIS2_PLACEMENT_3D('',#31027,#15345,#15346);
#12768=AXIS2_PLACEMENT_3D('',#31173,#15348,#15349);
#12769=AXIS2_PLACEMENT_3D('',#31319,#15351,#15352);
#12770=AXIS2_PLACEMENT_3D('',#31465,#15354,#15355);
#12771=AXIS2_PLACEMENT_3D('',#31611,#15357,#15358);
#12772=AXIS2_PLACEMENT_3D('',#31757,#15360,#15361);
#12773=AXIS2_PLACEMENT_3D('',#31903,#15363,#15364);
#12774=AXIS2_PLACEMENT_3D('',#32049,#15366,#15367);
#12775=AXIS2_PLACEMENT_3D('',#32195,#15369,#15370);
#12776=AXIS2_PLACEMENT_3D('',#32341,#15372,#15373);
#12777=AXIS2_PLACEMENT_3D('',#32487,#15375,#15376);
#12778=AXIS2_PLACEMENT_3D('',#32633,#15378,#15379);
#12779=AXIS2_PLACEMENT_3D('',#32779,#15381,#15382);
#12780=AXIS2_PLACEMENT_3D('',#32925,#15384,#15385);
#12781=AXIS2_PLACEMENT_3D('',#33071,#15387,#15388);
#12782=AXIS2_PLACEMENT_3D('',#33217,#15390,#15391);
#12783=AXIS2_PLACEMENT_3D('',#33363,#15393,#15394);
#12784=AXIS2_PLACEMENT_3D('',#33509,#15396,#15397);
#12785=AXIS2_PLACEMENT_3D('',#33655,#15399,#15400);
#12786=AXIS2_PLACEMENT_3D('',#33801,#15402,#15403);
#12787=AXIS2_PLACEMENT_3D('',#33947,#15405,#15406);
#12788=AXIS2_PLACEMENT_3D('',#34093,#15408,#15409);
#12789=AXIS2_PLACEMENT_3D('',#34239,#15411,#15412);
#12790=AXIS2_PLACEMENT_3D('',#34385,#15414,#15415);
#12791=AXIS2_PLACEMENT_3D('',#34531,#15417,#15418);
#12792=AXIS2_PLACEMENT_3D('',#34677,#15420,#15421);
#12793=AXIS2_PLACEMENT_3D('',#34823,#15423,#15424);
#12794=AXIS2_PLACEMENT_3D('',#34969,#15426,#15427);
#12795=AXIS2_PLACEMENT_3D('',#35115,#15429,#15430);
#12796=AXIS2_PLACEMENT_3D('',#35261,#15432,#15433);
#12797=AXIS2_PLACEMENT_3D('',#35407,#15435,#15436);
#12798=AXIS2_PLACEMENT_3D('',#35553,#15438,#15439);
#12799=AXIS2_PLACEMENT_3D('',#35699,#15441,#15442);
#12800=AXIS2_PLACEMENT_3D('',#35845,#15444,#15445);
#12801=AXIS2_PLACEMENT_3D('',#35989,#15447,#15448);
#12802=AXIS2_PLACEMENT_3D('',#35990,#15449,#15450);
#12803=AXIS2_PLACEMENT_3D('',#35991,#15451,#15452);
#12804=AXIS2_PLACEMENT_3D('',#35992,#15453,#15454);
#12805=AXIS2_PLACEMENT_3D('',#35994,#15455,#15456);
#12806=AXIS2_PLACEMENT_3D('',#35997,#15458,#15459);
#12807=AXIS2_PLACEMENT_3D('',#35998,#15460,#15461);
#12808=AXIS2_PLACEMENT_3D('',#36437,#15464,#15465);
#12809=AXIS2_PLACEMENT_3D('',#36439,#15467,#15468);
#12810=AXIS2_PLACEMENT_3D('',#36441,#15469,#15470);
#12811=AXIS2_PLACEMENT_3D('',#36879,#15473,#15474);
#12812=AXIS2_PLACEMENT_3D('',#36881,#15476,#15477);
#12813=AXIS2_PLACEMENT_3D('',#36883,#15478,#15479);
#12814=AXIS2_PLACEMENT_3D('',#37321,#15482,#15483);
#12815=AXIS2_PLACEMENT_3D('',#37323,#15485,#15486);
#12816=AXIS2_PLACEMENT_3D('',#37325,#15487,#15488);
#12817=AXIS2_PLACEMENT_3D('',#37763,#15491,#15492);
#12818=AXIS2_PLACEMENT_3D('',#37765,#15494,#15495);
#12819=AXIS2_PLACEMENT_3D('',#37767,#15496,#15497);
#12820=AXIS2_PLACEMENT_3D('',#38205,#15500,#15501);
#12821=AXIS2_PLACEMENT_3D('',#38207,#15503,#15504);
#12822=AXIS2_PLACEMENT_3D('',#38209,#15505,#15506);
#12823=AXIS2_PLACEMENT_3D('',#38647,#15509,#15510);
#12824=AXIS2_PLACEMENT_3D('',#38649,#15512,#15513);
#12825=AXIS2_PLACEMENT_3D('',#38651,#15514,#15515);
#12826=AXIS2_PLACEMENT_3D('',#39089,#15518,#15519);
#12827=AXIS2_PLACEMENT_3D('',#39091,#15521,#15522);
#12828=AXIS2_PLACEMENT_3D('',#39093,#15523,#15524);
#12829=AXIS2_PLACEMENT_3D('',#39531,#15527,#15528);
#12830=AXIS2_PLACEMENT_3D('',#39533,#15530,#15531);
#12831=AXIS2_PLACEMENT_3D('',#39535,#15532,#15533);
#12832=AXIS2_PLACEMENT_3D('',#39973,#15536,#15537);
#12833=AXIS2_PLACEMENT_3D('',#39975,#15539,#15540);
#12834=AXIS2_PLACEMENT_3D('',#39977,#15541,#15542);
#12835=AXIS2_PLACEMENT_3D('',#40415,#15545,#15546);
#12836=AXIS2_PLACEMENT_3D('',#40417,#15548,#15549);
#12837=AXIS2_PLACEMENT_3D('',#40419,#15550,#15551);
#12838=AXIS2_PLACEMENT_3D('',#40857,#15554,#15555);
#12839=AXIS2_PLACEMENT_3D('',#40859,#15557,#15558);
#12840=AXIS2_PLACEMENT_3D('',#40861,#15559,#15560);
#12841=AXIS2_PLACEMENT_3D('',#41299,#15563,#15564);
#12842=AXIS2_PLACEMENT_3D('',#41301,#15566,#15567);
#12843=AXIS2_PLACEMENT_3D('',#41303,#15568,#15569);
#12844=AXIS2_PLACEMENT_3D('',#41741,#15572,#15573);
#12845=AXIS2_PLACEMENT_3D('',#41743,#15575,#15576);
#12846=AXIS2_PLACEMENT_3D('',#41745,#15577,#15578);
#12847=AXIS2_PLACEMENT_3D('',#42183,#15581,#15582);
#12848=AXIS2_PLACEMENT_3D('',#42185,#15584,#15585);
#12849=AXIS2_PLACEMENT_3D('',#42187,#15586,#15587);
#12850=AXIS2_PLACEMENT_3D('',#42625,#15590,#15591);
#12851=AXIS2_PLACEMENT_3D('',#42627,#15593,#15594);
#12852=AXIS2_PLACEMENT_3D('',#42629,#15595,#15596);
#12853=AXIS2_PLACEMENT_3D('',#43067,#15599,#15600);
#12854=AXIS2_PLACEMENT_3D('',#43069,#15602,#15603);
#12855=AXIS2_PLACEMENT_3D('',#43071,#15604,#15605);
#12856=AXIS2_PLACEMENT_3D('',#43509,#15608,#15609);
#12857=AXIS2_PLACEMENT_3D('',#43511,#15611,#15612);
#12858=AXIS2_PLACEMENT_3D('',#43513,#15613,#15614);
#12859=AXIS2_PLACEMENT_3D('',#43951,#15617,#15618);
#12860=AXIS2_PLACEMENT_3D('',#43953,#15620,#15621);
#12861=AXIS2_PLACEMENT_3D('',#43955,#15622,#15623);
#12862=AXIS2_PLACEMENT_3D('',#44393,#15626,#15627);
#12863=AXIS2_PLACEMENT_3D('',#44395,#15629,#15630);
#12864=AXIS2_PLACEMENT_3D('',#44397,#15631,#15632);
#12865=AXIS2_PLACEMENT_3D('',#44835,#15635,#15636);
#12866=AXIS2_PLACEMENT_3D('',#44837,#15638,#15639);
#12867=AXIS2_PLACEMENT_3D('',#44839,#15640,#15641);
#12868=AXIS2_PLACEMENT_3D('',#45277,#15644,#15645);
#12869=AXIS2_PLACEMENT_3D('',#45279,#15647,#15648);
#12870=AXIS2_PLACEMENT_3D('',#45281,#15649,#15650);
#12871=AXIS2_PLACEMENT_3D('',#45719,#15653,#15654);
#12872=AXIS2_PLACEMENT_3D('',#45721,#15656,#15657);
#12873=AXIS2_PLACEMENT_3D('',#45723,#15658,#15659);
#12874=AXIS2_PLACEMENT_3D('',#46161,#15662,#15663);
#12875=AXIS2_PLACEMENT_3D('',#46163,#15665,#15666);
#12876=AXIS2_PLACEMENT_3D('',#46165,#15667,#15668);
#12877=AXIS2_PLACEMENT_3D('',#46603,#15671,#15672);
#12878=AXIS2_PLACEMENT_3D('',#46605,#15674,#15675);
#12879=AXIS2_PLACEMENT_3D('',#46607,#15676,#15677);
#12880=AXIS2_PLACEMENT_3D('',#47045,#15680,#15681);
#12881=AXIS2_PLACEMENT_3D('',#47047,#15683,#15684);
#12882=AXIS2_PLACEMENT_3D('',#47049,#15685,#15686);
#12883=AXIS2_PLACEMENT_3D('',#47487,#15689,#15690);
#12884=AXIS2_PLACEMENT_3D('',#47489,#15692,#15693);
#12885=AXIS2_PLACEMENT_3D('',#47491,#15694,#15695);
#12886=AXIS2_PLACEMENT_3D('',#47929,#15698,#15699);
#12887=AXIS2_PLACEMENT_3D('',#47931,#15701,#15702);
#12888=AXIS2_PLACEMENT_3D('',#47933,#15703,#15704);
#12889=AXIS2_PLACEMENT_3D('',#48371,#15707,#15708);
#12890=AXIS2_PLACEMENT_3D('',#48373,#15710,#15711);
#12891=AXIS2_PLACEMENT_3D('',#48375,#15712,#15713);
#12892=AXIS2_PLACEMENT_3D('',#48813,#15716,#15717);
#12893=AXIS2_PLACEMENT_3D('',#48815,#15719,#15720);
#12894=AXIS2_PLACEMENT_3D('',#48817,#15721,#15722);
#12895=AXIS2_PLACEMENT_3D('',#49255,#15725,#15726);
#12896=AXIS2_PLACEMENT_3D('',#49257,#15728,#15729);
#12897=AXIS2_PLACEMENT_3D('',#49259,#15730,#15731);
#12898=AXIS2_PLACEMENT_3D('',#49697,#15734,#15735);
#12899=AXIS2_PLACEMENT_3D('',#49699,#15737,#15738);
#12900=AXIS2_PLACEMENT_3D('',#49701,#15739,#15740);
#12901=AXIS2_PLACEMENT_3D('',#50139,#15743,#15744);
#12902=AXIS2_PLACEMENT_3D('',#50141,#15746,#15747);
#12903=AXIS2_PLACEMENT_3D('',#50143,#15748,#15749);
#12904=AXIS2_PLACEMENT_3D('',#50581,#15752,#15753);
#12905=AXIS2_PLACEMENT_3D('',#50583,#15755,#15756);
#12906=AXIS2_PLACEMENT_3D('',#50585,#15757,#15758);
#12907=AXIS2_PLACEMENT_3D('',#51023,#15761,#15762);
#12908=AXIS2_PLACEMENT_3D('',#51025,#15764,#15765);
#12909=AXIS2_PLACEMENT_3D('',#51027,#15766,#15767);
#12910=AXIS2_PLACEMENT_3D('',#51465,#15770,#15771);
#12911=AXIS2_PLACEMENT_3D('',#51467,#15773,#15774);
#12912=AXIS2_PLACEMENT_3D('',#51469,#15775,#15776);
#12913=AXIS2_PLACEMENT_3D('',#51907,#15779,#15780);
#12914=AXIS2_PLACEMENT_3D('',#51909,#15782,#15783);
#12915=AXIS2_PLACEMENT_3D('',#51911,#15784,#15785);
#12916=AXIS2_PLACEMENT_3D('',#52349,#15788,#15789);
#12917=AXIS2_PLACEMENT_3D('',#52351,#15791,#15792);
#12918=AXIS2_PLACEMENT_3D('',#52353,#15793,#15794);
#12919=AXIS2_PLACEMENT_3D('',#52791,#15797,#15798);
#12920=AXIS2_PLACEMENT_3D('',#52793,#15800,#15801);
#12921=AXIS2_PLACEMENT_3D('',#52795,#15802,#15803);
#12922=AXIS2_PLACEMENT_3D('',#53014,#15805,#15806);
#12923=AXIS2_PLACEMENT_3D('',#53235,#15809,#15810);
#12924=AXIS2_PLACEMENT_3D('',#53237,#15811,#15812);
#12925=AXIS2_PLACEMENT_3D('',#53675,#15815,#15816);
#12926=AXIS2_PLACEMENT_3D('',#53677,#15818,#15819);
#12927=AXIS2_PLACEMENT_3D('',#53678,#15820,#15821);
#12928=AXIS2_PLACEMENT_3D('',#53679,#15822,#15823);
#15307=DIRECTION('axis',(0.,0.,1.));
#15308=DIRECTION('refdir',(1.,0.,0.));
#15309=DIRECTION('center_axis',(1.,0.,0.));
#15310=DIRECTION('ref_axis',(0.,0.,-1.));
#15311=DIRECTION('',(0.,0.,1.));
#15312=DIRECTION('',(0.,1.,0.));
#15313=DIRECTION('',(0.,0.,-1.));
#15314=DIRECTION('',(0.,-1.,0.));
#15315=DIRECTION('center_axis',(0.,0.,-1.));
#15316=DIRECTION('ref_axis',(-1.,0.,0.));
#15317=DIRECTION('',(1.,0.,0.));
#15318=DIRECTION('',(0.,-1.,0.));
#15319=DIRECTION('',(-1.,0.,0.));
#15320=DIRECTION('center_axis',(-1.,0.,0.));
#15321=DIRECTION('ref_axis',(0.,0.,1.));
#15322=DIRECTION('',(0.,0.,-1.));
#15323=DIRECTION('',(0.,1.,0.));
#15324=DIRECTION('',(0.,0.,1.));
#15325=DIRECTION('center_axis',(0.,1.,0.));
#15326=DIRECTION('ref_axis',(1.,0.,0.));
#15327=DIRECTION('center_axis',(0.,-1.,0.));
#15328=DIRECTION('ref_axis',(1.,0.,0.));
#15329=DIRECTION('',(-0.309016994374948,0.,0.951056516295154));
#15330=DIRECTION('center_axis',(0.,-1.,0.));
#15331=DIRECTION('ref_axis',(1.,0.,0.));
#15332=DIRECTION('',(-0.453990499739547,0.,0.891006524188368));
#15333=DIRECTION('center_axis',(0.,-1.,0.));
#15334=DIRECTION('ref_axis',(1.,0.,0.));
#15335=DIRECTION('',(-0.587785252292473,0.,0.809016994374947));
#15336=DIRECTION('center_axis',(0.,-1.,0.));
#15337=DIRECTION('ref_axis',(1.,0.,0.));
#15338=DIRECTION('',(-0.707106781186548,0.,0.707106781186547));
#15339=DIRECTION('center_axis',(0.,-1.,0.));
#15340=DIRECTION('ref_axis',(1.,0.,0.));
#15341=DIRECTION('',(-0.809016994374948,0.,0.587785252292473));
#15342=DIRECTION('center_axis',(0.,-1.,0.));
#15343=DIRECTION('ref_axis',(1.,0.,0.));
#15344=DIRECTION('',(-0.891006524188368,0.,0.453990499739547));
#15345=DIRECTION('center_axis',(0.,-1.,0.));
#15346=DIRECTION('ref_axis',(1.,0.,0.));
#15347=DIRECTION('',(-0.951056516295154,0.,0.309016994374947));
#15348=DIRECTION('center_axis',(0.,-1.,0.));
#15349=DIRECTION('ref_axis',(1.,0.,0.));
#15350=DIRECTION('',(-0.987688340595138,0.,0.156434465040231));
#15351=DIRECTION('center_axis',(0.,-1.,0.));
#15352=DIRECTION('ref_axis',(1.,0.,0.));
#15353=DIRECTION('',(-1.,0.,-1.83697019872103E-16));
#15354=DIRECTION('center_axis',(0.,-1.,0.));
#15355=DIRECTION('ref_axis',(1.,0.,0.));
#15356=DIRECTION('',(-0.987688340595138,0.,-0.156434465040231));
#15357=DIRECTION('center_axis',(0.,-1.,0.));
#15358=DIRECTION('ref_axis',(1.,0.,0.));
#15359=DIRECTION('',(-0.951056516295154,0.,-0.309016994374948));
#15360=DIRECTION('center_axis',(0.,-1.,0.));
#15361=DIRECTION('ref_axis',(1.,0.,0.));
#15362=DIRECTION('',(-0.891006524188368,0.,-0.453990499739547));
#15363=DIRECTION('center_axis',(0.,-1.,0.));
#15364=DIRECTION('ref_axis',(1.,0.,0.));
#15365=DIRECTION('',(-0.809016994374947,0.,-0.587785252292473));
#15366=DIRECTION('center_axis',(0.,-1.,0.));
#15367=DIRECTION('ref_axis',(1.,0.,0.));
#15368=DIRECTION('',(-0.707106781186547,0.,-0.707106781186548));
#15369=DIRECTION('center_axis',(0.,-1.,0.));
#15370=DIRECTION('ref_axis',(1.,0.,0.));
#15371=DIRECTION('',(-0.587785252292473,0.,-0.809016994374948));
#15372=DIRECTION('center_axis',(0.,-1.,0.));
#15373=DIRECTION('ref_axis',(1.,0.,0.));
#15374=DIRECTION('',(-0.453990499739547,0.,-0.891006524188368));
#15375=DIRECTION('center_axis',(0.,-1.,0.));
#15376=DIRECTION('ref_axis',(1.,0.,0.));
#15377=DIRECTION('',(-0.309016994374947,0.,-0.951056516295154));
#15378=DIRECTION('center_axis',(0.,-1.,0.));
#15379=DIRECTION('ref_axis',(1.,0.,0.));
#15380=DIRECTION('',(-0.156434465040231,0.,-0.987688340595138));
#15381=DIRECTION('center_axis',(0.,-1.,0.));
#15382=DIRECTION('ref_axis',(1.,0.,0.));
#15383=DIRECTION('',(1.22464679914735E-16,0.,-1.));
#15384=DIRECTION('center_axis',(0.,-1.,0.));
#15385=DIRECTION('ref_axis',(1.,0.,0.));
#15386=DIRECTION('',(0.156434465040231,0.,-0.987688340595138));
#15387=DIRECTION('center_axis',(0.,-1.,0.));
#15388=DIRECTION('ref_axis',(1.,0.,0.));
#15389=DIRECTION('',(0.309016994374948,0.,-0.951056516295154));
#15390=DIRECTION('center_axis',(0.,-1.,0.));
#15391=DIRECTION('ref_axis',(1.,0.,0.));
#15392=DIRECTION('',(0.453990499739547,0.,-0.891006524188368));
#15393=DIRECTION('center_axis',(0.,-1.,0.));
#15394=DIRECTION('ref_axis',(1.,0.,0.));
#15395=DIRECTION('',(0.587785252292473,0.,-0.809016994374947));
#15396=DIRECTION('center_axis',(0.,-1.,0.));
#15397=DIRECTION('ref_axis',(1.,0.,0.));
#15398=DIRECTION('',(0.707106781186548,0.,-0.707106781186547));
#15399=DIRECTION('center_axis',(0.,-1.,0.));
#15400=DIRECTION('ref_axis',(1.,0.,0.));
#15401=DIRECTION('',(0.809016994374948,0.,-0.587785252292473));
#15402=DIRECTION('center_axis',(0.,-1.,0.));
#15403=DIRECTION('ref_axis',(1.,0.,0.));
#15404=DIRECTION('',(0.891006524188368,0.,-0.453990499739547));
#15405=DIRECTION('center_axis',(0.,-1.,0.));
#15406=DIRECTION('ref_axis',(1.,0.,0.));
#15407=DIRECTION('',(0.951056516295154,0.,-0.309016994374947));
#15408=DIRECTION('center_axis',(0.,-1.,0.));
#15409=DIRECTION('ref_axis',(1.,0.,0.));
#15410=DIRECTION('',(0.987688340595138,0.,-0.156434465040231));
#15411=DIRECTION('center_axis',(0.,-1.,0.));
#15412=DIRECTION('ref_axis',(1.,0.,0.));
#15413=DIRECTION('',(1.,0.,6.12323399573677E-17));
#15414=DIRECTION('center_axis',(0.,-1.,0.));
#15415=DIRECTION('ref_axis',(1.,0.,0.));
#15416=DIRECTION('',(0.987688340595138,0.,0.156434465040231));
#15417=DIRECTION('center_axis',(0.,-1.,0.));
#15418=DIRECTION('ref_axis',(1.,0.,0.));
#15419=DIRECTION('',(0.951056516295154,0.,0.309016994374948));
#15420=DIRECTION('center_axis',(0.,-1.,0.));
#15421=DIRECTION('ref_axis',(1.,0.,0.));
#15422=DIRECTION('',(0.891006524188368,0.,0.453990499739547));
#15423=DIRECTION('center_axis',(0.,-1.,0.));
#15424=DIRECTION('ref_axis',(1.,0.,0.));
#15425=DIRECTION('',(0.809016994374947,0.,0.587785252292473));
#15426=DIRECTION('center_axis',(0.,-1.,0.));
#15427=DIRECTION('ref_axis',(1.,0.,0.));
#15428=DIRECTION('',(0.707106781186547,0.,0.707106781186548));
#15429=DIRECTION('center_axis',(0.,-1.,0.));
#15430=DIRECTION('ref_axis',(1.,0.,0.));
#15431=DIRECTION('',(0.587785252292473,0.,0.809016994374947));
#15432=DIRECTION('center_axis',(0.,-1.,0.));
#15433=DIRECTION('ref_axis',(1.,0.,0.));
#15434=DIRECTION('',(0.453990499739547,0.,0.891006524188368));
#15435=DIRECTION('center_axis',(0.,-1.,0.));
#15436=DIRECTION('ref_axis',(1.,0.,0.));
#15437=DIRECTION('',(0.309016994374947,0.,0.951056516295154));
#15438=DIRECTION('center_axis',(0.,-1.,0.));
#15439=DIRECTION('ref_axis',(1.,0.,0.));
#15440=DIRECTION('',(0.156434465040231,0.,0.987688340595138));
#15441=DIRECTION('center_axis',(0.,-1.,0.));
#15442=DIRECTION('ref_axis',(1.,0.,0.));
#15443=DIRECTION('',(0.,0.,1.));
#15444=DIRECTION('center_axis',(0.,-1.,0.));
#15445=DIRECTION('ref_axis',(1.,0.,0.));
#15446=DIRECTION('',(-0.156434465040231,0.,0.987688340595138));
#15447=DIRECTION('center_axis',(0.,1.,0.));
#15448=DIRECTION('ref_axis',(1.,0.,0.));
#15449=DIRECTION('center_axis',(0.,1.,0.));
#15450=DIRECTION('ref_axis',(6.12323399573677E-17,0.,1.));
#15451=DIRECTION('center_axis',(0.,-1.,0.));
#15452=DIRECTION('ref_axis',(1.,0.,0.));
#15453=DIRECTION('center_axis',(0.,1.,0.));
#15454=DIRECTION('ref_axis',(1.,0.,0.));
#15455=DIRECTION('center_axis',(0.,1.,0.));
#15456=DIRECTION('ref_axis',(1.,0.,0.));
#15457=DIRECTION('',(0.,-1.,0.));
#15458=DIRECTION('center_axis',(0.,-1.,0.));
#15459=DIRECTION('ref_axis',(1.,0.,0.));
#15460=DIRECTION('center_axis',(0.,1.,0.));
#15461=DIRECTION('ref_axis',(1.,0.,0.));
#15462=DIRECTION('',(0.,1.,0.));
#15463=DIRECTION('',(0.,1.,0.));
#15464=DIRECTION('center_axis',(0.987688340595138,0.,0.156434465040231));
#15465=DIRECTION('ref_axis',(0.156434465040231,0.,-0.987688340595138));
#15466=DIRECTION('',(0.156434465040231,0.,-0.987688340595138));
#15467=DIRECTION('center_axis',(0.,1.,0.));
#15468=DIRECTION('ref_axis',(1.,0.,0.));
#15469=DIRECTION('center_axis',(0.,1.,0.));
#15470=DIRECTION('ref_axis',(1.,0.,0.));
#15471=DIRECTION('',(0.,1.,0.));
#15472=DIRECTION('',(0.,1.,0.));
#15473=DIRECTION('center_axis',(0.951056516295154,0.,0.309016994374948));
#15474=DIRECTION('ref_axis',(0.309016994374948,0.,-0.951056516295154));
#15475=DIRECTION('',(0.309016994374948,0.,-0.951056516295154));
#15476=DIRECTION('center_axis',(0.,1.,0.));
#15477=DIRECTION('ref_axis',(1.,0.,0.));
#15478=DIRECTION('center_axis',(0.,1.,0.));
#15479=DIRECTION('ref_axis',(1.,0.,0.));
#15480=DIRECTION('',(0.,1.,0.));
#15481=DIRECTION('',(0.,1.,0.));
#15482=DIRECTION('center_axis',(0.891006524188368,0.,0.453990499739547));
#15483=DIRECTION('ref_axis',(0.453990499739547,0.,-0.891006524188368));
#15484=DIRECTION('',(0.453990499739547,0.,-0.891006524188368));
#15485=DIRECTION('center_axis',(0.,1.,0.));
#15486=DIRECTION('ref_axis',(1.,0.,0.));
#15487=DIRECTION('center_axis',(0.,1.,0.));
#15488=DIRECTION('ref_axis',(1.,0.,0.));
#15489=DIRECTION('',(0.,1.,0.));
#15490=DIRECTION('',(0.,1.,0.));
#15491=DIRECTION('center_axis',(0.809016994374947,0.,0.587785252292473));
#15492=DIRECTION('ref_axis',(0.587785252292473,0.,-0.809016994374947));
#15493=DIRECTION('',(0.587785252292473,0.,-0.809016994374947));
#15494=DIRECTION('center_axis',(0.,1.,0.));
#15495=DIRECTION('ref_axis',(1.,0.,0.));
#15496=DIRECTION('center_axis',(0.,1.,0.));
#15497=DIRECTION('ref_axis',(1.,0.,0.));
#15498=DIRECTION('',(0.,1.,0.));
#15499=DIRECTION('',(0.,1.,0.));
#15500=DIRECTION('center_axis',(0.707106781186547,0.,0.707106781186548));
#15501=DIRECTION('ref_axis',(0.707106781186548,0.,-0.707106781186547));
#15502=DIRECTION('',(0.707106781186548,0.,-0.707106781186547));
#15503=DIRECTION('center_axis',(0.,1.,0.));
#15504=DIRECTION('ref_axis',(1.,0.,0.));
#15505=DIRECTION('center_axis',(0.,1.,0.));
#15506=DIRECTION('ref_axis',(1.,0.,0.));
#15507=DIRECTION('',(0.,1.,0.));
#15508=DIRECTION('',(0.,1.,0.));
#15509=DIRECTION('center_axis',(0.587785252292473,0.,0.809016994374948));
#15510=DIRECTION('ref_axis',(0.809016994374948,0.,-0.587785252292473));
#15511=DIRECTION('',(0.809016994374948,0.,-0.587785252292473));
#15512=DIRECTION('center_axis',(0.,1.,0.));
#15513=DIRECTION('ref_axis',(1.,0.,0.));
#15514=DIRECTION('center_axis',(0.,1.,0.));
#15515=DIRECTION('ref_axis',(1.,0.,0.));
#15516=DIRECTION('',(0.,1.,0.));
#15517=DIRECTION('',(0.,1.,0.));
#15518=DIRECTION('center_axis',(0.453990499739547,0.,0.891006524188368));
#15519=DIRECTION('ref_axis',(0.891006524188368,0.,-0.453990499739547));
#15520=DIRECTION('',(0.891006524188368,0.,-0.453990499739547));
#15521=DIRECTION('center_axis',(0.,1.,0.));
#15522=DIRECTION('ref_axis',(1.,0.,0.));
#15523=DIRECTION('center_axis',(0.,1.,0.));
#15524=DIRECTION('ref_axis',(1.,0.,0.));
#15525=DIRECTION('',(0.,1.,0.));
#15526=DIRECTION('',(0.,1.,0.));
#15527=DIRECTION('center_axis',(0.309016994374947,0.,0.951056516295154));
#15528=DIRECTION('ref_axis',(0.951056516295154,0.,-0.309016994374947));
#15529=DIRECTION('',(0.951056516295154,0.,-0.309016994374947));
#15530=DIRECTION('center_axis',(0.,1.,0.));
#15531=DIRECTION('ref_axis',(1.,0.,0.));
#15532=DIRECTION('center_axis',(0.,1.,0.));
#15533=DIRECTION('ref_axis',(1.,0.,0.));
#15534=DIRECTION('',(0.,1.,0.));
#15535=DIRECTION('',(0.,1.,0.));
#15536=DIRECTION('center_axis',(0.156434465040231,0.,0.987688340595138));
#15537=DIRECTION('ref_axis',(0.987688340595138,0.,-0.156434465040231));
#15538=DIRECTION('',(0.987688340595138,0.,-0.156434465040231));
#15539=DIRECTION('center_axis',(0.,1.,0.));
#15540=DIRECTION('ref_axis',(1.,0.,0.));
#15541=DIRECTION('center_axis',(0.,1.,0.));
#15542=DIRECTION('ref_axis',(1.,0.,0.));
#15543=DIRECTION('',(0.,1.,0.));
#15544=DIRECTION('',(0.,1.,0.));
#15545=DIRECTION('center_axis',(-1.83697019872103E-16,0.,1.));
#15546=DIRECTION('ref_axis',(1.,0.,1.83697019872103E-16));
#15547=DIRECTION('',(1.,0.,1.83697019872103E-16));
#15548=DIRECTION('center_axis',(0.,1.,0.));
#15549=DIRECTION('ref_axis',(1.,0.,0.));
#15550=DIRECTION('center_axis',(0.,1.,0.));
#15551=DIRECTION('ref_axis',(1.,0.,0.));
#15552=DIRECTION('',(0.,1.,0.));
#15553=DIRECTION('',(0.,1.,0.));
#15554=DIRECTION('center_axis',(-0.156434465040231,0.,0.987688340595138));
#15555=DIRECTION('ref_axis',(0.987688340595138,0.,0.156434465040231));
#15556=DIRECTION('',(0.987688340595138,0.,0.156434465040231));
#15557=DIRECTION('center_axis',(0.,1.,0.));
#15558=DIRECTION('ref_axis',(1.,0.,0.));
#15559=DIRECTION('center_axis',(0.,1.,0.));
#15560=DIRECTION('ref_axis',(1.,0.,0.));
#15561=DIRECTION('',(0.,1.,0.));
#15562=DIRECTION('',(0.,1.,0.));
#15563=DIRECTION('center_axis',(-0.309016994374948,0.,0.951056516295154));
#15564=DIRECTION('ref_axis',(0.951056516295154,0.,0.309016994374948));
#15565=DIRECTION('',(0.951056516295154,0.,0.309016994374948));
#15566=DIRECTION('center_axis',(0.,1.,0.));
#15567=DIRECTION('ref_axis',(1.,0.,0.));
#15568=DIRECTION('center_axis',(0.,1.,0.));
#15569=DIRECTION('ref_axis',(1.,0.,0.));
#15570=DIRECTION('',(0.,1.,0.));
#15571=DIRECTION('',(0.,1.,0.));
#15572=DIRECTION('center_axis',(-0.453990499739547,0.,0.891006524188368));
#15573=DIRECTION('ref_axis',(0.891006524188368,0.,0.453990499739547));
#15574=DIRECTION('',(0.891006524188368,0.,0.453990499739547));
#15575=DIRECTION('center_axis',(0.,1.,0.));
#15576=DIRECTION('ref_axis',(1.,0.,0.));
#15577=DIRECTION('center_axis',(0.,1.,0.));
#15578=DIRECTION('ref_axis',(1.,0.,0.));
#15579=DIRECTION('',(0.,1.,0.));
#15580=DIRECTION('',(0.,1.,0.));
#15581=DIRECTION('center_axis',(-0.587785252292473,0.,0.809016994374947));
#15582=DIRECTION('ref_axis',(0.809016994374947,0.,0.587785252292473));
#15583=DIRECTION('',(0.809016994374947,0.,0.587785252292473));
#15584=DIRECTION('center_axis',(0.,1.,0.));
#15585=DIRECTION('ref_axis',(1.,0.,0.));
#15586=DIRECTION('center_axis',(0.,1.,0.));
#15587=DIRECTION('ref_axis',(1.,0.,0.));
#15588=DIRECTION('',(0.,1.,0.));
#15589=DIRECTION('',(0.,1.,0.));
#15590=DIRECTION('center_axis',(-0.707106781186548,0.,0.707106781186547));
#15591=DIRECTION('ref_axis',(0.707106781186547,0.,0.707106781186548));
#15592=DIRECTION('',(0.707106781186547,0.,0.707106781186548));
#15593=DIRECTION('center_axis',(0.,1.,0.));
#15594=DIRECTION('ref_axis',(1.,0.,0.));
#15595=DIRECTION('center_axis',(0.,1.,0.));
#15596=DIRECTION('ref_axis',(1.,0.,0.));
#15597=DIRECTION('',(0.,1.,0.));
#15598=DIRECTION('',(0.,1.,0.));
#15599=DIRECTION('center_axis',(-0.809016994374948,0.,0.587785252292473));
#15600=DIRECTION('ref_axis',(0.587785252292473,0.,0.809016994374948));
#15601=DIRECTION('',(0.587785252292473,0.,0.809016994374948));
#15602=DIRECTION('center_axis',(0.,1.,0.));
#15603=DIRECTION('ref_axis',(1.,0.,0.));
#15604=DIRECTION('center_axis',(0.,1.,0.));
#15605=DIRECTION('ref_axis',(1.,0.,0.));
#15606=DIRECTION('',(0.,1.,0.));
#15607=DIRECTION('',(0.,1.,0.));
#15608=DIRECTION('center_axis',(-0.891006524188368,0.,0.453990499739547));
#15609=DIRECTION('ref_axis',(0.453990499739547,0.,0.891006524188368));
#15610=DIRECTION('',(0.453990499739547,0.,0.891006524188368));
#15611=DIRECTION('center_axis',(0.,1.,0.));
#15612=DIRECTION('ref_axis',(1.,0.,0.));
#15613=DIRECTION('center_axis',(0.,1.,0.));
#15614=DIRECTION('ref_axis',(1.,0.,0.));
#15615=DIRECTION('',(0.,1.,0.));
#15616=DIRECTION('',(0.,1.,0.));
#15617=DIRECTION('center_axis',(-0.951056516295154,0.,0.309016994374947));
#15618=DIRECTION('ref_axis',(0.309016994374947,0.,0.951056516295154));
#15619=DIRECTION('',(0.309016994374947,0.,0.951056516295154));
#15620=DIRECTION('center_axis',(0.,1.,0.));
#15621=DIRECTION('ref_axis',(1.,0.,0.));
#15622=DIRECTION('center_axis',(0.,1.,0.));
#15623=DIRECTION('ref_axis',(1.,0.,0.));
#15624=DIRECTION('',(0.,1.,0.));
#15625=DIRECTION('',(0.,1.,0.));
#15626=DIRECTION('center_axis',(-0.987688340595138,0.,0.156434465040231));
#15627=DIRECTION('ref_axis',(0.156434465040231,0.,0.987688340595138));
#15628=DIRECTION('',(0.156434465040231,0.,0.987688340595138));
#15629=DIRECTION('center_axis',(0.,1.,0.));
#15630=DIRECTION('ref_axis',(1.,0.,0.));
#15631=DIRECTION('center_axis',(0.,1.,0.));
#15632=DIRECTION('ref_axis',(1.,0.,0.));
#15633=DIRECTION('',(0.,1.,0.));
#15634=DIRECTION('',(0.,1.,0.));
#15635=DIRECTION('center_axis',(-1.,0.,-1.22464679914735E-16));
#15636=DIRECTION('ref_axis',(-1.22464679914735E-16,0.,1.));
#15637=DIRECTION('',(-1.22464679914735E-16,0.,1.));
#15638=DIRECTION('center_axis',(0.,1.,0.));
#15639=DIRECTION('ref_axis',(1.,0.,0.));
#15640=DIRECTION('center_axis',(0.,1.,0.));
#15641=DIRECTION('ref_axis',(1.,0.,0.));
#15642=DIRECTION('',(0.,1.,0.));
#15643=DIRECTION('',(0.,1.,0.));
#15644=DIRECTION('center_axis',(-0.987688340595138,0.,-0.156434465040231));
#15645=DIRECTION('ref_axis',(-0.156434465040231,0.,0.987688340595138));
#15646=DIRECTION('',(-0.156434465040231,0.,0.987688340595138));
#15647=DIRECTION('center_axis',(0.,1.,0.));
#15648=DIRECTION('ref_axis',(1.,0.,0.));
#15649=DIRECTION('center_axis',(0.,1.,0.));
#15650=DIRECTION('ref_axis',(1.,0.,0.));
#15651=DIRECTION('',(0.,1.,0.));
#15652=DIRECTION('',(0.,1.,0.));
#15653=DIRECTION('center_axis',(-0.951056516295154,0.,-0.309016994374948));
#15654=DIRECTION('ref_axis',(-0.309016994374948,0.,0.951056516295154));
#15655=DIRECTION('',(-0.309016994374948,0.,0.951056516295154));
#15656=DIRECTION('center_axis',(0.,1.,0.));
#15657=DIRECTION('ref_axis',(1.,0.,0.));
#15658=DIRECTION('center_axis',(0.,1.,0.));
#15659=DIRECTION('ref_axis',(1.,0.,0.));
#15660=DIRECTION('',(0.,1.,0.));
#15661=DIRECTION('',(0.,1.,0.));
#15662=DIRECTION('center_axis',(-0.891006524188368,0.,-0.453990499739547));
#15663=DIRECTION('ref_axis',(-0.453990499739547,0.,0.891006524188368));
#15664=DIRECTION('',(-0.453990499739547,0.,0.891006524188368));
#15665=DIRECTION('center_axis',(0.,1.,0.));
#15666=DIRECTION('ref_axis',(1.,0.,0.));
#15667=DIRECTION('center_axis',(0.,1.,0.));
#15668=DIRECTION('ref_axis',(1.,0.,0.));
#15669=DIRECTION('',(0.,1.,0.));
#15670=DIRECTION('',(0.,1.,0.));
#15671=DIRECTION('center_axis',(-0.809016994374947,0.,-0.587785252292473));
#15672=DIRECTION('ref_axis',(-0.587785252292473,0.,0.809016994374947));
#15673=DIRECTION('',(-0.587785252292473,0.,0.809016994374947));
#15674=DIRECTION('center_axis',(0.,1.,0.));
#15675=DIRECTION('ref_axis',(1.,0.,0.));
#15676=DIRECTION('center_axis',(0.,1.,0.));
#15677=DIRECTION('ref_axis',(1.,0.,0.));
#15678=DIRECTION('',(0.,1.,0.));
#15679=DIRECTION('',(0.,1.,0.));
#15680=DIRECTION('center_axis',(-0.707106781186547,0.,-0.707106781186548));
#15681=DIRECTION('ref_axis',(-0.707106781186548,0.,0.707106781186547));
#15682=DIRECTION('',(-0.707106781186548,0.,0.707106781186547));
#15683=DIRECTION('center_axis',(0.,1.,0.));
#15684=DIRECTION('ref_axis',(1.,0.,0.));
#15685=DIRECTION('center_axis',(0.,1.,0.));
#15686=DIRECTION('ref_axis',(1.,0.,0.));
#15687=DIRECTION('',(0.,1.,0.));
#15688=DIRECTION('',(0.,1.,0.));
#15689=DIRECTION('center_axis',(-0.587785252292473,0.,-0.809016994374948));
#15690=DIRECTION('ref_axis',(-0.809016994374948,0.,0.587785252292473));
#15691=DIRECTION('',(-0.809016994374948,0.,0.587785252292473));
#15692=DIRECTION('center_axis',(0.,1.,0.));
#15693=DIRECTION('ref_axis',(1.,0.,0.));
#15694=DIRECTION('center_axis',(0.,1.,0.));
#15695=DIRECTION('ref_axis',(1.,0.,0.));
#15696=DIRECTION('',(0.,1.,0.));
#15697=DIRECTION('',(0.,1.,0.));
#15698=DIRECTION('center_axis',(-0.453990499739547,0.,-0.891006524188368));
#15699=DIRECTION('ref_axis',(-0.891006524188368,0.,0.453990499739547));
#15700=DIRECTION('',(-0.891006524188368,0.,0.453990499739547));
#15701=DIRECTION('center_axis',(0.,1.,0.));
#15702=DIRECTION('ref_axis',(1.,0.,0.));
#15703=DIRECTION('center_axis',(0.,1.,0.));
#15704=DIRECTION('ref_axis',(1.,0.,0.));
#15705=DIRECTION('',(0.,1.,0.));
#15706=DIRECTION('',(0.,1.,0.));
#15707=DIRECTION('center_axis',(-0.309016994374947,0.,-0.951056516295154));
#15708=DIRECTION('ref_axis',(-0.951056516295154,0.,0.309016994374947));
#15709=DIRECTION('',(-0.951056516295154,0.,0.309016994374947));
#15710=DIRECTION('center_axis',(0.,1.,0.));
#15711=DIRECTION('ref_axis',(1.,0.,0.));
#15712=DIRECTION('center_axis',(0.,1.,0.));
#15713=DIRECTION('ref_axis',(1.,0.,0.));
#15714=DIRECTION('',(0.,1.,0.));
#15715=DIRECTION('',(0.,1.,0.));
#15716=DIRECTION('center_axis',(-0.156434465040231,0.,-0.987688340595138));
#15717=DIRECTION('ref_axis',(-0.987688340595138,0.,0.156434465040231));
#15718=DIRECTION('',(-0.987688340595138,0.,0.156434465040231));
#15719=DIRECTION('center_axis',(0.,1.,0.));
#15720=DIRECTION('ref_axis',(1.,0.,0.));
#15721=DIRECTION('center_axis',(0.,1.,0.));
#15722=DIRECTION('ref_axis',(1.,0.,0.));
#15723=DIRECTION('',(0.,1.,0.));
#15724=DIRECTION('',(0.,1.,0.));
#15725=DIRECTION('center_axis',(6.12323399573677E-17,0.,-1.));
#15726=DIRECTION('ref_axis',(-1.,0.,-6.12323399573677E-17));
#15727=DIRECTION('',(-1.,0.,-6.12323399573677E-17));
#15728=DIRECTION('center_axis',(0.,1.,0.));
#15729=DIRECTION('ref_axis',(1.,0.,0.));
#15730=DIRECTION('center_axis',(0.,1.,0.));
#15731=DIRECTION('ref_axis',(1.,0.,0.));
#15732=DIRECTION('',(0.,1.,0.));
#15733=DIRECTION('',(0.,1.,0.));
#15734=DIRECTION('center_axis',(0.156434465040231,0.,-0.987688340595138));
#15735=DIRECTION('ref_axis',(-0.987688340595138,0.,-0.156434465040231));
#15736=DIRECTION('',(-0.987688340595138,0.,-0.156434465040231));
#15737=DIRECTION('center_axis',(0.,1.,0.));
#15738=DIRECTION('ref_axis',(1.,0.,0.));
#15739=DIRECTION('center_axis',(0.,1.,0.));
#15740=DIRECTION('ref_axis',(1.,0.,0.));
#15741=DIRECTION('',(0.,1.,0.));
#15742=DIRECTION('',(0.,1.,0.));
#15743=DIRECTION('center_axis',(0.309016994374948,0.,-0.951056516295154));
#15744=DIRECTION('ref_axis',(-0.951056516295154,0.,-0.309016994374948));
#15745=DIRECTION('',(-0.951056516295154,0.,-0.309016994374948));
#15746=DIRECTION('center_axis',(0.,1.,0.));
#15747=DIRECTION('ref_axis',(1.,0.,0.));
#15748=DIRECTION('center_axis',(0.,1.,0.));
#15749=DIRECTION('ref_axis',(1.,0.,0.));
#15750=DIRECTION('',(0.,1.,0.));
#15751=DIRECTION('',(0.,1.,0.));
#15752=DIRECTION('center_axis',(0.453990499739547,0.,-0.891006524188368));
#15753=DIRECTION('ref_axis',(-0.891006524188368,0.,-0.453990499739547));
#15754=DIRECTION('',(-0.891006524188368,0.,-0.453990499739547));
#15755=DIRECTION('center_axis',(0.,1.,0.));
#15756=DIRECTION('ref_axis',(1.,0.,0.));
#15757=DIRECTION('center_axis',(0.,1.,0.));
#15758=DIRECTION('ref_axis',(1.,0.,0.));
#15759=DIRECTION('',(0.,1.,0.));
#15760=DIRECTION('',(0.,1.,0.));
#15761=DIRECTION('center_axis',(0.587785252292473,0.,-0.809016994374947));
#15762=DIRECTION('ref_axis',(-0.809016994374947,0.,-0.587785252292473));
#15763=DIRECTION('',(-0.809016994374947,0.,-0.587785252292473));
#15764=DIRECTION('center_axis',(0.,1.,0.));
#15765=DIRECTION('ref_axis',(1.,0.,0.));
#15766=DIRECTION('center_axis',(0.,1.,0.));
#15767=DIRECTION('ref_axis',(1.,0.,0.));
#15768=DIRECTION('',(0.,1.,0.));
#15769=DIRECTION('',(0.,1.,0.));
#15770=DIRECTION('center_axis',(0.707106781186548,0.,-0.707106781186547));
#15771=DIRECTION('ref_axis',(-0.707106781186547,0.,-0.707106781186548));
#15772=DIRECTION('',(-0.707106781186547,0.,-0.707106781186548));
#15773=DIRECTION('center_axis',(0.,1.,0.));
#15774=DIRECTION('ref_axis',(1.,0.,0.));
#15775=DIRECTION('center_axis',(0.,1.,0.));
#15776=DIRECTION('ref_axis',(1.,0.,0.));
#15777=DIRECTION('',(0.,1.,0.));
#15778=DIRECTION('',(0.,1.,0.));
#15779=DIRECTION('center_axis',(0.809016994374947,0.,-0.587785252292473));
#15780=DIRECTION('ref_axis',(-0.587785252292473,0.,-0.809016994374947));
#15781=DIRECTION('',(-0.587785252292473,0.,-0.809016994374947));
#15782=DIRECTION('center_axis',(0.,1.,0.));
#15783=DIRECTION('ref_axis',(1.,0.,0.));
#15784=DIRECTION('center_axis',(0.,1.,0.));
#15785=DIRECTION('ref_axis',(1.,0.,0.));
#15786=DIRECTION('',(0.,1.,0.));
#15787=DIRECTION('',(0.,1.,0.));
#15788=DIRECTION('center_axis',(0.891006524188368,0.,-0.453990499739547));
#15789=DIRECTION('ref_axis',(-0.453990499739547,0.,-0.891006524188368));
#15790=DIRECTION('',(-0.453990499739547,0.,-0.891006524188368));
#15791=DIRECTION('center_axis',(0.,1.,0.));
#15792=DIRECTION('ref_axis',(1.,0.,0.));
#15793=DIRECTION('center_axis',(0.,1.,0.));
#15794=DIRECTION('ref_axis',(1.,0.,0.));
#15795=DIRECTION('',(0.,1.,0.));
#15796=DIRECTION('',(0.,1.,0.));
#15797=DIRECTION('center_axis',(0.951056516295154,0.,-0.309016994374947));
#15798=DIRECTION('ref_axis',(-0.309016994374947,0.,-0.951056516295154));
#15799=DIRECTION('',(-0.309016994374947,0.,-0.951056516295154));
#15800=DIRECTION('center_axis',(0.,1.,0.));
#15801=DIRECTION('ref_axis',(1.,0.,0.));
#15802=DIRECTION('center_axis',(0.,1.,0.));
#15803=DIRECTION('ref_axis',(1.,0.,0.));
#15804=DIRECTION('',(0.,1.,0.));
#15805=DIRECTION('center_axis',(0.987688340595138,0.,-0.156434465040231));
#15806=DIRECTION('ref_axis',(-0.156434465040231,0.,-0.987688340595138));
#15807=DIRECTION('',(-0.156434465040231,0.,-0.987688340595138));
#15808=DIRECTION('',(0.,1.,0.));
#15809=DIRECTION('center_axis',(0.,1.,0.));
#15810=DIRECTION('ref_axis',(1.,0.,0.));
#15811=DIRECTION('center_axis',(0.,1.,0.));
#15812=DIRECTION('ref_axis',(1.,0.,0.));
#15813=DIRECTION('',(0.,1.,0.));
#15814=DIRECTION('',(0.,1.,0.));
#15815=DIRECTION('center_axis',(1.,0.,0.));
#15816=DIRECTION('ref_axis',(0.,0.,-1.));
#15817=DIRECTION('',(0.,0.,-1.));
#15818=DIRECTION('center_axis',(0.,1.,0.));
#15819=DIRECTION('ref_axis',(1.,0.,0.));
#15820=DIRECTION('center_axis',(0.,1.,0.));
#15821=DIRECTION('ref_axis',(1.,0.,0.));
#15822=DIRECTION('center_axis',(0.,1.,0.));
#15823=DIRECTION('ref_axis',(1.,0.,0.));
#30126=CARTESIAN_POINT('',(0.,0.,0.));
#30127=CARTESIAN_POINT('Origin',(0.3,0.,0.));
#30128=CARTESIAN_POINT('',(0.3,2.2,-1.28));
#30129=CARTESIAN_POINT('',(0.3,2.2,-0.953939201416946));
#30130=CARTESIAN_POINT('',(0.3,2.2,0.));
#30131=CARTESIAN_POINT('',(0.3,-1.,-1.28));
#30132=CARTESIAN_POINT('',(0.3,0.,-1.28));
#30133=CARTESIAN_POINT('',(0.3,-1.,-0.953939201416946));
#30134=CARTESIAN_POINT('',(0.3,-1.,0.));
#30135=CARTESIAN_POINT('',(0.3,0.,-0.953939201416946));
#30136=CARTESIAN_POINT('Origin',(0.3,0.,-1.28));
#30137=CARTESIAN_POINT('',(-0.3,2.2,-1.28));
#30138=CARTESIAN_POINT('',(0.15,2.2,-1.28));
#30139=CARTESIAN_POINT('',(-0.3,-1.,-1.28));
#30140=CARTESIAN_POINT('',(-0.3,0.,-1.28));
#30141=CARTESIAN_POINT('',(0.15,-1.,-1.28));
#30142=CARTESIAN_POINT('Origin',(-0.3,0.,-1.28));
#30143=CARTESIAN_POINT('',(-0.3,2.2,-0.953939201416946));
#30144=CARTESIAN_POINT('',(-0.3,2.2,-0.64));
#30145=CARTESIAN_POINT('',(-0.3,-1.,-0.953939201416946));
#30146=CARTESIAN_POINT('',(-0.3,0.,-0.953939201416946));
#30147=CARTESIAN_POINT('',(-0.3,-1.,-0.64));
#30148=CARTESIAN_POINT('Origin',(0.,-1.,0.));
#30149=CARTESIAN_POINT('',(3.66661143271685,-1.,0.786422660831985));
#30150=CARTESIAN_POINT('',(3.62400312501245,-1.,0.963899035117249));
#30151=CARTESIAN_POINT('Origin',(0.,-1.,0.));
#30152=CARTESIAN_POINT('',(4.01728681790024,-1.,1.22531898815164));
#30153=CARTESIAN_POINT('Ctrl Pts',(3.62400312501245,-1.,0.963899035117249));
#30154=CARTESIAN_POINT('Ctrl Pts',(3.6240482887845,-1.,0.963880158555582));
#30155=CARTESIAN_POINT('Ctrl Pts',(3.62424461507588,-1.,0.963861297423241));
#30156=CARTESIAN_POINT('Ctrl Pts',(3.62489305727662,-1.,0.963957782642844));
#30157=CARTESIAN_POINT('Ctrl Pts',(3.62652618145335,-1.,0.964373850166458));
#30158=CARTESIAN_POINT('Ctrl Pts',(3.62988252139846,-1.,0.965395153165294));
#30159=CARTESIAN_POINT('Ctrl Pts',(3.63492122081143,-1.,0.967052554541386));
#30160=CARTESIAN_POINT('Ctrl Pts',(3.64113946505766,-1.,0.969195124675866));
#30161=CARTESIAN_POINT('Ctrl Pts',(3.64819756447455,-1.,0.971722122061341));
#30162=CARTESIAN_POINT('Ctrl Pts',(3.65571576735126,-1.,0.974519971354849));
#30163=CARTESIAN_POINT('Ctrl Pts',(3.66333049637475,-1.,0.977478312751618));
#30164=CARTESIAN_POINT('Ctrl Pts',(3.67074983340361,-1.,0.980505922458267));
#30165=CARTESIAN_POINT('Ctrl Pts',(3.67782408841715,-1.,0.98355079147042));
#30166=CARTESIAN_POINT('Ctrl Pts',(3.68455317926068,-1.,0.986602639863838));
#30167=CARTESIAN_POINT('Ctrl Pts',(3.69102682138846,-1.,0.989676715398559));
#30168=CARTESIAN_POINT('Ctrl Pts',(3.69738123415662,-1.,0.992802218332011));
#30169=CARTESIAN_POINT('Ctrl Pts',(3.70375282282138,-1.,0.996009819772518));
#30170=CARTESIAN_POINT('Ctrl Pts',(3.71022439713938,-1.,0.999317260756531));
#30171=CARTESIAN_POINT('Ctrl Pts',(3.71680667125118,-1.,1.00272423396822));
#30172=CARTESIAN_POINT('Ctrl Pts',(3.72346803750595,-1.,1.0062200073571));
#30173=CARTESIAN_POINT('Ctrl Pts',(3.73015276704426,-1.,1.00978798539496));
#30174=CARTESIAN_POINT('Ctrl Pts',(3.73680245055734,-1.,1.01341114319903));
#30175=CARTESIAN_POINT('Ctrl Pts',(3.74337942504959,-1.,1.01707794311079));
#30176=CARTESIAN_POINT('Ctrl Pts',(3.74987777155834,-1.,1.02078510487428));
#30177=CARTESIAN_POINT('Ctrl Pts',(3.75631037456194,-1.,1.0245342944466));
#30178=CARTESIAN_POINT('Ctrl Pts',(3.76270122291232,-1.,1.02833014458181));
#30179=CARTESIAN_POINT('Ctrl Pts',(3.76907609832522,-1.,1.0321778660492));
#30180=CARTESIAN_POINT('Ctrl Pts',(3.77545283140445,-1.,1.03608074678013));
#30181=CARTESIAN_POINT('Ctrl Pts',(3.78183535008192,-1.,1.04003862055804));
#30182=CARTESIAN_POINT('Ctrl Pts',(3.78821910787195,-1.,1.04404924374426));
#30183=CARTESIAN_POINT('Ctrl Pts',(3.79459440308793,-1.,1.04810913267641));
#30184=CARTESIAN_POINT('Ctrl Pts',(3.80095039790678,-1.,1.05221457990015));
#30185=CARTESIAN_POINT('Ctrl Pts',(3.80727913637784,-1.,1.05636266918643));
#30186=CARTESIAN_POINT('Ctrl Pts',(3.81357866117485,-1.,1.06055206187298));
#30187=CARTESIAN_POINT('Ctrl Pts',(3.81985083953012,-1.,1.06478244038931));
#30188=CARTESIAN_POINT('Ctrl Pts',(3.82609989967278,-1.,1.0690541318036));
#30189=CARTESIAN_POINT('Ctrl Pts',(3.83233071195145,-1.,1.0733676663346));
#30190=CARTESIAN_POINT('Ctrl Pts',(3.83854714117486,-1.,1.07772335353856));
#30191=CARTESIAN_POINT('Ctrl Pts',(3.84475048030615,-1.,1.08212087917986));
#30192=CARTESIAN_POINT('Ctrl Pts',(3.8509402522269,-1.,1.08655950846377));
#30193=CARTESIAN_POINT('Ctrl Pts',(3.85711487933911,-1.,1.09103825516288));
#30194=CARTESIAN_POINT('Ctrl Pts',(3.86327241021242,-1.,1.09555606505012));
#30195=CARTESIAN_POINT('Ctrl Pts',(3.86941120134872,-1.,1.10011198761203));
#30196=CARTESIAN_POINT('Ctrl Pts',(3.87553067187566,-1.,1.10470536603303));
#30197=CARTESIAN_POINT('Ctrl Pts',(3.88163105531791,-1.,1.10933577224029));
#30198=CARTESIAN_POINT('Ctrl Pts',(3.88771308285229,-1.,1.11400292434447));
#30199=CARTESIAN_POINT('Ctrl Pts',(3.89377768340362,-1.,1.11870660794609));
#30200=CARTESIAN_POINT('Ctrl Pts',(3.89982569749978,-1.,1.12344660099029));
#30201=CARTESIAN_POINT('Ctrl Pts',(3.90585753318622,-1.,1.12822258281518));
#30202=CARTESIAN_POINT('Ctrl Pts',(3.91187321145495,-1.,1.13303414693849));
#30203=CARTESIAN_POINT('Ctrl Pts',(3.91787251936688,-1.,1.13788084225511));
#30204=CARTESIAN_POINT('Ctrl Pts',(3.92385513133937,-1.,1.14276220561575));
#30205=CARTESIAN_POINT('Ctrl Pts',(3.92982073294334,-1.,1.14767779451147));
#30206=CARTESIAN_POINT('Ctrl Pts',(3.9357691705651,-1.,1.15262722716391));
#30207=CARTESIAN_POINT('Ctrl Pts',(3.94170046685542,-1.,1.15761018341061));
#30208=CARTESIAN_POINT('Ctrl Pts',(3.9476147478092,-1.,1.16262637999261));
#30209=CARTESIAN_POINT('Ctrl Pts',(3.95351219510062,-1.,1.16767555244495));
#30210=CARTESIAN_POINT('Ctrl Pts',(3.95939299213164,-1.,1.17275743590327));
#30211=CARTESIAN_POINT('Ctrl Pts',(3.96525726357682,-1.,1.17787174135446));
#30212=CARTESIAN_POINT('Ctrl Pts',(3.9711050516465,-1.,1.18301815039596));
#30213=CARTESIAN_POINT('Ctrl Pts',(3.97693634766926,-1.,1.18819633715285));
#30214=CARTESIAN_POINT('Ctrl Pts',(3.98275111052015,-1.,1.19340598349307));
#30215=CARTESIAN_POINT('Ctrl Pts',(3.98854928957287,-1.,1.19864679609596));
#30216=CARTESIAN_POINT('Ctrl Pts',(3.99433084800649,-1.,1.2039185237544));
#30217=CARTESIAN_POINT('Ctrl Pts',(4.00009577952534,-1.,1.20922097030107));
#30218=CARTESIAN_POINT('Ctrl Pts',(4.00584409524937,-1.,1.21455398918813));
#30219=CARTESIAN_POINT('Ctrl Pts',(4.01042947142681,-1.,1.21884478244983));
#30220=CARTESIAN_POINT('Ctrl Pts',(4.01386104434674,-1.,1.22207656456199));
#30221=CARTESIAN_POINT('Ctrl Pts',(4.0161454457032,-1.,1.22423716681447));
#30222=CARTESIAN_POINT('Ctrl Pts',(4.01728681790024,-1.,1.22531898815164));
#30223=CARTESIAN_POINT('',(3.97027773754922,-1.,1.36999806084573));
#30224=CARTESIAN_POINT('',(4.01728681790024,-1.,1.22531898815164));
#30225=CARTESIAN_POINT('',(3.4984457533445,-1.,1.35032489087101));
#30226=CARTESIAN_POINT('Ctrl Pts',(3.97027773754922,-1.,1.36999806084573));
#30227=CARTESIAN_POINT('Ctrl Pts',(3.9687184694131,-1.,1.37020239094614));
#30228=CARTESIAN_POINT('Ctrl Pts',(3.96560037974645,-1.,1.37060761745635));
#30229=CARTESIAN_POINT('Ctrl Pts',(3.96092458506535,-1.,1.3712051561502));
#30230=CARTESIAN_POINT('Ctrl Pts',(3.95469287280914,-1.,1.37198126432386));
#30231=CARTESIAN_POINT('Ctrl Pts',(3.94690771785133,-1.,1.37291699202807));
#30232=CARTESIAN_POINT('Ctrl Pts',(3.93912709040818,-1.,1.37381821967165));
#30233=CARTESIAN_POINT('Ctrl Pts',(3.93135106761844,-1.,1.37468482215751));
#30234=CARTESIAN_POINT('Ctrl Pts',(3.92357976987672,-1.,1.37551664448242));
#30235=CARTESIAN_POINT('Ctrl Pts',(3.91581337462644,-1.,1.37631350505797));
#30236=CARTESIAN_POINT('Ctrl Pts',(3.90805209523486,-1.,1.3770751963402));
#30237=CARTESIAN_POINT('Ctrl Pts',(3.90029615196727,-1.,1.37780148512792));
#30238=CARTESIAN_POINT('Ctrl Pts',(3.89254574338496,-1.,1.3784921128802));
#30239=CARTESIAN_POINT('Ctrl Pts',(3.88480102249277,-1.,1.37914679719383));
#30240=CARTESIAN_POINT('Ctrl Pts',(3.87706205830532,-1.,1.37976523097073));
#30241=CARTESIAN_POINT('Ctrl Pts',(3.86932885813068,-1.,1.38034709213014));
#30242=CARTESIAN_POINT('Ctrl Pts',(3.86160143043959,-1.,1.3808920599299));
#30243=CARTESIAN_POINT('Ctrl Pts',(3.85387983979481,-1.,1.3813998311505));
#30244=CARTESIAN_POINT('Ctrl Pts',(3.84616425605764,-1.,1.38187013346109));
#30245=CARTESIAN_POINT('Ctrl Pts',(3.83845502790746,-1.,1.38230274828822));
#30246=CARTESIAN_POINT('Ctrl Pts',(3.8307526698229,-1.,1.38269750245138));
#30247=CARTESIAN_POINT('Ctrl Pts',(3.82305771743829,-1.,1.38305421262763));
#30248=CARTESIAN_POINT('Ctrl Pts',(3.81537060817811,-1.,1.38337263902782));
#30249=CARTESIAN_POINT('Ctrl Pts',(3.80769156398411,-1.,1.3836524404622));
#30250=CARTESIAN_POINT('Ctrl Pts',(3.80002044322111,-1.,1.38389311766682));
#30251=CARTESIAN_POINT('Ctrl Pts',(3.79235669640841,-1.,1.38409399694566));
#30252=CARTESIAN_POINT('Ctrl Pts',(3.78469969805082,-1.,1.38425435883756));
#30253=CARTESIAN_POINT('Ctrl Pts',(3.77704902230418,-1.,1.38437354551428));
#30254=CARTESIAN_POINT('Ctrl Pts',(3.76940473185779,-1.,1.38445107339518));
#30255=CARTESIAN_POINT('Ctrl Pts',(3.76176768271367,-1.,1.3844867525335));
#30256=CARTESIAN_POINT('Ctrl Pts',(3.7541397631875,-1.,1.38448077997163));
#30257=CARTESIAN_POINT('Ctrl Pts',(3.74652317167876,-1.,1.38443344984394));
#30258=CARTESIAN_POINT('Ctrl Pts',(3.73891976418104,-1.,1.38434489156458));
#30259=CARTESIAN_POINT('Ctrl Pts',(3.73133035859282,-1.,1.38421479111531));
#30260=CARTESIAN_POINT('Ctrl Pts',(3.72375409358803,-1.,1.3840421342895));
#30261=CARTESIAN_POINT('Ctrl Pts',(3.7161876605181,-1.,1.38382489984586));
#30262=CARTESIAN_POINT('Ctrl Pts',(3.70862680753347,-1.,1.38356065402124));
#30263=CARTESIAN_POINT('Ctrl Pts',(3.701067921679,-1.,1.38324717612865));
#30264=CARTESIAN_POINT('Ctrl Pts',(3.69350967899526,-1.,1.38288311171651));
#30265=CARTESIAN_POINT('Ctrl Pts',(3.68595444983837,-1.,1.38246852827182));
#30266=CARTESIAN_POINT('Ctrl Pts',(3.67841038482414,-1.,1.3820057429062));
#30267=CARTESIAN_POINT('Ctrl Pts',(3.67088843112262,-1.,1.38149812653868));
#30268=CARTESIAN_POINT('Ctrl Pts',(3.66339848520857,-1.,1.38094856333552));
#30269=CARTESIAN_POINT('Ctrl Pts',(3.6559455440439,-1.,1.38035791051213));
#30270=CARTESIAN_POINT('Ctrl Pts',(3.64852652756456,-1.,1.37972372481603));
#30271=CARTESIAN_POINT('Ctrl Pts',(3.64112507791141,-1.,1.37903818567359));
#30272=CARTESIAN_POINT('Ctrl Pts',(3.63371727442486,-1.,1.37829035457339));
#30273=CARTESIAN_POINT('Ctrl Pts',(3.62628098665145,-1.,1.37746987919881));
#30274=CARTESIAN_POINT('Ctrl Pts',(3.6188048116042,-1.,1.37657053403107));
#30275=CARTESIAN_POINT('Ctrl Pts',(3.61129546591064,-1.,1.37559314436634));
#30276=CARTESIAN_POINT('Ctrl Pts',(3.60379020123988,-1.,1.37455051379623));
#30277=CARTESIAN_POINT('Ctrl Pts',(3.59634627869048,-1.,1.37346320103157));
#30278=CARTESIAN_POINT('Ctrl Pts',(3.58901853846365,-1.,1.37235053660976));
#30279=CARTESIAN_POINT('Ctrl Pts',(3.58183885982715,-1.,1.37122241663062));
#30280=CARTESIAN_POINT('Ctrl Pts',(3.57479875549486,-1.,1.37007229485659));
#30281=CARTESIAN_POINT('Ctrl Pts',(3.5678208030466,-1.,1.36886584973389));
#30282=CARTESIAN_POINT('Ctrl Pts',(3.56077662028649,-1.,1.36754771771233));
#30283=CARTESIAN_POINT('Ctrl Pts',(3.55353883995949,-1.,1.3660614545677));
#30284=CARTESIAN_POINT('Ctrl Pts',(3.54602591832973,-1.,1.36436666257598));
#30285=CARTESIAN_POINT('Ctrl Pts',(3.53824396424961,-1.,1.36245507339307));
#30286=CARTESIAN_POINT('Ctrl Pts',(3.530344649616,-1.,1.36037259643734));
#30287=CARTESIAN_POINT('Ctrl Pts',(3.52261776116748,-1.,1.35821701528836));
#30288=CARTESIAN_POINT('Ctrl Pts',(3.51542230699556,-1.,1.35611275237152));
#30289=CARTESIAN_POINT('Ctrl Pts',(3.50913227059999,-1.,1.35419113575956));
#30290=CARTESIAN_POINT('Ctrl Pts',(3.50408168106261,-1.,1.35257032843486));
#30291=CARTESIAN_POINT('Ctrl Pts',(3.5007660381649,-1.,1.35142377279517));
#30292=CARTESIAN_POINT('Ctrl Pts',(3.49920025459723,-1.,1.35080045218587));
#30293=CARTESIAN_POINT('Ctrl Pts',(3.49861894124827,-1.,1.35049736560527));
#30294=CARTESIAN_POINT('Ctrl Pts',(3.49847119623846,-1.,1.35036670892966));
#30295=CARTESIAN_POINT('Ctrl Pts',(3.4984457533445,-1.,1.35032489087101));
#30296=CARTESIAN_POINT('',(3.42859860294378,-1.,1.51895082866166));
#30297=CARTESIAN_POINT('Origin',(0.,-1.,0.));
#30298=CARTESIAN_POINT('',(3.77614523045147,-1.,1.83867539237861));
#30299=CARTESIAN_POINT('Ctrl Pts',(3.42859860294378,-1.,1.51895082866166));
#30300=CARTESIAN_POINT('Ctrl Pts',(3.42864616361967,-1.,1.51893924967231));
#30301=CARTESIAN_POINT('Ctrl Pts',(3.42884302333978,-1.,1.51895133295017));
#30302=CARTESIAN_POINT('Ctrl Pts',(3.42946838852728,-1.,1.51914806898539));
#30303=CARTESIAN_POINT('Ctrl Pts',(3.4310163189349,-1.,1.5198144909343));
#30304=CARTESIAN_POINT('Ctrl Pts',(3.43417156977749,-1.,1.52134826724227));
#30305=CARTESIAN_POINT('Ctrl Pts',(3.43888895974182,-1.,1.52377348950429));
#30306=CARTESIAN_POINT('Ctrl Pts',(3.44469547527,-1.,1.52686242875717));
#30307=CARTESIAN_POINT('Ctrl Pts',(3.45127136828667,-1.,1.530462444618));
#30308=CARTESIAN_POINT('Ctrl Pts',(3.45825932955273,-1.,1.53440195378902));
#30309=CARTESIAN_POINT('Ctrl Pts',(3.46531752207222,-1.,1.53851507915533));
#30310=CARTESIAN_POINT('Ctrl Pts',(3.47217189224576,-1.,1.54266605398152));
#30311=CARTESIAN_POINT('Ctrl Pts',(3.47868272898599,-1.,1.54678009290207));
#30312=CARTESIAN_POINT('Ctrl Pts',(3.48485155928414,-1.,1.55084702970382));
#30313=CARTESIAN_POINT('Ctrl Pts',(3.49076460877317,-1.,1.5548959590107));
#30314=CARTESIAN_POINT('Ctrl Pts',(3.49655185179623,-1.,1.55897703097859));
#30315=CARTESIAN_POINT('Ctrl Pts',(3.50234321621607,-1.,1.56314187758689));
#30316=CARTESIAN_POINT('Ctrl Pts',(3.50821771695427,-1.,1.56742097575041));
#30317=CARTESIAN_POINT('Ctrl Pts',(3.51418598431733,-1.,1.57181569799774));
#30318=CARTESIAN_POINT('Ctrl Pts',(3.52021847865961,-1.,1.5763104998818));
#30319=CARTESIAN_POINT('Ctrl Pts',(3.52626275334899,-1.,1.58088027227856));
#30320=CARTESIAN_POINT('Ctrl Pts',(3.53226378147068,-1.,1.58549906268083));
#30321=CARTESIAN_POINT('Ctrl Pts',(3.53818616861045,-1.,1.59014958368725));
#30322=CARTESIAN_POINT('Ctrl Pts',(3.544024581823,-1.,1.5948276694975));
#30323=CARTESIAN_POINT('Ctrl Pts',(3.54979148634426,-1.,1.59953698113444));
#30324=CARTESIAN_POINT('Ctrl Pts',(3.55550985096117,-1.,1.60428584699848));
#30325=CARTESIAN_POINT('Ctrl Pts',(3.56120432482986,-1.,1.60908344685459));
#30326=CARTESIAN_POINT('Ctrl Pts',(3.56689200468404,-1.,1.61393581747522));
#30327=CARTESIAN_POINT('Ctrl Pts',(3.57257679609826,-1.,1.61884340915412));
#30328=CARTESIAN_POINT('Ctrl Pts',(3.57825455954405,-1.,1.62380329464851));
#30329=CARTESIAN_POINT('Ctrl Pts',(3.5839162577435,-1.,1.62881051550748));
#30330=CARTESIAN_POINT('Ctrl Pts',(3.58955176627876,-1.,1.63385971451259));
#30331=CARTESIAN_POINT('Ctrl Pts',(3.59515368334887,-1.,1.63894676675349));
#30332=CARTESIAN_POINT('Ctrl Pts',(3.6007202851384,-1.,1.6440700438558));
#30333=CARTESIAN_POINT('Ctrl Pts',(3.60625346556992,-1.,1.64922952425833));
#30334=CARTESIAN_POINT('Ctrl Pts',(3.61175734965129,-1.,1.65442619244327));
#30335=CARTESIAN_POINT('Ctrl Pts',(3.61723666482457,-1.,1.65966133399186));
#30336=CARTESIAN_POINT('Ctrl Pts',(3.62269517989104,-1.,1.66493585923853));
#30337=CARTESIAN_POINT('Ctrl Pts',(3.62813422105257,-1.,1.67024966008037));
#30338=CARTESIAN_POINT('Ctrl Pts',(3.63355343201211,-1.,1.67560193613145));
#30339=CARTESIAN_POINT('Ctrl Pts',(3.63895140887443,-1.,1.68099146651577));
#30340=CARTESIAN_POINT('Ctrl Pts',(3.64432638915199,-1.,1.68641690471455));
#30341=CARTESIAN_POINT('Ctrl Pts',(3.64967689827393,-1.,1.691877054817));
#30342=CARTESIAN_POINT('Ctrl Pts',(3.65500246526798,-1.,1.69737117722559));
#30343=CARTESIAN_POINT('Ctrl Pts',(3.6603033877491,-1.,1.70289888566904));
#30344=CARTESIAN_POINT('Ctrl Pts',(3.6655804319893,-1.,1.70846001610983));
#30345=CARTESIAN_POINT('Ctrl Pts',(3.67083454901629,-1.,1.71405450210392));
#30346=CARTESIAN_POINT('Ctrl Pts',(3.67606660374665,-1.,1.71968225581787));
#30347=CARTESIAN_POINT('Ctrl Pts',(3.68127704936472,-1.,1.72534302437003));
#30348=CARTESIAN_POINT('Ctrl Pts',(3.68646597019188,-1.,1.73103640956647));
#30349=CARTESIAN_POINT('Ctrl Pts',(3.69163322647906,-1.,1.73676193254493));
#30350=CARTESIAN_POINT('Ctrl Pts',(3.6967785691046,-1.,1.74251908492589));
#30351=CARTESIAN_POINT('Ctrl Pts',(3.70190175673422,-1.,1.74830738046092));
#30352=CARTESIAN_POINT('Ctrl Pts',(3.70700269736876,-1.,1.75412641804148));
#30353=CARTESIAN_POINT('Ctrl Pts',(3.71208146346454,-1.,1.75997588499021));
#30354=CARTESIAN_POINT('Ctrl Pts',(3.71713822377675,-1.,1.76585552124549));
#30355=CARTESIAN_POINT('Ctrl Pts',(3.72217319911429,-1.,1.77176509401846));
#30356=CARTESIAN_POINT('Ctrl Pts',(3.72718661205504,-1.,1.77770437039606));
#30357=CARTESIAN_POINT('Ctrl Pts',(3.73217863095022,-1.,1.78367308442682));
#30358=CARTESIAN_POINT('Ctrl Pts',(3.73714934729962,-1.,1.78967092823139));
#30359=CARTESIAN_POINT('Ctrl Pts',(3.74209880351667,-1.,1.79569757859041));
#30360=CARTESIAN_POINT('Ctrl Pts',(3.74702700874954,-1.,1.80175271485519));
#30361=CARTESIAN_POINT('Ctrl Pts',(3.75193395888069,-1.,1.80783603939662));
#30362=CARTESIAN_POINT('Ctrl Pts',(3.75681965683995,-1.,1.81394729834032));
#30363=CARTESIAN_POINT('Ctrl Pts',(3.76168412709652,-1.,1.82008629694924));
#30364=CARTESIAN_POINT('Ctrl Pts',(3.76652740355856,-1.,1.82625289221933));
#30365=CARTESIAN_POINT('Ctrl Pts',(3.77038509819777,-1.,1.83120816956515));
#30366=CARTESIAN_POINT('Ctrl Pts',(3.77326886065484,-1.,1.83493697935064));
#30367=CARTESIAN_POINT('Ctrl Pts',(3.77518714458232,-1.,1.83742834010821));
#30368=CARTESIAN_POINT('Ctrl Pts',(3.77614523045147,-1.,1.83867539237861));
#30369=CARTESIAN_POINT('',(3.70708211654725,-1.,1.97421938526992));
#30370=CARTESIAN_POINT('',(3.77614523045147,-1.,1.83867539237861));
#30371=CARTESIAN_POINT('',(3.24413672884902,-1.,1.88097764062542));
#30372=CARTESIAN_POINT('Ctrl Pts',(3.70708211654725,-1.,1.97421938526992));
#30373=CARTESIAN_POINT('Ctrl Pts',(3.7055100813194,-1.,1.974177276451));
#30374=CARTESIAN_POINT('Ctrl Pts',(3.70236698911837,-1.,1.97408973726149));
#30375=CARTESIAN_POINT('Ctrl Pts',(3.69765528558292,-1.,1.97394846382289));
#30376=CARTESIAN_POINT('Ctrl Pts',(3.69137888597855,-1.,1.97374016224397));
#30377=CARTESIAN_POINT('Ctrl Pts',(3.68354319913416,-1.,1.97344650303631));
#30378=CARTESIAN_POINT('Ctrl Pts',(3.67571738106175,-1.,1.97311947678035));
#30379=CARTESIAN_POINT('Ctrl Pts',(3.66790152751984,-1.,1.9727589719863));
#30380=CARTESIAN_POINT('Ctrl Pts',(3.66009578166865,-1.,1.97236485439317));
#30381=CARTESIAN_POINT('Ctrl Pts',(3.65230034717364,-1.,1.97193697240645));
#30382=CARTESIAN_POINT('Ctrl Pts',(3.64451546724221,-1.,1.97147515441539));
#30383=CARTESIAN_POINT('Ctrl Pts',(3.63674139590853,-1.,1.97097920454698));
#30384=CARTESIAN_POINT('Ctrl Pts',(3.62897836973397,-1.,1.97044889850518));
#30385=CARTESIAN_POINT('Ctrl Pts',(3.62122658401722,-1.,1.96988398129888));
#30386=CARTESIAN_POINT('Ctrl Pts',(3.61348615496393,-1.,1.96928416040712));
#30387=CARTESIAN_POINT('Ctrl Pts',(3.60575714017676,-1.,1.96864911885775));
#30388=CARTESIAN_POINT('Ctrl Pts',(3.59803959819725,-1.,1.96797854118257));
#30389=CARTESIAN_POINT('Ctrl Pts',(3.5903336402273,-1.,1.96727213799507));
#30390=CARTESIAN_POINT('Ctrl Pts',(3.58263947663884,-1.,1.9665296668894));
#30391=CARTESIAN_POINT('Ctrl Pts',(3.57495748601088,-1.,1.96575096652857));
#30392=CARTESIAN_POINT('Ctrl Pts',(3.56728820357933,-1.,1.96493594634643));
#30393=CARTESIAN_POINT('Ctrl Pts',(3.55963218706201,-1.,1.96408450906868));
#30394=CARTESIAN_POINT('Ctrl Pts',(3.55198990600929,-1.,1.96319648628667));
#30395=CARTESIAN_POINT('Ctrl Pts',(3.54436163300425,-1.,1.96227157573058));
#30396=CARTESIAN_POINT('Ctrl Pts',(3.53674730625759,-1.,1.96130926212661));
#30397=CARTESIAN_POINT('Ctrl Pts',(3.52914648844289,-1.,1.96030879411534));
#30398=CARTESIAN_POINT('Ctrl Pts',(3.52155867431438,-1.,1.95926936324436));
#30399=CARTESIAN_POINT('Ctrl Pts',(3.51398354617772,-1.,1.95819025316768));
#30400=CARTESIAN_POINT('Ctrl Pts',(3.50642124159913,-1.,1.95707099606514));
#30401=CARTESIAN_POINT('Ctrl Pts',(3.49887263575602,-1.,1.9559115382367));
#30402=CARTESIAN_POINT('Ctrl Pts',(3.49133956289154,-1.,1.95471236969653));
#30403=CARTESIAN_POINT('Ctrl Pts',(3.48382414832648,-1.,1.95347412486316));
#30404=CARTESIAN_POINT('Ctrl Pts',(3.47632820495926,-1.,1.95219722189878));
#30405=CARTESIAN_POINT('Ctrl Pts',(3.4688525897419,-1.,1.95088147859876));
#30406=CARTESIAN_POINT('Ctrl Pts',(3.46139661060959,-1.,1.94952575850196));
#30407=CARTESIAN_POINT('Ctrl Pts',(3.45395731584051,-1.,1.94812754766524));
#30408=CARTESIAN_POINT('Ctrl Pts',(3.44653088665685,-1.,1.94668377715332));
#30409=CARTESIAN_POINT('Ctrl Pts',(3.43911410197693,-1.,1.94519168842883));
#30410=CARTESIAN_POINT('Ctrl Pts',(3.43170586602436,-1.,1.94364973660285));
#30411=CARTESIAN_POINT('Ctrl Pts',(3.42430850941497,-1.,1.94205835913692));
#30412=CARTESIAN_POINT('Ctrl Pts',(3.41692971994082,-1.,1.94042111965237));
#30413=CARTESIAN_POINT('Ctrl Pts',(3.40957978266622,-1.,1.93874306008132));
#30414=CARTESIAN_POINT('Ctrl Pts',(3.40226802104093,-1.,1.93702857723089));
#30415=CARTESIAN_POINT('Ctrl Pts',(3.39499923640789,-1.,1.93527929945982));
#30416=CARTESIAN_POINT('Ctrl Pts',(3.38777076883267,-1.,1.93349233176794));
#30417=CARTESIAN_POINT('Ctrl Pts',(3.38056768525577,-1.,1.93165739093292));
#30418=CARTESIAN_POINT('Ctrl Pts',(3.37336807068078,-1.,1.92975993109897));
#30419=CARTESIAN_POINT('Ctrl Pts',(3.36615168657597,-1.,1.92778626543803));
#30420=CARTESIAN_POINT('Ctrl Pts',(3.35890824422976,-1.,1.92572846125763));
#30421=CARTESIAN_POINT('Ctrl Pts',(3.35164424847206,-1.,1.92358838440518));
#30422=CARTESIAN_POINT('Ctrl Pts',(3.34439448941915,-1.,1.92138450828378));
#30423=CARTESIAN_POINT('Ctrl Pts',(3.33721230709948,-1.,1.91914609610173));
#30424=CARTESIAN_POINT('Ctrl Pts',(3.33014884257812,-1.,1.91690081930297));
#30425=CARTESIAN_POINT('Ctrl Pts',(3.32323403454507,-1.,1.91466343916612));
#30426=CARTESIAN_POINT('Ctrl Pts',(3.31646052426395,-1.,1.91242616234459));
#30427=CARTESIAN_POINT('Ctrl Pts',(3.30975721158694,-1.,1.91014297830502));
#30428=CARTESIAN_POINT('Ctrl Pts',(3.30300595568341,-1.,1.90773912171424));
#30429=CARTESIAN_POINT('Ctrl Pts',(3.29608978722258,-1.,1.9051389186417));
#30430=CARTESIAN_POINT('Ctrl Pts',(3.28893448600364,-1.,1.9022897124757));
#30431=CARTESIAN_POINT('Ctrl Pts',(3.28154737912287,-1.,1.89918429230425));
#30432=CARTESIAN_POINT('Ctrl Pts',(3.27407108932908,-1.,1.89589172903662));
#30433=CARTESIAN_POINT('Ctrl Pts',(3.2667765388833,-1.,1.89255393500769));
#30434=CARTESIAN_POINT('Ctrl Pts',(3.2599988519361,-1.,1.88934996203508));
#30435=CARTESIAN_POINT('Ctrl Pts',(3.25408686339298,-1.,1.88646802523372));
#30436=CARTESIAN_POINT('Ctrl Pts',(3.24935200512055,-1.,1.88407708646435));
#30437=CARTESIAN_POINT('Ctrl Pts',(3.24625654410705,-1.,1.88242596600422));
#30438=CARTESIAN_POINT('Ctrl Pts',(3.24480754675942,-1.,1.88156537699118));
#30439=CARTESIAN_POINT('Ctrl Pts',(3.24428080352952,-1.,1.88117508446657));
#30440=CARTESIAN_POINT('Ctrl Pts',(3.2441553167131,-1.,1.88102292397987));
#30441=CARTESIAN_POINT('Ctrl Pts',(3.24413672884902,-1.,1.88097764062542));
#30442=CARTESIAN_POINT('',(3.14877060440425,-1.,2.03660101169564));
#30443=CARTESIAN_POINT('Origin',(0.,-1.,0.));
#30444=CARTESIAN_POINT('',(3.44202241512147,-1.,2.40675750623143));
#30445=CARTESIAN_POINT('Ctrl Pts',(3.14877060440425,-1.,2.03660101169564));
#30446=CARTESIAN_POINT('Ctrl Pts',(3.1488193908823,-1.,2.03659701539175));
#30447=CARTESIAN_POINT('Ctrl Pts',(3.14901193669147,-1.,2.03663974554941));
#30448=CARTESIAN_POINT('Ctrl Pts',(3.14959882629936,-1.,2.03693188810614));
#30449=CARTESIAN_POINT('Ctrl Pts',(3.15102344775396,-1.,2.03783225496023));
#30450=CARTESIAN_POINT('Ctrl Pts',(3.1538999167466,-1.,2.03984073791432));
#30451=CARTESIAN_POINT('Ctrl Pts',(3.15817983946525,-1.,2.04297406404132));
#30452=CARTESIAN_POINT('Ctrl Pts',(3.16343165059235,-1.,2.0469333124766));
#30453=CARTESIAN_POINT('Ctrl Pts',(3.16936341689859,-1.,2.05151770247452));
#30454=CARTESIAN_POINT('Ctrl Pts',(3.17564906975592,-1.,2.05650186773279));
#30455=CARTESIAN_POINT('Ctrl Pts',(3.18197692964677,-1.,2.06166849827143));
#30456=CARTESIAN_POINT('Ctrl Pts',(3.18809755562297,-1.,2.06684062744065));
#30457=CARTESIAN_POINT('Ctrl Pts',(3.19388465568113,-1.,2.07192253497765));
#30458=CARTESIAN_POINT('Ctrl Pts',(3.19934132835879,-1.,2.0769044187063));
#30459=CARTESIAN_POINT('Ctrl Pts',(3.20454818630635,-1.,2.08182850370816));
#30460=CARTESIAN_POINT('Ctrl Pts',(3.20962575845433,-1.,2.08676465517435));
#30461=CARTESIAN_POINT('Ctrl Pts',(3.2146942960168,-1.,2.0917841946046));
#30462=CARTESIAN_POINT('Ctrl Pts',(3.21982707347067,-1.,2.09692958434933));
#30463=CARTESIAN_POINT('Ctrl Pts',(3.22503437553496,-1.,2.10220384298534));
#30464=CARTESIAN_POINT('Ctrl Pts',(3.23028945793334,-1.,2.1075869964248));
#30465=CARTESIAN_POINT('Ctrl Pts',(3.23554444767115,-1.,2.11304604021784));
#30466=CARTESIAN_POINT('Ctrl Pts',(3.24074905517282,-1.,2.11854673326972));
#30467=CARTESIAN_POINT('Ctrl Pts',(3.24587102613347,-1.,2.12406646410943));
#30468=CARTESIAN_POINT('Ctrl Pts',(3.25090574493994,-1.,2.1296002839681));
#30469=CARTESIAN_POINT('Ctrl Pts',(3.25586495065027,-1.,2.13515375878786));
#30470=CARTESIAN_POINT('Ctrl Pts',(3.26077002641868,-1.,2.14073870754258));
#30471=CARTESIAN_POINT('Ctrl Pts',(3.26564388189764,-1.,2.14636805295663));
#30472=CARTESIAN_POINT('Ctrl Pts',(3.27050245897244,-1.,2.15205043199818));
#30473=CARTESIAN_POINT('Ctrl Pts',(3.27534954469206,-1.,2.15778690038359));
#30474=CARTESIAN_POINT('Ctrl Pts',(3.28018150841414,-1.,2.16357391934434));
#30475=CARTESIAN_POINT('Ctrl Pts',(3.2849901997973,-1.,2.16940517773459));
#30476=CARTESIAN_POINT('Ctrl Pts',(3.28976645712566,-1.,2.17527380048422));
#30477=CARTESIAN_POINT('Ctrl Pts',(3.29450361500484,-1.,2.18117455557062));
#30478=CARTESIAN_POINT('Ctrl Pts',(3.29920022557635,-1.,2.18710556500325));
#30479=CARTESIAN_POINT('Ctrl Pts',(3.30385816281831,-1.,2.19306710376112));
#30480=CARTESIAN_POINT('Ctrl Pts',(3.30848134694596,-1.,2.19906078949925));
#30481=CARTESIAN_POINT('Ctrl Pts',(3.3130742460895,-1.,2.20508863150608));
#30482=CARTESIAN_POINT('Ctrl Pts',(3.31764044024231,-1.,2.21115211847872));
#30483=CARTESIAN_POINT('Ctrl Pts',(3.32218125618955,-1.,2.21725135110889));
#30484=CARTESIAN_POINT('Ctrl Pts',(3.32669646722871,-1.,2.22338548312759));
#30485=CARTESIAN_POINT('Ctrl Pts',(3.33118487773593,-1.,2.22955308907221));
#30486=CARTESIAN_POINT('Ctrl Pts',(3.33564495756478,-1.,2.2357525632881));
#30487=CARTESIAN_POINT('Ctrl Pts',(3.34007543738044,-1.,2.24198249391437));
#30488=CARTESIAN_POINT('Ctrl Pts',(3.34447596770768,-1.,2.24824207678288));
#30489=CARTESIAN_POINT('Ctrl Pts',(3.34884690292342,-1.,2.25453097693524));
#30490=CARTESIAN_POINT('Ctrl Pts',(3.35318902552676,-1.,2.26084915222484));
#30491=CARTESIAN_POINT('Ctrl Pts',(3.35750328523077,-1.,2.26719668579921));
#30492=CARTESIAN_POINT('Ctrl Pts',(3.36179055004369,-1.,2.27357362620902));
#30493=CARTESIAN_POINT('Ctrl Pts',(3.36605130712978,-1.,2.27997979457968));
#30494=CARTESIAN_POINT('Ctrl Pts',(3.37028570206357,-1.,2.28641481081045));
#30495=CARTESIAN_POINT('Ctrl Pts',(3.37449367172707,-1.,2.2928781800731));
#30496=CARTESIAN_POINT('Ctrl Pts',(3.37867504959382,-1.,2.29936936127588));
#30497=CARTESIAN_POINT('Ctrl Pts',(3.38282967336676,-1.,2.30588783640389));
#30498=CARTESIAN_POINT('Ctrl Pts',(3.38695751492659,-1.,2.31243319489505));
#30499=CARTESIAN_POINT('Ctrl Pts',(3.39105869475112,-1.,2.31900513925627));
#30500=CARTESIAN_POINT('Ctrl Pts',(3.39513342020045,-1.,2.32560343902683));
#30501=CARTESIAN_POINT('Ctrl Pts',(3.39918194578115,-1.,2.33222789882601));
#30502=CARTESIAN_POINT('Ctrl Pts',(3.40320452776646,-1.,2.33887832342715));
#30503=CARTESIAN_POINT('Ctrl Pts',(3.40720137403888,-1.,2.34555447648901));
#30504=CARTESIAN_POINT('Ctrl Pts',(3.41117262313464,-1.,2.35225606823649));
#30505=CARTESIAN_POINT('Ctrl Pts',(3.4151183675076,-1.,2.35898278606449));
#30506=CARTESIAN_POINT('Ctrl Pts',(3.41903866635384,-1.,2.36573431470314));
#30507=CARTESIAN_POINT('Ctrl Pts',(3.42293356216595,-1.,2.37251035954351));
#30508=CARTESIAN_POINT('Ctrl Pts',(3.42680309755241,-1.,2.37931067029517));
#30509=CARTESIAN_POINT('Ctrl Pts',(3.43064732714472,-1.,2.38613505844641));
#30510=CARTESIAN_POINT('Ctrl Pts',(3.43446630680436,-1.,2.39298338805823));
#30511=CARTESIAN_POINT('Ctrl Pts',(3.43750133066036,-1.,2.39848113411429));
#30512=CARTESIAN_POINT('Ctrl Pts',(3.43976627485223,-1.,2.40261515590099));
#30513=CARTESIAN_POINT('Ctrl Pts',(3.44127120683402,-1.,2.40537592959345));
#30514=CARTESIAN_POINT('Ctrl Pts',(3.44202241512147,-1.,2.40675750623143));
#30515=CARTESIAN_POINT('',(3.35260583073571,-1.,2.52982887637028));
#30516=CARTESIAN_POINT('',(3.44202241512147,-1.,2.40675750623143));
#30517=CARTESIAN_POINT('',(2.90994629141676,-1.,2.36531447826074));
#30518=CARTESIAN_POINT('Ctrl Pts',(3.35260583073571,-1.,2.52982887637028));
#30519=CARTESIAN_POINT('Ctrl Pts',(3.35105973714071,-1.,2.5295413654909));
#30520=CARTESIAN_POINT('Ctrl Pts',(3.34796903576663,-1.,2.52896321610703));
#30521=CARTESIAN_POINT('Ctrl Pts',(3.34333744115511,-1.,2.52808660915689));
#30522=CARTESIAN_POINT('Ctrl Pts',(3.33717089999103,-1.,2.52689902690158));
#30523=CARTESIAN_POINT('Ctrl Pts',(3.32947762187533,-1.,2.52538321164634));
#30524=CARTESIAN_POINT('Ctrl Pts',(3.32179931078699,-1.,2.5238359839626));
#30525=CARTESIAN_POINT('Ctrl Pts',(3.31413607874645,-1.,2.52225724871313));
#30526=CARTESIAN_POINT('Ctrl Pts',(3.30648808815442,-1.,2.52064689568511));
#30527=CARTESIAN_POINT('Ctrl Pts',(3.29885556388352,-1.,2.51900480701069));
#30528=CARTESIAN_POINT('Ctrl Pts',(3.2912387729927,-1.,2.51733085123797));
#30529=CARTESIAN_POINT('Ctrl Pts',(3.28363799702982,-1.,2.51562487464514));
#30530=CARTESIAN_POINT('Ctrl Pts',(3.27605350473142,-1.,2.513886692704));
#30531=CARTESIAN_POINT('Ctrl Pts',(3.26848552888115,-1.,2.51211608411423));
#30532=CARTESIAN_POINT('Ctrl Pts',(3.26093423001434,-1.,2.51031277813486));
#30533=CARTESIAN_POINT('Ctrl Pts',(3.25339971460982,-1.,2.50847647070723));
#30534=CARTESIAN_POINT('Ctrl Pts',(3.24588208983849,-1.,2.506606859405));
#30535=CARTESIAN_POINT('Ctrl Pts',(3.23838151080319,-1.,2.5047036758003));
#30536=CARTESIAN_POINT('Ctrl Pts',(3.23089822320646,-1.,2.50276671338111));
#30537=CARTESIAN_POINT('Ctrl Pts',(3.22343262620503,-1.,2.50079587201958));
#30538=CARTESIAN_POINT('Ctrl Pts',(3.21598526261286,-1.,2.4987911459939));
#30539=CARTESIAN_POINT('Ctrl Pts',(3.20855669849836,-1.,2.4967525264737));
#30540=CARTESIAN_POINT('Ctrl Pts',(3.20114742397588,-1.,2.49467992057755));
#30541=CARTESIAN_POINT('Ctrl Pts',(3.19375775555798,-1.,2.49257307239848));
#30542=CARTESIAN_POINT('Ctrl Pts',(3.18638771282266,-1.,2.49043146334059));
#30543=CARTESIAN_POINT('Ctrl Pts',(3.17903698136622,-1.,2.48825428288201));
#30544=CARTESIAN_POINT('Ctrl Pts',(3.17170518863313,-1.,2.48604065348587));
#30545=CARTESIAN_POINT('Ctrl Pts',(3.16439213290161,-1.,2.48378981792725));
#30546=CARTESIAN_POINT('Ctrl Pts',(3.15709802322739,-1.,2.48150133566571));
#30547=CARTESIAN_POINT('Ctrl Pts',(3.14982373241352,-1.,2.47917529057029));
#30548=CARTESIAN_POINT('Ctrl Pts',(3.1425709954655,-1.,2.47681245356109));
#30549=CARTESIAN_POINT('Ctrl Pts',(3.13534181229295,-1.,2.47441378371932));
#30550=CARTESIAN_POINT('Ctrl Pts',(3.12813790805952,-1.,2.47197997765871));
#30551=CARTESIAN_POINT('Ctrl Pts',(3.12096015766983,-1.,2.46951098947469));
#30552=CARTESIAN_POINT('Ctrl Pts',(3.11380805536122,-1.,2.46700558843506));
#30553=CARTESIAN_POINT('Ctrl Pts',(3.1066790790198,-1.,2.46446082979646));
#30554=CARTESIAN_POINT('Ctrl Pts',(3.09956993697052,-1.,2.46187308501884));
#30555=CARTESIAN_POINT('Ctrl Pts',(3.09247787931887,-1.,2.4592391256388));
#30556=CARTESIAN_POINT('Ctrl Pts',(3.08540206545315,-1.,2.45655725437039));
#30557=CARTESIAN_POINT('Ctrl Pts',(3.07834472886139,-1.,2.4538282678779));
#30558=CARTESIAN_POINT('Ctrl Pts',(3.07131290521297,-1.,2.45105688854422));
#30559=CARTESIAN_POINT('Ctrl Pts',(3.06431596421405,-1.,2.44824970516544));
#30560=CARTESIAN_POINT('Ctrl Pts',(3.05736242671506,-1.,2.44541251892556));
#30561=CARTESIAN_POINT('Ctrl Pts',(3.05045678021504,-1.,2.44254768923105));
#30562=CARTESIAN_POINT('Ctrl Pts',(3.04359685040555,-1.,2.43965194061857));
#30563=CARTESIAN_POINT('Ctrl Pts',(3.03676949672821,-1.,2.43671278042414));
#30564=CARTESIAN_POINT('Ctrl Pts',(3.02995534946978,-1.,2.43371241361488));
#30565=CARTESIAN_POINT('Ctrl Pts',(3.02313656036004,-1.,2.43063415586637));
#30566=CARTESIAN_POINT('Ctrl Pts',(3.01630420830504,-1.,2.42746856264168));
#30567=CARTESIAN_POINT('Ctrl Pts',(3.00946442616658,-1.,2.42421849439613));
#30568=CARTESIAN_POINT('Ctrl Pts',(3.00264868585996,-1.,2.42090763946779));
#30569=CARTESIAN_POINT('Ctrl Pts',(2.99590509293503,-1.,2.41757324500514));
#30570=CARTESIAN_POINT('Ctrl Pts',(2.98927983005796,-1.,2.41425064199586));
#30571=CARTESIAN_POINT('Ctrl Pts',(2.98280015815107,-1.,2.41095909342571));
#30572=CARTESIAN_POINT('Ctrl Pts',(2.97646002822422,-1.,2.40768975073713));
#30573=CARTESIAN_POINT('Ctrl Pts',(2.9701964131236,-1.,2.40438604734919));
#30574=CARTESIAN_POINT('Ctrl Pts',(2.96390432240312,-1.,2.4009556571164));
#30575=CARTESIAN_POINT('Ctrl Pts',(2.95748006482942,-1.,2.39730553974517));
#30576=CARTESIAN_POINT('Ctrl Pts',(2.95085857128439,-1.,2.39337207631667));
#30577=CARTESIAN_POINT('Ctrl Pts',(2.94404820669076,-1.,2.38914929090759));
#30578=CARTESIAN_POINT('Ctrl Pts',(2.93717903280391,-1.,2.38472771516311));
#30579=CARTESIAN_POINT('Ctrl Pts',(2.93049643640206,-1.,2.38028989582073));
#30580=CARTESIAN_POINT('Ctrl Pts',(2.92430340582608,-1.,2.3760651052403));
#30581=CARTESIAN_POINT('Ctrl Pts',(2.91891503791411,-1.,2.37229381109821));
#30582=CARTESIAN_POINT('Ctrl Pts',(2.9146124988314,-1.,2.36919161373173));
#30583=CARTESIAN_POINT('Ctrl Pts',(2.91181344022548,-1.,2.36707658451664));
#30584=CARTESIAN_POINT('Ctrl Pts',(2.91051690822156,-1.,2.36599991765749));
#30585=CARTESIAN_POINT('Ctrl Pts',(2.91005770527719,-1.,2.36553202948613));
#30586=CARTESIAN_POINT('Ctrl Pts',(2.90995756655606,-1.,2.36536211188453));
#30587=CARTESIAN_POINT('Ctrl Pts',(2.90994629141676,-1.,2.36531447826074));
#30588=CARTESIAN_POINT('',(2.79140942341378,-1.,2.50410331873042));
#30589=CARTESIAN_POINT('Origin',(0.,-1.,0.));
#30590=CARTESIAN_POINT('',(3.02314558451372,-1.,2.91557726271063));
#30591=CARTESIAN_POINT('Ctrl Pts',(2.79140942341378,-1.,2.50410331873043));
#30592=CARTESIAN_POINT('Ctrl Pts',(2.79145823440899,-1.,2.50410700351427));
#30593=CARTESIAN_POINT('Ctrl Pts',(2.79164172519039,-1.,2.50417932839343));
#30594=CARTESIAN_POINT('Ctrl Pts',(2.79217568804874,-1.,2.50455968395235));
#30595=CARTESIAN_POINT('Ctrl Pts',(2.79344192164204,-1.,2.50567182569153));
#30596=CARTESIAN_POINT('Ctrl Pts',(2.7959687805717,-1.,2.50810555977564));
#30597=CARTESIAN_POINT('Ctrl Pts',(2.79970585014308,-1.,2.51186983687947));
#30598=CARTESIAN_POINT('Ctrl Pts',(2.80427363984939,-1.,2.51660190466067));
#30599=CARTESIAN_POINT('Ctrl Pts',(2.80941521967234,-1.,2.52205778589922));
#30600=CARTESIAN_POINT('Ctrl Pts',(2.8148437904867,-1.,2.52796388055457));
#30601=CARTESIAN_POINT('Ctrl Pts',(2.82028550483744,-1.,2.53405679667463));
#30602=CARTESIAN_POINT('Ctrl Pts',(2.82552167649157,-1.,2.54012272520141));
#30603=CARTESIAN_POINT('Ctrl Pts',(2.83044254225794,-1.,2.54604736792542));
#30604=CARTESIAN_POINT('Ctrl Pts',(2.83505269592412,-1.,2.55182152806964));
#30605=CARTESIAN_POINT('Ctrl Pts',(2.83942515220699,-1.,2.55749952145165));
#30606=CARTESIAN_POINT('Ctrl Pts',(2.84366802680211,-1.,2.56316920798489));
#30607=CARTESIAN_POINT('Ctrl Pts',(2.84788893329091,-1.,2.56891984251743));
#30608=CARTESIAN_POINT('Ctrl Pts',(2.85215360144482,-1.,2.57480482727128));
#30609=CARTESIAN_POINT('Ctrl Pts',(2.85647171715147,-1.,2.58082875254407));
#30610=CARTESIAN_POINT('Ctrl Pts',(2.86081999003668,-1.,2.5869677064356));
#30611=CARTESIAN_POINT('Ctrl Pts',(2.86515629953528,-1.,2.59318160184921));
#30612=CARTESIAN_POINT('Ctrl Pts',(2.86943633170712,-1.,2.59942875223202));
#30613=CARTESIAN_POINT('Ctrl Pts',(2.87363176656475,-1.,2.6056817788128));
#30614=CARTESIAN_POINT('Ctrl Pts',(2.87773881947885,-1.,2.61193507170928));
#30615=CARTESIAN_POINT('Ctrl Pts',(2.88176821427502,-1.,2.61819596473087));
#30616=CARTESIAN_POINT('Ctrl Pts',(2.88573922195049,-1.,2.62447947640253));
#30617=CARTESIAN_POINT('Ctrl Pts',(2.88967244854243,-1.,2.63080195420771));
#30618=CARTESIAN_POINT('Ctrl Pts',(2.89358228854557,-1.,2.63717442263944));
#30619=CARTESIAN_POINT('Ctrl Pts',(2.89747231723361,-1.,2.64359851684146));
#30620=CARTESIAN_POINT('Ctrl Pts',(2.90133950224879,-1.,2.65007017365576));
#30621=CARTESIAN_POINT('Ctrl Pts',(2.90517678087467,-1.,2.65658188464287));
#30622=CARTESIAN_POINT('Ctrl Pts',(2.90897617968921,-1.,2.66312542616809));
#30623=CARTESIAN_POINT('Ctrl Pts',(2.91273193382876,-1.,2.66969458792627));
#30624=CARTESIAN_POINT('Ctrl Pts',(2.91644290704281,-1.,2.67628728855309));
#30625=CARTESIAN_POINT('Ctrl Pts',(2.92011090722152,-1.,2.68290409279689));
#30626=CARTESIAN_POINT('Ctrl Pts',(2.92373955325876,-1.,2.68954721165342));
#30627=CARTESIAN_POINT('Ctrl Pts',(2.92733294395268,-1.,2.69621932864302));
#30628=CARTESIAN_POINT('Ctrl Pts',(2.93089438233746,-1.,2.70292247416881));
#30629=CARTESIAN_POINT('Ctrl Pts',(2.93442516311167,-1.,2.70965695523776));
#30630=CARTESIAN_POINT('Ctrl Pts',(2.93792519474955,-1.,2.71642190053575));
#30631=CARTESIAN_POINT('Ctrl Pts',(2.94139351933882,-1.,2.72321571511322));
#30632=CARTESIAN_POINT('Ctrl Pts',(2.94482887675139,-1.,2.73003657371613));
#30633=CARTESIAN_POINT('Ctrl Pts',(2.94823023414381,-1.,2.73688288329825));
#30634=CARTESIAN_POINT('Ctrl Pts',(2.95159737214304,-1.,2.7437537949221));
#30635=CARTESIAN_POINT('Ctrl Pts',(2.95493069316211,-1.,2.75064903318996));
#30636=CARTESIAN_POINT('Ctrl Pts',(2.9582309766594,-1.,2.75756867888393));
#30637=CARTESIAN_POINT('Ctrl Pts',(2.96149914764832,-1.,2.76451296269571));
#30638=CARTESIAN_POINT('Ctrl Pts',(2.96473605585548,-1.,2.77148206836464));
#30639=CARTESIAN_POINT('Ctrl Pts',(2.9679422104295,-1.,2.77847589542767));
#30640=CARTESIAN_POINT('Ctrl Pts',(2.97111781461349,-1.,2.78549409123657));
#30641=CARTESIAN_POINT('Ctrl Pts',(2.97426288347475,-1.,2.79253615718147));
#30642=CARTESIAN_POINT('Ctrl Pts',(2.97737733718242,-1.,2.79960153278186));
#30643=CARTESIAN_POINT('Ctrl Pts',(2.98046109647299,-1.,2.80668968101162));
#30644=CARTESIAN_POINT('Ctrl Pts',(2.9835141977994,-1.,2.81380019196454));
#30645=CARTESIAN_POINT('Ctrl Pts',(2.98653680669434,-1.,2.82093279065704));
#30646=CARTESIAN_POINT('Ctrl Pts',(2.98952916401699,-1.,2.82808728190402));
#30647=CARTESIAN_POINT('Ctrl Pts',(2.99249155170479,-1.,2.83526351254383));
#30648=CARTESIAN_POINT('Ctrl Pts',(2.995424253416,-1.,2.84246132984334));
#30649=CARTESIAN_POINT('Ctrl Pts',(2.99832751144566,-1.,2.84968053289104));
#30650=CARTESIAN_POINT('Ctrl Pts',(3.0012015079552,-1.,2.85692085715129));
#30651=CARTESIAN_POINT('Ctrl Pts',(3.00404638316245,-1.,2.86418200833065));
#30652=CARTESIAN_POINT('Ctrl Pts',(3.00686224485374,-1.,2.87146368430104));
#30653=CARTESIAN_POINT('Ctrl Pts',(3.0096491810855,-1.,2.87876560072799));
#30654=CARTESIAN_POINT('Ctrl Pts',(3.01240727309568,-1.,2.88608751706796));
#30655=CARTESIAN_POINT('Ctrl Pts',(3.01513660433291,-1.,2.8934292556764));
#30656=CARTESIAN_POINT('Ctrl Pts',(3.01783725123646,-1.,2.90079069102661));
#30657=CARTESIAN_POINT('Ctrl Pts',(3.01997487194926,-1.,2.90669553303902));
#30658=CARTESIAN_POINT('Ctrl Pts',(3.02156522743299,-1.,2.91113297349052));
#30659=CARTESIAN_POINT('Ctrl Pts',(3.02261975104912,-1.,2.91409518070707));
#30660=CARTESIAN_POINT('Ctrl Pts',(3.02314558451372,-1.,2.91557726271063));
#30661=CARTESIAN_POINT('',(2.91557726271063,-1.,3.02314558451372));
#30662=CARTESIAN_POINT('',(3.02314558451372,-1.,2.91557726271063));
#30663=CARTESIAN_POINT('',(2.50410331873176,-1.,2.79140942341258));
#30664=CARTESIAN_POINT('Ctrl Pts',(2.91557726271063,-1.,3.02314558451372));
#30665=CARTESIAN_POINT('Ctrl Pts',(2.91409518070399,-1.,3.02261975104593));
#30666=CARTESIAN_POINT('Ctrl Pts',(2.91113297348212,-1.,3.02156522742431));
#30667=CARTESIAN_POINT('Ctrl Pts',(2.90669553302526,-1.,3.01997487193503));
#30668=CARTESIAN_POINT('Ctrl Pts',(2.9007906910105,-1.,3.01783725121981));
#30669=CARTESIAN_POINT('Ctrl Pts',(2.89342925566321,-1.,3.01513660431928));
#30670=CARTESIAN_POINT('Ctrl Pts',(2.8860875170608,-1.,3.01240727308829));
#30671=CARTESIAN_POINT('Ctrl Pts',(2.87876560072727,-1.,3.00964918108476));
#30672=CARTESIAN_POINT('Ctrl Pts',(2.87146368430501,-1.,3.00686224485784));
#30673=CARTESIAN_POINT('Ctrl Pts',(2.86418200833667,-1.,3.00404638316867));
#30674=CARTESIAN_POINT('Ctrl Pts',(2.85692085715685,-1.,3.00120150796095));
#30675=CARTESIAN_POINT('Ctrl Pts',(2.84968053289451,-1.,2.99832751144925));
#30676=CARTESIAN_POINT('Ctrl Pts',(2.84246132984415,-1.,2.99542425341685));
#30677=CARTESIAN_POINT('Ctrl Pts',(2.83526351254248,-1.,2.9924915517034));
#30678=CARTESIAN_POINT('Ctrl Pts',(2.82808728190157,-1.,2.98952916401446));
#30679=CARTESIAN_POINT('Ctrl Pts',(2.82093279065457,-1.,2.9865368066918));
#30680=CARTESIAN_POINT('Ctrl Pts',(2.81380019196286,-1.,2.98351419779767));
#30681=CARTESIAN_POINT('Ctrl Pts',(2.80668968101106,-1.,2.98046109647241));
#30682=CARTESIAN_POINT('Ctrl Pts',(2.7996015327823,-1.,2.97737733718287));
#30683=CARTESIAN_POINT('Ctrl Pts',(2.79253615718248,-1.,2.9742628834758));
#30684=CARTESIAN_POINT('Ctrl Pts',(2.78549409123769,-1.,2.97111781461465));
#30685=CARTESIAN_POINT('Ctrl Pts',(2.7784758954285,-1.,2.96794221043036));
#30686=CARTESIAN_POINT('Ctrl Pts',(2.77148206836498,-1.,2.96473605585583));
#30687=CARTESIAN_POINT('Ctrl Pts',(2.76451296269557,-1.,2.96149914764818));
#30688=CARTESIAN_POINT('Ctrl Pts',(2.7575686788835,-1.,2.95823097665896));
#30689=CARTESIAN_POINT('Ctrl Pts',(2.75064903318947,-1.,2.95493069316161));
#30690=CARTESIAN_POINT('Ctrl Pts',(2.74375379492172,-1.,2.95159737214266));
#30691=CARTESIAN_POINT('Ctrl Pts',(2.73688288329808,-1.,2.94823023414364));
#30692=CARTESIAN_POINT('Ctrl Pts',(2.73003657371616,-1.,2.94482887675143));
#30693=CARTESIAN_POINT('Ctrl Pts',(2.72321571511337,-1.,2.94139351933897));
#30694=CARTESIAN_POINT('Ctrl Pts',(2.71642190053592,-1.,2.93792519474972));
#30695=CARTESIAN_POINT('Ctrl Pts',(2.70965695523787,-1.,2.93442516311179));
#30696=CARTESIAN_POINT('Ctrl Pts',(2.70292247416885,-1.,2.9308943823375));
#30697=CARTESIAN_POINT('Ctrl Pts',(2.69621932864301,-1.,2.92733294395267));
#30698=CARTESIAN_POINT('Ctrl Pts',(2.68954721165339,-1.,2.92373955325875));
#30699=CARTESIAN_POINT('Ctrl Pts',(2.68290409279688,-1.,2.92011090722152));
#30700=CARTESIAN_POINT('Ctrl Pts',(2.67628728855312,-1.,2.91644290704285));
#30701=CARTESIAN_POINT('Ctrl Pts',(2.66969458792631,-1.,2.91273193382882));
#30702=CARTESIAN_POINT('Ctrl Pts',(2.6631254261681,-1.,2.90897617968923));
#30703=CARTESIAN_POINT('Ctrl Pts',(2.65658188464282,-1.,2.90517678087461));
#30704=CARTESIAN_POINT('Ctrl Pts',(2.65007017365564,-1.,2.90133950224867));
#30705=CARTESIAN_POINT('Ctrl Pts',(2.64359851684131,-1.,2.89747231723345));
#30706=CARTESIAN_POINT('Ctrl Pts',(2.63717442263932,-1.,2.89358228854544));
#30707=CARTESIAN_POINT('Ctrl Pts',(2.63080195420767,-1.,2.88967244854239));
#30708=CARTESIAN_POINT('Ctrl Pts',(2.62447947640262,-1.,2.88573922195059));
#30709=CARTESIAN_POINT('Ctrl Pts',(2.61819596473108,-1.,2.88176821427525));
#30710=CARTESIAN_POINT('Ctrl Pts',(2.61193507170955,-1.,2.87773881947916));
#30711=CARTESIAN_POINT('Ctrl Pts',(2.60568177881303,-1.,2.87363176656501));
#30712=CARTESIAN_POINT('Ctrl Pts',(2.5994287522321,-1.,2.86943633170722));
#30713=CARTESIAN_POINT('Ctrl Pts',(2.59318160184908,-1.,2.86515629953513));
#30714=CARTESIAN_POINT('Ctrl Pts',(2.58696770643524,-1.,2.86081999003629));
#30715=CARTESIAN_POINT('Ctrl Pts',(2.58082875254357,-1.,2.85647171715092));
#30716=CARTESIAN_POINT('Ctrl Pts',(2.57480482727081,-1.,2.85215360144431));
#30717=CARTESIAN_POINT('Ctrl Pts',(2.56891984251721,-1.,2.84788893329067));
#30718=CARTESIAN_POINT('Ctrl Pts',(2.56316920798513,-1.,2.84366802680237));
#30719=CARTESIAN_POINT('Ctrl Pts',(2.55749952145241,-1.,2.83942515220782));
#30720=CARTESIAN_POINT('Ctrl Pts',(2.55182152807077,-1.,2.83505269592536));
#30721=CARTESIAN_POINT('Ctrl Pts',(2.54604736792655,-1.,2.83044254225917));
#30722=CARTESIAN_POINT('Ctrl Pts',(2.54012272520199,-1.,2.8255216764922));
#30723=CARTESIAN_POINT('Ctrl Pts',(2.53405679667412,-1.,2.82028550483689));
#30724=CARTESIAN_POINT('Ctrl Pts',(2.52796388055278,-1.,2.81484379048475));
#30725=CARTESIAN_POINT('Ctrl Pts',(2.52205778589653,-1.,2.80941521966941));
#30726=CARTESIAN_POINT('Ctrl Pts',(2.51660190465805,-1.,2.80427363984653));
#30727=CARTESIAN_POINT('Ctrl Pts',(2.51186983687818,-1.,2.79970585014168));
#30728=CARTESIAN_POINT('Ctrl Pts',(2.5081055597767,-1.,2.79596878057287));
#30729=CARTESIAN_POINT('Ctrl Pts',(2.50567182569081,-1.,2.79344192164147));
#30730=CARTESIAN_POINT('Ctrl Pts',(2.50455968395146,-1.,2.79217568804755));
#30731=CARTESIAN_POINT('Ctrl Pts',(2.50417932839313,-1.,2.79164172518905));
#30732=CARTESIAN_POINT('Ctrl Pts',(2.50410700351493,-1.,2.79145823440781));
#30733=CARTESIAN_POINT('Ctrl Pts',(2.50410331873176,-1.,2.79140942341258));
#30734=CARTESIAN_POINT('',(2.36531447826213,-1.,2.90994629141563));
#30735=CARTESIAN_POINT('Origin',(0.,-1.,0.));
#30736=CARTESIAN_POINT('',(2.52982887637028,-1.,3.35260583073571));
#30737=CARTESIAN_POINT('Ctrl Pts',(2.36531447826213,-1.,2.90994629141563));
#30738=CARTESIAN_POINT('Ctrl Pts',(2.3653621118858,-1.,2.90995756655559));
#30739=CARTESIAN_POINT('Ctrl Pts',(2.36553202948741,-1.,2.9100577052777));
#30740=CARTESIAN_POINT('Ctrl Pts',(2.36599991765853,-1.,2.91051690822262));
#30741=CARTESIAN_POINT('Ctrl Pts',(2.36707658451709,-1.,2.91181344022628));
#30742=CARTESIAN_POINT('Ctrl Pts',(2.36919161373074,-1.,2.91461249883016));
#30743=CARTESIAN_POINT('Ctrl Pts',(2.37229381109939,-1.,2.9189150379156));
#30744=CARTESIAN_POINT('Ctrl Pts',(2.37606510524271,-1.,2.92430340582912));
#30745=CARTESIAN_POINT('Ctrl Pts',(2.3802898958232,-1.,2.93049643640517));
#30746=CARTESIAN_POINT('Ctrl Pts',(2.38472771516476,-1.,2.93717903280599));
#30747=CARTESIAN_POINT('Ctrl Pts',(2.38914929090806,-1.,2.94404820669135));
#30748=CARTESIAN_POINT('Ctrl Pts',(2.39337207631613,-1.,2.95085857128372));
#30749=CARTESIAN_POINT('Ctrl Pts',(2.39730553974412,-1.,2.95748006482811));
#30750=CARTESIAN_POINT('Ctrl Pts',(2.40095565711535,-1.,2.96390432240181));
#30751=CARTESIAN_POINT('Ctrl Pts',(2.40438604734848,-1.,2.97019641312272));
#30752=CARTESIAN_POINT('Ctrl Pts',(2.40768975073691,-1.,2.97646002822395));
#30753=CARTESIAN_POINT('Ctrl Pts',(2.41095909342591,-1.,2.98280015815132));
#30754=CARTESIAN_POINT('Ctrl Pts',(2.4142506419963,-1.,2.98927983005851));
#30755=CARTESIAN_POINT('Ctrl Pts',(2.4175732450056,-1.,2.99590509293561));
#30756=CARTESIAN_POINT('Ctrl Pts',(2.42090763946812,-1.,3.00264868586038));
#30757=CARTESIAN_POINT('Ctrl Pts',(2.42421849439625,-1.,3.00946442616674));
#30758=CARTESIAN_POINT('Ctrl Pts',(2.4274685626416,-1.,3.01630420830494));
#30759=CARTESIAN_POINT('Ctrl Pts',(2.43063415586615,-1.,3.02313656035977));
#30760=CARTESIAN_POINT('Ctrl Pts',(2.43371241361462,-1.,3.02995534946946));
#30761=CARTESIAN_POINT('Ctrl Pts',(2.43671278042394,-1.,3.03676949672797));
#30762=CARTESIAN_POINT('Ctrl Pts',(2.43965194061849,-1.,3.04359685040545));
#30763=CARTESIAN_POINT('Ctrl Pts',(2.44254768923109,-1.,3.05045678021509));
#30764=CARTESIAN_POINT('Ctrl Pts',(2.44541251892568,-1.,3.05736242671521));
#30765=CARTESIAN_POINT('Ctrl Pts',(2.44824970516557,-1.,3.06431596421422));
#30766=CARTESIAN_POINT('Ctrl Pts',(2.45105688854432,-1.,3.0713129052131));
#30767=CARTESIAN_POINT('Ctrl Pts',(2.45382826787795,-1.,3.07834472886145));
#30768=CARTESIAN_POINT('Ctrl Pts',(2.45655725437037,-1.,3.08540206545313));
#30769=CARTESIAN_POINT('Ctrl Pts',(2.45923912563875,-1.,3.09247787931881));
#30770=CARTESIAN_POINT('Ctrl Pts',(2.4618730850188,-1.,3.09956993697048));
#30771=CARTESIAN_POINT('Ctrl Pts',(2.46446082979645,-1.,3.10667907901981));
#30772=CARTESIAN_POINT('Ctrl Pts',(2.46700558843507,-1.,3.11380805536124));
#30773=CARTESIAN_POINT('Ctrl Pts',(2.4695109894747,-1.,3.12096015766984));
#30774=CARTESIAN_POINT('Ctrl Pts',(2.47197997765868,-1.,3.12813790805948));
#30775=CARTESIAN_POINT('Ctrl Pts',(2.47441378371923,-1.,3.13534181229282));
#30776=CARTESIAN_POINT('Ctrl Pts',(2.47681245356095,-1.,3.14257099546531));
#30777=CARTESIAN_POINT('Ctrl Pts',(2.47917529057016,-1.,3.14982373241335));
#30778=CARTESIAN_POINT('Ctrl Pts',(2.48150133566568,-1.,3.15709802322735));
#30779=CARTESIAN_POINT('Ctrl Pts',(2.48378981792739,-1.,3.16439213290181));
#30780=CARTESIAN_POINT('Ctrl Pts',(2.48604065348619,-1.,3.17170518863357));
#30781=CARTESIAN_POINT('Ctrl Pts',(2.48825428288242,-1.,3.17903698136679));
#30782=CARTESIAN_POINT('Ctrl Pts',(2.49043146334095,-1.,3.18638771282315));
#30783=CARTESIAN_POINT('Ctrl Pts',(2.4925730723986,-1.,3.19375775555814));
#30784=CARTESIAN_POINT('Ctrl Pts',(2.49467992057726,-1.,3.20114742397549));
#30785=CARTESIAN_POINT('Ctrl Pts',(2.49675252647298,-1.,3.2085566984974));
#30786=CARTESIAN_POINT('Ctrl Pts',(2.49879114599293,-1.,3.21598526261157));
#30787=CARTESIAN_POINT('Ctrl Pts',(2.5007958720187,-1.,3.22343262620387));
#30788=CARTESIAN_POINT('Ctrl Pts',(2.50276671338074,-1.,3.23089822320596));
#30789=CARTESIAN_POINT('Ctrl Pts',(2.50470367580078,-1.,3.23838151080383));
#30790=CARTESIAN_POINT('Ctrl Pts',(2.50660685940645,-1.,3.24588208984042));
#30791=CARTESIAN_POINT('Ctrl Pts',(2.50847647070936,-1.,3.25339971461265));
#30792=CARTESIAN_POINT('Ctrl Pts',(2.51031277813697,-1.,3.26093423001716));
#30793=CARTESIAN_POINT('Ctrl Pts',(2.51211608411539,-1.,3.26848552888271));
#30794=CARTESIAN_POINT('Ctrl Pts',(2.51388669270329,-1.,3.27605350473048));
#30795=CARTESIAN_POINT('Ctrl Pts',(2.51562487464214,-1.,3.28363799702583));
#30796=CARTESIAN_POINT('Ctrl Pts',(2.51733085123316,-1.,3.2912387729863));
#30797=CARTESIAN_POINT('Ctrl Pts',(2.51900480700548,-1.,3.29885556387661));
#30798=CARTESIAN_POINT('Ctrl Pts',(2.52064689568167,-1.,3.30648808814986));
#30799=CARTESIAN_POINT('Ctrl Pts',(2.52225724871375,-1.,3.31413607874727));
#30800=CARTESIAN_POINT('Ctrl Pts',(2.52383598396878,-1.,3.32179931079521));
#30801=CARTESIAN_POINT('Ctrl Pts',(2.52538321165774,-1.,3.32947762189049));
#30802=CARTESIAN_POINT('Ctrl Pts',(2.52689902691551,-1.,3.33717090000955));
#30803=CARTESIAN_POINT('Ctrl Pts',(2.52808660916879,-1.,3.34333744117093));
#30804=CARTESIAN_POINT('Ctrl Pts',(2.5289632161143,-1.,3.34796903577628));
#30805=CARTESIAN_POINT('Ctrl Pts',(2.52954136549357,-1.,3.35105973714426));
#30806=CARTESIAN_POINT('Ctrl Pts',(2.52982887637028,-1.,3.35260583073571));
#30807=CARTESIAN_POINT('',(2.40675750623143,-1.,3.44202241512147));
#30808=CARTESIAN_POINT('',(2.52982887637028,-1.,3.35260583073571));
#30809=CARTESIAN_POINT('',(2.03660101169714,-1.,3.14877060440328));
#30810=CARTESIAN_POINT('Ctrl Pts',(2.40675750623143,-1.,3.44202241512147));
#30811=CARTESIAN_POINT('Ctrl Pts',(2.4053759295909,-1.,3.44127120683039));
#30812=CARTESIAN_POINT('Ctrl Pts',(2.40261515589405,-1.,3.43976627484234));
#30813=CARTESIAN_POINT('Ctrl Pts',(2.39848113410292,-1.,3.43750133064416));
#30814=CARTESIAN_POINT('Ctrl Pts',(2.39298338804493,-1.,3.4344663067854));
#30815=CARTESIAN_POINT('Ctrl Pts',(2.38613505843552,-1.,3.4306473271292));
#30816=CARTESIAN_POINT('Ctrl Pts',(2.37931067028926,-1.,3.42680309754399));
#30817=CARTESIAN_POINT('Ctrl Pts',(2.37251035954292,-1.,3.42293356216511));
#30818=CARTESIAN_POINT('Ctrl Pts',(2.36573431470642,-1.,3.41903866635852));
#30819=CARTESIAN_POINT('Ctrl Pts',(2.35898278606946,-1.,3.41511836751469));
#30820=CARTESIAN_POINT('Ctrl Pts',(2.35225606824109,-1.,3.41117262314119));
#30821=CARTESIAN_POINT('Ctrl Pts',(2.34555447649188,-1.,3.40720137404297));
#30822=CARTESIAN_POINT('Ctrl Pts',(2.33887832342782,-1.,3.40320452776743));
#30823=CARTESIAN_POINT('Ctrl Pts',(2.33222789882489,-1.,3.39918194577956));
#30824=CARTESIAN_POINT('Ctrl Pts',(2.3256034390248,-1.,3.39513342019756));
#30825=CARTESIAN_POINT('Ctrl Pts',(2.31900513925424,-1.,3.39105869474822));
#30826=CARTESIAN_POINT('Ctrl Pts',(2.31243319489367,-1.,3.38695751492462));
#30827=CARTESIAN_POINT('Ctrl Pts',(2.30588783640343,-1.,3.3828296733661));
#30828=CARTESIAN_POINT('Ctrl Pts',(2.29936936127624,-1.,3.37867504959433));
#30829=CARTESIAN_POINT('Ctrl Pts',(2.29287818007393,-1.,3.37449367172826));
#30830=CARTESIAN_POINT('Ctrl Pts',(2.28641481081137,-1.,3.37028570206488));
#30831=CARTESIAN_POINT('Ctrl Pts',(2.27997979458037,-1.,3.36605130713076));
#30832=CARTESIAN_POINT('Ctrl Pts',(2.2735736262093,-1.,3.36179055004409));
#30833=CARTESIAN_POINT('Ctrl Pts',(2.26719668579909,-1.,3.35750328523061));
#30834=CARTESIAN_POINT('Ctrl Pts',(2.26084915222449,-1.,3.35318902552626));
#30835=CARTESIAN_POINT('Ctrl Pts',(2.25453097693483,-1.,3.34884690292285));
#30836=CARTESIAN_POINT('Ctrl Pts',(2.24824207678256,-1.,3.34447596770723));
#30837=CARTESIAN_POINT('Ctrl Pts',(2.24198249391422,-1.,3.34007543738025));
#30838=CARTESIAN_POINT('Ctrl Pts',(2.23575256328812,-1.,3.33564495756482));
#30839=CARTESIAN_POINT('Ctrl Pts',(2.22955308907233,-1.,3.33118487773611));
#30840=CARTESIAN_POINT('Ctrl Pts',(2.22338548312772,-1.,3.3266964672289));
#30841=CARTESIAN_POINT('Ctrl Pts',(2.21725135110898,-1.,3.32218125618968));
#30842=CARTESIAN_POINT('Ctrl Pts',(2.21115211847875,-1.,3.31764044024235));
#30843=CARTESIAN_POINT('Ctrl Pts',(2.20508863150607,-1.,3.31307424608949));
#30844=CARTESIAN_POINT('Ctrl Pts',(2.19906078949922,-1.,3.30848134694595));
#30845=CARTESIAN_POINT('Ctrl Pts',(2.19306710376111,-1.,3.30385816281831));
#30846=CARTESIAN_POINT('Ctrl Pts',(2.18710556500327,-1.,3.29920022557639));
#30847=CARTESIAN_POINT('Ctrl Pts',(2.18117455557065,-1.,3.2945036150049));
#30848=CARTESIAN_POINT('Ctrl Pts',(2.17527380048423,-1.,3.28976645712568));
#30849=CARTESIAN_POINT('Ctrl Pts',(2.16940517773455,-1.,3.28499019979724));
#30850=CARTESIAN_POINT('Ctrl Pts',(2.16357391934425,-1.,3.280181508414));
#30851=CARTESIAN_POINT('Ctrl Pts',(2.15778690038347,-1.,3.27534954469187));
#30852=CARTESIAN_POINT('Ctrl Pts',(2.15205043199808,-1.,3.27050245897228));
#30853=CARTESIAN_POINT('Ctrl Pts',(2.1463680529566,-1.,3.26564388189759));
#30854=CARTESIAN_POINT('Ctrl Pts',(2.14073870754264,-1.,3.26077002641879));
#30855=CARTESIAN_POINT('Ctrl Pts',(2.13515375878803,-1.,3.25586495065054));
#30856=CARTESIAN_POINT('Ctrl Pts',(2.12960028396832,-1.,3.25090574494028));
#30857=CARTESIAN_POINT('Ctrl Pts',(2.12406646410962,-1.,3.24587102613376));
#30858=CARTESIAN_POINT('Ctrl Pts',(2.11854673326979,-1.,3.24074905517293));
#30859=CARTESIAN_POINT('Ctrl Pts',(2.11304604021773,-1.,3.23554444767099));
#30860=CARTESIAN_POINT('Ctrl Pts',(2.10758699642451,-1.,3.23028945793289));
#30861=CARTESIAN_POINT('Ctrl Pts',(2.10220384298492,-1.,3.22503437553434));
#30862=CARTESIAN_POINT('Ctrl Pts',(2.09692958434895,-1.,3.21982707347009));
#30863=CARTESIAN_POINT('Ctrl Pts',(2.09178419460443,-1.,3.21469429601654));
#30864=CARTESIAN_POINT('Ctrl Pts',(2.08676465517455,-1.,3.20962575845463));
#30865=CARTESIAN_POINT('Ctrl Pts',(2.08182850370878,-1.,3.2045481863073));
#30866=CARTESIAN_POINT('Ctrl Pts',(2.07690441870722,-1.,3.19934132836019));
#30867=CARTESIAN_POINT('Ctrl Pts',(2.07192253497857,-1.,3.19388465568252));
#30868=CARTESIAN_POINT('Ctrl Pts',(2.06684062744112,-1.,3.18809755562368));
#30869=CARTESIAN_POINT('Ctrl Pts',(2.06166849827101,-1.,3.18197692964614));
#30870=CARTESIAN_POINT('Ctrl Pts',(2.05650186773132,-1.,3.17564906975371));
#30871=CARTESIAN_POINT('Ctrl Pts',(2.05151770247233,-1.,3.16936341689527));
#30872=CARTESIAN_POINT('Ctrl Pts',(2.04693331247446,-1.,3.16343165058912));
#30873=CARTESIAN_POINT('Ctrl Pts',(2.04297406404027,-1.,3.15817983946367));
#30874=CARTESIAN_POINT('Ctrl Pts',(2.03984073791519,-1.,3.15389991674792));
#30875=CARTESIAN_POINT('Ctrl Pts',(2.03783225495961,-1.,3.15102344775328));
#30876=CARTESIAN_POINT('Ctrl Pts',(2.03693188810544,-1.,3.14959882629805));
#30877=CARTESIAN_POINT('Ctrl Pts',(2.03663974554932,-1.,3.1490119366901));
#30878=CARTESIAN_POINT('Ctrl Pts',(2.03659701539259,-1.,3.14881939088124));
#30879=CARTESIAN_POINT('Ctrl Pts',(2.03660101169714,-1.,3.14877060440328));
#30880=CARTESIAN_POINT('',(1.88097764062697,-1.,3.24413672884812));
#30881=CARTESIAN_POINT('Origin',(0.,-1.,0.));
#30882=CARTESIAN_POINT('',(1.97421938526992,-1.,3.70708211654725));
#30883=CARTESIAN_POINT('Ctrl Pts',(1.88097764062697,-1.,3.24413672884812));
#30884=CARTESIAN_POINT('Ctrl Pts',(1.8810229239812,-1.,3.24415531671284));
#30885=CARTESIAN_POINT('Ctrl Pts',(1.88117508446775,-1.,3.24428080353022));
#30886=CARTESIAN_POINT('Ctrl Pts',(1.88156537699203,-1.,3.24480754676064));
#30887=CARTESIAN_POINT('Ctrl Pts',(1.88242596600454,-1.,3.2462565441079));
#30888=CARTESIAN_POINT('Ctrl Pts',(1.88407708646357,-1.,3.24935200511918));
#30889=CARTESIAN_POINT('Ctrl Pts',(1.88646802523466,-1.,3.25408686339463));
#30890=CARTESIAN_POINT('Ctrl Pts',(1.88934996203698,-1.,3.25999885193947));
#30891=CARTESIAN_POINT('Ctrl Pts',(1.89255393500965,-1.,3.26677653888676));
#30892=CARTESIAN_POINT('Ctrl Pts',(1.89589172903793,-1.,3.27407108933139));
#30893=CARTESIAN_POINT('Ctrl Pts',(1.89918429230462,-1.,3.28154737912352));
#30894=CARTESIAN_POINT('Ctrl Pts',(1.90228971247527,-1.,3.2889344860029));
#30895=CARTESIAN_POINT('Ctrl Pts',(1.90513891864087,-1.,3.29608978722113));
#30896=CARTESIAN_POINT('Ctrl Pts',(1.90773912171341,-1.,3.30300595568195));
#30897=CARTESIAN_POINT('Ctrl Pts',(1.91014297830446,-1.,3.30975721158596));
#30898=CARTESIAN_POINT('Ctrl Pts',(1.91242616234442,-1.,3.31646052426364));
#30899=CARTESIAN_POINT('Ctrl Pts',(1.91466343916627,-1.,3.32323403454535));
#30900=CARTESIAN_POINT('Ctrl Pts',(1.91690081930331,-1.,3.33014884257873));
#30901=CARTESIAN_POINT('Ctrl Pts',(1.9191460961021,-1.,3.33721230710012));
#30902=CARTESIAN_POINT('Ctrl Pts',(1.92138450828404,-1.,3.34439448941961));
#30903=CARTESIAN_POINT('Ctrl Pts',(1.92358838440528,-1.,3.35164424847223));
#30904=CARTESIAN_POINT('Ctrl Pts',(1.92572846125756,-1.,3.35890824422965));
#30905=CARTESIAN_POINT('Ctrl Pts',(1.92778626543786,-1.,3.36615168657567));
#30906=CARTESIAN_POINT('Ctrl Pts',(1.92975993109877,-1.,3.37336807068043));
#30907=CARTESIAN_POINT('Ctrl Pts',(1.93165739093276,-1.,3.3805676852555));
#30908=CARTESIAN_POINT('Ctrl Pts',(1.93349233176788,-1.,3.38777076883256));
#30909=CARTESIAN_POINT('Ctrl Pts',(1.93527929945985,-1.,3.39499923640795));
#30910=CARTESIAN_POINT('Ctrl Pts',(1.93702857723098,-1.,3.40226802104109));
#30911=CARTESIAN_POINT('Ctrl Pts',(1.93874306008143,-1.,3.40957978266642));
#30912=CARTESIAN_POINT('Ctrl Pts',(1.94042111965246,-1.,3.41692971994096));
#30913=CARTESIAN_POINT('Ctrl Pts',(1.94205835913696,-1.,3.42430850941503));
#30914=CARTESIAN_POINT('Ctrl Pts',(1.94364973660284,-1.,3.43170586602434));
#30915=CARTESIAN_POINT('Ctrl Pts',(1.94519168842879,-1.,3.43911410197687));
#30916=CARTESIAN_POINT('Ctrl Pts',(1.94668377715329,-1.,3.44653088665681));
#30917=CARTESIAN_POINT('Ctrl Pts',(1.94812754766524,-1.,3.45395731584051));
#30918=CARTESIAN_POINT('Ctrl Pts',(1.94952575850197,-1.,3.46139661060962));
#30919=CARTESIAN_POINT('Ctrl Pts',(1.95088147859876,-1.,3.46885258974191));
#30920=CARTESIAN_POINT('Ctrl Pts',(1.95219722189876,-1.,3.47632820495921));
#30921=CARTESIAN_POINT('Ctrl Pts',(1.95347412486308,-1.,3.48382414832634));
#30922=CARTESIAN_POINT('Ctrl Pts',(1.95471236969643,-1.,3.49133956289133));
#30923=CARTESIAN_POINT('Ctrl Pts',(1.95591153823661,-1.,3.49887263575583));
#30924=CARTESIAN_POINT('Ctrl Pts',(1.95707099606511,-1.,3.50642124159909));
#30925=CARTESIAN_POINT('Ctrl Pts',(1.95819025316779,-1.,3.51398354617794));
#30926=CARTESIAN_POINT('Ctrl Pts',(1.95926936324461,-1.,3.52155867431486));
#30927=CARTESIAN_POINT('Ctrl Pts',(1.96030879411566,-1.,3.52914648844351));
#30928=CARTESIAN_POINT('Ctrl Pts',(1.96130926212689,-1.,3.53674730625813));
#30929=CARTESIAN_POINT('Ctrl Pts',(1.96227157573067,-1.,3.54436163300443));
#30930=CARTESIAN_POINT('Ctrl Pts',(1.96319648628644,-1.,3.55198990600886));
#30931=CARTESIAN_POINT('Ctrl Pts',(1.96408450906812,-1.,3.55963218706096));
#30932=CARTESIAN_POINT('Ctrl Pts',(1.96493594634567,-1.,3.56728820357791));
#30933=CARTESIAN_POINT('Ctrl Pts',(1.96575096652789,-1.,3.57495748600959));
#30934=CARTESIAN_POINT('Ctrl Pts',(1.96652966688911,-1.,3.58263947663829));
#30935=CARTESIAN_POINT('Ctrl Pts',(1.96727213799544,-1.,3.59033364022801));
#30936=CARTESIAN_POINT('Ctrl Pts',(1.96797854118369,-1.,3.59803959819938));
#30937=CARTESIAN_POINT('Ctrl Pts',(1.9686491188594,-1.,3.60575714017989));
#30938=CARTESIAN_POINT('Ctrl Pts',(1.96928416040877,-1.,3.61348615496704));
#30939=CARTESIAN_POINT('Ctrl Pts',(1.96988398129978,-1.,3.62122658401893));
#30940=CARTESIAN_POINT('Ctrl Pts',(1.97044889850463,-1.,3.62897836973293));
#30941=CARTESIAN_POINT('Ctrl Pts',(1.97097920454464,-1.,3.63674139590412));
#30942=CARTESIAN_POINT('Ctrl Pts',(1.97147515441164,-1.,3.64451546723514));
#30943=CARTESIAN_POINT('Ctrl Pts',(1.97193697240239,-1.,3.652300347166));
#30944=CARTESIAN_POINT('Ctrl Pts',(1.9723648543905,-1.,3.6600957816636));
#30945=CARTESIAN_POINT('Ctrl Pts',(1.97275897198678,-1.,3.66790152752075));
#30946=CARTESIAN_POINT('Ctrl Pts',(1.97311947678516,-1.,3.67571738107084));
#30947=CARTESIAN_POINT('Ctrl Pts',(1.97344650304519,-1.,3.68354319915092));
#30948=CARTESIAN_POINT('Ctrl Pts',(1.97374016225483,-1.,3.69137888599902));
#30949=CARTESIAN_POINT('Ctrl Pts',(1.97394846383216,-1.,3.6976552856004));
#30950=CARTESIAN_POINT('Ctrl Pts',(1.97408973726715,-1.,3.70236698912904));
#30951=CARTESIAN_POINT('Ctrl Pts',(1.97417727645308,-1.,3.70551008132332));
#30952=CARTESIAN_POINT('Ctrl Pts',(1.97421938526992,-1.,3.70708211654725));
#30953=CARTESIAN_POINT('',(1.8386753923786,-1.,3.77614523045147));
#30954=CARTESIAN_POINT('',(1.97421938526992,-1.,3.70708211654725));
#30955=CARTESIAN_POINT('',(1.5189508286633,-1.,3.42859860294306));
#30956=CARTESIAN_POINT('Ctrl Pts',(1.8386753923786,-1.,3.77614523045147));
#30957=CARTESIAN_POINT('Ctrl Pts',(1.83742834010626,-1.,3.77518714457833));
#30958=CARTESIAN_POINT('Ctrl Pts',(1.83493697934534,-1.,3.77326886064398));
#30959=CARTESIAN_POINT('Ctrl Pts',(1.83120816955645,-1.,3.77038509817999));
#30960=CARTESIAN_POINT('Ctrl Pts',(1.82625289220915,-1.,3.76652740353775));
#30961=CARTESIAN_POINT('Ctrl Pts',(1.82008629694091,-1.,3.76168412707948));
#30962=CARTESIAN_POINT('Ctrl Pts',(1.8139472983358,-1.,3.75681965683071));
#30963=CARTESIAN_POINT('Ctrl Pts',(1.80783603939617,-1.,3.75193395887977));
#30964=CARTESIAN_POINT('Ctrl Pts',(1.8017527148577,-1.,3.74702700875467));
#30965=CARTESIAN_POINT('Ctrl Pts',(1.79569757859422,-1.,3.74209880352445));
#30966=CARTESIAN_POINT('Ctrl Pts',(1.78967092823491,-1.,3.73714934730681));
#30967=CARTESIAN_POINT('Ctrl Pts',(1.78367308442901,-1.,3.7321786309547));
#30968=CARTESIAN_POINT('Ctrl Pts',(1.77770437039658,-1.,3.72718661205609));
#30969=CARTESIAN_POINT('Ctrl Pts',(1.77176509401761,-1.,3.72217319911254));
#30970=CARTESIAN_POINT('Ctrl Pts',(1.76585552124394,-1.,3.71713822377359));
#30971=CARTESIAN_POINT('Ctrl Pts',(1.75997588498865,-1.,3.71208146346136));
#30972=CARTESIAN_POINT('Ctrl Pts',(1.75412641804042,-1.,3.70700269736659));
#30973=CARTESIAN_POINT('Ctrl Pts',(1.74830738046057,-1.,3.7019017567335));
#30974=CARTESIAN_POINT('Ctrl Pts',(1.74251908492617,-1.,3.69677856910517));
#30975=CARTESIAN_POINT('Ctrl Pts',(1.73676193254557,-1.,3.69163322648036));
#30976=CARTESIAN_POINT('Ctrl Pts',(1.73103640956717,-1.,3.68646597019332));
#30977=CARTESIAN_POINT('Ctrl Pts',(1.72534302437056,-1.,3.68127704936579));
#30978=CARTESIAN_POINT('Ctrl Pts',(1.71968225581808,-1.,3.67606660374709));
#30979=CARTESIAN_POINT('Ctrl Pts',(1.71405450210383,-1.,3.67083454901611));
#30980=CARTESIAN_POINT('Ctrl Pts',(1.70846001610956,-1.,3.66558043198876));
#30981=CARTESIAN_POINT('Ctrl Pts',(1.70289888566873,-1.,3.66030338774847));
#30982=CARTESIAN_POINT('Ctrl Pts',(1.69737117722534,-1.,3.65500246526749));
#30983=CARTESIAN_POINT('Ctrl Pts',(1.69187705481689,-1.,3.64967689827371));
#30984=CARTESIAN_POINT('Ctrl Pts',(1.68641690471457,-1.,3.64432638915203));
#30985=CARTESIAN_POINT('Ctrl Pts',(1.68099146651586,-1.,3.63895140887462));
#30986=CARTESIAN_POINT('Ctrl Pts',(1.67560193613156,-1.,3.63355343201232));
#30987=CARTESIAN_POINT('Ctrl Pts',(1.67024966008044,-1.,3.62813422105271));
#30988=CARTESIAN_POINT('Ctrl Pts',(1.66493585923855,-1.,3.62269517989109));
#30989=CARTESIAN_POINT('Ctrl Pts',(1.65966133399186,-1.,3.61723666482456));
#30990=CARTESIAN_POINT('Ctrl Pts',(1.65442619244325,-1.,3.61175734965127));
#30991=CARTESIAN_POINT('Ctrl Pts',(1.64922952425832,-1.,3.60625346556992));
#30992=CARTESIAN_POINT('Ctrl Pts',(1.64407004385582,-1.,3.60072028513845));
#30993=CARTESIAN_POINT('Ctrl Pts',(1.63894676675352,-1.,3.59515368334893));
#30994=CARTESIAN_POINT('Ctrl Pts',(1.6338597145126,-1.,3.58955176627879));
#30995=CARTESIAN_POINT('Ctrl Pts',(1.62881051550745,-1.,3.58391625774343));
#30996=CARTESIAN_POINT('Ctrl Pts',(1.62380329464844,-1.,3.5782545595439));
#30997=CARTESIAN_POINT('Ctrl Pts',(1.61884340915404,-1.,3.57257679609806));
#30998=CARTESIAN_POINT('Ctrl Pts',(1.61393581747514,-1.,3.56689200468387));
#30999=CARTESIAN_POINT('Ctrl Pts',(1.60908344685457,-1.,3.5612043248298));
#31000=CARTESIAN_POINT('Ctrl Pts',(1.60428584699853,-1.,3.55550985096129));
#31001=CARTESIAN_POINT('Ctrl Pts',(1.59953698113457,-1.,3.54979148634454));
#31002=CARTESIAN_POINT('Ctrl Pts',(1.59482766949766,-1.,3.54402458182337));
#31003=CARTESIAN_POINT('Ctrl Pts',(1.59014958368739,-1.,3.53818616861077));
#31004=CARTESIAN_POINT('Ctrl Pts',(1.58549906268088,-1.,3.5322637814708));
#31005=CARTESIAN_POINT('Ctrl Pts',(1.58088027227848,-1.,3.52626275334881));
#31006=CARTESIAN_POINT('Ctrl Pts',(1.57631049988158,-1.,3.52021847865912));
#31007=CARTESIAN_POINT('Ctrl Pts',(1.57181569799743,-1.,3.51418598431665));
#31008=CARTESIAN_POINT('Ctrl Pts',(1.56742097575012,-1.,3.50821771695363));
#31009=CARTESIAN_POINT('Ctrl Pts',(1.56314187758675,-1.,3.50234321621578));
#31010=CARTESIAN_POINT('Ctrl Pts',(1.55897703097874,-1.,3.49655185179655));
#31011=CARTESIAN_POINT('Ctrl Pts',(1.55489595901116,-1.,3.4907646087742));
#31012=CARTESIAN_POINT('Ctrl Pts',(1.55084702970452,-1.,3.48485155928567));
#31013=CARTESIAN_POINT('Ctrl Pts',(1.54678009290276,-1.,3.47868272898751));
#31014=CARTESIAN_POINT('Ctrl Pts',(1.54266605398187,-1.,3.47217189224653));
#31015=CARTESIAN_POINT('Ctrl Pts',(1.53851507915502,-1.,3.46531752207153));
#31016=CARTESIAN_POINT('Ctrl Pts',(1.53440195378792,-1.,3.45825932955032));
#31017=CARTESIAN_POINT('Ctrl Pts',(1.53046244461635,-1.,3.45127136828305));
#31018=CARTESIAN_POINT('Ctrl Pts',(1.52686242875556,-1.,3.44469547526647));
#31019=CARTESIAN_POINT('Ctrl Pts',(1.5237734895035,-1.,3.4388889597401));
#31020=CARTESIAN_POINT('Ctrl Pts',(1.52134826724292,-1.,3.43417156977893));
#31021=CARTESIAN_POINT('Ctrl Pts',(1.5198144909338,-1.,3.43101631893414));
#31022=CARTESIAN_POINT('Ctrl Pts',(1.51914806898491,-1.,3.42946838852587));
#31023=CARTESIAN_POINT('Ctrl Pts',(1.5189513329503,-1.,3.42884302333841));
#31024=CARTESIAN_POINT('Ctrl Pts',(1.51893924967331,-1.,3.42864616361875));
#31025=CARTESIAN_POINT('Ctrl Pts',(1.5189508286633,-1.,3.42859860294306));
#31026=CARTESIAN_POINT('',(1.35032489087269,-1.,3.49844575334386));
#31027=CARTESIAN_POINT('Origin',(0.,-1.,0.));
#31028=CARTESIAN_POINT('',(1.36999806084572,-1.,3.97027773754922));
#31029=CARTESIAN_POINT('Ctrl Pts',(1.35032489087269,-1.,3.49844575334386));
#31030=CARTESIAN_POINT('Ctrl Pts',(1.35036670893102,-1.,3.49847119623841));
#31031=CARTESIAN_POINT('Ctrl Pts',(1.35049736560633,-1.,3.49861894124915));
#31032=CARTESIAN_POINT('Ctrl Pts',(1.35080045218652,-1.,3.49920025459856));
#31033=CARTESIAN_POINT('Ctrl Pts',(1.35142377279535,-1.,3.5007660381658));
#31034=CARTESIAN_POINT('Ctrl Pts',(1.3525703284343,-1.,3.50408168106113));
#31035=CARTESIAN_POINT('Ctrl Pts',(1.35419113576022,-1.,3.50913227060177));
#31036=CARTESIAN_POINT('Ctrl Pts',(1.35611275237288,-1.,3.51542230699919));
#31037=CARTESIAN_POINT('Ctrl Pts',(1.35821701528975,-1.,3.52261776117121));
#31038=CARTESIAN_POINT('Ctrl Pts',(1.36037259643827,-1.,3.53034464961849));
#31039=CARTESIAN_POINT('Ctrl Pts',(1.36245507339334,-1.,3.53824396425032));
#31040=CARTESIAN_POINT('Ctrl Pts',(1.36436666257567,-1.,3.54602591832893));
#31041=CARTESIAN_POINT('Ctrl Pts',(1.36606145456711,-1.,3.55353883995793));
#31042=CARTESIAN_POINT('Ctrl Pts',(1.36754771771174,-1.,3.56077662028492));
#31043=CARTESIAN_POINT('Ctrl Pts',(1.36886584973349,-1.,3.56782080304554));
#31044=CARTESIAN_POINT('Ctrl Pts',(1.37007229485646,-1.,3.57479875549453));
#31045=CARTESIAN_POINT('Ctrl Pts',(1.37122241663073,-1.,3.58183885982745));
#31046=CARTESIAN_POINT('Ctrl Pts',(1.37235053661,-1.,3.5890185384643));
#31047=CARTESIAN_POINT('Ctrl Pts',(1.37346320103184,-1.,3.59634627869117));
#31048=CARTESIAN_POINT('Ctrl Pts',(1.37455051379642,-1.,3.60379020124038));
#31049=CARTESIAN_POINT('Ctrl Pts',(1.37559314436641,-1.,3.61129546591082));
#31050=CARTESIAN_POINT('Ctrl Pts',(1.37657053403102,-1.,3.61880481160408));
#31051=CARTESIAN_POINT('Ctrl Pts',(1.37746987919868,-1.,3.62628098665112));
#31052=CARTESIAN_POINT('Ctrl Pts',(1.37829035457324,-1.,3.63371727442448));
#31053=CARTESIAN_POINT('Ctrl Pts',(1.37903818567347,-1.,3.64112507791112));
#31054=CARTESIAN_POINT('Ctrl Pts',(1.37972372481598,-1.,3.64852652756444));
#31055=CARTESIAN_POINT('Ctrl Pts',(1.38035791051215,-1.,3.65594554404396));
#31056=CARTESIAN_POINT('Ctrl Pts',(1.38094856333558,-1.,3.66339848520874));
#31057=CARTESIAN_POINT('Ctrl Pts',(1.38149812653876,-1.,3.67088843112282));
#31058=CARTESIAN_POINT('Ctrl Pts',(1.38200574290626,-1.,3.6784103848243));
#31059=CARTESIAN_POINT('Ctrl Pts',(1.38246852827185,-1.,3.68595444983844));
#31060=CARTESIAN_POINT('Ctrl Pts',(1.38288311171649,-1.,3.69350967899523));
#31061=CARTESIAN_POINT('Ctrl Pts',(1.38324717612862,-1.,3.70106792167894));
#31062=CARTESIAN_POINT('Ctrl Pts',(1.38356065402122,-1.,3.70862680753343));
#31063=CARTESIAN_POINT('Ctrl Pts',(1.38382489984585,-1.,3.7161876605181));
#31064=CARTESIAN_POINT('Ctrl Pts',(1.3840421342895,-1.,3.72375409358805));
#31065=CARTESIAN_POINT('Ctrl Pts',(1.38421479111531,-1.,3.73133035859283));
#31066=CARTESIAN_POINT('Ctrl Pts',(1.38434489156456,-1.,3.73891976418099));
#31067=CARTESIAN_POINT('Ctrl Pts',(1.38443344984389,-1.,3.7465231716786));
#31068=CARTESIAN_POINT('Ctrl Pts',(1.38448077997155,-1.,3.75413976318727));
#31069=CARTESIAN_POINT('Ctrl Pts',(1.38448675253343,-1.,3.76176768271347));
#31070=CARTESIAN_POINT('Ctrl Pts',(1.38445107339517,-1.,3.76940473185775));
#31071=CARTESIAN_POINT('Ctrl Pts',(1.38437354551435,-1.,3.77704902230441));
#31072=CARTESIAN_POINT('Ctrl Pts',(1.38425435883773,-1.,3.78469969805134));
#31073=CARTESIAN_POINT('Ctrl Pts',(1.38409399694588,-1.,3.79235669640907));
#31074=CARTESIAN_POINT('Ctrl Pts',(1.38389311766701,-1.,3.80002044322169));
#31075=CARTESIAN_POINT('Ctrl Pts',(1.38365244046226,-1.,3.80769156398429));
#31076=CARTESIAN_POINT('Ctrl Pts',(1.38337263902766,-1.,3.81537060817765));
#31077=CARTESIAN_POINT('Ctrl Pts',(1.38305421262724,-1.,3.82305771743715));
#31078=CARTESIAN_POINT('Ctrl Pts',(1.38269750245086,-1.,3.83075266982138));
#31079=CARTESIAN_POINT('Ctrl Pts',(1.38230274828774,-1.,3.83845502790609));
#31080=CARTESIAN_POINT('Ctrl Pts',(1.38187013346089,-1.,3.84616425605705));
#31081=CARTESIAN_POINT('Ctrl Pts',(1.38139983115075,-1.,3.85387983979557));
#31082=CARTESIAN_POINT('Ctrl Pts',(1.38089205993067,-1.,3.86160143044187));
#31083=CARTESIAN_POINT('Ctrl Pts',(1.38034709213129,-1.,3.86932885813403));
#31084=CARTESIAN_POINT('Ctrl Pts',(1.37976523097187,-1.,3.87706205830865));
#31085=CARTESIAN_POINT('Ctrl Pts',(1.37914679719446,-1.,3.88480102249461));
#31086=CARTESIAN_POINT('Ctrl Pts',(1.37849211287981,-1.,3.89254574338385));
#31087=CARTESIAN_POINT('Ctrl Pts',(1.3778014851263,-1.,3.90029615196255));
#31088=CARTESIAN_POINT('Ctrl Pts',(1.3770751963376,-1.,3.90805209522729));
#31089=CARTESIAN_POINT('Ctrl Pts',(1.37631350505516,-1.,3.91581337461825));
#31090=CARTESIAN_POINT('Ctrl Pts',(1.37551664448057,-1.,3.92357976987132));
#31091=CARTESIAN_POINT('Ctrl Pts',(1.37468482215784,-1.,3.93135106761941));
#31092=CARTESIAN_POINT('Ctrl Pts',(1.37381821967499,-1.,3.93912709041791));
#31093=CARTESIAN_POINT('Ctrl Pts',(1.37291699203423,-1.,3.94690771786926));
#31094=CARTESIAN_POINT('Ctrl Pts',(1.37198126433139,-1.,3.95469287283105));
#31095=CARTESIAN_POINT('Ctrl Pts',(1.37120515615663,-1.,3.96092458508407));
#31096=CARTESIAN_POINT('Ctrl Pts',(1.37060761746027,-1.,3.96560037975788));
#31097=CARTESIAN_POINT('Ctrl Pts',(1.37020239094758,-1.,3.9687184694173));
#31098=CARTESIAN_POINT('Ctrl Pts',(1.36999806084572,-1.,3.97027773754922));
#31099=CARTESIAN_POINT('',(1.22531898815164,-1.,4.01728681790024));
#31100=CARTESIAN_POINT('',(1.36999806084572,-1.,3.97027773754922));
#31101=CARTESIAN_POINT('',(0.963899035118985,-1.,3.62400312501199));
#31102=CARTESIAN_POINT('Ctrl Pts',(1.22531898815164,-1.,4.01728681790024));
#31103=CARTESIAN_POINT('Ctrl Pts',(1.22423716681317,-1.,4.01614544569895));
#31104=CARTESIAN_POINT('Ctrl Pts',(1.22207656455845,-1.,4.01386104433519));
#31105=CARTESIAN_POINT('Ctrl Pts',(1.21884478244403,-1.,4.01042947140789));
#31106=CARTESIAN_POINT('Ctrl Pts',(1.21455398918133,-1.,4.00584409522722));
#31107=CARTESIAN_POINT('Ctrl Pts',(1.20922097029551,-1.,4.00009577950721));
#31108=CARTESIAN_POINT('Ctrl Pts',(1.20391852375138,-1.,3.99433084799666));
#31109=CARTESIAN_POINT('Ctrl Pts',(1.19864679609566,-1.,3.98854928957189));
#31110=CARTESIAN_POINT('Ctrl Pts',(1.19340598349475,-1.,3.98275111052561));
#31111=CARTESIAN_POINT('Ctrl Pts',(1.18819633715539,-1.,3.97693634767754));
#31112=CARTESIAN_POINT('Ctrl Pts',(1.18301815039831,-1.,3.97110505165415));
#31113=CARTESIAN_POINT('Ctrl Pts',(1.17787174135592,-1.,3.96525726358159));
#31114=CARTESIAN_POINT('Ctrl Pts',(1.17275743590361,-1.,3.95939299213276));
#31115=CARTESIAN_POINT('Ctrl Pts',(1.16767555244438,-1.,3.95351219509876));
#31116=CARTESIAN_POINT('Ctrl Pts',(1.16262637999157,-1.,3.94761474780583));
#31117=CARTESIAN_POINT('Ctrl Pts',(1.15761018340956,-1.,3.94170046685203));
#31118=CARTESIAN_POINT('Ctrl Pts',(1.1526272271632,-1.,3.9357691705628));
#31119=CARTESIAN_POINT('Ctrl Pts',(1.14767779451123,-1.,3.92982073294257));
#31120=CARTESIAN_POINT('Ctrl Pts',(1.14276220561593,-1.,3.92385513133997));
#31121=CARTESIAN_POINT('Ctrl Pts',(1.13788084225554,-1.,3.91787251936827));
#31122=CARTESIAN_POINT('Ctrl Pts',(1.13303414693896,-1.,3.91187321145649));
#31123=CARTESIAN_POINT('Ctrl Pts',(1.12822258281553,-1.,3.90585753318737));
#31124=CARTESIAN_POINT('Ctrl Pts',(1.12344660099043,-1.,3.89982569750025));
#31125=CARTESIAN_POINT('Ctrl Pts',(1.11870660794603,-1.,3.89377768340344));
#31126=CARTESIAN_POINT('Ctrl Pts',(1.11400292434429,-1.,3.88771308285171));
#31127=CARTESIAN_POINT('Ctrl Pts',(1.10933577224008,-1.,3.88163105531724));
#31128=CARTESIAN_POINT('Ctrl Pts',(1.10470536603287,-1.,3.87553067187514));
#31129=CARTESIAN_POINT('Ctrl Pts',(1.10011198761195,-1.,3.86941120134849));
#31130=CARTESIAN_POINT('Ctrl Pts',(1.09555606505013,-1.,3.86327241021247));
#31131=CARTESIAN_POINT('Ctrl Pts',(1.09103825516294,-1.,3.85711487933931));
#31132=CARTESIAN_POINT('Ctrl Pts',(1.08655950846384,-1.,3.85094025222713));
#31133=CARTESIAN_POINT('Ctrl Pts',(1.08212087917991,-1.,3.8447504803063));
#31134=CARTESIAN_POINT('Ctrl Pts',(1.07772335353858,-1.,3.83854714117491));
#31135=CARTESIAN_POINT('Ctrl Pts',(1.07336766633459,-1.,3.83233071195144));
#31136=CARTESIAN_POINT('Ctrl Pts',(1.06905413180359,-1.,3.82609989967276));
#31137=CARTESIAN_POINT('Ctrl Pts',(1.0647824403893,-1.,3.81985083953012));
#31138=CARTESIAN_POINT('Ctrl Pts',(1.06055206187299,-1.,3.8135786611749));
#31139=CARTESIAN_POINT('Ctrl Pts',(1.05636266918644,-1.,3.80727913637791));
#31140=CARTESIAN_POINT('Ctrl Pts',(1.05221457990016,-1.,3.80095039790681));
#31141=CARTESIAN_POINT('Ctrl Pts',(1.04810913267639,-1.,3.79459440308786));
#31142=CARTESIAN_POINT('Ctrl Pts',(1.04404924374422,-1.,3.78821910787179));
#31143=CARTESIAN_POINT('Ctrl Pts',(1.04003862055798,-1.,3.7818353500817));
#31144=CARTESIAN_POINT('Ctrl Pts',(1.03608074678008,-1.,3.77545283140427));
#31145=CARTESIAN_POINT('Ctrl Pts',(1.03217786604919,-1.,3.76907609832516));
#31146=CARTESIAN_POINT('Ctrl Pts',(1.02833014458184,-1.,3.76270122291245));
#31147=CARTESIAN_POINT('Ctrl Pts',(1.02453429444668,-1.,3.75631037456224));
#31148=CARTESIAN_POINT('Ctrl Pts',(1.02078510487439,-1.,3.74987777155873));
#31149=CARTESIAN_POINT('Ctrl Pts',(1.01707794311088,-1.,3.74337942504993));
#31150=CARTESIAN_POINT('Ctrl Pts',(1.01341114319906,-1.,3.73680245055747));
#31151=CARTESIAN_POINT('Ctrl Pts',(1.00978798539491,-1.,3.73015276704407));
#31152=CARTESIAN_POINT('Ctrl Pts',(1.00622000735696,-1.,3.72346803750544));
#31153=CARTESIAN_POINT('Ctrl Pts',(1.00272423396802,-1.,3.71680667125047));
#31154=CARTESIAN_POINT('Ctrl Pts',(0.999317260756344,-1.,3.7102243971387));
#31155=CARTESIAN_POINT('Ctrl Pts',(0.996009819772431,-1.,3.70375282282107));
#31156=CARTESIAN_POINT('Ctrl Pts',(0.992802218332103,-1.,3.69738123415696));
#31157=CARTESIAN_POINT('Ctrl Pts',(0.989676715398858,-1.,3.69102682138955));
#31158=CARTESIAN_POINT('Ctrl Pts',(0.986602639864285,-1.,3.6845531792623));
#31159=CARTESIAN_POINT('Ctrl Pts',(0.983550791470864,-1.,3.67782408841876));
#31160=CARTESIAN_POINT('Ctrl Pts',(0.980505922458494,-1.,3.67074983340444));
#31161=CARTESIAN_POINT('Ctrl Pts',(0.977478312751416,-1.,3.66333049637403));
#31162=CARTESIAN_POINT('Ctrl Pts',(0.974519971354138,-1.,3.6557157673487));
#31163=CARTESIAN_POINT('Ctrl Pts',(0.971722122060277,-1.,3.64819756447072));
#31164=CARTESIAN_POINT('Ctrl Pts',(0.969195124674828,-1.,3.64113946505393));
#31165=CARTESIAN_POINT('Ctrl Pts',(0.967052554540877,-1.,3.6349212208096));
#31166=CARTESIAN_POINT('Ctrl Pts',(0.965395153165715,-1.,3.62988252139998));
#31167=CARTESIAN_POINT('Ctrl Pts',(0.964373850166081,-1.,3.62652618145252));
#31168=CARTESIAN_POINT('Ctrl Pts',(0.963957782642589,-1.,3.62489305727516));
#31169=CARTESIAN_POINT('Ctrl Pts',(0.963861297423578,-1.,3.62424461507455));
#31170=CARTESIAN_POINT('Ctrl Pts',(0.963880158556713,-1.,3.62404828878374));
#31171=CARTESIAN_POINT('Ctrl Pts',(0.963899035118985,-1.,3.62400312501199));
#31172=CARTESIAN_POINT('',(0.786422660833742,-1.,3.66661143271648));
#31173=CARTESIAN_POINT('Origin',(0.,-1.,0.));
#31174=CARTESIAN_POINT('',(0.732042837400619,-1.,4.13571194405636));
#31175=CARTESIAN_POINT('Ctrl Pts',(0.786422660833742,-1.,3.66661143271648));
#31176=CARTESIAN_POINT('Ctrl Pts',(0.786459983896781,-1.,3.66664310415236));
#31177=CARTESIAN_POINT('Ctrl Pts',(0.786565919559889,-1.,3.66680946938396));
#31178=CARTESIAN_POINT('Ctrl Pts',(0.786774337198499,-1.,3.66743103898844));
#31179=CARTESIAN_POINT('Ctrl Pts',(0.787145041181588,-1.,3.66907505398769));
#31180=CARTESIAN_POINT('Ctrl Pts',(0.787758799995426,-1.,3.672529236635));
#31181=CARTESIAN_POINT('Ctrl Pts',(0.788569566220662,-1.,3.67777119516438));
#31182=CARTESIAN_POINT('Ctrl Pts',(0.789483546065158,-1.,3.68428439784285));
#31183=CARTESIAN_POINT('Ctrl Pts',(0.790436284989579,-1.,3.69172044327754));
#31184=CARTESIAN_POINT('Ctrl Pts',(0.791356575696508,-1.,3.69968940808982));
#31185=CARTESIAN_POINT('Ctrl Pts',(0.792177688845967,-1.,3.70781724021879));
#31186=CARTESIAN_POINT('Ctrl Pts',(0.792848377370115,-1.,3.7158024239604));
#31187=CARTESIAN_POINT('Ctrl Pts',(0.79334702378387,-1.,3.7234879729357));
#31188=CARTESIAN_POINT('Ctrl Pts',(0.793682750269347,-1.,3.7308691469564));
#31189=CARTESIAN_POINT('Ctrl Pts',(0.79388270093679,-1.,3.73803280541576));
#31190=CARTESIAN_POINT('Ctrl Pts',(0.79398270045988,-1.,3.74511357728827));
#31191=CARTESIAN_POINT('Ctrl Pts',(0.79401734737144,-1.,3.75224692493895));
#31192=CARTESIAN_POINT('Ctrl Pts',(0.794008429135046,-1.,3.75951468666325));
#31193=CARTESIAN_POINT('Ctrl Pts',(0.793961083689141,-1.,3.76692626931184));
#31194=CARTESIAN_POINT('Ctrl Pts',(0.793870523787515,-1.,3.77444863801264));
#31195=CARTESIAN_POINT('Ctrl Pts',(0.793726235781339,-1.,3.78202460377617));
#31196=CARTESIAN_POINT('Ctrl Pts',(0.793516871680965,-1.,3.78959439439222));
#31197=CARTESIAN_POINT('Ctrl Pts',(0.7932356129732,-1.,3.79711921389862));
#31198=CARTESIAN_POINT('Ctrl Pts',(0.792882695234692,-1.,3.80459229925598));
#31199=CARTESIAN_POINT('Ctrl Pts',(0.792462483517568,-1.,3.81202588694726));
#31200=CARTESIAN_POINT('Ctrl Pts',(0.791981740718606,-1.,3.81944345442237));
#31201=CARTESIAN_POINT('Ctrl Pts',(0.791447528662381,-1.,3.82687033899799));
#31202=CARTESIAN_POINT('Ctrl Pts',(0.790865012705339,-1.,3.83432392054804));
#31203=CARTESIAN_POINT('Ctrl Pts',(0.790236124191289,-1.,3.84180762342476));
#31204=CARTESIAN_POINT('Ctrl Pts',(0.789560798155618,-1.,3.8493163780891));
#31205=CARTESIAN_POINT('Ctrl Pts',(0.788837734090688,-1.,3.85683995872536));
#31206=CARTESIAN_POINT('Ctrl Pts',(0.78806531509377,-1.,3.86436702561342));
#31207=CARTESIAN_POINT('Ctrl Pts',(0.78724252761798,-1.,3.87188916600905));
#31208=CARTESIAN_POINT('Ctrl Pts',(0.786369675812591,-1.,3.87940402818186));
#31209=CARTESIAN_POINT('Ctrl Pts',(0.785447890340723,-1.,3.88691313167399));
#31210=CARTESIAN_POINT('Ctrl Pts',(0.784478799358335,-1.,3.89442039235105));
#31211=CARTESIAN_POINT('Ctrl Pts',(0.783464141529082,-1.,3.90193039043971));
#31212=CARTESIAN_POINT('Ctrl Pts',(0.782405395622758,-1.,3.90944671004536));
#31213=CARTESIAN_POINT('Ctrl Pts',(0.781303428618343,-1.,3.9169703605466));
#31214=CARTESIAN_POINT('Ctrl Pts',(0.780158678615506,-1.,3.92450058323799));
#31215=CARTESIAN_POINT('Ctrl Pts',(0.778971308134786,-1.,3.93203552473153));
#31216=CARTESIAN_POINT('Ctrl Pts',(0.777741370568549,-1.,3.93957296768098));
#31217=CARTESIAN_POINT('Ctrl Pts',(0.776468966697959,-1.,3.94711101619471));
#31218=CARTESIAN_POINT('Ctrl Pts',(0.775154418039441,-1.,3.95464885452364));
#31219=CARTESIAN_POINT('Ctrl Pts',(0.773798212026682,-1.,3.96218649639876));
#31220=CARTESIAN_POINT('Ctrl Pts',(0.772400931772238,-1.,3.96972446532832));
#31221=CARTESIAN_POINT('Ctrl Pts',(0.770963190030503,-1.,3.97726349165507));
#31222=CARTESIAN_POINT('Ctrl Pts',(0.769485566245459,-1.,3.98480422348403));
#31223=CARTESIAN_POINT('Ctrl Pts',(0.767968531377707,-1.,3.99234687880892));
#31224=CARTESIAN_POINT('Ctrl Pts',(0.766412457135785,-1.,3.99989129179464));
#31225=CARTESIAN_POINT('Ctrl Pts',(0.764817648784946,-1.,4.00743706791366));
#31226=CARTESIAN_POINT('Ctrl Pts',(0.763184371182826,-1.,4.01498370680434));
#31227=CARTESIAN_POINT('Ctrl Pts',(0.761512875859941,-1.,4.02253072741347));
#31228=CARTESIAN_POINT('Ctrl Pts',(0.759803433244165,-1.,4.0300778195465));
#31229=CARTESIAN_POINT('Ctrl Pts',(0.758056338885553,-1.,4.03762485803468));
#31230=CARTESIAN_POINT('Ctrl Pts',(0.756271902370186,-1.,4.04517182654344));
#31231=CARTESIAN_POINT('Ctrl Pts',(0.754450441816411,-1.,4.05271876688106));
#31232=CARTESIAN_POINT('Ctrl Pts',(0.752592276482868,-1.,4.06026572221399));
#31233=CARTESIAN_POINT('Ctrl Pts',(0.750697720483175,-1.,4.06781267241886));
#31234=CARTESIAN_POINT('Ctrl Pts',(0.748767076679176,-1.,4.07535951055363));
#31235=CARTESIAN_POINT('Ctrl Pts',(0.746800631490821,-1.,4.08290608094789));
#31236=CARTESIAN_POINT('Ctrl Pts',(0.744798649705513,-1.,4.09045220253011));
#31237=CARTESIAN_POINT('Ctrl Pts',(0.742761369690017,-1.,4.09799769702712));
#31238=CARTESIAN_POINT('Ctrl Pts',(0.740688998555151,-1.,4.1055424175856));
#31239=CARTESIAN_POINT('Ctrl Pts',(0.738581708229118,-1.,4.11308626953795));
#31240=CARTESIAN_POINT('Ctrl Pts',(0.736439634335347,-1.,4.12062919626082));
#31241=CARTESIAN_POINT('Ctrl Pts',(0.734698226767512,-1.,4.12666277572794));
#31242=CARTESIAN_POINT('Ctrl Pts',(0.733376589325634,-1.,4.13118752796397));
#31243=CARTESIAN_POINT('Ctrl Pts',(0.732488575135925,-1.,4.13420383737278));
#31244=CARTESIAN_POINT('Ctrl Pts',(0.732042837400619,-1.,4.13571194405636));
#31245=CARTESIAN_POINT('',(0.581791163835814,-1.,4.15950947128175));
#31246=CARTESIAN_POINT('',(0.732042837400619,-1.,4.13571194405636));
#31247=CARTESIAN_POINT('',(0.385112848332549,-1.,3.73017266276632));
#31248=CARTESIAN_POINT('Ctrl Pts',(0.581791163835814,-1.,4.15950947128175));
#31249=CARTESIAN_POINT('Ctrl Pts',(0.580901211462913,-1.,4.15821291712391));
#31250=CARTESIAN_POINT('Ctrl Pts',(0.579124568912543,-1.,4.15561864787379));
#31251=CARTESIAN_POINT('Ctrl Pts',(0.576469391673916,-1.,4.1517237611974));
#31252=CARTESIAN_POINT('Ctrl Pts',(0.572948736066276,-1.,4.14652361065787));
#31253=CARTESIAN_POINT('Ctrl Pts',(0.568580610187115,-1.,4.14001179828669));
#31254=CARTESIAN_POINT('Ctrl Pts',(0.564245279535705,-1.,4.13348835726086));
#31255=CARTESIAN_POINT('Ctrl Pts',(0.559942890594628,-1.,4.12695329951859));
#31256=CARTESIAN_POINT('Ctrl Pts',(0.555673636130778,-1.,4.1204066619623));
#31257=CARTESIAN_POINT('Ctrl Pts',(0.551437758498246,-1.,4.11384852025578));
#31258=CARTESIAN_POINT('Ctrl Pts',(0.547235539486759,-1.,4.1072789702877));
#31259=CARTESIAN_POINT('Ctrl Pts',(0.543067286878457,-1.,4.10069810244473));
#31260=CARTESIAN_POINT('Ctrl Pts',(0.53893332117992,-1.,4.09410597627116));
#31261=CARTESIAN_POINT('Ctrl Pts',(0.534833963476999,-1.,4.08750259988693));
#31262=CARTESIAN_POINT('Ctrl Pts',(0.530769518728075,-1.,4.08088789536488));
#31263=CARTESIAN_POINT('Ctrl Pts',(0.526740277226999,-1.,4.07426172299496));
#31264=CARTESIAN_POINT('Ctrl Pts',(0.522746528602767,-1.,4.06762394471075));
#31265=CARTESIAN_POINT('Ctrl Pts',(0.518788572336809,-1.,4.06097448037934));
#31266=CARTESIAN_POINT('Ctrl Pts',(0.514866728193103,-1.,4.05431335771261));
#31267=CARTESIAN_POINT('Ctrl Pts',(0.510981349219173,-1.,4.04764078815591));
#31268=CARTESIAN_POINT('Ctrl Pts',(0.507132823288361,-1.,4.04095715149074));
#31269=CARTESIAN_POINT('Ctrl Pts',(0.503321556915513,-1.,4.0342628417439));
#31270=CARTESIAN_POINT('Ctrl Pts',(0.499547962340889,-1.,4.0275581398015));
#31271=CARTESIAN_POINT('Ctrl Pts',(0.495812444326222,-1.,4.02084308851813));
#31272=CARTESIAN_POINT('Ctrl Pts',(0.49211538341793,-1.,4.01411733503486));
#31273=CARTESIAN_POINT('Ctrl Pts',(0.48845713042453,-1.,4.0073800839092));
#31274=CARTESIAN_POINT('Ctrl Pts',(0.484838042421754,-1.,4.00063045119234));
#31275=CARTESIAN_POINT('Ctrl Pts',(0.481258512209637,-1.,3.99386775880655));
#31276=CARTESIAN_POINT('Ctrl Pts',(0.477718999122033,-1.,3.98709184306743));
#31277=CARTESIAN_POINT('Ctrl Pts',(0.474220061019542,-1.,3.9803033804443));
#31278=CARTESIAN_POINT('Ctrl Pts',(0.470762379613477,-1.,3.97350414289415));
#31279=CARTESIAN_POINT('Ctrl Pts',(0.467346690880671,-1.,3.96669622273946));
#31280=CARTESIAN_POINT('Ctrl Pts',(0.463973722115744,-1.,3.95988133243543));
#31281=CARTESIAN_POINT('Ctrl Pts',(0.460644124429119,-1.,3.95306005817363));
#31282=CARTESIAN_POINT('Ctrl Pts',(0.457358410451673,-1.,3.94623117206675));
#31283=CARTESIAN_POINT('Ctrl Pts',(0.454116879027575,-1.,3.93939080846298));
#31284=CARTESIAN_POINT('Ctrl Pts',(0.450919768356346,-1.,3.93253407403128));
#31285=CARTESIAN_POINT('Ctrl Pts',(0.447767416837296,-1.,3.92565674143424));
#31286=CARTESIAN_POINT('Ctrl Pts',(0.444660430230592,-1.,3.91875701610721));
#31287=CARTESIAN_POINT('Ctrl Pts',(0.441599824524047,-1.,3.91183704069146));
#31288=CARTESIAN_POINT('Ctrl Pts',(0.438587235458233,-1.,3.90490512938546));
#31289=CARTESIAN_POINT('Ctrl Pts',(0.435624629433505,-1.,3.8979725665544));
#31290=CARTESIAN_POINT('Ctrl Pts',(0.432713929544439,-1.,3.89104947940592));
#31291=CARTESIAN_POINT('Ctrl Pts',(0.429856640579733,-1.,3.88414070943334));
#31292=CARTESIAN_POINT('Ctrl Pts',(0.427053541173469,-1.,3.87724240306609));
#31293=CARTESIAN_POINT('Ctrl Pts',(0.424304173195142,-1.,3.87033643487882));
#31294=CARTESIAN_POINT('Ctrl Pts',(0.421607423177575,-1.,3.86339652542749));
#31295=CARTESIAN_POINT('Ctrl Pts',(0.418962468086809,-1.,3.85639825648031));
#31296=CARTESIAN_POINT('Ctrl Pts',(0.41636967805292,-1.,3.8493286415751));
#31297=CARTESIAN_POINT('Ctrl Pts',(0.413831367016726,-1.,3.84219403994742));
#31298=CARTESIAN_POINT('Ctrl Pts',(0.411353038798459,-1.,3.83503345578645));
#31299=CARTESIAN_POINT('Ctrl Pts',(0.408942371447376,-1.,3.82790724256397));
#31300=CARTESIAN_POINT('Ctrl Pts',(0.406607038258906,-1.,3.82087303913741));
#31301=CARTESIAN_POINT('Ctrl Pts',(0.404352694628236,-1.,3.81396374287762));
#31302=CARTESIAN_POINT('Ctrl Pts',(0.402181320148474,-1.,3.80716881962763));
#31303=CARTESIAN_POINT('Ctrl Pts',(0.400088346504726,-1.,3.80040370384659));
#31304=CARTESIAN_POINT('Ctrl Pts',(0.398064818684158,-1.,3.79352887163457));
#31305=CARTESIAN_POINT('Ctrl Pts',(0.396103205335028,-1.,3.78640521279479));
#31306=CARTESIAN_POINT('Ctrl Pts',(0.394202481011595,-1.,3.77894173114368));
#31307=CARTESIAN_POINT('Ctrl Pts',(0.392372786223346,-1.,3.77114011595892));
#31308=CARTESIAN_POINT('Ctrl Pts',(0.390642072979258,-1.,3.76315635032993));
#31309=CARTESIAN_POINT('Ctrl Pts',(0.38905477589825,-1.,3.75529302894757));
#31310=CARTESIAN_POINT('Ctrl Pts',(0.387663020050396,-1.,3.74792651696269));
#31311=CARTESIAN_POINT('Ctrl Pts',(0.386519576222035,-1.,3.74144965781088));
#31312=CARTESIAN_POINT('Ctrl Pts',(0.385670806454744,-1.,3.73621371845475));
#31313=CARTESIAN_POINT('Ctrl Pts',(0.385187124633964,-1.,3.73273893363318));
#31314=CARTESIAN_POINT('Ctrl Pts',(0.385031656499141,-1.,3.73106082862399));
#31315=CARTESIAN_POINT('Ctrl Pts',(0.385037797882046,-1.,3.73040527620929));
#31316=CARTESIAN_POINT('Ctrl Pts',(0.385087139001608,-1.,3.73021431755218));
#31317=CARTESIAN_POINT('Ctrl Pts',(0.385112848332549,-1.,3.73017266276632));
#31318=CARTESIAN_POINT('',(0.203156094897895,-1.,3.74449296982994));
#31319=CARTESIAN_POINT('Origin',(0.,-1.,0.));
#31320=CARTESIAN_POINT('',(0.0760622897878233,-1.,4.19931119685982));
#31321=CARTESIAN_POINT('Ctrl Pts',(0.203156094897895,-1.,3.74449296982994));
#31322=CARTESIAN_POINT('Ctrl Pts',(0.203188003947964,-1.,3.74453008995129));
#31323=CARTESIAN_POINT('Ctrl Pts',(0.203266610111263,-1.,3.74471097893961));
#31324=CARTESIAN_POINT('Ctrl Pts',(0.203375226874331,-1.,3.74535749969262));
#31325=CARTESIAN_POINT('Ctrl Pts',(0.203484186269314,-1.,3.74703926501843));
#31326=CARTESIAN_POINT('Ctrl Pts',(0.203550035479096,-1.,3.75054693397716));
#31327=CARTESIAN_POINT('Ctrl Pts',(0.203530796848403,-1.,3.75585118707924));
#31328=CARTESIAN_POINT('Ctrl Pts',(0.203414634707646,-1.,3.76242717937273));
#31329=CARTESIAN_POINT('Ctrl Pts',(0.203192390045337,-1.,3.76992071595267));
#31330=CARTESIAN_POINT('Ctrl Pts',(0.202854729699196,-1.,3.77793553476879));
#31331=CARTESIAN_POINT('Ctrl Pts',(0.202394260512192,-1.,3.78609175019317));
#31332=CARTESIAN_POINT('Ctrl Pts',(0.201807533800798,-1.,3.79408354187274));
#31333=CARTESIAN_POINT('Ctrl Pts',(0.201097756307251,-1.,3.80175247447171));
#31334=CARTESIAN_POINT('Ctrl Pts',(0.200274679433289,-1.,3.80909529318501));
#31335=CARTESIAN_POINT('Ctrl Pts',(0.199351525297396,-1.,3.81620203429702));
#31336=CARTESIAN_POINT('Ctrl Pts',(0.198342616900469,-1.,3.82321127348981));
#31337=CARTESIAN_POINT('Ctrl Pts',(0.197260935827375,-1.,3.83026221776488));
#31338=CARTESIAN_POINT('Ctrl Pts',(0.196115198971889,-1.,3.83743910616265));
#31339=CARTESIAN_POINT('Ctrl Pts',(0.194909009460254,-1.,3.84475203347052));
#31340=CARTESIAN_POINT('Ctrl Pts',(0.193642806777747,-1.,3.85216762264019));
#31341=CARTESIAN_POINT('Ctrl Pts',(0.192315153044979,-1.,3.85962774407652));
#31342=CARTESIAN_POINT('Ctrl Pts',(0.190924190418612,-1.,3.8670715862477));
#31343=CARTESIAN_POINT('Ctrl Pts',(0.189469253358254,-1.,3.87445976418377));
#31344=CARTESIAN_POINT('Ctrl Pts',(0.187951632512663,-1.,3.88178563496187));
#31345=CARTESIAN_POINT('Ctrl Pts',(0.186373724985263,-1.,3.88906196725817));
#31346=CARTESIAN_POINT('Ctrl Pts',(0.184738537728034,-1.,3.89631300742633));
#31347=CARTESIAN_POINT('Ctrl Pts',(0.183049081993193,-1.,3.90356488555138));
#31348=CARTESIAN_POINT('Ctrl Pts',(0.181307740731795,-1.,3.91083557557193));
#31349=CARTESIAN_POINT('Ctrl Pts',(0.179515885822894,-1.,3.91812876180948));
#31350=CARTESIAN_POINT('Ctrl Pts',(0.177674246152328,-1.,3.92543942697672));
#31351=CARTESIAN_POINT('Ctrl Pts',(0.175783136893872,-1.,3.93275726771049));
#31352=CARTESIAN_POINT('Ctrl Pts',(0.173842734974607,-1.,3.94007083096214));
#31353=CARTESIAN_POINT('Ctrl Pts',(0.171853355369232,-1.,3.94737164900861));
#31354=CARTESIAN_POINT('Ctrl Pts',(0.16981566637413,-1.,3.95465744665263));
#31355=CARTESIAN_POINT('Ctrl Pts',(0.167730547023312,-1.,3.96192990160296));
#31356=CARTESIAN_POINT('Ctrl Pts',(0.165598992851097,-1.,3.9691931362141));
#31357=CARTESIAN_POINT('Ctrl Pts',(0.163422004609998,-1.,3.97645194630944));
#31358=CARTESIAN_POINT('Ctrl Pts',(0.161200482186087,-1.,3.98371010319866));
#31359=CARTESIAN_POINT('Ctrl Pts',(0.158935123982796,-1.,3.99096873945862));
#31360=CARTESIAN_POINT('Ctrl Pts',(0.156626481393735,-1.,3.99822717425869));
#31361=CARTESIAN_POINT('Ctrl Pts',(0.154275004872309,-1.,4.00548360245297));
#31362=CARTESIAN_POINT('Ctrl Pts',(0.151881094022909,-1.,4.01273584234684));
#31363=CARTESIAN_POINT('Ctrl Pts',(0.149445144968707,-1.,4.01998203715588));
#31364=CARTESIAN_POINT('Ctrl Pts',(0.146967602878998,-1.,4.02722143147048));
#31365=CARTESIAN_POINT('Ctrl Pts',(0.144448947038352,-1.,4.03445411510403));
#31366=CARTESIAN_POINT('Ctrl Pts',(0.141889671485507,-1.,4.04168069633842));
#31367=CARTESIAN_POINT('Ctrl Pts',(0.139290267180059,-1.,4.04890199238056));
#31368=CARTESIAN_POINT('Ctrl Pts',(0.136651205046111,-1.,4.05611873400122));
#31369=CARTESIAN_POINT('Ctrl Pts',(0.133972916144225,-1.,4.06333121018476));
#31370=CARTESIAN_POINT('Ctrl Pts',(0.131255793548914,-1.,4.07053931528579));
#31371=CARTESIAN_POINT('Ctrl Pts',(0.128500200484813,-1.,4.07774270738809));
#31372=CARTESIAN_POINT('Ctrl Pts',(0.125706476822529,-1.,4.08494093372315));
#31373=CARTESIAN_POINT('Ctrl Pts',(0.122874946249119,-1.,4.09213355850836));
#31374=CARTESIAN_POINT('Ctrl Pts',(0.120005924388162,-1.,4.09932031767243));
#31375=CARTESIAN_POINT('Ctrl Pts',(0.117099722731704,-1.,4.10650113382187));
#31376=CARTESIAN_POINT('Ctrl Pts',(0.114156649609601,-1.,4.11367603925313));
#31377=CARTESIAN_POINT('Ctrl Pts',(0.111177012683377,-1.,4.12084512502444));
#31378=CARTESIAN_POINT('Ctrl Pts',(0.10816112052835,-1.,4.12800848371386));
#31379=CARTESIAN_POINT('Ctrl Pts',(0.105109286538864,-1.,4.13516614458396));
#31380=CARTESIAN_POINT('Ctrl Pts',(0.102021826577453,-1.,4.14231804938737));
#31381=CARTESIAN_POINT('Ctrl Pts',(0.0988990478899809,-1.,4.1494640891762));
#31382=CARTESIAN_POINT('Ctrl Pts',(0.0957412403297065,-1.,4.15660412653006));
#31383=CARTESIAN_POINT('Ctrl Pts',(0.0925486672167687,-1.,4.16373802265942));
#31384=CARTESIAN_POINT('Ctrl Pts',(0.0893215560850325,-1.,4.17086566491823));
#31385=CARTESIAN_POINT('Ctrl Pts',(0.0860600915552512,-1.,4.17798698669991));
#31386=CARTESIAN_POINT('Ctrl Pts',(0.0827644164389507,-1.,4.1851019532944));
#31387=CARTESIAN_POINT('Ctrl Pts',(0.08010058871176,-1.,4.19078883322483));
#31388=CARTESIAN_POINT('Ctrl Pts',(0.0780873956244399,-1.,4.19505112860624));
#31389=CARTESIAN_POINT('Ctrl Pts',(0.0767384596142192,-1.,4.19789138621624));
#31390=CARTESIAN_POINT('Ctrl Pts',(0.0760622897878233,-1.,4.19931119685982));
#31391=CARTESIAN_POINT('',(-0.0760622897878249,-1.,4.19931119685982));
#31392=CARTESIAN_POINT('',(0.0760622897878233,-1.,4.19931119685982));
#31393=CARTESIAN_POINT('',(-0.203156094896101,-1.,3.74449296983004));
#31394=CARTESIAN_POINT('Ctrl Pts',(-0.0760622897878249,-1.,4.19931119685982));
#31395=CARTESIAN_POINT('Ctrl Pts',(-0.0767384596141467,-1.,4.1978913862118));
#31396=CARTESIAN_POINT('Ctrl Pts',(-0.07808739562424,-1.,4.19505112859416));
#31397=CARTESIAN_POINT('Ctrl Pts',(-0.0801005887114322,-1.,4.19078883320504));
#31398=CARTESIAN_POINT('Ctrl Pts',(-0.0827644164385681,-1.,4.18510195327123));
#31399=CARTESIAN_POINT('Ctrl Pts',(-0.0860600915549399,-1.,4.17798698668094));
#31400=CARTESIAN_POINT('Ctrl Pts',(-0.0893215560848652,-1.,4.17086566490794));
#31401=CARTESIAN_POINT('Ctrl Pts',(-0.0925486672167534,-1.,4.16373802265839));
#31402=CARTESIAN_POINT('Ctrl Pts',(-0.0957412403298009,-1.,4.15660412653577));
#31403=CARTESIAN_POINT('Ctrl Pts',(-0.0988990478901228,-1.,4.14946408918485));
#31404=CARTESIAN_POINT('Ctrl Pts',(-0.102021826577584,-1.,4.14231804939538));
#31405=CARTESIAN_POINT('Ctrl Pts',(-0.105109286538945,-1.,4.13516614458895));
#31406=CARTESIAN_POINT('Ctrl Pts',(-0.10816112052837,-1.,4.12800848371504));
#31407=CARTESIAN_POINT('Ctrl Pts',(-0.111177012683347,-1.,4.1208451250225));
#31408=CARTESIAN_POINT('Ctrl Pts',(-0.114156649609546,-1.,4.11367603924961));
#31409=CARTESIAN_POINT('Ctrl Pts',(-0.117099722731648,-1.,4.10650113381833));
#31410=CARTESIAN_POINT('Ctrl Pts',(-0.120005924388124,-1.,4.09932031767002));
#31411=CARTESIAN_POINT('Ctrl Pts',(-0.122874946249107,-1.,4.09213355850756));
#31412=CARTESIAN_POINT('Ctrl Pts',(-0.12570647682254,-1.,4.08494093372377));
#31413=CARTESIAN_POINT('Ctrl Pts',(-0.128500200484838,-1.,4.07774270738954));
#31414=CARTESIAN_POINT('Ctrl Pts',(-0.131255793548941,-1.,4.0705393152874));
#31415=CARTESIAN_POINT('Ctrl Pts',(-0.133972916144245,-1.,4.06333121018596));
#31416=CARTESIAN_POINT('Ctrl Pts',(-0.136651205046119,-1.,4.05611873400172));
#31417=CARTESIAN_POINT('Ctrl Pts',(-0.139290267180057,-1.,4.04890199238036));
#31418=CARTESIAN_POINT('Ctrl Pts',(-0.1418896714855,-1.,4.04168069633781));
#31419=CARTESIAN_POINT('Ctrl Pts',(-0.144448947038345,-1.,4.03445411510333));
#31420=CARTESIAN_POINT('Ctrl Pts',(-0.146967602878994,-1.,4.02722143146994));
#31421=CARTESIAN_POINT('Ctrl Pts',(-0.149445144968707,-1.,4.01998203715564));
#31422=CARTESIAN_POINT('Ctrl Pts',(-0.151881094022911,-1.,4.01273584234689));
#31423=CARTESIAN_POINT('Ctrl Pts',(-0.154275004872311,-1.,4.00548360245319));
#31424=CARTESIAN_POINT('Ctrl Pts',(-0.156626481393734,-1.,3.99822717425893));
#31425=CARTESIAN_POINT('Ctrl Pts',(-0.158935123982793,-1.,3.99096873945878));
#31426=CARTESIAN_POINT('Ctrl Pts',(-0.161200482186085,-1.,3.98371010319872));
#31427=CARTESIAN_POINT('Ctrl Pts',(-0.163422004609999,-1.,3.97645194630943));
#31428=CARTESIAN_POINT('Ctrl Pts',(-0.165598992851102,-1.,3.96919313621407));
#31429=CARTESIAN_POINT('Ctrl Pts',(-0.16773054702332,-1.,3.96192990160296));
#31430=CARTESIAN_POINT('Ctrl Pts',(-0.169815666374139,-1.,3.95465744665268));
#31431=CARTESIAN_POINT('Ctrl Pts',(-0.17185335536924,-1.,3.94737164900868));
#31432=CARTESIAN_POINT('Ctrl Pts',(-0.17384273497461,-1.,3.94007083096217));
#31433=CARTESIAN_POINT('Ctrl Pts',(-0.175783136893868,-1.,3.93275726771042));
#31434=CARTESIAN_POINT('Ctrl Pts',(-0.177674246152318,-1.,3.92543942697655));
#31435=CARTESIAN_POINT('Ctrl Pts',(-0.179515885822882,-1.,3.91812876180926));
#31436=CARTESIAN_POINT('Ctrl Pts',(-0.181307740731786,-1.,3.91083557557175));
#31437=CARTESIAN_POINT('Ctrl Pts',(-0.183049081993191,-1.,3.90356488555132));
#31438=CARTESIAN_POINT('Ctrl Pts',(-0.184738537728043,-1.,3.89631300742646));
#31439=CARTESIAN_POINT('Ctrl Pts',(-0.186373724985281,-1.,3.88906196725848));
#31440=CARTESIAN_POINT('Ctrl Pts',(-0.187951632512685,-1.,3.88178563496228));
#31441=CARTESIAN_POINT('Ctrl Pts',(-0.189469253358273,-1.,3.87445976418412));
#31442=CARTESIAN_POINT('Ctrl Pts',(-0.19092419041862,-1.,3.86707158624783));
#31443=CARTESIAN_POINT('Ctrl Pts',(-0.192315153044971,-1.,3.85962774407633));
#31444=CARTESIAN_POINT('Ctrl Pts',(-0.193642806777723,-1.,3.85216762263966));
#31445=CARTESIAN_POINT('Ctrl Pts',(-0.194909009460221,-1.,3.84475203346977));
#31446=CARTESIAN_POINT('Ctrl Pts',(-0.196115198971859,-1.,3.83743910616195));
#31447=CARTESIAN_POINT('Ctrl Pts',(-0.197260935827362,-1.,3.83026221776456));
#31448=CARTESIAN_POINT('Ctrl Pts',(-0.198342616900487,-1.,3.82321127349016));
#31449=CARTESIAN_POINT('Ctrl Pts',(-0.199351525297447,-1.,3.81620203429815));
#31450=CARTESIAN_POINT('Ctrl Pts',(-0.200274679433365,-1.,3.80909529318669));
#31451=CARTESIAN_POINT('Ctrl Pts',(-0.201097756307326,-1.,3.80175247447337));
#31452=CARTESIAN_POINT('Ctrl Pts',(-0.201807533800837,-1.,3.7940835418736));
#31453=CARTESIAN_POINT('Ctrl Pts',(-0.20239426051216,-1.,3.78609175019242));
#31454=CARTESIAN_POINT('Ctrl Pts',(-0.202854729699081,-1.,3.77793553476614));
#31455=CARTESIAN_POINT('Ctrl Pts',(-0.203192390045165,-1.,3.7699207159487));
#31456=CARTESIAN_POINT('Ctrl Pts',(-0.203414634707479,-1.,3.76242717936885));
#31457=CARTESIAN_POINT('Ctrl Pts',(-0.203530796848322,-1.,3.75585118707734));
#31458=CARTESIAN_POINT('Ctrl Pts',(-0.203550035479166,-1.,3.75054693397875));
#31459=CARTESIAN_POINT('Ctrl Pts',(-0.203484186269415,-1.,3.74703926501752));
#31460=CARTESIAN_POINT('Ctrl Pts',(-0.203375226874122,-1.,3.74535749969115));
#31461=CARTESIAN_POINT('Ctrl Pts',(-0.203266610110531,-1.,3.74471097893845));
#31462=CARTESIAN_POINT('Ctrl Pts',(-0.203188003946657,-1.,3.74453008995092));
#31463=CARTESIAN_POINT('Ctrl Pts',(-0.203156094896101,-1.,3.74449296983004));
#31464=CARTESIAN_POINT('',(-0.385112848330762,-1.,3.73017266276651));
#31465=CARTESIAN_POINT('Origin',(0.,-1.,0.));
#31466=CARTESIAN_POINT('',(-0.581791163835815,-1.,4.15950947128175));
#31467=CARTESIAN_POINT('Ctrl Pts',(-0.385112848330762,-1.,3.73017266276651));
#31468=CARTESIAN_POINT('Ctrl Pts',(-0.385087139000375,-1.,3.73021431755274));
#31469=CARTESIAN_POINT('Ctrl Pts',(-0.385037797881504,-1.,3.73040527621055));
#31470=CARTESIAN_POINT('Ctrl Pts',(-0.385031656499164,-1.,3.73106082862548));
#31471=CARTESIAN_POINT('Ctrl Pts',(-0.385187124634206,-1.,3.73273893363406));
#31472=CARTESIAN_POINT('Ctrl Pts',(-0.385670806454566,-1.,3.73621371845318));
#31473=CARTESIAN_POINT('Ctrl Pts',(-0.386519576222251,-1.,3.74144965781276));
#31474=CARTESIAN_POINT('Ctrl Pts',(-0.387663020050836,-1.,3.74792651696654));
#31475=CARTESIAN_POINT('Ctrl Pts',(-0.389054775898702,-1.,3.75529302895152));
#31476=CARTESIAN_POINT('Ctrl Pts',(-0.39064207297956,-1.,3.76315635033257));
#31477=CARTESIAN_POINT('Ctrl Pts',(-0.392372786223433,-1.,3.77114011595967));
#31478=CARTESIAN_POINT('Ctrl Pts',(-0.394202481011499,-1.,3.77894173114283));
#31479=CARTESIAN_POINT('Ctrl Pts',(-0.396103205334841,-1.,3.78640521279313));
#31480=CARTESIAN_POINT('Ctrl Pts',(-0.39806481868397,-1.,3.7935288716329));
#31481=CARTESIAN_POINT('Ctrl Pts',(-0.4000883465046,-1.,3.80040370384546));
#31482=CARTESIAN_POINT('Ctrl Pts',(-0.402181320148436,-1.,3.80716881962728));
#31483=CARTESIAN_POINT('Ctrl Pts',(-0.404352694628273,-1.,3.81396374287793));
#31484=CARTESIAN_POINT('Ctrl Pts',(-0.406607038258985,-1.,3.8208730391381));
#31485=CARTESIAN_POINT('Ctrl Pts',(-0.40894237144746,-1.,3.82790724256471));
#31486=CARTESIAN_POINT('Ctrl Pts',(-0.411353038798519,-1.,3.83503345578698));
#31487=CARTESIAN_POINT('Ctrl Pts',(-0.413831367016748,-1.,3.84219403994762));
#31488=CARTESIAN_POINT('Ctrl Pts',(-0.416369678052907,-1.,3.84932864157497));
#31489=CARTESIAN_POINT('Ctrl Pts',(-0.418962468086773,-1.,3.85639825647996));
#31490=CARTESIAN_POINT('Ctrl Pts',(-0.421607423177534,-1.,3.86339652542709));
#31491=CARTESIAN_POINT('Ctrl Pts',(-0.424304173195111,-1.,3.87033643487851));
#31492=CARTESIAN_POINT('Ctrl Pts',(-0.427053541173457,-1.,3.87724240306597));
#31493=CARTESIAN_POINT('Ctrl Pts',(-0.429856640579741,-1.,3.88414070943341));
#31494=CARTESIAN_POINT('Ctrl Pts',(-0.432713929544458,-1.,3.89104947940611));
#31495=CARTESIAN_POINT('Ctrl Pts',(-0.435624629433528,-1.,3.89797256655462));
#31496=CARTESIAN_POINT('Ctrl Pts',(-0.43858723545825,-1.,3.90490512938563));
#31497=CARTESIAN_POINT('Ctrl Pts',(-0.441599824524054,-1.,3.91183704069153));
#31498=CARTESIAN_POINT('Ctrl Pts',(-0.444660430230591,-1.,3.91875701610719));
#31499=CARTESIAN_POINT('Ctrl Pts',(-0.447767416837293,-1.,3.92565674143416));
#31500=CARTESIAN_POINT('Ctrl Pts',(-0.450919768356348,-1.,3.93253407403123));
#31501=CARTESIAN_POINT('Ctrl Pts',(-0.454116879027584,-1.,3.93939080846298));
#31502=CARTESIAN_POINT('Ctrl Pts',(-0.457358410451683,-1.,3.94623117206678));
#31503=CARTESIAN_POINT('Ctrl Pts',(-0.460644124429121,-1.,3.95306005817364));
#31504=CARTESIAN_POINT('Ctrl Pts',(-0.463973722115733,-1.,3.95988133243538));
#31505=CARTESIAN_POINT('Ctrl Pts',(-0.467346690880643,-1.,3.9666962227393));
#31506=CARTESIAN_POINT('Ctrl Pts',(-0.470762379613439,-1.,3.97350414289392));
#31507=CARTESIAN_POINT('Ctrl Pts',(-0.47422006101951,-1.,3.98030338044409));
#31508=CARTESIAN_POINT('Ctrl Pts',(-0.477718999122027,-1.,3.98709184306738));
#31509=CARTESIAN_POINT('Ctrl Pts',(-0.481258512209675,-1.,3.99386775880679));
#31510=CARTESIAN_POINT('Ctrl Pts',(-0.484838042421835,-1.,4.00063045119288));
#31511=CARTESIAN_POINT('Ctrl Pts',(-0.488457130424633,-1.,4.0073800839099));
#31512=CARTESIAN_POINT('Ctrl Pts',(-0.492115383418018,-1.,4.01411733503546));
#31513=CARTESIAN_POINT('Ctrl Pts',(-0.495812444326251,-1.,4.02084308851832));
#31514=CARTESIAN_POINT('Ctrl Pts',(-0.499547962340821,-1.,4.02755813980101));
#31515=CARTESIAN_POINT('Ctrl Pts',(-0.503321556915346,-1.,4.03426284174272));
#31516=CARTESIAN_POINT('Ctrl Pts',(-0.507132823288136,-1.,4.04095715148915));
#31517=CARTESIAN_POINT('Ctrl Pts',(-0.51098134921897,-1.,4.04764078815447));
#31518=CARTESIAN_POINT('Ctrl Pts',(-0.514866728193017,-1.,4.05431335771199));
#31519=CARTESIAN_POINT('Ctrl Pts',(-0.518788572336924,-1.,4.06097448038013));
#31520=CARTESIAN_POINT('Ctrl Pts',(-0.522746528603107,-1.,4.06762394471314));
#31521=CARTESIAN_POINT('Ctrl Pts',(-0.526740277227498,-1.,4.07426172299847));
#31522=CARTESIAN_POINT('Ctrl Pts',(-0.530769518728571,-1.,4.08088789536836));
#31523=CARTESIAN_POINT('Ctrl Pts',(-0.534833963477273,-1.,4.08750259988885));
#31524=CARTESIAN_POINT('Ctrl Pts',(-0.538933321179756,-1.,4.09410597627));
#31525=CARTESIAN_POINT('Ctrl Pts',(-0.543067286877757,-1.,4.10069810243979));
#31526=CARTESIAN_POINT('Ctrl Pts',(-0.547235539485637,-1.,4.10727897027977));
#31527=CARTESIAN_POINT('Ctrl Pts',(-0.551437758497033,-1.,4.11384852024721));
#31528=CARTESIAN_POINT('Ctrl Pts',(-0.555673636129977,-1.,4.12040666195664));
#31529=CARTESIAN_POINT('Ctrl Pts',(-0.559942890594774,-1.,4.12695329951961));
#31530=CARTESIAN_POINT('Ctrl Pts',(-0.564245279537149,-1.,4.13348835727104));
#31531=CARTESIAN_POINT('Ctrl Pts',(-0.568580610189775,-1.,4.14001179830547));
#31532=CARTESIAN_POINT('Ctrl Pts',(-0.572948736069522,-1.,4.14652361068081));
#31533=CARTESIAN_POINT('Ctrl Pts',(-0.576469391676688,-1.,4.151723761217));
#31534=CARTESIAN_POINT('Ctrl Pts',(-0.579124568914235,-1.,4.15561864788576));
#31535=CARTESIAN_POINT('Ctrl Pts',(-0.580901211463535,-1.,4.1582129171283));
#31536=CARTESIAN_POINT('Ctrl Pts',(-0.581791163835815,-1.,4.15950947128175));
#31537=CARTESIAN_POINT('',(-0.73204283740062,-1.,4.13571194405636));
#31538=CARTESIAN_POINT('',(-0.581791163835815,-1.,4.15950947128175));
#31539=CARTESIAN_POINT('',(-0.786422660831985,-1.,3.66661143271685));
#31540=CARTESIAN_POINT('Ctrl Pts',(-0.73204283740062,-1.,4.13571194405636));
#31541=CARTESIAN_POINT('Ctrl Pts',(-0.73248857513516,-1.,4.1342038373684));
#31542=CARTESIAN_POINT('Ctrl Pts',(-0.733376589323546,-1.,4.13118752795207));
#31543=CARTESIAN_POINT('Ctrl Pts',(-0.734698226764092,-1.,4.12666277570844));
#31544=CARTESIAN_POINT('Ctrl Pts',(-0.736439634331345,-1.,4.120629196238));
#31545=CARTESIAN_POINT('Ctrl Pts',(-0.738581708225844,-1.,4.11308626951927));
#31546=CARTESIAN_POINT('Ctrl Pts',(-0.740688998553377,-1.,4.10554241757547));
#31547=CARTESIAN_POINT('Ctrl Pts',(-0.742761369689841,-1.,4.09799769702611));
#31548=CARTESIAN_POINT('Ctrl Pts',(-0.7447986497065,-1.,4.09045220253573));
#31549=CARTESIAN_POINT('Ctrl Pts',(-0.746800631492315,-1.,4.08290608095642));
#31550=CARTESIAN_POINT('Ctrl Pts',(-0.748767076680557,-1.,4.07535951056152));
#31551=CARTESIAN_POINT('Ctrl Pts',(-0.750697720484036,-1.,4.06781267242378));
#31552=CARTESIAN_POINT('Ctrl Pts',(-0.752592276483072,-1.,4.06026572221515));
#31553=CARTESIAN_POINT('Ctrl Pts',(-0.754450441816078,-1.,4.05271876687915));
#31554=CARTESIAN_POINT('Ctrl Pts',(-0.756271902369581,-1.,4.04517182653997));
#31555=CARTESIAN_POINT('Ctrl Pts',(-0.758056338884944,-1.,4.03762485803119));
#31556=CARTESIAN_POINT('Ctrl Pts',(-0.759803433243752,-1.,4.03007781954412));
#31557=CARTESIAN_POINT('Ctrl Pts',(-0.761512875859804,-1.,4.02253072741268));
#31558=CARTESIAN_POINT('Ctrl Pts',(-0.763184371182935,-1.,4.01498370680496));
#31559=CARTESIAN_POINT('Ctrl Pts',(-0.764817648785198,-1.,4.00743706791509));
#31560=CARTESIAN_POINT('Ctrl Pts',(-0.766412457136064,-1.,3.99989129179622));
#31561=CARTESIAN_POINT('Ctrl Pts',(-0.767968531377915,-1.,3.9923468788101));
#31562=CARTESIAN_POINT('Ctrl Pts',(-0.769485566245544,-1.,3.98480422348451));
#31563=CARTESIAN_POINT('Ctrl Pts',(-0.770963190030471,-1.,3.97726349165488));
#31564=CARTESIAN_POINT('Ctrl Pts',(-0.772400931772136,-1.,3.96972446532772));
#31565=CARTESIAN_POINT('Ctrl Pts',(-0.773798212026566,-1.,3.96218649639807));
#31566=CARTESIAN_POINT('Ctrl Pts',(-0.775154418039352,-1.,3.9546488545231));
#31567=CARTESIAN_POINT('Ctrl Pts',(-0.776468966697921,-1.,3.94711101619447));
#31568=CARTESIAN_POINT('Ctrl Pts',(-0.777741370568559,-1.,3.93957296768103));
#31569=CARTESIAN_POINT('Ctrl Pts',(-0.778971308134821,-1.,3.93203552473174));
#31570=CARTESIAN_POINT('Ctrl Pts',(-0.780158678615543,-1.,3.92450058323823));
#31571=CARTESIAN_POINT('Ctrl Pts',(-0.781303428618367,-1.,3.91697036054676));
#31572=CARTESIAN_POINT('Ctrl Pts',(-0.782405395622764,-1.,3.90944671004542));
#31573=CARTESIAN_POINT('Ctrl Pts',(-0.783464141529081,-1.,3.9019303904397));
#31574=CARTESIAN_POINT('Ctrl Pts',(-0.784478799358336,-1.,3.89442039235103));
#31575=CARTESIAN_POINT('Ctrl Pts',(-0.78544789034073,-1.,3.88691313167398));
#31576=CARTESIAN_POINT('Ctrl Pts',(-0.786369675812609,-1.,3.8794040281819));
#31577=CARTESIAN_POINT('Ctrl Pts',(-0.787242527617999,-1.,3.87188916600912));
#31578=CARTESIAN_POINT('Ctrl Pts',(-0.788065315093778,-1.,3.86436702561345));
#31579=CARTESIAN_POINT('Ctrl Pts',(-0.788837734090672,-1.,3.85683995872529));
#31580=CARTESIAN_POINT('Ctrl Pts',(-0.789560798155582,-1.,3.84931637808894));
#31581=CARTESIAN_POINT('Ctrl Pts',(-0.790236124191242,-1.,3.84180762342454));
#31582=CARTESIAN_POINT('Ctrl Pts',(-0.790865012705301,-1.,3.83432392054786));
#31583=CARTESIAN_POINT('Ctrl Pts',(-0.791447528662369,-1.,3.82687033899792));
#31584=CARTESIAN_POINT('Ctrl Pts',(-0.791981740718635,-1.,3.81944345442249));
#31585=CARTESIAN_POINT('Ctrl Pts',(-0.792462483517634,-1.,3.81202588694756));
#31586=CARTESIAN_POINT('Ctrl Pts',(-0.792882695234778,-1.,3.80459229925637));
#31587=CARTESIAN_POINT('Ctrl Pts',(-0.793235612973273,-1.,3.79711921389897));
#31588=CARTESIAN_POINT('Ctrl Pts',(-0.793516871680993,-1.,3.78959439439235));
#31589=CARTESIAN_POINT('Ctrl Pts',(-0.7937262357813,-1.,3.78202460377598));
#31590=CARTESIAN_POINT('Ctrl Pts',(-0.793870523787408,-1.,3.77444863801212));
#31591=CARTESIAN_POINT('Ctrl Pts',(-0.793961083688992,-1.,3.76692626931111));
#31592=CARTESIAN_POINT('Ctrl Pts',(-0.794008429134907,-1.,3.75951468666257));
#31593=CARTESIAN_POINT('Ctrl Pts',(-0.794017347371377,-1.,3.75224692493864));
#31594=CARTESIAN_POINT('Ctrl Pts',(-0.793982700459952,-1.,3.74511357728861));
#31595=CARTESIAN_POINT('Ctrl Pts',(-0.793882700937017,-1.,3.73803280541687));
#31596=CARTESIAN_POINT('Ctrl Pts',(-0.793682750269684,-1.,3.73086914695805));
#31597=CARTESIAN_POINT('Ctrl Pts',(-0.793347023784205,-1.,3.72348797293734));
#31598=CARTESIAN_POINT('Ctrl Pts',(-0.792848377370287,-1.,3.71580242396124));
#31599=CARTESIAN_POINT('Ctrl Pts',(-0.792177688845818,-1.,3.70781724021806));
#31600=CARTESIAN_POINT('Ctrl Pts',(-0.79135657569598,-1.,3.69968940808721));
#31601=CARTESIAN_POINT('Ctrl Pts',(-0.790436284988788,-1.,3.69172044327364));
#31602=CARTESIAN_POINT('Ctrl Pts',(-0.789483546064387,-1.,3.68428439783905));
#31603=CARTESIAN_POINT('Ctrl Pts',(-0.788569566220285,-1.,3.67777119516252));
#31604=CARTESIAN_POINT('Ctrl Pts',(-0.787758799995743,-1.,3.67252923663655));
#31605=CARTESIAN_POINT('Ctrl Pts',(-0.787145041181546,-1.,3.66907505398677));
#31606=CARTESIAN_POINT('Ctrl Pts',(-0.786774337198062,-1.,3.66743103898702));
#31607=CARTESIAN_POINT('Ctrl Pts',(-0.786565919558984,-1.,3.66680946938292));
#31608=CARTESIAN_POINT('Ctrl Pts',(-0.786459983895432,-1.,3.6666431041522));
#31609=CARTESIAN_POINT('Ctrl Pts',(-0.786422660831985,-1.,3.66661143271685));
#31610=CARTESIAN_POINT('',(-0.963899035117249,-1.,3.62400312501245));
#31611=CARTESIAN_POINT('Origin',(0.,-1.,0.));
#31612=CARTESIAN_POINT('',(-1.22531898815164,-1.,4.01728681790024));
#31613=CARTESIAN_POINT('Ctrl Pts',(-0.963899035117249,-1.,3.62400312501245));
#31614=CARTESIAN_POINT('Ctrl Pts',(-0.963880158555582,-1.,3.6240482887845));
#31615=CARTESIAN_POINT('Ctrl Pts',(-0.963861297423241,-1.,3.62424461507588));
#31616=CARTESIAN_POINT('Ctrl Pts',(-0.963957782642843,-1.,3.62489305727662));
#31617=CARTESIAN_POINT('Ctrl Pts',(-0.964373850166458,-1.,3.62652618145335));
#31618=CARTESIAN_POINT('Ctrl Pts',(-0.965395153165293,-1.,3.62988252139846));
#31619=CARTESIAN_POINT('Ctrl Pts',(-0.967052554541386,-1.,3.63492122081143));
#31620=CARTESIAN_POINT('Ctrl Pts',(-0.969195124675866,-1.,3.64113946505766));
#31621=CARTESIAN_POINT('Ctrl Pts',(-0.971722122061341,-1.,3.64819756447455));
#31622=CARTESIAN_POINT('Ctrl Pts',(-0.974519971354848,-1.,3.65571576735126));
#31623=CARTESIAN_POINT('Ctrl Pts',(-0.977478312751618,-1.,3.66333049637475));
#31624=CARTESIAN_POINT('Ctrl Pts',(-0.980505922458267,-1.,3.67074983340361));
#31625=CARTESIAN_POINT('Ctrl Pts',(-0.983550791470419,-1.,3.67782408841715));
#31626=CARTESIAN_POINT('Ctrl Pts',(-0.986602639863838,-1.,3.68455317926068));
#31627=CARTESIAN_POINT('Ctrl Pts',(-0.989676715398558,-1.,3.69102682138846));
#31628=CARTESIAN_POINT('Ctrl Pts',(-0.99280221833201,-1.,3.69738123415662));
#31629=CARTESIAN_POINT('Ctrl Pts',(-0.996009819772518,-1.,3.70375282282138));
#31630=CARTESIAN_POINT('Ctrl Pts',(-0.999317260756531,-1.,3.71022439713938));
#31631=CARTESIAN_POINT('Ctrl Pts',(-1.00272423396822,-1.,3.71680667125118));
#31632=CARTESIAN_POINT('Ctrl Pts',(-1.0062200073571,-1.,3.72346803750595));
#31633=CARTESIAN_POINT('Ctrl Pts',(-1.00978798539496,-1.,3.73015276704426));
#31634=CARTESIAN_POINT('Ctrl Pts',(-1.01341114319903,-1.,3.73680245055734));
#31635=CARTESIAN_POINT('Ctrl Pts',(-1.01707794311079,-1.,3.74337942504959));
#31636=CARTESIAN_POINT('Ctrl Pts',(-1.02078510487428,-1.,3.74987777155834));
#31637=CARTESIAN_POINT('Ctrl Pts',(-1.0245342944466,-1.,3.75631037456194));
#31638=CARTESIAN_POINT('Ctrl Pts',(-1.02833014458181,-1.,3.76270122291232));
#31639=CARTESIAN_POINT('Ctrl Pts',(-1.0321778660492,-1.,3.76907609832522));
#31640=CARTESIAN_POINT('Ctrl Pts',(-1.03608074678013,-1.,3.77545283140445));
#31641=CARTESIAN_POINT('Ctrl Pts',(-1.04003862055804,-1.,3.78183535008192));
#31642=CARTESIAN_POINT('Ctrl Pts',(-1.04404924374426,-1.,3.78821910787195));
#31643=CARTESIAN_POINT('Ctrl Pts',(-1.04810913267641,-1.,3.79459440308793));
#31644=CARTESIAN_POINT('Ctrl Pts',(-1.05221457990015,-1.,3.80095039790678));
#31645=CARTESIAN_POINT('Ctrl Pts',(-1.05636266918643,-1.,3.80727913637784));
#31646=CARTESIAN_POINT('Ctrl Pts',(-1.06055206187298,-1.,3.81357866117485));
#31647=CARTESIAN_POINT('Ctrl Pts',(-1.06478244038931,-1.,3.81985083953012));
#31648=CARTESIAN_POINT('Ctrl Pts',(-1.0690541318036,-1.,3.82609989967278));
#31649=CARTESIAN_POINT('Ctrl Pts',(-1.0733676663346,-1.,3.83233071195145));
#31650=CARTESIAN_POINT('Ctrl Pts',(-1.07772335353856,-1.,3.83854714117486));
#31651=CARTESIAN_POINT('Ctrl Pts',(-1.08212087917986,-1.,3.84475048030615));
#31652=CARTESIAN_POINT('Ctrl Pts',(-1.08655950846377,-1.,3.8509402522269));
#31653=CARTESIAN_POINT('Ctrl Pts',(-1.09103825516288,-1.,3.85711487933911));
#31654=CARTESIAN_POINT('Ctrl Pts',(-1.09555606505012,-1.,3.86327241021242));
#31655=CARTESIAN_POINT('Ctrl Pts',(-1.10011198761202,-1.,3.86941120134872));
#31656=CARTESIAN_POINT('Ctrl Pts',(-1.10470536603303,-1.,3.87553067187566));
#31657=CARTESIAN_POINT('Ctrl Pts',(-1.10933577224029,-1.,3.88163105531791));
#31658=CARTESIAN_POINT('Ctrl Pts',(-1.11400292434447,-1.,3.88771308285229));
#31659=CARTESIAN_POINT('Ctrl Pts',(-1.11870660794609,-1.,3.89377768340362));
#31660=CARTESIAN_POINT('Ctrl Pts',(-1.12344660099029,-1.,3.89982569749978));
#31661=CARTESIAN_POINT('Ctrl Pts',(-1.12822258281518,-1.,3.90585753318622));
#31662=CARTESIAN_POINT('Ctrl Pts',(-1.13303414693849,-1.,3.91187321145495));
#31663=CARTESIAN_POINT('Ctrl Pts',(-1.13788084225511,-1.,3.91787251936688));
#31664=CARTESIAN_POINT('Ctrl Pts',(-1.14276220561575,-1.,3.92385513133937));
#31665=CARTESIAN_POINT('Ctrl Pts',(-1.14767779451147,-1.,3.92982073294334));
#31666=CARTESIAN_POINT('Ctrl Pts',(-1.15262722716391,-1.,3.9357691705651));
#31667=CARTESIAN_POINT('Ctrl Pts',(-1.1576101834106,-1.,3.94170046685542));
#31668=CARTESIAN_POINT('Ctrl Pts',(-1.16262637999261,-1.,3.9476147478092));
#31669=CARTESIAN_POINT('Ctrl Pts',(-1.16767555244495,-1.,3.95351219510062));
#31670=CARTESIAN_POINT('Ctrl Pts',(-1.17275743590327,-1.,3.95939299213164));
#31671=CARTESIAN_POINT('Ctrl Pts',(-1.17787174135445,-1.,3.96525726357682));
#31672=CARTESIAN_POINT('Ctrl Pts',(-1.18301815039596,-1.,3.9711050516465));
#31673=CARTESIAN_POINT('Ctrl Pts',(-1.18819633715285,-1.,3.97693634766926));
#31674=CARTESIAN_POINT('Ctrl Pts',(-1.19340598349307,-1.,3.98275111052015));
#31675=CARTESIAN_POINT('Ctrl Pts',(-1.19864679609596,-1.,3.98854928957287));
#31676=CARTESIAN_POINT('Ctrl Pts',(-1.2039185237544,-1.,3.99433084800649));
#31677=CARTESIAN_POINT('Ctrl Pts',(-1.20922097030107,-1.,4.00009577952534));
#31678=CARTESIAN_POINT('Ctrl Pts',(-1.21455398918813,-1.,4.00584409524937));
#31679=CARTESIAN_POINT('Ctrl Pts',(-1.21884478244983,-1.,4.01042947142681));
#31680=CARTESIAN_POINT('Ctrl Pts',(-1.22207656456199,-1.,4.01386104434674));
#31681=CARTESIAN_POINT('Ctrl Pts',(-1.22423716681447,-1.,4.0161454457032));
#31682=CARTESIAN_POINT('Ctrl Pts',(-1.22531898815164,-1.,4.01728681790024));
#31683=CARTESIAN_POINT('',(-1.36999806084572,-1.,3.97027773754922));
#31684=CARTESIAN_POINT('',(-1.22531898815164,-1.,4.01728681790024));
#31685=CARTESIAN_POINT('',(-1.35032489087101,-1.,3.4984457533445));
#31686=CARTESIAN_POINT('Ctrl Pts',(-1.36999806084572,-1.,3.97027773754922));
#31687=CARTESIAN_POINT('Ctrl Pts',(-1.37020239094614,-1.,3.9687184694131));
#31688=CARTESIAN_POINT('Ctrl Pts',(-1.37060761745635,-1.,3.96560037974645));
#31689=CARTESIAN_POINT('Ctrl Pts',(-1.3712051561502,-1.,3.96092458506535));
#31690=CARTESIAN_POINT('Ctrl Pts',(-1.37198126432386,-1.,3.95469287280914));
#31691=CARTESIAN_POINT('Ctrl Pts',(-1.37291699202807,-1.,3.94690771785133));
#31692=CARTESIAN_POINT('Ctrl Pts',(-1.37381821967165,-1.,3.93912709040818));
#31693=CARTESIAN_POINT('Ctrl Pts',(-1.37468482215751,-1.,3.93135106761844));
#31694=CARTESIAN_POINT('Ctrl Pts',(-1.37551664448242,-1.,3.92357976987672));
#31695=CARTESIAN_POINT('Ctrl Pts',(-1.37631350505797,-1.,3.91581337462644));
#31696=CARTESIAN_POINT('Ctrl Pts',(-1.3770751963402,-1.,3.90805209523486));
#31697=CARTESIAN_POINT('Ctrl Pts',(-1.37780148512792,-1.,3.90029615196727));
#31698=CARTESIAN_POINT('Ctrl Pts',(-1.3784921128802,-1.,3.89254574338496));
#31699=CARTESIAN_POINT('Ctrl Pts',(-1.37914679719383,-1.,3.88480102249277));
#31700=CARTESIAN_POINT('Ctrl Pts',(-1.37976523097073,-1.,3.87706205830532));
#31701=CARTESIAN_POINT('Ctrl Pts',(-1.38034709213014,-1.,3.86932885813068));
#31702=CARTESIAN_POINT('Ctrl Pts',(-1.38089205992989,-1.,3.86160143043959));
#31703=CARTESIAN_POINT('Ctrl Pts',(-1.38139983115049,-1.,3.85387983979481));
#31704=CARTESIAN_POINT('Ctrl Pts',(-1.38187013346109,-1.,3.84616425605764));
#31705=CARTESIAN_POINT('Ctrl Pts',(-1.38230274828822,-1.,3.83845502790746));
#31706=CARTESIAN_POINT('Ctrl Pts',(-1.38269750245138,-1.,3.8307526698229));
#31707=CARTESIAN_POINT('Ctrl Pts',(-1.38305421262763,-1.,3.82305771743829));
#31708=CARTESIAN_POINT('Ctrl Pts',(-1.38337263902782,-1.,3.81537060817811));
#31709=CARTESIAN_POINT('Ctrl Pts',(-1.3836524404622,-1.,3.80769156398411));
#31710=CARTESIAN_POINT('Ctrl Pts',(-1.38389311766682,-1.,3.80002044322111));
#31711=CARTESIAN_POINT('Ctrl Pts',(-1.38409399694566,-1.,3.79235669640841));
#31712=CARTESIAN_POINT('Ctrl Pts',(-1.38425435883756,-1.,3.78469969805082));
#31713=CARTESIAN_POINT('Ctrl Pts',(-1.38437354551428,-1.,3.77704902230418));
#31714=CARTESIAN_POINT('Ctrl Pts',(-1.38445107339518,-1.,3.76940473185779));
#31715=CARTESIAN_POINT('Ctrl Pts',(-1.3844867525335,-1.,3.76176768271367));
#31716=CARTESIAN_POINT('Ctrl Pts',(-1.38448077997163,-1.,3.7541397631875));
#31717=CARTESIAN_POINT('Ctrl Pts',(-1.38443344984394,-1.,3.74652317167876));
#31718=CARTESIAN_POINT('Ctrl Pts',(-1.38434489156458,-1.,3.73891976418104));
#31719=CARTESIAN_POINT('Ctrl Pts',(-1.38421479111531,-1.,3.73133035859282));
#31720=CARTESIAN_POINT('Ctrl Pts',(-1.3840421342895,-1.,3.72375409358803));
#31721=CARTESIAN_POINT('Ctrl Pts',(-1.38382489984586,-1.,3.7161876605181));
#31722=CARTESIAN_POINT('Ctrl Pts',(-1.38356065402124,-1.,3.70862680753347));
#31723=CARTESIAN_POINT('Ctrl Pts',(-1.38324717612865,-1.,3.701067921679));
#31724=CARTESIAN_POINT('Ctrl Pts',(-1.38288311171651,-1.,3.69350967899526));
#31725=CARTESIAN_POINT('Ctrl Pts',(-1.38246852827182,-1.,3.68595444983837));
#31726=CARTESIAN_POINT('Ctrl Pts',(-1.3820057429062,-1.,3.67841038482414));
#31727=CARTESIAN_POINT('Ctrl Pts',(-1.38149812653868,-1.,3.67088843112262));
#31728=CARTESIAN_POINT('Ctrl Pts',(-1.38094856333552,-1.,3.66339848520857));
#31729=CARTESIAN_POINT('Ctrl Pts',(-1.38035791051213,-1.,3.6559455440439));
#31730=CARTESIAN_POINT('Ctrl Pts',(-1.37972372481603,-1.,3.64852652756456));
#31731=CARTESIAN_POINT('Ctrl Pts',(-1.37903818567359,-1.,3.64112507791141));
#31732=CARTESIAN_POINT('Ctrl Pts',(-1.37829035457339,-1.,3.63371727442486));
#31733=CARTESIAN_POINT('Ctrl Pts',(-1.37746987919881,-1.,3.62628098665145));
#31734=CARTESIAN_POINT('Ctrl Pts',(-1.37657053403107,-1.,3.6188048116042));
#31735=CARTESIAN_POINT('Ctrl Pts',(-1.37559314436634,-1.,3.61129546591064));
#31736=CARTESIAN_POINT('Ctrl Pts',(-1.37455051379623,-1.,3.60379020123988));
#31737=CARTESIAN_POINT('Ctrl Pts',(-1.37346320103157,-1.,3.59634627869048));
#31738=CARTESIAN_POINT('Ctrl Pts',(-1.37235053660976,-1.,3.58901853846365));
#31739=CARTESIAN_POINT('Ctrl Pts',(-1.37122241663062,-1.,3.58183885982715));
#31740=CARTESIAN_POINT('Ctrl Pts',(-1.37007229485659,-1.,3.57479875549486));
#31741=CARTESIAN_POINT('Ctrl Pts',(-1.36886584973389,-1.,3.5678208030466));
#31742=CARTESIAN_POINT('Ctrl Pts',(-1.36754771771233,-1.,3.56077662028649));
#31743=CARTESIAN_POINT('Ctrl Pts',(-1.3660614545677,-1.,3.55353883995949));
#31744=CARTESIAN_POINT('Ctrl Pts',(-1.36436666257598,-1.,3.54602591832973));
#31745=CARTESIAN_POINT('Ctrl Pts',(-1.36245507339307,-1.,3.53824396424961));
#31746=CARTESIAN_POINT('Ctrl Pts',(-1.36037259643734,-1.,3.530344649616));
#31747=CARTESIAN_POINT('Ctrl Pts',(-1.35821701528836,-1.,3.52261776116748));
#31748=CARTESIAN_POINT('Ctrl Pts',(-1.35611275237152,-1.,3.51542230699556));
#31749=CARTESIAN_POINT('Ctrl Pts',(-1.35419113575956,-1.,3.50913227059999));
#31750=CARTESIAN_POINT('Ctrl Pts',(-1.35257032843486,-1.,3.50408168106261));
#31751=CARTESIAN_POINT('Ctrl Pts',(-1.35142377279517,-1.,3.5007660381649));
#31752=CARTESIAN_POINT('Ctrl Pts',(-1.35080045218587,-1.,3.49920025459723));
#31753=CARTESIAN_POINT('Ctrl Pts',(-1.35049736560527,-1.,3.49861894124827));
#31754=CARTESIAN_POINT('Ctrl Pts',(-1.35036670892966,-1.,3.49847119623846));
#31755=CARTESIAN_POINT('Ctrl Pts',(-1.35032489087101,-1.,3.4984457533445));
#31756=CARTESIAN_POINT('',(-1.51895082866166,-1.,3.42859860294378));
#31757=CARTESIAN_POINT('Origin',(0.,-1.,0.));
#31758=CARTESIAN_POINT('',(-1.83867539237861,-1.,3.77614523045147));
#31759=CARTESIAN_POINT('Ctrl Pts',(-1.51895082866166,-1.,3.42859860294378));
#31760=CARTESIAN_POINT('Ctrl Pts',(-1.51893924967231,-1.,3.42864616361967));
#31761=CARTESIAN_POINT('Ctrl Pts',(-1.51895133295017,-1.,3.42884302333978));
#31762=CARTESIAN_POINT('Ctrl Pts',(-1.51914806898539,-1.,3.42946838852728));
#31763=CARTESIAN_POINT('Ctrl Pts',(-1.5198144909343,-1.,3.4310163189349));
#31764=CARTESIAN_POINT('Ctrl Pts',(-1.52134826724227,-1.,3.43417156977749));
#31765=CARTESIAN_POINT('Ctrl Pts',(-1.52377348950429,-1.,3.43888895974182));
#31766=CARTESIAN_POINT('Ctrl Pts',(-1.52686242875717,-1.,3.44469547527));
#31767=CARTESIAN_POINT('Ctrl Pts',(-1.530462444618,-1.,3.45127136828667));
#31768=CARTESIAN_POINT('Ctrl Pts',(-1.53440195378902,-1.,3.45825932955273));
#31769=CARTESIAN_POINT('Ctrl Pts',(-1.53851507915533,-1.,3.46531752207222));
#31770=CARTESIAN_POINT('Ctrl Pts',(-1.54266605398152,-1.,3.47217189224576));
#31771=CARTESIAN_POINT('Ctrl Pts',(-1.54678009290207,-1.,3.47868272898599));
#31772=CARTESIAN_POINT('Ctrl Pts',(-1.55084702970382,-1.,3.48485155928414));
#31773=CARTESIAN_POINT('Ctrl Pts',(-1.5548959590107,-1.,3.49076460877317));
#31774=CARTESIAN_POINT('Ctrl Pts',(-1.55897703097859,-1.,3.49655185179623));
#31775=CARTESIAN_POINT('Ctrl Pts',(-1.56314187758689,-1.,3.50234321621607));
#31776=CARTESIAN_POINT('Ctrl Pts',(-1.56742097575041,-1.,3.50821771695427));
#31777=CARTESIAN_POINT('Ctrl Pts',(-1.57181569799774,-1.,3.51418598431733));
#31778=CARTESIAN_POINT('Ctrl Pts',(-1.5763104998818,-1.,3.52021847865961));
#31779=CARTESIAN_POINT('Ctrl Pts',(-1.58088027227856,-1.,3.52626275334899));
#31780=CARTESIAN_POINT('Ctrl Pts',(-1.58549906268083,-1.,3.53226378147068));
#31781=CARTESIAN_POINT('Ctrl Pts',(-1.59014958368725,-1.,3.53818616861045));
#31782=CARTESIAN_POINT('Ctrl Pts',(-1.5948276694975,-1.,3.544024581823));
#31783=CARTESIAN_POINT('Ctrl Pts',(-1.59953698113444,-1.,3.54979148634426));
#31784=CARTESIAN_POINT('Ctrl Pts',(-1.60428584699848,-1.,3.55550985096117));
#31785=CARTESIAN_POINT('Ctrl Pts',(-1.60908344685459,-1.,3.56120432482986));
#31786=CARTESIAN_POINT('Ctrl Pts',(-1.61393581747522,-1.,3.56689200468404));
#31787=CARTESIAN_POINT('Ctrl Pts',(-1.61884340915412,-1.,3.57257679609826));
#31788=CARTESIAN_POINT('Ctrl Pts',(-1.62380329464851,-1.,3.57825455954405));
#31789=CARTESIAN_POINT('Ctrl Pts',(-1.62881051550748,-1.,3.5839162577435));
#31790=CARTESIAN_POINT('Ctrl Pts',(-1.63385971451259,-1.,3.58955176627876));
#31791=CARTESIAN_POINT('Ctrl Pts',(-1.63894676675349,-1.,3.59515368334887));
#31792=CARTESIAN_POINT('Ctrl Pts',(-1.6440700438558,-1.,3.6007202851384));
#31793=CARTESIAN_POINT('Ctrl Pts',(-1.64922952425833,-1.,3.60625346556992));
#31794=CARTESIAN_POINT('Ctrl Pts',(-1.65442619244327,-1.,3.61175734965129));
#31795=CARTESIAN_POINT('Ctrl Pts',(-1.65966133399186,-1.,3.61723666482457));
#31796=CARTESIAN_POINT('Ctrl Pts',(-1.66493585923853,-1.,3.62269517989104));
#31797=CARTESIAN_POINT('Ctrl Pts',(-1.67024966008037,-1.,3.62813422105257));
#31798=CARTESIAN_POINT('Ctrl Pts',(-1.67560193613145,-1.,3.63355343201211));
#31799=CARTESIAN_POINT('Ctrl Pts',(-1.68099146651577,-1.,3.63895140887443));
#31800=CARTESIAN_POINT('Ctrl Pts',(-1.68641690471455,-1.,3.64432638915199));
#31801=CARTESIAN_POINT('Ctrl Pts',(-1.691877054817,-1.,3.64967689827393));
#31802=CARTESIAN_POINT('Ctrl Pts',(-1.69737117722559,-1.,3.65500246526798));
#31803=CARTESIAN_POINT('Ctrl Pts',(-1.70289888566904,-1.,3.6603033877491));
#31804=CARTESIAN_POINT('Ctrl Pts',(-1.70846001610983,-1.,3.6655804319893));
#31805=CARTESIAN_POINT('Ctrl Pts',(-1.71405450210392,-1.,3.67083454901629));
#31806=CARTESIAN_POINT('Ctrl Pts',(-1.71968225581787,-1.,3.67606660374665));
#31807=CARTESIAN_POINT('Ctrl Pts',(-1.72534302437003,-1.,3.68127704936472));
#31808=CARTESIAN_POINT('Ctrl Pts',(-1.73103640956647,-1.,3.68646597019188));
#31809=CARTESIAN_POINT('Ctrl Pts',(-1.73676193254493,-1.,3.69163322647906));
#31810=CARTESIAN_POINT('Ctrl Pts',(-1.74251908492589,-1.,3.6967785691046));
#31811=CARTESIAN_POINT('Ctrl Pts',(-1.74830738046092,-1.,3.70190175673422));
#31812=CARTESIAN_POINT('Ctrl Pts',(-1.75412641804148,-1.,3.70700269736876));
#31813=CARTESIAN_POINT('Ctrl Pts',(-1.75997588499021,-1.,3.71208146346454));
#31814=CARTESIAN_POINT('Ctrl Pts',(-1.76585552124549,-1.,3.71713822377675));
#31815=CARTESIAN_POINT('Ctrl Pts',(-1.77176509401846,-1.,3.72217319911429));
#31816=CARTESIAN_POINT('Ctrl Pts',(-1.77770437039606,-1.,3.72718661205504));
#31817=CARTESIAN_POINT('Ctrl Pts',(-1.78367308442682,-1.,3.73217863095022));
#31818=CARTESIAN_POINT('Ctrl Pts',(-1.78967092823139,-1.,3.73714934729962));
#31819=CARTESIAN_POINT('Ctrl Pts',(-1.79569757859041,-1.,3.74209880351667));
#31820=CARTESIAN_POINT('Ctrl Pts',(-1.80175271485519,-1.,3.74702700874954));
#31821=CARTESIAN_POINT('Ctrl Pts',(-1.80783603939662,-1.,3.75193395888069));
#31822=CARTESIAN_POINT('Ctrl Pts',(-1.81394729834032,-1.,3.75681965683995));
#31823=CARTESIAN_POINT('Ctrl Pts',(-1.82008629694924,-1.,3.76168412709652));
#31824=CARTESIAN_POINT('Ctrl Pts',(-1.82625289221933,-1.,3.76652740355856));
#31825=CARTESIAN_POINT('Ctrl Pts',(-1.83120816956515,-1.,3.77038509819777));
#31826=CARTESIAN_POINT('Ctrl Pts',(-1.83493697935064,-1.,3.77326886065484));
#31827=CARTESIAN_POINT('Ctrl Pts',(-1.83742834010821,-1.,3.77518714458232));
#31828=CARTESIAN_POINT('Ctrl Pts',(-1.83867539237861,-1.,3.77614523045147));
#31829=CARTESIAN_POINT('',(-1.97421938526992,-1.,3.70708211654725));
#31830=CARTESIAN_POINT('',(-1.83867539237861,-1.,3.77614523045147));
#31831=CARTESIAN_POINT('',(-1.88097764062542,-1.,3.24413672884902));
#31832=CARTESIAN_POINT('Ctrl Pts',(-1.97421938526992,-1.,3.70708211654725));
#31833=CARTESIAN_POINT('Ctrl Pts',(-1.974177276451,-1.,3.7055100813194));
#31834=CARTESIAN_POINT('Ctrl Pts',(-1.97408973726149,-1.,3.70236698911837));
#31835=CARTESIAN_POINT('Ctrl Pts',(-1.97394846382289,-1.,3.69765528558292));
#31836=CARTESIAN_POINT('Ctrl Pts',(-1.97374016224397,-1.,3.69137888597855));
#31837=CARTESIAN_POINT('Ctrl Pts',(-1.97344650303631,-1.,3.68354319913416));
#31838=CARTESIAN_POINT('Ctrl Pts',(-1.97311947678035,-1.,3.67571738106175));
#31839=CARTESIAN_POINT('Ctrl Pts',(-1.9727589719863,-1.,3.66790152751984));
#31840=CARTESIAN_POINT('Ctrl Pts',(-1.97236485439317,-1.,3.66009578166865));
#31841=CARTESIAN_POINT('Ctrl Pts',(-1.97193697240645,-1.,3.65230034717364));
#31842=CARTESIAN_POINT('Ctrl Pts',(-1.97147515441539,-1.,3.64451546724221));
#31843=CARTESIAN_POINT('Ctrl Pts',(-1.97097920454698,-1.,3.63674139590853));
#31844=CARTESIAN_POINT('Ctrl Pts',(-1.97044889850518,-1.,3.62897836973397));
#31845=CARTESIAN_POINT('Ctrl Pts',(-1.96988398129888,-1.,3.62122658401722));
#31846=CARTESIAN_POINT('Ctrl Pts',(-1.96928416040712,-1.,3.61348615496393));
#31847=CARTESIAN_POINT('Ctrl Pts',(-1.96864911885775,-1.,3.60575714017676));
#31848=CARTESIAN_POINT('Ctrl Pts',(-1.96797854118257,-1.,3.59803959819725));
#31849=CARTESIAN_POINT('Ctrl Pts',(-1.96727213799507,-1.,3.5903336402273));
#31850=CARTESIAN_POINT('Ctrl Pts',(-1.9665296668894,-1.,3.58263947663884));
#31851=CARTESIAN_POINT('Ctrl Pts',(-1.96575096652857,-1.,3.57495748601088));
#31852=CARTESIAN_POINT('Ctrl Pts',(-1.96493594634643,-1.,3.56728820357933));
#31853=CARTESIAN_POINT('Ctrl Pts',(-1.96408450906868,-1.,3.55963218706201));
#31854=CARTESIAN_POINT('Ctrl Pts',(-1.96319648628667,-1.,3.55198990600929));
#31855=CARTESIAN_POINT('Ctrl Pts',(-1.96227157573058,-1.,3.54436163300425));
#31856=CARTESIAN_POINT('Ctrl Pts',(-1.96130926212661,-1.,3.53674730625759));
#31857=CARTESIAN_POINT('Ctrl Pts',(-1.96030879411534,-1.,3.52914648844289));
#31858=CARTESIAN_POINT('Ctrl Pts',(-1.95926936324436,-1.,3.52155867431438));
#31859=CARTESIAN_POINT('Ctrl Pts',(-1.95819025316768,-1.,3.51398354617772));
#31860=CARTESIAN_POINT('Ctrl Pts',(-1.95707099606514,-1.,3.50642124159913));
#31861=CARTESIAN_POINT('Ctrl Pts',(-1.9559115382367,-1.,3.49887263575602));
#31862=CARTESIAN_POINT('Ctrl Pts',(-1.95471236969653,-1.,3.49133956289154));
#31863=CARTESIAN_POINT('Ctrl Pts',(-1.95347412486316,-1.,3.48382414832648));
#31864=CARTESIAN_POINT('Ctrl Pts',(-1.95219722189878,-1.,3.47632820495926));
#31865=CARTESIAN_POINT('Ctrl Pts',(-1.95088147859876,-1.,3.4688525897419));
#31866=CARTESIAN_POINT('Ctrl Pts',(-1.94952575850196,-1.,3.46139661060959));
#31867=CARTESIAN_POINT('Ctrl Pts',(-1.94812754766524,-1.,3.45395731584051));
#31868=CARTESIAN_POINT('Ctrl Pts',(-1.94668377715332,-1.,3.44653088665685));
#31869=CARTESIAN_POINT('Ctrl Pts',(-1.94519168842883,-1.,3.43911410197693));
#31870=CARTESIAN_POINT('Ctrl Pts',(-1.94364973660285,-1.,3.43170586602436));
#31871=CARTESIAN_POINT('Ctrl Pts',(-1.94205835913692,-1.,3.42430850941497));
#31872=CARTESIAN_POINT('Ctrl Pts',(-1.94042111965237,-1.,3.41692971994082));
#31873=CARTESIAN_POINT('Ctrl Pts',(-1.93874306008132,-1.,3.40957978266622));
#31874=CARTESIAN_POINT('Ctrl Pts',(-1.93702857723089,-1.,3.40226802104093));
#31875=CARTESIAN_POINT('Ctrl Pts',(-1.93527929945982,-1.,3.39499923640789));
#31876=CARTESIAN_POINT('Ctrl Pts',(-1.93349233176794,-1.,3.38777076883267));
#31877=CARTESIAN_POINT('Ctrl Pts',(-1.93165739093292,-1.,3.38056768525577));
#31878=CARTESIAN_POINT('Ctrl Pts',(-1.92975993109897,-1.,3.37336807068078));
#31879=CARTESIAN_POINT('Ctrl Pts',(-1.92778626543803,-1.,3.36615168657597));
#31880=CARTESIAN_POINT('Ctrl Pts',(-1.92572846125763,-1.,3.35890824422976));
#31881=CARTESIAN_POINT('Ctrl Pts',(-1.92358838440518,-1.,3.35164424847206));
#31882=CARTESIAN_POINT('Ctrl Pts',(-1.92138450828378,-1.,3.34439448941915));
#31883=CARTESIAN_POINT('Ctrl Pts',(-1.91914609610173,-1.,3.33721230709948));
#31884=CARTESIAN_POINT('Ctrl Pts',(-1.91690081930297,-1.,3.33014884257812));
#31885=CARTESIAN_POINT('Ctrl Pts',(-1.91466343916612,-1.,3.32323403454507));
#31886=CARTESIAN_POINT('Ctrl Pts',(-1.91242616234459,-1.,3.31646052426395));
#31887=CARTESIAN_POINT('Ctrl Pts',(-1.91014297830502,-1.,3.30975721158694));
#31888=CARTESIAN_POINT('Ctrl Pts',(-1.90773912171424,-1.,3.30300595568341));
#31889=CARTESIAN_POINT('Ctrl Pts',(-1.9051389186417,-1.,3.29608978722258));
#31890=CARTESIAN_POINT('Ctrl Pts',(-1.9022897124757,-1.,3.28893448600364));
#31891=CARTESIAN_POINT('Ctrl Pts',(-1.89918429230425,-1.,3.28154737912287));
#31892=CARTESIAN_POINT('Ctrl Pts',(-1.89589172903662,-1.,3.27407108932908));
#31893=CARTESIAN_POINT('Ctrl Pts',(-1.89255393500769,-1.,3.2667765388833));
#31894=CARTESIAN_POINT('Ctrl Pts',(-1.88934996203508,-1.,3.2599988519361));
#31895=CARTESIAN_POINT('Ctrl Pts',(-1.88646802523372,-1.,3.25408686339298));
#31896=CARTESIAN_POINT('Ctrl Pts',(-1.88407708646435,-1.,3.24935200512055));
#31897=CARTESIAN_POINT('Ctrl Pts',(-1.88242596600422,-1.,3.24625654410705));
#31898=CARTESIAN_POINT('Ctrl Pts',(-1.88156537699118,-1.,3.24480754675942));
#31899=CARTESIAN_POINT('Ctrl Pts',(-1.88117508446657,-1.,3.24428080352952));
#31900=CARTESIAN_POINT('Ctrl Pts',(-1.88102292397987,-1.,3.2441553167131));
#31901=CARTESIAN_POINT('Ctrl Pts',(-1.88097764062542,-1.,3.24413672884902));
#31902=CARTESIAN_POINT('',(-2.03660101169564,-1.,3.14877060440425));
#31903=CARTESIAN_POINT('Origin',(0.,-1.,0.));
#31904=CARTESIAN_POINT('',(-2.40675750623143,-1.,3.44202241512147));
#31905=CARTESIAN_POINT('Ctrl Pts',(-2.03660101169564,-1.,3.14877060440425));
#31906=CARTESIAN_POINT('Ctrl Pts',(-2.03659701539175,-1.,3.1488193908823));
#31907=CARTESIAN_POINT('Ctrl Pts',(-2.03663974554941,-1.,3.14901193669147));
#31908=CARTESIAN_POINT('Ctrl Pts',(-2.03693188810614,-1.,3.14959882629936));
#31909=CARTESIAN_POINT('Ctrl Pts',(-2.03783225496023,-1.,3.15102344775396));
#31910=CARTESIAN_POINT('Ctrl Pts',(-2.03984073791432,-1.,3.1538999167466));
#31911=CARTESIAN_POINT('Ctrl Pts',(-2.04297406404132,-1.,3.15817983946525));
#31912=CARTESIAN_POINT('Ctrl Pts',(-2.0469333124766,-1.,3.16343165059235));
#31913=CARTESIAN_POINT('Ctrl Pts',(-2.05151770247452,-1.,3.16936341689859));
#31914=CARTESIAN_POINT('Ctrl Pts',(-2.05650186773279,-1.,3.17564906975592));
#31915=CARTESIAN_POINT('Ctrl Pts',(-2.06166849827143,-1.,3.18197692964677));
#31916=CARTESIAN_POINT('Ctrl Pts',(-2.06684062744065,-1.,3.18809755562297));
#31917=CARTESIAN_POINT('Ctrl Pts',(-2.07192253497765,-1.,3.19388465568113));
#31918=CARTESIAN_POINT('Ctrl Pts',(-2.0769044187063,-1.,3.19934132835879));
#31919=CARTESIAN_POINT('Ctrl Pts',(-2.08182850370816,-1.,3.20454818630635));
#31920=CARTESIAN_POINT('Ctrl Pts',(-2.08676465517435,-1.,3.20962575845433));
#31921=CARTESIAN_POINT('Ctrl Pts',(-2.0917841946046,-1.,3.2146942960168));
#31922=CARTESIAN_POINT('Ctrl Pts',(-2.09692958434933,-1.,3.21982707347067));
#31923=CARTESIAN_POINT('Ctrl Pts',(-2.10220384298533,-1.,3.22503437553496));
#31924=CARTESIAN_POINT('Ctrl Pts',(-2.1075869964248,-1.,3.23028945793334));
#31925=CARTESIAN_POINT('Ctrl Pts',(-2.11304604021784,-1.,3.23554444767115));
#31926=CARTESIAN_POINT('Ctrl Pts',(-2.11854673326972,-1.,3.24074905517282));
#31927=CARTESIAN_POINT('Ctrl Pts',(-2.12406646410943,-1.,3.24587102613347));
#31928=CARTESIAN_POINT('Ctrl Pts',(-2.1296002839681,-1.,3.25090574493994));
#31929=CARTESIAN_POINT('Ctrl Pts',(-2.13515375878786,-1.,3.25586495065027));
#31930=CARTESIAN_POINT('Ctrl Pts',(-2.14073870754257,-1.,3.26077002641868));
#31931=CARTESIAN_POINT('Ctrl Pts',(-2.14636805295663,-1.,3.26564388189764));
#31932=CARTESIAN_POINT('Ctrl Pts',(-2.15205043199818,-1.,3.27050245897244));
#31933=CARTESIAN_POINT('Ctrl Pts',(-2.15778690038359,-1.,3.27534954469206));
#31934=CARTESIAN_POINT('Ctrl Pts',(-2.16357391934434,-1.,3.28018150841414));
#31935=CARTESIAN_POINT('Ctrl Pts',(-2.16940517773459,-1.,3.2849901997973));
#31936=CARTESIAN_POINT('Ctrl Pts',(-2.17527380048422,-1.,3.28976645712566));
#31937=CARTESIAN_POINT('Ctrl Pts',(-2.18117455557062,-1.,3.29450361500484));
#31938=CARTESIAN_POINT('Ctrl Pts',(-2.18710556500325,-1.,3.29920022557635));
#31939=CARTESIAN_POINT('Ctrl Pts',(-2.19306710376112,-1.,3.30385816281831));
#31940=CARTESIAN_POINT('Ctrl Pts',(-2.19906078949924,-1.,3.30848134694596));
#31941=CARTESIAN_POINT('Ctrl Pts',(-2.20508863150608,-1.,3.3130742460895));
#31942=CARTESIAN_POINT('Ctrl Pts',(-2.21115211847872,-1.,3.31764044024231));
#31943=CARTESIAN_POINT('Ctrl Pts',(-2.21725135110889,-1.,3.32218125618955));
#31944=CARTESIAN_POINT('Ctrl Pts',(-2.22338548312758,-1.,3.32669646722871));
#31945=CARTESIAN_POINT('Ctrl Pts',(-2.22955308907221,-1.,3.33118487773593));
#31946=CARTESIAN_POINT('Ctrl Pts',(-2.2357525632881,-1.,3.33564495756478));
#31947=CARTESIAN_POINT('Ctrl Pts',(-2.24198249391437,-1.,3.34007543738044));
#31948=CARTESIAN_POINT('Ctrl Pts',(-2.24824207678288,-1.,3.34447596770768));
#31949=CARTESIAN_POINT('Ctrl Pts',(-2.25453097693524,-1.,3.34884690292342));
#31950=CARTESIAN_POINT('Ctrl Pts',(-2.26084915222484,-1.,3.35318902552676));
#31951=CARTESIAN_POINT('Ctrl Pts',(-2.26719668579921,-1.,3.35750328523077));
#31952=CARTESIAN_POINT('Ctrl Pts',(-2.27357362620902,-1.,3.36179055004369));
#31953=CARTESIAN_POINT('Ctrl Pts',(-2.27997979457968,-1.,3.36605130712978));
#31954=CARTESIAN_POINT('Ctrl Pts',(-2.28641481081045,-1.,3.37028570206357));
#31955=CARTESIAN_POINT('Ctrl Pts',(-2.2928781800731,-1.,3.37449367172707));
#31956=CARTESIAN_POINT('Ctrl Pts',(-2.29936936127588,-1.,3.37867504959382));
#31957=CARTESIAN_POINT('Ctrl Pts',(-2.30588783640389,-1.,3.38282967336676));
#31958=CARTESIAN_POINT('Ctrl Pts',(-2.31243319489505,-1.,3.38695751492659));
#31959=CARTESIAN_POINT('Ctrl Pts',(-2.31900513925627,-1.,3.39105869475112));
#31960=CARTESIAN_POINT('Ctrl Pts',(-2.32560343902683,-1.,3.39513342020045));
#31961=CARTESIAN_POINT('Ctrl Pts',(-2.33222789882601,-1.,3.39918194578115));
#31962=CARTESIAN_POINT('Ctrl Pts',(-2.33887832342715,-1.,3.40320452776646));
#31963=CARTESIAN_POINT('Ctrl Pts',(-2.34555447648901,-1.,3.40720137403888));
#31964=CARTESIAN_POINT('Ctrl Pts',(-2.35225606823649,-1.,3.41117262313464));
#31965=CARTESIAN_POINT('Ctrl Pts',(-2.35898278606449,-1.,3.4151183675076));
#31966=CARTESIAN_POINT('Ctrl Pts',(-2.36573431470314,-1.,3.41903866635384));
#31967=CARTESIAN_POINT('Ctrl Pts',(-2.37251035954351,-1.,3.42293356216595));
#31968=CARTESIAN_POINT('Ctrl Pts',(-2.37931067029517,-1.,3.42680309755241));
#31969=CARTESIAN_POINT('Ctrl Pts',(-2.38613505844641,-1.,3.43064732714472));
#31970=CARTESIAN_POINT('Ctrl Pts',(-2.39298338805823,-1.,3.43446630680436));
#31971=CARTESIAN_POINT('Ctrl Pts',(-2.39848113411429,-1.,3.43750133066036));
#31972=CARTESIAN_POINT('Ctrl Pts',(-2.40261515590099,-1.,3.43976627485223));
#31973=CARTESIAN_POINT('Ctrl Pts',(-2.40537592959345,-1.,3.44127120683402));
#31974=CARTESIAN_POINT('Ctrl Pts',(-2.40675750623143,-1.,3.44202241512147));
#31975=CARTESIAN_POINT('',(-2.52982887637028,-1.,3.35260583073571));
#31976=CARTESIAN_POINT('',(-2.40675750623143,-1.,3.44202241512147));
#31977=CARTESIAN_POINT('',(-2.36531447826073,-1.,2.90994629141676));
#31978=CARTESIAN_POINT('Ctrl Pts',(-2.52982887637028,-1.,3.35260583073571));
#31979=CARTESIAN_POINT('Ctrl Pts',(-2.5295413654909,-1.,3.35105973714071));
#31980=CARTESIAN_POINT('Ctrl Pts',(-2.52896321610703,-1.,3.34796903576663));
#31981=CARTESIAN_POINT('Ctrl Pts',(-2.52808660915689,-1.,3.34333744115511));
#31982=CARTESIAN_POINT('Ctrl Pts',(-2.52689902690158,-1.,3.33717089999103));
#31983=CARTESIAN_POINT('Ctrl Pts',(-2.52538321164634,-1.,3.32947762187533));
#31984=CARTESIAN_POINT('Ctrl Pts',(-2.5238359839626,-1.,3.32179931078699));
#31985=CARTESIAN_POINT('Ctrl Pts',(-2.52225724871313,-1.,3.31413607874645));
#31986=CARTESIAN_POINT('Ctrl Pts',(-2.52064689568511,-1.,3.30648808815442));
#31987=CARTESIAN_POINT('Ctrl Pts',(-2.51900480701069,-1.,3.29885556388352));
#31988=CARTESIAN_POINT('Ctrl Pts',(-2.51733085123797,-1.,3.2912387729927));
#31989=CARTESIAN_POINT('Ctrl Pts',(-2.51562487464514,-1.,3.28363799702982));
#31990=CARTESIAN_POINT('Ctrl Pts',(-2.513886692704,-1.,3.27605350473142));
#31991=CARTESIAN_POINT('Ctrl Pts',(-2.51211608411423,-1.,3.26848552888115));
#31992=CARTESIAN_POINT('Ctrl Pts',(-2.51031277813486,-1.,3.26093423001434));
#31993=CARTESIAN_POINT('Ctrl Pts',(-2.50847647070723,-1.,3.25339971460982));
#31994=CARTESIAN_POINT('Ctrl Pts',(-2.506606859405,-1.,3.24588208983849));
#31995=CARTESIAN_POINT('Ctrl Pts',(-2.5047036758003,-1.,3.23838151080319));
#31996=CARTESIAN_POINT('Ctrl Pts',(-2.50276671338111,-1.,3.23089822320646));
#31997=CARTESIAN_POINT('Ctrl Pts',(-2.50079587201957,-1.,3.22343262620503));
#31998=CARTESIAN_POINT('Ctrl Pts',(-2.4987911459939,-1.,3.21598526261286));
#31999=CARTESIAN_POINT('Ctrl Pts',(-2.4967525264737,-1.,3.20855669849836));
#32000=CARTESIAN_POINT('Ctrl Pts',(-2.49467992057755,-1.,3.20114742397588));
#32001=CARTESIAN_POINT('Ctrl Pts',(-2.49257307239848,-1.,3.19375775555798));
#32002=CARTESIAN_POINT('Ctrl Pts',(-2.49043146334059,-1.,3.18638771282266));
#32003=CARTESIAN_POINT('Ctrl Pts',(-2.48825428288201,-1.,3.17903698136622));
#32004=CARTESIAN_POINT('Ctrl Pts',(-2.48604065348587,-1.,3.17170518863313));
#32005=CARTESIAN_POINT('Ctrl Pts',(-2.48378981792725,-1.,3.16439213290161));
#32006=CARTESIAN_POINT('Ctrl Pts',(-2.48150133566571,-1.,3.15709802322739));
#32007=CARTESIAN_POINT('Ctrl Pts',(-2.47917529057029,-1.,3.14982373241352));
#32008=CARTESIAN_POINT('Ctrl Pts',(-2.47681245356109,-1.,3.1425709954655));
#32009=CARTESIAN_POINT('Ctrl Pts',(-2.47441378371932,-1.,3.13534181229295));
#32010=CARTESIAN_POINT('Ctrl Pts',(-2.47197997765871,-1.,3.12813790805952));
#32011=CARTESIAN_POINT('Ctrl Pts',(-2.46951098947469,-1.,3.12096015766983));
#32012=CARTESIAN_POINT('Ctrl Pts',(-2.46700558843506,-1.,3.11380805536122));
#32013=CARTESIAN_POINT('Ctrl Pts',(-2.46446082979646,-1.,3.1066790790198));
#32014=CARTESIAN_POINT('Ctrl Pts',(-2.46187308501884,-1.,3.09956993697052));
#32015=CARTESIAN_POINT('Ctrl Pts',(-2.4592391256388,-1.,3.09247787931887));
#32016=CARTESIAN_POINT('Ctrl Pts',(-2.45655725437039,-1.,3.08540206545315));
#32017=CARTESIAN_POINT('Ctrl Pts',(-2.4538282678779,-1.,3.07834472886139));
#32018=CARTESIAN_POINT('Ctrl Pts',(-2.45105688854422,-1.,3.07131290521297));
#32019=CARTESIAN_POINT('Ctrl Pts',(-2.44824970516544,-1.,3.06431596421405));
#32020=CARTESIAN_POINT('Ctrl Pts',(-2.44541251892556,-1.,3.05736242671506));
#32021=CARTESIAN_POINT('Ctrl Pts',(-2.44254768923105,-1.,3.05045678021504));
#32022=CARTESIAN_POINT('Ctrl Pts',(-2.43965194061857,-1.,3.04359685040555));
#32023=CARTESIAN_POINT('Ctrl Pts',(-2.43671278042414,-1.,3.03676949672821));
#32024=CARTESIAN_POINT('Ctrl Pts',(-2.43371241361488,-1.,3.02995534946978));
#32025=CARTESIAN_POINT('Ctrl Pts',(-2.43063415586637,-1.,3.02313656036004));
#32026=CARTESIAN_POINT('Ctrl Pts',(-2.42746856264168,-1.,3.01630420830504));
#32027=CARTESIAN_POINT('Ctrl Pts',(-2.42421849439613,-1.,3.00946442616658));
#32028=CARTESIAN_POINT('Ctrl Pts',(-2.42090763946779,-1.,3.00264868585996));
#32029=CARTESIAN_POINT('Ctrl Pts',(-2.41757324500514,-1.,2.99590509293503));
#32030=CARTESIAN_POINT('Ctrl Pts',(-2.41425064199586,-1.,2.98927983005796));
#32031=CARTESIAN_POINT('Ctrl Pts',(-2.41095909342571,-1.,2.98280015815107));
#32032=CARTESIAN_POINT('Ctrl Pts',(-2.40768975073713,-1.,2.97646002822422));
#32033=CARTESIAN_POINT('Ctrl Pts',(-2.40438604734919,-1.,2.9701964131236));
#32034=CARTESIAN_POINT('Ctrl Pts',(-2.4009556571164,-1.,2.96390432240312));
#32035=CARTESIAN_POINT('Ctrl Pts',(-2.39730553974517,-1.,2.95748006482942));
#32036=CARTESIAN_POINT('Ctrl Pts',(-2.39337207631667,-1.,2.95085857128439));
#32037=CARTESIAN_POINT('Ctrl Pts',(-2.38914929090759,-1.,2.94404820669076));
#32038=CARTESIAN_POINT('Ctrl Pts',(-2.38472771516311,-1.,2.93717903280391));
#32039=CARTESIAN_POINT('Ctrl Pts',(-2.38028989582073,-1.,2.93049643640206));
#32040=CARTESIAN_POINT('Ctrl Pts',(-2.3760651052403,-1.,2.92430340582608));
#32041=CARTESIAN_POINT('Ctrl Pts',(-2.37229381109821,-1.,2.91891503791411));
#32042=CARTESIAN_POINT('Ctrl Pts',(-2.36919161373173,-1.,2.9146124988314));
#32043=CARTESIAN_POINT('Ctrl Pts',(-2.36707658451664,-1.,2.91181344022549));
#32044=CARTESIAN_POINT('Ctrl Pts',(-2.36599991765749,-1.,2.91051690822156));
#32045=CARTESIAN_POINT('Ctrl Pts',(-2.36553202948613,-1.,2.91005770527719));
#32046=CARTESIAN_POINT('Ctrl Pts',(-2.36536211188453,-1.,2.90995756655606));
#32047=CARTESIAN_POINT('Ctrl Pts',(-2.36531447826074,-1.,2.90994629141676));
#32048=CARTESIAN_POINT('',(-2.50410331873042,-1.,2.79140942341378));
#32049=CARTESIAN_POINT('Origin',(0.,-1.,0.));
#32050=CARTESIAN_POINT('',(-2.91557726271063,-1.,3.02314558451372));
#32051=CARTESIAN_POINT('Ctrl Pts',(-2.50410331873042,-1.,2.79140942341378));
#32052=CARTESIAN_POINT('Ctrl Pts',(-2.50410700351426,-1.,2.79145823440899));
#32053=CARTESIAN_POINT('Ctrl Pts',(-2.50417932839343,-1.,2.79164172519039));
#32054=CARTESIAN_POINT('Ctrl Pts',(-2.50455968395235,-1.,2.79217568804874));
#32055=CARTESIAN_POINT('Ctrl Pts',(-2.50567182569153,-1.,2.79344192164204));
#32056=CARTESIAN_POINT('Ctrl Pts',(-2.50810555977564,-1.,2.7959687805717));
#32057=CARTESIAN_POINT('Ctrl Pts',(-2.51186983687947,-1.,2.79970585014308));
#32058=CARTESIAN_POINT('Ctrl Pts',(-2.51660190466067,-1.,2.80427363984939));
#32059=CARTESIAN_POINT('Ctrl Pts',(-2.52205778589922,-1.,2.80941521967234));
#32060=CARTESIAN_POINT('Ctrl Pts',(-2.52796388055457,-1.,2.8148437904867));
#32061=CARTESIAN_POINT('Ctrl Pts',(-2.53405679667463,-1.,2.82028550483744));
#32062=CARTESIAN_POINT('Ctrl Pts',(-2.54012272520141,-1.,2.82552167649157));
#32063=CARTESIAN_POINT('Ctrl Pts',(-2.54604736792542,-1.,2.83044254225794));
#32064=CARTESIAN_POINT('Ctrl Pts',(-2.55182152806964,-1.,2.83505269592412));
#32065=CARTESIAN_POINT('Ctrl Pts',(-2.55749952145165,-1.,2.83942515220699));
#32066=CARTESIAN_POINT('Ctrl Pts',(-2.56316920798489,-1.,2.84366802680211));
#32067=CARTESIAN_POINT('Ctrl Pts',(-2.56891984251743,-1.,2.84788893329091));
#32068=CARTESIAN_POINT('Ctrl Pts',(-2.57480482727128,-1.,2.85215360144483));
#32069=CARTESIAN_POINT('Ctrl Pts',(-2.58082875254407,-1.,2.85647171715147));
#32070=CARTESIAN_POINT('Ctrl Pts',(-2.5869677064356,-1.,2.86081999003668));
#32071=CARTESIAN_POINT('Ctrl Pts',(-2.59318160184921,-1.,2.86515629953528));
#32072=CARTESIAN_POINT('Ctrl Pts',(-2.59942875223202,-1.,2.86943633170712));
#32073=CARTESIAN_POINT('Ctrl Pts',(-2.6056817788128,-1.,2.87363176656475));
#32074=CARTESIAN_POINT('Ctrl Pts',(-2.61193507170928,-1.,2.87773881947885));
#32075=CARTESIAN_POINT('Ctrl Pts',(-2.61819596473087,-1.,2.88176821427502));
#32076=CARTESIAN_POINT('Ctrl Pts',(-2.62447947640253,-1.,2.88573922195049));
#32077=CARTESIAN_POINT('Ctrl Pts',(-2.63080195420771,-1.,2.88967244854243));
#32078=CARTESIAN_POINT('Ctrl Pts',(-2.63717442263944,-1.,2.89358228854557));
#32079=CARTESIAN_POINT('Ctrl Pts',(-2.64359851684146,-1.,2.89747231723361));
#32080=CARTESIAN_POINT('Ctrl Pts',(-2.65007017365576,-1.,2.90133950224879));
#32081=CARTESIAN_POINT('Ctrl Pts',(-2.65658188464287,-1.,2.90517678087467));
#32082=CARTESIAN_POINT('Ctrl Pts',(-2.66312542616809,-1.,2.90897617968921));
#32083=CARTESIAN_POINT('Ctrl Pts',(-2.66969458792627,-1.,2.91273193382876));
#32084=CARTESIAN_POINT('Ctrl Pts',(-2.67628728855309,-1.,2.91644290704281));
#32085=CARTESIAN_POINT('Ctrl Pts',(-2.68290409279689,-1.,2.92011090722152));
#32086=CARTESIAN_POINT('Ctrl Pts',(-2.68954721165342,-1.,2.92373955325876));
#32087=CARTESIAN_POINT('Ctrl Pts',(-2.69621932864302,-1.,2.92733294395268));
#32088=CARTESIAN_POINT('Ctrl Pts',(-2.70292247416881,-1.,2.93089438233746));
#32089=CARTESIAN_POINT('Ctrl Pts',(-2.70965695523776,-1.,2.93442516311168));
#32090=CARTESIAN_POINT('Ctrl Pts',(-2.71642190053575,-1.,2.93792519474955));
#32091=CARTESIAN_POINT('Ctrl Pts',(-2.72321571511322,-1.,2.94139351933882));
#32092=CARTESIAN_POINT('Ctrl Pts',(-2.73003657371613,-1.,2.94482887675139));
#32093=CARTESIAN_POINT('Ctrl Pts',(-2.73688288329825,-1.,2.94823023414381));
#32094=CARTESIAN_POINT('Ctrl Pts',(-2.7437537949221,-1.,2.95159737214305));
#32095=CARTESIAN_POINT('Ctrl Pts',(-2.75064903318996,-1.,2.95493069316211));
#32096=CARTESIAN_POINT('Ctrl Pts',(-2.75756867888393,-1.,2.9582309766594));
#32097=CARTESIAN_POINT('Ctrl Pts',(-2.76451296269571,-1.,2.96149914764832));
#32098=CARTESIAN_POINT('Ctrl Pts',(-2.77148206836464,-1.,2.96473605585548));
#32099=CARTESIAN_POINT('Ctrl Pts',(-2.77847589542767,-1.,2.9679422104295));
#32100=CARTESIAN_POINT('Ctrl Pts',(-2.78549409123657,-1.,2.97111781461349));
#32101=CARTESIAN_POINT('Ctrl Pts',(-2.79253615718147,-1.,2.97426288347475));
#32102=CARTESIAN_POINT('Ctrl Pts',(-2.79960153278186,-1.,2.97737733718242));
#32103=CARTESIAN_POINT('Ctrl Pts',(-2.80668968101162,-1.,2.98046109647299));
#32104=CARTESIAN_POINT('Ctrl Pts',(-2.81380019196454,-1.,2.9835141977994));
#32105=CARTESIAN_POINT('Ctrl Pts',(-2.82093279065704,-1.,2.98653680669434));
#32106=CARTESIAN_POINT('Ctrl Pts',(-2.82808728190402,-1.,2.98952916401699));
#32107=CARTESIAN_POINT('Ctrl Pts',(-2.83526351254383,-1.,2.99249155170479));
#32108=CARTESIAN_POINT('Ctrl Pts',(-2.84246132984334,-1.,2.995424253416));
#32109=CARTESIAN_POINT('Ctrl Pts',(-2.84968053289104,-1.,2.99832751144566));
#32110=CARTESIAN_POINT('Ctrl Pts',(-2.85692085715129,-1.,3.0012015079552));
#32111=CARTESIAN_POINT('Ctrl Pts',(-2.86418200833065,-1.,3.00404638316245));
#32112=CARTESIAN_POINT('Ctrl Pts',(-2.87146368430104,-1.,3.00686224485374));
#32113=CARTESIAN_POINT('Ctrl Pts',(-2.87876560072799,-1.,3.0096491810855));
#32114=CARTESIAN_POINT('Ctrl Pts',(-2.88608751706796,-1.,3.01240727309568));
#32115=CARTESIAN_POINT('Ctrl Pts',(-2.8934292556764,-1.,3.01513660433291));
#32116=CARTESIAN_POINT('Ctrl Pts',(-2.90079069102661,-1.,3.01783725123646));
#32117=CARTESIAN_POINT('Ctrl Pts',(-2.90669553303902,-1.,3.01997487194926));
#32118=CARTESIAN_POINT('Ctrl Pts',(-2.91113297349052,-1.,3.02156522743299));
#32119=CARTESIAN_POINT('Ctrl Pts',(-2.91409518070707,-1.,3.02261975104912));
#32120=CARTESIAN_POINT('Ctrl Pts',(-2.91557726271063,-1.,3.02314558451372));
#32121=CARTESIAN_POINT('',(-3.02314558451372,-1.,2.91557726271063));
#32122=CARTESIAN_POINT('',(-2.91557726271063,-1.,3.02314558451372));
#32123=CARTESIAN_POINT('',(-2.79140942341258,-1.,2.50410331873176));
#32124=CARTESIAN_POINT('Ctrl Pts',(-3.02314558451372,-1.,2.91557726271063));
#32125=CARTESIAN_POINT('Ctrl Pts',(-3.02261975104593,-1.,2.91409518070399));
#32126=CARTESIAN_POINT('Ctrl Pts',(-3.02156522742431,-1.,2.91113297348212));
#32127=CARTESIAN_POINT('Ctrl Pts',(-3.01997487193503,-1.,2.90669553302526));
#32128=CARTESIAN_POINT('Ctrl Pts',(-3.01783725121981,-1.,2.9007906910105));
#32129=CARTESIAN_POINT('Ctrl Pts',(-3.01513660431928,-1.,2.89342925566321));
#32130=CARTESIAN_POINT('Ctrl Pts',(-3.01240727308829,-1.,2.8860875170608));
#32131=CARTESIAN_POINT('Ctrl Pts',(-3.00964918108476,-1.,2.87876560072727));
#32132=CARTESIAN_POINT('Ctrl Pts',(-3.00686224485784,-1.,2.87146368430502));
#32133=CARTESIAN_POINT('Ctrl Pts',(-3.00404638316867,-1.,2.86418200833667));
#32134=CARTESIAN_POINT('Ctrl Pts',(-3.00120150796095,-1.,2.85692085715686));
#32135=CARTESIAN_POINT('Ctrl Pts',(-2.99832751144925,-1.,2.84968053289451));
#32136=CARTESIAN_POINT('Ctrl Pts',(-2.99542425341685,-1.,2.84246132984415));
#32137=CARTESIAN_POINT('Ctrl Pts',(-2.9924915517034,-1.,2.83526351254248));
#32138=CARTESIAN_POINT('Ctrl Pts',(-2.98952916401446,-1.,2.82808728190157));
#32139=CARTESIAN_POINT('Ctrl Pts',(-2.9865368066918,-1.,2.82093279065457));
#32140=CARTESIAN_POINT('Ctrl Pts',(-2.98351419779767,-1.,2.81380019196286));
#32141=CARTESIAN_POINT('Ctrl Pts',(-2.98046109647241,-1.,2.80668968101106));
#32142=CARTESIAN_POINT('Ctrl Pts',(-2.97737733718287,-1.,2.7996015327823));
#32143=CARTESIAN_POINT('Ctrl Pts',(-2.9742628834758,-1.,2.79253615718248));
#32144=CARTESIAN_POINT('Ctrl Pts',(-2.97111781461465,-1.,2.78549409123769));
#32145=CARTESIAN_POINT('Ctrl Pts',(-2.96794221043036,-1.,2.7784758954285));
#32146=CARTESIAN_POINT('Ctrl Pts',(-2.96473605585583,-1.,2.77148206836498));
#32147=CARTESIAN_POINT('Ctrl Pts',(-2.96149914764818,-1.,2.76451296269557));
#32148=CARTESIAN_POINT('Ctrl Pts',(-2.95823097665896,-1.,2.7575686788835));
#32149=CARTESIAN_POINT('Ctrl Pts',(-2.95493069316161,-1.,2.75064903318947));
#32150=CARTESIAN_POINT('Ctrl Pts',(-2.95159737214266,-1.,2.74375379492172));
#32151=CARTESIAN_POINT('Ctrl Pts',(-2.94823023414364,-1.,2.73688288329808));
#32152=CARTESIAN_POINT('Ctrl Pts',(-2.94482887675143,-1.,2.73003657371617));
#32153=CARTESIAN_POINT('Ctrl Pts',(-2.94139351933897,-1.,2.72321571511337));
#32154=CARTESIAN_POINT('Ctrl Pts',(-2.93792519474972,-1.,2.71642190053592));
#32155=CARTESIAN_POINT('Ctrl Pts',(-2.93442516311179,-1.,2.70965695523787));
#32156=CARTESIAN_POINT('Ctrl Pts',(-2.9308943823375,-1.,2.70292247416885));
#32157=CARTESIAN_POINT('Ctrl Pts',(-2.92733294395267,-1.,2.69621932864301));
#32158=CARTESIAN_POINT('Ctrl Pts',(-2.92373955325875,-1.,2.68954721165339));
#32159=CARTESIAN_POINT('Ctrl Pts',(-2.92011090722152,-1.,2.68290409279688));
#32160=CARTESIAN_POINT('Ctrl Pts',(-2.91644290704285,-1.,2.67628728855312));
#32161=CARTESIAN_POINT('Ctrl Pts',(-2.91273193382882,-1.,2.66969458792631));
#32162=CARTESIAN_POINT('Ctrl Pts',(-2.90897617968923,-1.,2.6631254261681));
#32163=CARTESIAN_POINT('Ctrl Pts',(-2.90517678087461,-1.,2.65658188464282));
#32164=CARTESIAN_POINT('Ctrl Pts',(-2.90133950224867,-1.,2.65007017365564));
#32165=CARTESIAN_POINT('Ctrl Pts',(-2.89747231723345,-1.,2.64359851684131));
#32166=CARTESIAN_POINT('Ctrl Pts',(-2.89358228854544,-1.,2.63717442263932));
#32167=CARTESIAN_POINT('Ctrl Pts',(-2.88967244854239,-1.,2.63080195420767));
#32168=CARTESIAN_POINT('Ctrl Pts',(-2.88573922195059,-1.,2.62447947640262));
#32169=CARTESIAN_POINT('Ctrl Pts',(-2.88176821427525,-1.,2.61819596473108));
#32170=CARTESIAN_POINT('Ctrl Pts',(-2.87773881947916,-1.,2.61193507170955));
#32171=CARTESIAN_POINT('Ctrl Pts',(-2.87363176656501,-1.,2.60568177881303));
#32172=CARTESIAN_POINT('Ctrl Pts',(-2.86943633170722,-1.,2.5994287522321));
#32173=CARTESIAN_POINT('Ctrl Pts',(-2.86515629953513,-1.,2.59318160184908));
#32174=CARTESIAN_POINT('Ctrl Pts',(-2.86081999003629,-1.,2.58696770643524));
#32175=CARTESIAN_POINT('Ctrl Pts',(-2.85647171715092,-1.,2.58082875254357));
#32176=CARTESIAN_POINT('Ctrl Pts',(-2.85215360144431,-1.,2.57480482727081));
#32177=CARTESIAN_POINT('Ctrl Pts',(-2.84788893329067,-1.,2.56891984251721));
#32178=CARTESIAN_POINT('Ctrl Pts',(-2.84366802680237,-1.,2.56316920798513));
#32179=CARTESIAN_POINT('Ctrl Pts',(-2.83942515220782,-1.,2.55749952145241));
#32180=CARTESIAN_POINT('Ctrl Pts',(-2.83505269592536,-1.,2.55182152807077));
#32181=CARTESIAN_POINT('Ctrl Pts',(-2.83044254225917,-1.,2.54604736792655));
#32182=CARTESIAN_POINT('Ctrl Pts',(-2.8255216764922,-1.,2.54012272520199));
#32183=CARTESIAN_POINT('Ctrl Pts',(-2.82028550483689,-1.,2.53405679667412));
#32184=CARTESIAN_POINT('Ctrl Pts',(-2.81484379048475,-1.,2.52796388055278));
#32185=CARTESIAN_POINT('Ctrl Pts',(-2.80941521966941,-1.,2.52205778589653));
#32186=CARTESIAN_POINT('Ctrl Pts',(-2.80427363984653,-1.,2.51660190465805));
#32187=CARTESIAN_POINT('Ctrl Pts',(-2.79970585014168,-1.,2.51186983687818));
#32188=CARTESIAN_POINT('Ctrl Pts',(-2.79596878057287,-1.,2.50810555977671));
#32189=CARTESIAN_POINT('Ctrl Pts',(-2.79344192164147,-1.,2.50567182569081));
#32190=CARTESIAN_POINT('Ctrl Pts',(-2.79217568804755,-1.,2.50455968395146));
#32191=CARTESIAN_POINT('Ctrl Pts',(-2.79164172518905,-1.,2.50417932839313));
#32192=CARTESIAN_POINT('Ctrl Pts',(-2.79145823440781,-1.,2.50410700351493));
#32193=CARTESIAN_POINT('Ctrl Pts',(-2.79140942341258,-1.,2.50410331873176));
#32194=CARTESIAN_POINT('',(-2.90994629141562,-1.,2.36531447826213));
#32195=CARTESIAN_POINT('Origin',(0.,-1.,0.));
#32196=CARTESIAN_POINT('',(-3.35260583073571,-1.,2.52982887637028));
#32197=CARTESIAN_POINT('Ctrl Pts',(-2.90994629141562,-1.,2.36531447826213));
#32198=CARTESIAN_POINT('Ctrl Pts',(-2.90995756655558,-1.,2.3653621118858));
#32199=CARTESIAN_POINT('Ctrl Pts',(-2.9100577052777,-1.,2.36553202948741));
#32200=CARTESIAN_POINT('Ctrl Pts',(-2.91051690822262,-1.,2.36599991765853));
#32201=CARTESIAN_POINT('Ctrl Pts',(-2.91181344022628,-1.,2.36707658451709));
#32202=CARTESIAN_POINT('Ctrl Pts',(-2.91461249883016,-1.,2.36919161373074));
#32203=CARTESIAN_POINT('Ctrl Pts',(-2.9189150379156,-1.,2.37229381109939));
#32204=CARTESIAN_POINT('Ctrl Pts',(-2.92430340582912,-1.,2.37606510524271));
#32205=CARTESIAN_POINT('Ctrl Pts',(-2.93049643640517,-1.,2.3802898958232));
#32206=CARTESIAN_POINT('Ctrl Pts',(-2.93717903280599,-1.,2.38472771516476));
#32207=CARTESIAN_POINT('Ctrl Pts',(-2.94404820669135,-1.,2.38914929090806));
#32208=CARTESIAN_POINT('Ctrl Pts',(-2.95085857128372,-1.,2.39337207631613));
#32209=CARTESIAN_POINT('Ctrl Pts',(-2.95748006482811,-1.,2.39730553974412));
#32210=CARTESIAN_POINT('Ctrl Pts',(-2.96390432240181,-1.,2.40095565711535));
#32211=CARTESIAN_POINT('Ctrl Pts',(-2.97019641312272,-1.,2.40438604734848));
#32212=CARTESIAN_POINT('Ctrl Pts',(-2.97646002822395,-1.,2.40768975073691));
#32213=CARTESIAN_POINT('Ctrl Pts',(-2.98280015815132,-1.,2.41095909342591));
#32214=CARTESIAN_POINT('Ctrl Pts',(-2.98927983005851,-1.,2.4142506419963));
#32215=CARTESIAN_POINT('Ctrl Pts',(-2.99590509293561,-1.,2.4175732450056));
#32216=CARTESIAN_POINT('Ctrl Pts',(-3.00264868586038,-1.,2.42090763946812));
#32217=CARTESIAN_POINT('Ctrl Pts',(-3.00946442616674,-1.,2.42421849439625));
#32218=CARTESIAN_POINT('Ctrl Pts',(-3.01630420830494,-1.,2.4274685626416));
#32219=CARTESIAN_POINT('Ctrl Pts',(-3.02313656035977,-1.,2.43063415586615));
#32220=CARTESIAN_POINT('Ctrl Pts',(-3.02995534946946,-1.,2.43371241361462));
#32221=CARTESIAN_POINT('Ctrl Pts',(-3.03676949672797,-1.,2.43671278042394));
#32222=CARTESIAN_POINT('Ctrl Pts',(-3.04359685040545,-1.,2.43965194061849));
#32223=CARTESIAN_POINT('Ctrl Pts',(-3.05045678021509,-1.,2.44254768923109));
#32224=CARTESIAN_POINT('Ctrl Pts',(-3.05736242671521,-1.,2.44541251892568));
#32225=CARTESIAN_POINT('Ctrl Pts',(-3.06431596421422,-1.,2.44824970516558));
#32226=CARTESIAN_POINT('Ctrl Pts',(-3.0713129052131,-1.,2.45105688854432));
#32227=CARTESIAN_POINT('Ctrl Pts',(-3.07834472886145,-1.,2.45382826787795));
#32228=CARTESIAN_POINT('Ctrl Pts',(-3.08540206545313,-1.,2.45655725437037));
#32229=CARTESIAN_POINT('Ctrl Pts',(-3.09247787931881,-1.,2.45923912563875));
#32230=CARTESIAN_POINT('Ctrl Pts',(-3.09956993697048,-1.,2.4618730850188));
#32231=CARTESIAN_POINT('Ctrl Pts',(-3.10667907901981,-1.,2.46446082979645));
#32232=CARTESIAN_POINT('Ctrl Pts',(-3.11380805536124,-1.,2.46700558843507));
#32233=CARTESIAN_POINT('Ctrl Pts',(-3.12096015766984,-1.,2.4695109894747));
#32234=CARTESIAN_POINT('Ctrl Pts',(-3.12813790805948,-1.,2.47197997765868));
#32235=CARTESIAN_POINT('Ctrl Pts',(-3.13534181229282,-1.,2.47441378371923));
#32236=CARTESIAN_POINT('Ctrl Pts',(-3.14257099546531,-1.,2.47681245356095));
#32237=CARTESIAN_POINT('Ctrl Pts',(-3.14982373241335,-1.,2.47917529057016));
#32238=CARTESIAN_POINT('Ctrl Pts',(-3.15709802322735,-1.,2.48150133566568));
#32239=CARTESIAN_POINT('Ctrl Pts',(-3.16439213290181,-1.,2.48378981792739));
#32240=CARTESIAN_POINT('Ctrl Pts',(-3.17170518863357,-1.,2.48604065348619));
#32241=CARTESIAN_POINT('Ctrl Pts',(-3.17903698136679,-1.,2.48825428288243));
#32242=CARTESIAN_POINT('Ctrl Pts',(-3.18638771282315,-1.,2.49043146334095));
#32243=CARTESIAN_POINT('Ctrl Pts',(-3.19375775555814,-1.,2.4925730723986));
#32244=CARTESIAN_POINT('Ctrl Pts',(-3.20114742397549,-1.,2.49467992057726));
#32245=CARTESIAN_POINT('Ctrl Pts',(-3.2085566984974,-1.,2.49675252647298));
#32246=CARTESIAN_POINT('Ctrl Pts',(-3.21598526261157,-1.,2.49879114599293));
#32247=CARTESIAN_POINT('Ctrl Pts',(-3.22343262620387,-1.,2.5007958720187));
#32248=CARTESIAN_POINT('Ctrl Pts',(-3.23089822320596,-1.,2.50276671338074));
#32249=CARTESIAN_POINT('Ctrl Pts',(-3.23838151080383,-1.,2.50470367580078));
#32250=CARTESIAN_POINT('Ctrl Pts',(-3.24588208984042,-1.,2.50660685940645));
#32251=CARTESIAN_POINT('Ctrl Pts',(-3.25339971461265,-1.,2.50847647070936));
#32252=CARTESIAN_POINT('Ctrl Pts',(-3.26093423001716,-1.,2.51031277813697));
#32253=CARTESIAN_POINT('Ctrl Pts',(-3.26848552888271,-1.,2.51211608411539));
#32254=CARTESIAN_POINT('Ctrl Pts',(-3.27605350473048,-1.,2.51388669270329));
#32255=CARTESIAN_POINT('Ctrl Pts',(-3.28363799702583,-1.,2.51562487464215));
#32256=CARTESIAN_POINT('Ctrl Pts',(-3.2912387729863,-1.,2.51733085123316));
#32257=CARTESIAN_POINT('Ctrl Pts',(-3.29885556387661,-1.,2.51900480700548));
#32258=CARTESIAN_POINT('Ctrl Pts',(-3.30648808814986,-1.,2.52064689568167));
#32259=CARTESIAN_POINT('Ctrl Pts',(-3.31413607874727,-1.,2.52225724871375));
#32260=CARTESIAN_POINT('Ctrl Pts',(-3.32179931079521,-1.,2.52383598396878));
#32261=CARTESIAN_POINT('Ctrl Pts',(-3.32947762189049,-1.,2.52538321165774));
#32262=CARTESIAN_POINT('Ctrl Pts',(-3.33717090000955,-1.,2.52689902691551));
#32263=CARTESIAN_POINT('Ctrl Pts',(-3.34333744117093,-1.,2.52808660916879));
#32264=CARTESIAN_POINT('Ctrl Pts',(-3.34796903577628,-1.,2.5289632161143));
#32265=CARTESIAN_POINT('Ctrl Pts',(-3.35105973714426,-1.,2.52954136549357));
#32266=CARTESIAN_POINT('Ctrl Pts',(-3.35260583073571,-1.,2.52982887637028));
#32267=CARTESIAN_POINT('',(-3.44202241512147,-1.,2.40675750623143));
#32268=CARTESIAN_POINT('',(-3.35260583073571,-1.,2.52982887637028));
#32269=CARTESIAN_POINT('',(-3.14877060440327,-1.,2.03660101169715));
#32270=CARTESIAN_POINT('Ctrl Pts',(-3.44202241512147,-1.,2.40675750623143));
#32271=CARTESIAN_POINT('Ctrl Pts',(-3.44127120683039,-1.,2.4053759295909));
#32272=CARTESIAN_POINT('Ctrl Pts',(-3.43976627484234,-1.,2.40261515589405));
#32273=CARTESIAN_POINT('Ctrl Pts',(-3.43750133064416,-1.,2.39848113410292));
#32274=CARTESIAN_POINT('Ctrl Pts',(-3.4344663067854,-1.,2.39298338804493));
#32275=CARTESIAN_POINT('Ctrl Pts',(-3.4306473271292,-1.,2.38613505843552));
#32276=CARTESIAN_POINT('Ctrl Pts',(-3.42680309754399,-1.,2.37931067028926));
#32277=CARTESIAN_POINT('Ctrl Pts',(-3.42293356216511,-1.,2.37251035954292));
#32278=CARTESIAN_POINT('Ctrl Pts',(-3.41903866635852,-1.,2.36573431470642));
#32279=CARTESIAN_POINT('Ctrl Pts',(-3.41511836751469,-1.,2.35898278606946));
#32280=CARTESIAN_POINT('Ctrl Pts',(-3.41117262314119,-1.,2.35225606824109));
#32281=CARTESIAN_POINT('Ctrl Pts',(-3.40720137404297,-1.,2.34555447649188));
#32282=CARTESIAN_POINT('Ctrl Pts',(-3.40320452776743,-1.,2.33887832342782));
#32283=CARTESIAN_POINT('Ctrl Pts',(-3.39918194577956,-1.,2.33222789882489));
#32284=CARTESIAN_POINT('Ctrl Pts',(-3.39513342019756,-1.,2.3256034390248));
#32285=CARTESIAN_POINT('Ctrl Pts',(-3.39105869474822,-1.,2.31900513925424));
#32286=CARTESIAN_POINT('Ctrl Pts',(-3.38695751492462,-1.,2.31243319489367));
#32287=CARTESIAN_POINT('Ctrl Pts',(-3.3828296733661,-1.,2.30588783640343));
#32288=CARTESIAN_POINT('Ctrl Pts',(-3.37867504959433,-1.,2.29936936127624));
#32289=CARTESIAN_POINT('Ctrl Pts',(-3.37449367172826,-1.,2.29287818007393));
#32290=CARTESIAN_POINT('Ctrl Pts',(-3.37028570206488,-1.,2.28641481081137));
#32291=CARTESIAN_POINT('Ctrl Pts',(-3.36605130713076,-1.,2.27997979458037));
#32292=CARTESIAN_POINT('Ctrl Pts',(-3.36179055004409,-1.,2.2735736262093));
#32293=CARTESIAN_POINT('Ctrl Pts',(-3.35750328523061,-1.,2.2671966857991));
#32294=CARTESIAN_POINT('Ctrl Pts',(-3.35318902552626,-1.,2.26084915222449));
#32295=CARTESIAN_POINT('Ctrl Pts',(-3.34884690292285,-1.,2.25453097693483));
#32296=CARTESIAN_POINT('Ctrl Pts',(-3.34447596770723,-1.,2.24824207678256));
#32297=CARTESIAN_POINT('Ctrl Pts',(-3.34007543738025,-1.,2.24198249391422));
#32298=CARTESIAN_POINT('Ctrl Pts',(-3.33564495756482,-1.,2.23575256328812));
#32299=CARTESIAN_POINT('Ctrl Pts',(-3.33118487773611,-1.,2.22955308907233));
#32300=CARTESIAN_POINT('Ctrl Pts',(-3.3266964672289,-1.,2.22338548312772));
#32301=CARTESIAN_POINT('Ctrl Pts',(-3.32218125618968,-1.,2.21725135110898));
#32302=CARTESIAN_POINT('Ctrl Pts',(-3.31764044024235,-1.,2.21115211847875));
#32303=CARTESIAN_POINT('Ctrl Pts',(-3.31307424608949,-1.,2.20508863150607));
#32304=CARTESIAN_POINT('Ctrl Pts',(-3.30848134694595,-1.,2.19906078949923));
#32305=CARTESIAN_POINT('Ctrl Pts',(-3.30385816281831,-1.,2.19306710376111));
#32306=CARTESIAN_POINT('Ctrl Pts',(-3.29920022557639,-1.,2.18710556500327));
#32307=CARTESIAN_POINT('Ctrl Pts',(-3.2945036150049,-1.,2.18117455557065));
#32308=CARTESIAN_POINT('Ctrl Pts',(-3.28976645712568,-1.,2.17527380048423));
#32309=CARTESIAN_POINT('Ctrl Pts',(-3.28499019979724,-1.,2.16940517773455));
#32310=CARTESIAN_POINT('Ctrl Pts',(-3.280181508414,-1.,2.16357391934425));
#32311=CARTESIAN_POINT('Ctrl Pts',(-3.27534954469187,-1.,2.15778690038347));
#32312=CARTESIAN_POINT('Ctrl Pts',(-3.27050245897228,-1.,2.15205043199808));
#32313=CARTESIAN_POINT('Ctrl Pts',(-3.26564388189759,-1.,2.1463680529566));
#32314=CARTESIAN_POINT('Ctrl Pts',(-3.26077002641879,-1.,2.14073870754264));
#32315=CARTESIAN_POINT('Ctrl Pts',(-3.25586495065054,-1.,2.13515375878803));
#32316=CARTESIAN_POINT('Ctrl Pts',(-3.25090574494028,-1.,2.12960028396832));
#32317=CARTESIAN_POINT('Ctrl Pts',(-3.24587102613376,-1.,2.12406646410962));
#32318=CARTESIAN_POINT('Ctrl Pts',(-3.24074905517293,-1.,2.11854673326979));
#32319=CARTESIAN_POINT('Ctrl Pts',(-3.23554444767099,-1.,2.11304604021773));
#32320=CARTESIAN_POINT('Ctrl Pts',(-3.23028945793289,-1.,2.10758699642451));
#32321=CARTESIAN_POINT('Ctrl Pts',(-3.22503437553434,-1.,2.10220384298492));
#32322=CARTESIAN_POINT('Ctrl Pts',(-3.21982707347009,-1.,2.09692958434895));
#32323=CARTESIAN_POINT('Ctrl Pts',(-3.21469429601654,-1.,2.09178419460443));
#32324=CARTESIAN_POINT('Ctrl Pts',(-3.20962575845463,-1.,2.08676465517455));
#32325=CARTESIAN_POINT('Ctrl Pts',(-3.2045481863073,-1.,2.08182850370878));
#32326=CARTESIAN_POINT('Ctrl Pts',(-3.19934132836019,-1.,2.07690441870722));
#32327=CARTESIAN_POINT('Ctrl Pts',(-3.19388465568252,-1.,2.07192253497857));
#32328=CARTESIAN_POINT('Ctrl Pts',(-3.18809755562368,-1.,2.06684062744112));
#32329=CARTESIAN_POINT('Ctrl Pts',(-3.18197692964614,-1.,2.06166849827101));
#32330=CARTESIAN_POINT('Ctrl Pts',(-3.17564906975371,-1.,2.05650186773132));
#32331=CARTESIAN_POINT('Ctrl Pts',(-3.16936341689527,-1.,2.05151770247233));
#32332=CARTESIAN_POINT('Ctrl Pts',(-3.16343165058912,-1.,2.04693331247446));
#32333=CARTESIAN_POINT('Ctrl Pts',(-3.15817983946367,-1.,2.04297406404027));
#32334=CARTESIAN_POINT('Ctrl Pts',(-3.15389991674792,-1.,2.03984073791519));
#32335=CARTESIAN_POINT('Ctrl Pts',(-3.15102344775328,-1.,2.03783225495961));
#32336=CARTESIAN_POINT('Ctrl Pts',(-3.14959882629805,-1.,2.03693188810544));
#32337=CARTESIAN_POINT('Ctrl Pts',(-3.1490119366901,-1.,2.03663974554932));
#32338=CARTESIAN_POINT('Ctrl Pts',(-3.14881939088124,-1.,2.03659701539259));
#32339=CARTESIAN_POINT('Ctrl Pts',(-3.14877060440328,-1.,2.03660101169715));
#32340=CARTESIAN_POINT('',(-3.24413672884812,-1.,1.88097764062697));
#32341=CARTESIAN_POINT('Origin',(0.,-1.,0.));
#32342=CARTESIAN_POINT('',(-3.70708211654725,-1.,1.97421938526992));
#32343=CARTESIAN_POINT('Ctrl Pts',(-3.24413672884812,-1.,1.88097764062697));
#32344=CARTESIAN_POINT('Ctrl Pts',(-3.24415531671284,-1.,1.8810229239812));
#32345=CARTESIAN_POINT('Ctrl Pts',(-3.24428080353022,-1.,1.88117508446775));
#32346=CARTESIAN_POINT('Ctrl Pts',(-3.24480754676064,-1.,1.88156537699203));
#32347=CARTESIAN_POINT('Ctrl Pts',(-3.2462565441079,-1.,1.88242596600454));
#32348=CARTESIAN_POINT('Ctrl Pts',(-3.24935200511918,-1.,1.88407708646357));
#32349=CARTESIAN_POINT('Ctrl Pts',(-3.25408686339463,-1.,1.88646802523466));
#32350=CARTESIAN_POINT('Ctrl Pts',(-3.25999885193947,-1.,1.88934996203698));
#32351=CARTESIAN_POINT('Ctrl Pts',(-3.26677653888676,-1.,1.89255393500965));
#32352=CARTESIAN_POINT('Ctrl Pts',(-3.27407108933139,-1.,1.89589172903793));
#32353=CARTESIAN_POINT('Ctrl Pts',(-3.28154737912352,-1.,1.89918429230462));
#32354=CARTESIAN_POINT('Ctrl Pts',(-3.2889344860029,-1.,1.90228971247527));
#32355=CARTESIAN_POINT('Ctrl Pts',(-3.29608978722113,-1.,1.90513891864087));
#32356=CARTESIAN_POINT('Ctrl Pts',(-3.30300595568195,-1.,1.90773912171341));
#32357=CARTESIAN_POINT('Ctrl Pts',(-3.30975721158596,-1.,1.91014297830446));
#32358=CARTESIAN_POINT('Ctrl Pts',(-3.31646052426364,-1.,1.91242616234442));
#32359=CARTESIAN_POINT('Ctrl Pts',(-3.32323403454535,-1.,1.91466343916628));
#32360=CARTESIAN_POINT('Ctrl Pts',(-3.33014884257873,-1.,1.91690081930331));
#32361=CARTESIAN_POINT('Ctrl Pts',(-3.33721230710012,-1.,1.9191460961021));
#32362=CARTESIAN_POINT('Ctrl Pts',(-3.34439448941961,-1.,1.92138450828404));
#32363=CARTESIAN_POINT('Ctrl Pts',(-3.35164424847223,-1.,1.92358838440528));
#32364=CARTESIAN_POINT('Ctrl Pts',(-3.35890824422965,-1.,1.92572846125756));
#32365=CARTESIAN_POINT('Ctrl Pts',(-3.36615168657567,-1.,1.92778626543786));
#32366=CARTESIAN_POINT('Ctrl Pts',(-3.37336807068043,-1.,1.92975993109877));
#32367=CARTESIAN_POINT('Ctrl Pts',(-3.3805676852555,-1.,1.93165739093276));
#32368=CARTESIAN_POINT('Ctrl Pts',(-3.38777076883256,-1.,1.93349233176788));
#32369=CARTESIAN_POINT('Ctrl Pts',(-3.39499923640795,-1.,1.93527929945985));
#32370=CARTESIAN_POINT('Ctrl Pts',(-3.40226802104109,-1.,1.93702857723098));
#32371=CARTESIAN_POINT('Ctrl Pts',(-3.40957978266642,-1.,1.93874306008143));
#32372=CARTESIAN_POINT('Ctrl Pts',(-3.41692971994096,-1.,1.94042111965246));
#32373=CARTESIAN_POINT('Ctrl Pts',(-3.42430850941503,-1.,1.94205835913696));
#32374=CARTESIAN_POINT('Ctrl Pts',(-3.43170586602434,-1.,1.94364973660284));
#32375=CARTESIAN_POINT('Ctrl Pts',(-3.43911410197687,-1.,1.94519168842879));
#32376=CARTESIAN_POINT('Ctrl Pts',(-3.44653088665681,-1.,1.94668377715329));
#32377=CARTESIAN_POINT('Ctrl Pts',(-3.45395731584051,-1.,1.94812754766524));
#32378=CARTESIAN_POINT('Ctrl Pts',(-3.46139661060962,-1.,1.94952575850197));
#32379=CARTESIAN_POINT('Ctrl Pts',(-3.46885258974191,-1.,1.95088147859876));
#32380=CARTESIAN_POINT('Ctrl Pts',(-3.47632820495921,-1.,1.95219722189876));
#32381=CARTESIAN_POINT('Ctrl Pts',(-3.48382414832634,-1.,1.95347412486308));
#32382=CARTESIAN_POINT('Ctrl Pts',(-3.49133956289133,-1.,1.95471236969643));
#32383=CARTESIAN_POINT('Ctrl Pts',(-3.49887263575583,-1.,1.95591153823661));
#32384=CARTESIAN_POINT('Ctrl Pts',(-3.50642124159909,-1.,1.95707099606511));
#32385=CARTESIAN_POINT('Ctrl Pts',(-3.51398354617794,-1.,1.95819025316779));
#32386=CARTESIAN_POINT('Ctrl Pts',(-3.52155867431486,-1.,1.95926936324461));
#32387=CARTESIAN_POINT('Ctrl Pts',(-3.52914648844351,-1.,1.96030879411566));
#32388=CARTESIAN_POINT('Ctrl Pts',(-3.53674730625813,-1.,1.96130926212689));
#32389=CARTESIAN_POINT('Ctrl Pts',(-3.54436163300443,-1.,1.96227157573067));
#32390=CARTESIAN_POINT('Ctrl Pts',(-3.55198990600886,-1.,1.96319648628644));
#32391=CARTESIAN_POINT('Ctrl Pts',(-3.55963218706096,-1.,1.96408450906812));
#32392=CARTESIAN_POINT('Ctrl Pts',(-3.56728820357791,-1.,1.96493594634567));
#32393=CARTESIAN_POINT('Ctrl Pts',(-3.57495748600959,-1.,1.96575096652789));
#32394=CARTESIAN_POINT('Ctrl Pts',(-3.58263947663829,-1.,1.96652966688911));
#32395=CARTESIAN_POINT('Ctrl Pts',(-3.59033364022801,-1.,1.96727213799544));
#32396=CARTESIAN_POINT('Ctrl Pts',(-3.59803959819938,-1.,1.96797854118369));
#32397=CARTESIAN_POINT('Ctrl Pts',(-3.60575714017989,-1.,1.9686491188594));
#32398=CARTESIAN_POINT('Ctrl Pts',(-3.61348615496704,-1.,1.96928416040877));
#32399=CARTESIAN_POINT('Ctrl Pts',(-3.62122658401893,-1.,1.96988398129978));
#32400=CARTESIAN_POINT('Ctrl Pts',(-3.62897836973293,-1.,1.97044889850463));
#32401=CARTESIAN_POINT('Ctrl Pts',(-3.63674139590412,-1.,1.97097920454464));
#32402=CARTESIAN_POINT('Ctrl Pts',(-3.64451546723514,-1.,1.97147515441164));
#32403=CARTESIAN_POINT('Ctrl Pts',(-3.652300347166,-1.,1.9719369724024));
#32404=CARTESIAN_POINT('Ctrl Pts',(-3.6600957816636,-1.,1.9723648543905));
#32405=CARTESIAN_POINT('Ctrl Pts',(-3.66790152752075,-1.,1.97275897198678));
#32406=CARTESIAN_POINT('Ctrl Pts',(-3.67571738107084,-1.,1.97311947678516));
#32407=CARTESIAN_POINT('Ctrl Pts',(-3.68354319915092,-1.,1.97344650304519));
#32408=CARTESIAN_POINT('Ctrl Pts',(-3.69137888599902,-1.,1.97374016225483));
#32409=CARTESIAN_POINT('Ctrl Pts',(-3.6976552856004,-1.,1.97394846383216));
#32410=CARTESIAN_POINT('Ctrl Pts',(-3.70236698912904,-1.,1.97408973726715));
#32411=CARTESIAN_POINT('Ctrl Pts',(-3.70551008132332,-1.,1.97417727645308));
#32412=CARTESIAN_POINT('Ctrl Pts',(-3.70708211654725,-1.,1.97421938526992));
#32413=CARTESIAN_POINT('',(-3.77614523045147,-1.,1.8386753923786));
#32414=CARTESIAN_POINT('',(-3.70708211654725,-1.,1.97421938526992));
#32415=CARTESIAN_POINT('',(-3.42859860294306,-1.,1.5189508286633));
#32416=CARTESIAN_POINT('Ctrl Pts',(-3.77614523045147,-1.,1.8386753923786));
#32417=CARTESIAN_POINT('Ctrl Pts',(-3.77518714457833,-1.,1.83742834010626));
#32418=CARTESIAN_POINT('Ctrl Pts',(-3.77326886064398,-1.,1.83493697934534));
#32419=CARTESIAN_POINT('Ctrl Pts',(-3.77038509817999,-1.,1.83120816955645));
#32420=CARTESIAN_POINT('Ctrl Pts',(-3.76652740353775,-1.,1.82625289220915));
#32421=CARTESIAN_POINT('Ctrl Pts',(-3.76168412707948,-1.,1.82008629694091));
#32422=CARTESIAN_POINT('Ctrl Pts',(-3.75681965683071,-1.,1.8139472983358));
#32423=CARTESIAN_POINT('Ctrl Pts',(-3.75193395887977,-1.,1.80783603939617));
#32424=CARTESIAN_POINT('Ctrl Pts',(-3.74702700875467,-1.,1.8017527148577));
#32425=CARTESIAN_POINT('Ctrl Pts',(-3.74209880352445,-1.,1.79569757859422));
#32426=CARTESIAN_POINT('Ctrl Pts',(-3.73714934730681,-1.,1.78967092823491));
#32427=CARTESIAN_POINT('Ctrl Pts',(-3.7321786309547,-1.,1.78367308442901));
#32428=CARTESIAN_POINT('Ctrl Pts',(-3.72718661205609,-1.,1.77770437039658));
#32429=CARTESIAN_POINT('Ctrl Pts',(-3.72217319911254,-1.,1.77176509401761));
#32430=CARTESIAN_POINT('Ctrl Pts',(-3.71713822377359,-1.,1.76585552124394));
#32431=CARTESIAN_POINT('Ctrl Pts',(-3.71208146346136,-1.,1.75997588498865));
#32432=CARTESIAN_POINT('Ctrl Pts',(-3.70700269736659,-1.,1.75412641804042));
#32433=CARTESIAN_POINT('Ctrl Pts',(-3.7019017567335,-1.,1.74830738046057));
#32434=CARTESIAN_POINT('Ctrl Pts',(-3.69677856910517,-1.,1.74251908492617));
#32435=CARTESIAN_POINT('Ctrl Pts',(-3.69163322648036,-1.,1.73676193254557));
#32436=CARTESIAN_POINT('Ctrl Pts',(-3.68646597019332,-1.,1.73103640956717));
#32437=CARTESIAN_POINT('Ctrl Pts',(-3.68127704936579,-1.,1.72534302437056));
#32438=CARTESIAN_POINT('Ctrl Pts',(-3.67606660374709,-1.,1.71968225581808));
#32439=CARTESIAN_POINT('Ctrl Pts',(-3.67083454901611,-1.,1.71405450210383));
#32440=CARTESIAN_POINT('Ctrl Pts',(-3.66558043198876,-1.,1.70846001610956));
#32441=CARTESIAN_POINT('Ctrl Pts',(-3.66030338774847,-1.,1.70289888566873));
#32442=CARTESIAN_POINT('Ctrl Pts',(-3.65500246526749,-1.,1.69737117722534));
#32443=CARTESIAN_POINT('Ctrl Pts',(-3.64967689827371,-1.,1.69187705481689));
#32444=CARTESIAN_POINT('Ctrl Pts',(-3.64432638915203,-1.,1.68641690471457));
#32445=CARTESIAN_POINT('Ctrl Pts',(-3.63895140887462,-1.,1.68099146651586));
#32446=CARTESIAN_POINT('Ctrl Pts',(-3.63355343201232,-1.,1.67560193613156));
#32447=CARTESIAN_POINT('Ctrl Pts',(-3.62813422105271,-1.,1.67024966008045));
#32448=CARTESIAN_POINT('Ctrl Pts',(-3.62269517989109,-1.,1.66493585923855));
#32449=CARTESIAN_POINT('Ctrl Pts',(-3.61723666482456,-1.,1.65966133399186));
#32450=CARTESIAN_POINT('Ctrl Pts',(-3.61175734965127,-1.,1.65442619244325));
#32451=CARTESIAN_POINT('Ctrl Pts',(-3.60625346556992,-1.,1.64922952425832));
#32452=CARTESIAN_POINT('Ctrl Pts',(-3.60072028513845,-1.,1.64407004385582));
#32453=CARTESIAN_POINT('Ctrl Pts',(-3.59515368334893,-1.,1.63894676675352));
#32454=CARTESIAN_POINT('Ctrl Pts',(-3.58955176627879,-1.,1.6338597145126));
#32455=CARTESIAN_POINT('Ctrl Pts',(-3.58391625774343,-1.,1.62881051550745));
#32456=CARTESIAN_POINT('Ctrl Pts',(-3.5782545595439,-1.,1.62380329464844));
#32457=CARTESIAN_POINT('Ctrl Pts',(-3.57257679609806,-1.,1.61884340915404));
#32458=CARTESIAN_POINT('Ctrl Pts',(-3.56689200468387,-1.,1.61393581747514));
#32459=CARTESIAN_POINT('Ctrl Pts',(-3.5612043248298,-1.,1.60908344685457));
#32460=CARTESIAN_POINT('Ctrl Pts',(-3.55550985096129,-1.,1.60428584699853));
#32461=CARTESIAN_POINT('Ctrl Pts',(-3.54979148634454,-1.,1.59953698113457));
#32462=CARTESIAN_POINT('Ctrl Pts',(-3.54402458182337,-1.,1.59482766949766));
#32463=CARTESIAN_POINT('Ctrl Pts',(-3.53818616861077,-1.,1.59014958368739));
#32464=CARTESIAN_POINT('Ctrl Pts',(-3.5322637814708,-1.,1.58549906268088));
#32465=CARTESIAN_POINT('Ctrl Pts',(-3.52626275334881,-1.,1.58088027227848));
#32466=CARTESIAN_POINT('Ctrl Pts',(-3.52021847865912,-1.,1.57631049988158));
#32467=CARTESIAN_POINT('Ctrl Pts',(-3.51418598431665,-1.,1.57181569799743));
#32468=CARTESIAN_POINT('Ctrl Pts',(-3.50821771695363,-1.,1.56742097575012));
#32469=CARTESIAN_POINT('Ctrl Pts',(-3.50234321621578,-1.,1.56314187758675));
#32470=CARTESIAN_POINT('Ctrl Pts',(-3.49655185179655,-1.,1.55897703097874));
#32471=CARTESIAN_POINT('Ctrl Pts',(-3.4907646087742,-1.,1.55489595901116));
#32472=CARTESIAN_POINT('Ctrl Pts',(-3.48485155928567,-1.,1.55084702970452));
#32473=CARTESIAN_POINT('Ctrl Pts',(-3.47868272898751,-1.,1.54678009290276));
#32474=CARTESIAN_POINT('Ctrl Pts',(-3.47217189224653,-1.,1.54266605398187));
#32475=CARTESIAN_POINT('Ctrl Pts',(-3.46531752207153,-1.,1.53851507915502));
#32476=CARTESIAN_POINT('Ctrl Pts',(-3.45825932955032,-1.,1.53440195378792));
#32477=CARTESIAN_POINT('Ctrl Pts',(-3.45127136828305,-1.,1.53046244461635));
#32478=CARTESIAN_POINT('Ctrl Pts',(-3.44469547526647,-1.,1.52686242875556));
#32479=CARTESIAN_POINT('Ctrl Pts',(-3.4388889597401,-1.,1.5237734895035));
#32480=CARTESIAN_POINT('Ctrl Pts',(-3.43417156977893,-1.,1.52134826724292));
#32481=CARTESIAN_POINT('Ctrl Pts',(-3.43101631893414,-1.,1.5198144909338));
#32482=CARTESIAN_POINT('Ctrl Pts',(-3.42946838852587,-1.,1.51914806898491));
#32483=CARTESIAN_POINT('Ctrl Pts',(-3.42884302333841,-1.,1.5189513329503));
#32484=CARTESIAN_POINT('Ctrl Pts',(-3.42864616361875,-1.,1.51893924967331));
#32485=CARTESIAN_POINT('Ctrl Pts',(-3.42859860294306,-1.,1.5189508286633));
#32486=CARTESIAN_POINT('',(-3.49844575334386,-1.,1.35032489087269));
#32487=CARTESIAN_POINT('Origin',(0.,-1.,0.));
#32488=CARTESIAN_POINT('',(-3.97027773754922,-1.,1.36999806084572));
#32489=CARTESIAN_POINT('Ctrl Pts',(-3.49844575334386,-1.,1.35032489087269));
#32490=CARTESIAN_POINT('Ctrl Pts',(-3.49847119623841,-1.,1.35036670893102));
#32491=CARTESIAN_POINT('Ctrl Pts',(-3.49861894124915,-1.,1.35049736560633));
#32492=CARTESIAN_POINT('Ctrl Pts',(-3.49920025459856,-1.,1.35080045218652));
#32493=CARTESIAN_POINT('Ctrl Pts',(-3.5007660381658,-1.,1.35142377279535));
#32494=CARTESIAN_POINT('Ctrl Pts',(-3.50408168106113,-1.,1.3525703284343));
#32495=CARTESIAN_POINT('Ctrl Pts',(-3.50913227060177,-1.,1.35419113576022));
#32496=CARTESIAN_POINT('Ctrl Pts',(-3.51542230699919,-1.,1.35611275237288));
#32497=CARTESIAN_POINT('Ctrl Pts',(-3.52261776117121,-1.,1.35821701528975));
#32498=CARTESIAN_POINT('Ctrl Pts',(-3.53034464961849,-1.,1.36037259643827));
#32499=CARTESIAN_POINT('Ctrl Pts',(-3.53824396425032,-1.,1.36245507339334));
#32500=CARTESIAN_POINT('Ctrl Pts',(-3.54602591832893,-1.,1.36436666257567));
#32501=CARTESIAN_POINT('Ctrl Pts',(-3.55353883995793,-1.,1.36606145456711));
#32502=CARTESIAN_POINT('Ctrl Pts',(-3.56077662028492,-1.,1.36754771771174));
#32503=CARTESIAN_POINT('Ctrl Pts',(-3.56782080304554,-1.,1.36886584973349));
#32504=CARTESIAN_POINT('Ctrl Pts',(-3.57479875549453,-1.,1.37007229485646));
#32505=CARTESIAN_POINT('Ctrl Pts',(-3.58183885982745,-1.,1.37122241663073));
#32506=CARTESIAN_POINT('Ctrl Pts',(-3.5890185384643,-1.,1.37235053661));
#32507=CARTESIAN_POINT('Ctrl Pts',(-3.59634627869117,-1.,1.37346320103184));
#32508=CARTESIAN_POINT('Ctrl Pts',(-3.60379020124038,-1.,1.37455051379642));
#32509=CARTESIAN_POINT('Ctrl Pts',(-3.61129546591082,-1.,1.37559314436641));
#32510=CARTESIAN_POINT('Ctrl Pts',(-3.61880481160408,-1.,1.37657053403102));
#32511=CARTESIAN_POINT('Ctrl Pts',(-3.62628098665112,-1.,1.37746987919868));
#32512=CARTESIAN_POINT('Ctrl Pts',(-3.63371727442448,-1.,1.37829035457324));
#32513=CARTESIAN_POINT('Ctrl Pts',(-3.64112507791112,-1.,1.37903818567347));
#32514=CARTESIAN_POINT('Ctrl Pts',(-3.64852652756444,-1.,1.37972372481598));
#32515=CARTESIAN_POINT('Ctrl Pts',(-3.65594554404396,-1.,1.38035791051215));
#32516=CARTESIAN_POINT('Ctrl Pts',(-3.66339848520874,-1.,1.38094856333558));
#32517=CARTESIAN_POINT('Ctrl Pts',(-3.67088843112282,-1.,1.38149812653876));
#32518=CARTESIAN_POINT('Ctrl Pts',(-3.6784103848243,-1.,1.38200574290626));
#32519=CARTESIAN_POINT('Ctrl Pts',(-3.68595444983844,-1.,1.38246852827185));
#32520=CARTESIAN_POINT('Ctrl Pts',(-3.69350967899523,-1.,1.38288311171649));
#32521=CARTESIAN_POINT('Ctrl Pts',(-3.70106792167894,-1.,1.38324717612862));
#32522=CARTESIAN_POINT('Ctrl Pts',(-3.70862680753343,-1.,1.38356065402122));
#32523=CARTESIAN_POINT('Ctrl Pts',(-3.7161876605181,-1.,1.38382489984585));
#32524=CARTESIAN_POINT('Ctrl Pts',(-3.72375409358805,-1.,1.3840421342895));
#32525=CARTESIAN_POINT('Ctrl Pts',(-3.73133035859283,-1.,1.38421479111531));
#32526=CARTESIAN_POINT('Ctrl Pts',(-3.73891976418099,-1.,1.38434489156456));
#32527=CARTESIAN_POINT('Ctrl Pts',(-3.7465231716786,-1.,1.38443344984389));
#32528=CARTESIAN_POINT('Ctrl Pts',(-3.75413976318727,-1.,1.38448077997155));
#32529=CARTESIAN_POINT('Ctrl Pts',(-3.76176768271347,-1.,1.38448675253343));
#32530=CARTESIAN_POINT('Ctrl Pts',(-3.76940473185775,-1.,1.38445107339517));
#32531=CARTESIAN_POINT('Ctrl Pts',(-3.77704902230441,-1.,1.38437354551435));
#32532=CARTESIAN_POINT('Ctrl Pts',(-3.78469969805134,-1.,1.38425435883773));
#32533=CARTESIAN_POINT('Ctrl Pts',(-3.79235669640907,-1.,1.38409399694588));
#32534=CARTESIAN_POINT('Ctrl Pts',(-3.80002044322169,-1.,1.38389311766701));
#32535=CARTESIAN_POINT('Ctrl Pts',(-3.80769156398429,-1.,1.38365244046226));
#32536=CARTESIAN_POINT('Ctrl Pts',(-3.81537060817765,-1.,1.38337263902766));
#32537=CARTESIAN_POINT('Ctrl Pts',(-3.82305771743715,-1.,1.38305421262724));
#32538=CARTESIAN_POINT('Ctrl Pts',(-3.83075266982138,-1.,1.38269750245086));
#32539=CARTESIAN_POINT('Ctrl Pts',(-3.83845502790609,-1.,1.38230274828774));
#32540=CARTESIAN_POINT('Ctrl Pts',(-3.84616425605705,-1.,1.38187013346089));
#32541=CARTESIAN_POINT('Ctrl Pts',(-3.85387983979557,-1.,1.38139983115075));
#32542=CARTESIAN_POINT('Ctrl Pts',(-3.86160143044187,-1.,1.38089205993067));
#32543=CARTESIAN_POINT('Ctrl Pts',(-3.86932885813403,-1.,1.38034709213129));
#32544=CARTESIAN_POINT('Ctrl Pts',(-3.87706205830865,-1.,1.37976523097187));
#32545=CARTESIAN_POINT('Ctrl Pts',(-3.88480102249461,-1.,1.37914679719446));
#32546=CARTESIAN_POINT('Ctrl Pts',(-3.89254574338385,-1.,1.37849211287981));
#32547=CARTESIAN_POINT('Ctrl Pts',(-3.90029615196255,-1.,1.3778014851263));
#32548=CARTESIAN_POINT('Ctrl Pts',(-3.90805209522729,-1.,1.3770751963376));
#32549=CARTESIAN_POINT('Ctrl Pts',(-3.91581337461825,-1.,1.37631350505516));
#32550=CARTESIAN_POINT('Ctrl Pts',(-3.92357976987132,-1.,1.37551664448057));
#32551=CARTESIAN_POINT('Ctrl Pts',(-3.93135106761941,-1.,1.37468482215784));
#32552=CARTESIAN_POINT('Ctrl Pts',(-3.93912709041791,-1.,1.37381821967499));
#32553=CARTESIAN_POINT('Ctrl Pts',(-3.94690771786926,-1.,1.37291699203423));
#32554=CARTESIAN_POINT('Ctrl Pts',(-3.95469287283105,-1.,1.37198126433139));
#32555=CARTESIAN_POINT('Ctrl Pts',(-3.96092458508407,-1.,1.37120515615663));
#32556=CARTESIAN_POINT('Ctrl Pts',(-3.96560037975788,-1.,1.37060761746027));
#32557=CARTESIAN_POINT('Ctrl Pts',(-3.9687184694173,-1.,1.37020239094758));
#32558=CARTESIAN_POINT('Ctrl Pts',(-3.97027773754922,-1.,1.36999806084572));
#32559=CARTESIAN_POINT('',(-4.01728681790024,-1.,1.22531898815164));
#32560=CARTESIAN_POINT('',(-3.97027773754922,-1.,1.36999806084572));
#32561=CARTESIAN_POINT('',(-3.62400312501199,-1.,0.963899035118985));
#32562=CARTESIAN_POINT('Ctrl Pts',(-4.01728681790024,-1.,1.22531898815164));
#32563=CARTESIAN_POINT('Ctrl Pts',(-4.01614544569895,-1.,1.22423716681317));
#32564=CARTESIAN_POINT('Ctrl Pts',(-4.01386104433519,-1.,1.22207656455845));
#32565=CARTESIAN_POINT('Ctrl Pts',(-4.01042947140789,-1.,1.21884478244403));
#32566=CARTESIAN_POINT('Ctrl Pts',(-4.00584409522722,-1.,1.21455398918133));
#32567=CARTESIAN_POINT('Ctrl Pts',(-4.00009577950721,-1.,1.20922097029551));
#32568=CARTESIAN_POINT('Ctrl Pts',(-3.99433084799666,-1.,1.20391852375139));
#32569=CARTESIAN_POINT('Ctrl Pts',(-3.98854928957189,-1.,1.19864679609566));
#32570=CARTESIAN_POINT('Ctrl Pts',(-3.98275111052561,-1.,1.19340598349475));
#32571=CARTESIAN_POINT('Ctrl Pts',(-3.97693634767754,-1.,1.18819633715539));
#32572=CARTESIAN_POINT('Ctrl Pts',(-3.97110505165415,-1.,1.18301815039831));
#32573=CARTESIAN_POINT('Ctrl Pts',(-3.96525726358159,-1.,1.17787174135592));
#32574=CARTESIAN_POINT('Ctrl Pts',(-3.95939299213276,-1.,1.17275743590361));
#32575=CARTESIAN_POINT('Ctrl Pts',(-3.95351219509876,-1.,1.16767555244438));
#32576=CARTESIAN_POINT('Ctrl Pts',(-3.94761474780583,-1.,1.16262637999157));
#32577=CARTESIAN_POINT('Ctrl Pts',(-3.94170046685203,-1.,1.15761018340956));
#32578=CARTESIAN_POINT('Ctrl Pts',(-3.9357691705628,-1.,1.1526272271632));
#32579=CARTESIAN_POINT('Ctrl Pts',(-3.92982073294257,-1.,1.14767779451123));
#32580=CARTESIAN_POINT('Ctrl Pts',(-3.92385513133997,-1.,1.14276220561593));
#32581=CARTESIAN_POINT('Ctrl Pts',(-3.91787251936827,-1.,1.13788084225554));
#32582=CARTESIAN_POINT('Ctrl Pts',(-3.91187321145649,-1.,1.13303414693896));
#32583=CARTESIAN_POINT('Ctrl Pts',(-3.90585753318737,-1.,1.12822258281553));
#32584=CARTESIAN_POINT('Ctrl Pts',(-3.89982569750025,-1.,1.12344660099043));
#32585=CARTESIAN_POINT('Ctrl Pts',(-3.89377768340344,-1.,1.11870660794603));
#32586=CARTESIAN_POINT('Ctrl Pts',(-3.88771308285171,-1.,1.11400292434429));
#32587=CARTESIAN_POINT('Ctrl Pts',(-3.88163105531724,-1.,1.10933577224008));
#32588=CARTESIAN_POINT('Ctrl Pts',(-3.87553067187514,-1.,1.10470536603287));
#32589=CARTESIAN_POINT('Ctrl Pts',(-3.86941120134849,-1.,1.10011198761195));
#32590=CARTESIAN_POINT('Ctrl Pts',(-3.86327241021247,-1.,1.09555606505013));
#32591=CARTESIAN_POINT('Ctrl Pts',(-3.85711487933931,-1.,1.09103825516294));
#32592=CARTESIAN_POINT('Ctrl Pts',(-3.85094025222713,-1.,1.08655950846384));
#32593=CARTESIAN_POINT('Ctrl Pts',(-3.8447504803063,-1.,1.08212087917991));
#32594=CARTESIAN_POINT('Ctrl Pts',(-3.83854714117491,-1.,1.07772335353858));
#32595=CARTESIAN_POINT('Ctrl Pts',(-3.83233071195144,-1.,1.07336766633459));
#32596=CARTESIAN_POINT('Ctrl Pts',(-3.82609989967276,-1.,1.06905413180359));
#32597=CARTESIAN_POINT('Ctrl Pts',(-3.81985083953012,-1.,1.0647824403893));
#32598=CARTESIAN_POINT('Ctrl Pts',(-3.8135786611749,-1.,1.06055206187299));
#32599=CARTESIAN_POINT('Ctrl Pts',(-3.80727913637791,-1.,1.05636266918644));
#32600=CARTESIAN_POINT('Ctrl Pts',(-3.80095039790681,-1.,1.05221457990016));
#32601=CARTESIAN_POINT('Ctrl Pts',(-3.79459440308786,-1.,1.04810913267639));
#32602=CARTESIAN_POINT('Ctrl Pts',(-3.78821910787179,-1.,1.04404924374422));
#32603=CARTESIAN_POINT('Ctrl Pts',(-3.7818353500817,-1.,1.04003862055798));
#32604=CARTESIAN_POINT('Ctrl Pts',(-3.77545283140427,-1.,1.03608074678008));
#32605=CARTESIAN_POINT('Ctrl Pts',(-3.76907609832516,-1.,1.03217786604919));
#32606=CARTESIAN_POINT('Ctrl Pts',(-3.76270122291245,-1.,1.02833014458184));
#32607=CARTESIAN_POINT('Ctrl Pts',(-3.75631037456224,-1.,1.02453429444668));
#32608=CARTESIAN_POINT('Ctrl Pts',(-3.74987777155873,-1.,1.02078510487439));
#32609=CARTESIAN_POINT('Ctrl Pts',(-3.74337942504993,-1.,1.01707794311088));
#32610=CARTESIAN_POINT('Ctrl Pts',(-3.73680245055747,-1.,1.01341114319906));
#32611=CARTESIAN_POINT('Ctrl Pts',(-3.73015276704407,-1.,1.00978798539491));
#32612=CARTESIAN_POINT('Ctrl Pts',(-3.72346803750544,-1.,1.00622000735696));
#32613=CARTESIAN_POINT('Ctrl Pts',(-3.71680667125047,-1.,1.00272423396802));
#32614=CARTESIAN_POINT('Ctrl Pts',(-3.7102243971387,-1.,0.999317260756344));
#32615=CARTESIAN_POINT('Ctrl Pts',(-3.70375282282107,-1.,0.996009819772431));
#32616=CARTESIAN_POINT('Ctrl Pts',(-3.69738123415696,-1.,0.992802218332103));
#32617=CARTESIAN_POINT('Ctrl Pts',(-3.69102682138955,-1.,0.989676715398858));
#32618=CARTESIAN_POINT('Ctrl Pts',(-3.6845531792623,-1.,0.986602639864285));
#32619=CARTESIAN_POINT('Ctrl Pts',(-3.67782408841876,-1.,0.983550791470864));
#32620=CARTESIAN_POINT('Ctrl Pts',(-3.67074983340444,-1.,0.980505922458494));
#32621=CARTESIAN_POINT('Ctrl Pts',(-3.66333049637403,-1.,0.977478312751416));
#32622=CARTESIAN_POINT('Ctrl Pts',(-3.6557157673487,-1.,0.974519971354138));
#32623=CARTESIAN_POINT('Ctrl Pts',(-3.64819756447072,-1.,0.971722122060277));
#32624=CARTESIAN_POINT('Ctrl Pts',(-3.64113946505393,-1.,0.969195124674829));
#32625=CARTESIAN_POINT('Ctrl Pts',(-3.6349212208096,-1.,0.967052554540877));
#32626=CARTESIAN_POINT('Ctrl Pts',(-3.62988252139998,-1.,0.965395153165716));
#32627=CARTESIAN_POINT('Ctrl Pts',(-3.62652618145252,-1.,0.964373850166081));
#32628=CARTESIAN_POINT('Ctrl Pts',(-3.62489305727516,-1.,0.963957782642589));
#32629=CARTESIAN_POINT('Ctrl Pts',(-3.62424461507455,-1.,0.963861297423579));
#32630=CARTESIAN_POINT('Ctrl Pts',(-3.62404828878375,-1.,0.963880158556713));
#32631=CARTESIAN_POINT('Ctrl Pts',(-3.62400312501199,-1.,0.963899035118985));
#32632=CARTESIAN_POINT('',(-3.66661143271648,-1.,0.786422660833743));
#32633=CARTESIAN_POINT('Origin',(0.,-1.,0.));
#32634=CARTESIAN_POINT('',(-4.13571194405636,-1.,0.732042837400619));
#32635=CARTESIAN_POINT('Ctrl Pts',(-3.66661143271648,-1.,0.786422660833743));
#32636=CARTESIAN_POINT('Ctrl Pts',(-3.66664310415236,-1.,0.786459983896781));
#32637=CARTESIAN_POINT('Ctrl Pts',(-3.66680946938396,-1.,0.78656591955989));
#32638=CARTESIAN_POINT('Ctrl Pts',(-3.66743103898844,-1.,0.786774337198499));
#32639=CARTESIAN_POINT('Ctrl Pts',(-3.66907505398769,-1.,0.787145041181588));
#32640=CARTESIAN_POINT('Ctrl Pts',(-3.672529236635,-1.,0.787758799995426));
#32641=CARTESIAN_POINT('Ctrl Pts',(-3.67777119516438,-1.,0.788569566220662));
#32642=CARTESIAN_POINT('Ctrl Pts',(-3.68428439784285,-1.,0.789483546065158));
#32643=CARTESIAN_POINT('Ctrl Pts',(-3.69172044327754,-1.,0.79043628498958));
#32644=CARTESIAN_POINT('Ctrl Pts',(-3.69968940808982,-1.,0.791356575696509));
#32645=CARTESIAN_POINT('Ctrl Pts',(-3.70781724021879,-1.,0.792177688845967));
#32646=CARTESIAN_POINT('Ctrl Pts',(-3.7158024239604,-1.,0.792848377370115));
#32647=CARTESIAN_POINT('Ctrl Pts',(-3.7234879729357,-1.,0.79334702378387));
#32648=CARTESIAN_POINT('Ctrl Pts',(-3.7308691469564,-1.,0.793682750269347));
#32649=CARTESIAN_POINT('Ctrl Pts',(-3.73803280541576,-1.,0.79388270093679));
#32650=CARTESIAN_POINT('Ctrl Pts',(-3.74511357728827,-1.,0.79398270045988));
#32651=CARTESIAN_POINT('Ctrl Pts',(-3.75224692493895,-1.,0.79401734737144));
#32652=CARTESIAN_POINT('Ctrl Pts',(-3.75951468666325,-1.,0.794008429135047));
#32653=CARTESIAN_POINT('Ctrl Pts',(-3.76692626931184,-1.,0.793961083689141));
#32654=CARTESIAN_POINT('Ctrl Pts',(-3.77444863801264,-1.,0.793870523787515));
#32655=CARTESIAN_POINT('Ctrl Pts',(-3.78202460377617,-1.,0.793726235781339));
#32656=CARTESIAN_POINT('Ctrl Pts',(-3.78959439439222,-1.,0.793516871680966));
#32657=CARTESIAN_POINT('Ctrl Pts',(-3.79711921389862,-1.,0.7932356129732));
#32658=CARTESIAN_POINT('Ctrl Pts',(-3.80459229925598,-1.,0.792882695234693));
#32659=CARTESIAN_POINT('Ctrl Pts',(-3.81202588694726,-1.,0.792462483517568));
#32660=CARTESIAN_POINT('Ctrl Pts',(-3.81944345442237,-1.,0.791981740718606));
#32661=CARTESIAN_POINT('Ctrl Pts',(-3.82687033899799,-1.,0.791447528662381));
#32662=CARTESIAN_POINT('Ctrl Pts',(-3.83432392054804,-1.,0.79086501270534));
#32663=CARTESIAN_POINT('Ctrl Pts',(-3.84180762342476,-1.,0.790236124191289));
#32664=CARTESIAN_POINT('Ctrl Pts',(-3.8493163780891,-1.,0.789560798155618));
#32665=CARTESIAN_POINT('Ctrl Pts',(-3.85683995872536,-1.,0.788837734090688));
#32666=CARTESIAN_POINT('Ctrl Pts',(-3.86436702561342,-1.,0.788065315093771));
#32667=CARTESIAN_POINT('Ctrl Pts',(-3.87188916600905,-1.,0.78724252761798));
#32668=CARTESIAN_POINT('Ctrl Pts',(-3.87940402818186,-1.,0.786369675812592));
#32669=CARTESIAN_POINT('Ctrl Pts',(-3.88691313167399,-1.,0.785447890340723));
#32670=CARTESIAN_POINT('Ctrl Pts',(-3.89442039235105,-1.,0.784478799358335));
#32671=CARTESIAN_POINT('Ctrl Pts',(-3.90193039043971,-1.,0.783464141529082));
#32672=CARTESIAN_POINT('Ctrl Pts',(-3.90944671004536,-1.,0.782405395622758));
#32673=CARTESIAN_POINT('Ctrl Pts',(-3.9169703605466,-1.,0.781303428618343));
#32674=CARTESIAN_POINT('Ctrl Pts',(-3.92450058323799,-1.,0.780158678615506));
#32675=CARTESIAN_POINT('Ctrl Pts',(-3.93203552473153,-1.,0.778971308134786));
#32676=CARTESIAN_POINT('Ctrl Pts',(-3.93957296768098,-1.,0.777741370568549));
#32677=CARTESIAN_POINT('Ctrl Pts',(-3.94711101619471,-1.,0.77646896669796));
#32678=CARTESIAN_POINT('Ctrl Pts',(-3.95464885452364,-1.,0.775154418039441));
#32679=CARTESIAN_POINT('Ctrl Pts',(-3.96218649639876,-1.,0.773798212026682));
#32680=CARTESIAN_POINT('Ctrl Pts',(-3.96972446532832,-1.,0.772400931772238));
#32681=CARTESIAN_POINT('Ctrl Pts',(-3.97726349165507,-1.,0.770963190030503));
#32682=CARTESIAN_POINT('Ctrl Pts',(-3.98480422348403,-1.,0.769485566245459));
#32683=CARTESIAN_POINT('Ctrl Pts',(-3.99234687880892,-1.,0.767968531377708));
#32684=CARTESIAN_POINT('Ctrl Pts',(-3.99989129179464,-1.,0.766412457135785));
#32685=CARTESIAN_POINT('Ctrl Pts',(-4.00743706791366,-1.,0.764817648784946));
#32686=CARTESIAN_POINT('Ctrl Pts',(-4.01498370680434,-1.,0.763184371182826));
#32687=CARTESIAN_POINT('Ctrl Pts',(-4.02253072741347,-1.,0.761512875859941));
#32688=CARTESIAN_POINT('Ctrl Pts',(-4.0300778195465,-1.,0.759803433244166));
#32689=CARTESIAN_POINT('Ctrl Pts',(-4.03762485803468,-1.,0.758056338885553));
#32690=CARTESIAN_POINT('Ctrl Pts',(-4.04517182654344,-1.,0.756271902370186));
#32691=CARTESIAN_POINT('Ctrl Pts',(-4.05271876688106,-1.,0.754450441816411));
#32692=CARTESIAN_POINT('Ctrl Pts',(-4.06026572221399,-1.,0.752592276482869));
#32693=CARTESIAN_POINT('Ctrl Pts',(-4.06781267241886,-1.,0.750697720483175));
#32694=CARTESIAN_POINT('Ctrl Pts',(-4.07535951055363,-1.,0.748767076679177));
#32695=CARTESIAN_POINT('Ctrl Pts',(-4.08290608094789,-1.,0.746800631490821));
#32696=CARTESIAN_POINT('Ctrl Pts',(-4.09045220253011,-1.,0.744798649705514));
#32697=CARTESIAN_POINT('Ctrl Pts',(-4.09799769702712,-1.,0.742761369690017));
#32698=CARTESIAN_POINT('Ctrl Pts',(-4.1055424175856,-1.,0.740688998555151));
#32699=CARTESIAN_POINT('Ctrl Pts',(-4.11308626953795,-1.,0.738581708229118));
#32700=CARTESIAN_POINT('Ctrl Pts',(-4.12062919626082,-1.,0.736439634335347));
#32701=CARTESIAN_POINT('Ctrl Pts',(-4.12666277572794,-1.,0.734698226767512));
#32702=CARTESIAN_POINT('Ctrl Pts',(-4.13118752796397,-1.,0.733376589325634));
#32703=CARTESIAN_POINT('Ctrl Pts',(-4.13420383737278,-1.,0.732488575135926));
#32704=CARTESIAN_POINT('Ctrl Pts',(-4.13571194405636,-1.,0.732042837400619));
#32705=CARTESIAN_POINT('',(-4.15950947128175,-1.,0.581791163835814));
#32706=CARTESIAN_POINT('',(-4.13571194405636,-1.,0.732042837400619));
#32707=CARTESIAN_POINT('',(-3.73017266276632,-1.,0.385112848332549));
#32708=CARTESIAN_POINT('Ctrl Pts',(-4.15950947128175,-1.,0.581791163835814));
#32709=CARTESIAN_POINT('Ctrl Pts',(-4.15821291712391,-1.,0.580901211462913));
#32710=CARTESIAN_POINT('Ctrl Pts',(-4.15561864787379,-1.,0.579124568912543));
#32711=CARTESIAN_POINT('Ctrl Pts',(-4.1517237611974,-1.,0.576469391673916));
#32712=CARTESIAN_POINT('Ctrl Pts',(-4.14652361065787,-1.,0.572948736066276));
#32713=CARTESIAN_POINT('Ctrl Pts',(-4.14001179828669,-1.,0.568580610187116));
#32714=CARTESIAN_POINT('Ctrl Pts',(-4.13348835726086,-1.,0.564245279535705));
#32715=CARTESIAN_POINT('Ctrl Pts',(-4.12695329951859,-1.,0.559942890594628));
#32716=CARTESIAN_POINT('Ctrl Pts',(-4.1204066619623,-1.,0.555673636130778));
#32717=CARTESIAN_POINT('Ctrl Pts',(-4.11384852025578,-1.,0.551437758498246));
#32718=CARTESIAN_POINT('Ctrl Pts',(-4.1072789702877,-1.,0.547235539486759));
#32719=CARTESIAN_POINT('Ctrl Pts',(-4.10069810244473,-1.,0.543067286878457));
#32720=CARTESIAN_POINT('Ctrl Pts',(-4.09410597627116,-1.,0.53893332117992));
#32721=CARTESIAN_POINT('Ctrl Pts',(-4.08750259988693,-1.,0.534833963476999));
#32722=CARTESIAN_POINT('Ctrl Pts',(-4.08088789536488,-1.,0.530769518728075));
#32723=CARTESIAN_POINT('Ctrl Pts',(-4.07426172299496,-1.,0.526740277226999));
#32724=CARTESIAN_POINT('Ctrl Pts',(-4.06762394471075,-1.,0.522746528602767));
#32725=CARTESIAN_POINT('Ctrl Pts',(-4.06097448037934,-1.,0.518788572336809));
#32726=CARTESIAN_POINT('Ctrl Pts',(-4.05431335771261,-1.,0.514866728193104));
#32727=CARTESIAN_POINT('Ctrl Pts',(-4.04764078815591,-1.,0.510981349219173));
#32728=CARTESIAN_POINT('Ctrl Pts',(-4.04095715149074,-1.,0.507132823288361));
#32729=CARTESIAN_POINT('Ctrl Pts',(-4.0342628417439,-1.,0.503321556915513));
#32730=CARTESIAN_POINT('Ctrl Pts',(-4.0275581398015,-1.,0.499547962340889));
#32731=CARTESIAN_POINT('Ctrl Pts',(-4.02084308851813,-1.,0.495812444326223));
#32732=CARTESIAN_POINT('Ctrl Pts',(-4.01411733503486,-1.,0.49211538341793));
#32733=CARTESIAN_POINT('Ctrl Pts',(-4.0073800839092,-1.,0.48845713042453));
#32734=CARTESIAN_POINT('Ctrl Pts',(-4.00063045119234,-1.,0.484838042421754));
#32735=CARTESIAN_POINT('Ctrl Pts',(-3.99386775880655,-1.,0.481258512209638));
#32736=CARTESIAN_POINT('Ctrl Pts',(-3.98709184306743,-1.,0.477718999122033));
#32737=CARTESIAN_POINT('Ctrl Pts',(-3.9803033804443,-1.,0.474220061019542));
#32738=CARTESIAN_POINT('Ctrl Pts',(-3.97350414289415,-1.,0.470762379613477));
#32739=CARTESIAN_POINT('Ctrl Pts',(-3.96669622273946,-1.,0.467346690880671));
#32740=CARTESIAN_POINT('Ctrl Pts',(-3.95988133243543,-1.,0.463973722115744));
#32741=CARTESIAN_POINT('Ctrl Pts',(-3.95306005817363,-1.,0.460644124429119));
#32742=CARTESIAN_POINT('Ctrl Pts',(-3.94623117206675,-1.,0.457358410451674));
#32743=CARTESIAN_POINT('Ctrl Pts',(-3.93939080846298,-1.,0.454116879027576));
#32744=CARTESIAN_POINT('Ctrl Pts',(-3.93253407403128,-1.,0.450919768356347));
#32745=CARTESIAN_POINT('Ctrl Pts',(-3.92565674143424,-1.,0.447767416837296));
#32746=CARTESIAN_POINT('Ctrl Pts',(-3.91875701610721,-1.,0.444660430230592));
#32747=CARTESIAN_POINT('Ctrl Pts',(-3.91183704069146,-1.,0.441599824524047));
#32748=CARTESIAN_POINT('Ctrl Pts',(-3.90490512938546,-1.,0.438587235458233));
#32749=CARTESIAN_POINT('Ctrl Pts',(-3.8979725665544,-1.,0.435624629433505));
#32750=CARTESIAN_POINT('Ctrl Pts',(-3.89104947940592,-1.,0.432713929544439));
#32751=CARTESIAN_POINT('Ctrl Pts',(-3.88414070943334,-1.,0.429856640579733));
#32752=CARTESIAN_POINT('Ctrl Pts',(-3.87724240306609,-1.,0.427053541173469));
#32753=CARTESIAN_POINT('Ctrl Pts',(-3.87033643487882,-1.,0.424304173195142));
#32754=CARTESIAN_POINT('Ctrl Pts',(-3.86339652542749,-1.,0.421607423177575));
#32755=CARTESIAN_POINT('Ctrl Pts',(-3.85639825648031,-1.,0.418962468086809));
#32756=CARTESIAN_POINT('Ctrl Pts',(-3.8493286415751,-1.,0.41636967805292));
#32757=CARTESIAN_POINT('Ctrl Pts',(-3.84219403994742,-1.,0.413831367016726));
#32758=CARTESIAN_POINT('Ctrl Pts',(-3.83503345578645,-1.,0.411353038798459));
#32759=CARTESIAN_POINT('Ctrl Pts',(-3.82790724256397,-1.,0.408942371447377));
#32760=CARTESIAN_POINT('Ctrl Pts',(-3.82087303913741,-1.,0.406607038258906));
#32761=CARTESIAN_POINT('Ctrl Pts',(-3.81396374287762,-1.,0.404352694628236));
#32762=CARTESIAN_POINT('Ctrl Pts',(-3.80716881962763,-1.,0.402181320148474));
#32763=CARTESIAN_POINT('Ctrl Pts',(-3.80040370384659,-1.,0.400088346504726));
#32764=CARTESIAN_POINT('Ctrl Pts',(-3.79352887163457,-1.,0.398064818684158));
#32765=CARTESIAN_POINT('Ctrl Pts',(-3.78640521279479,-1.,0.396103205335028));
#32766=CARTESIAN_POINT('Ctrl Pts',(-3.77894173114368,-1.,0.394202481011595));
#32767=CARTESIAN_POINT('Ctrl Pts',(-3.77114011595892,-1.,0.392372786223346));
#32768=CARTESIAN_POINT('Ctrl Pts',(-3.76315635032993,-1.,0.390642072979259));
#32769=CARTESIAN_POINT('Ctrl Pts',(-3.75529302894757,-1.,0.389054775898251));
#32770=CARTESIAN_POINT('Ctrl Pts',(-3.74792651696269,-1.,0.387663020050396));
#32771=CARTESIAN_POINT('Ctrl Pts',(-3.74144965781088,-1.,0.386519576222035));
#32772=CARTESIAN_POINT('Ctrl Pts',(-3.73621371845475,-1.,0.385670806454744));
#32773=CARTESIAN_POINT('Ctrl Pts',(-3.73273893363318,-1.,0.385187124633964));
#32774=CARTESIAN_POINT('Ctrl Pts',(-3.73106082862399,-1.,0.385031656499141));
#32775=CARTESIAN_POINT('Ctrl Pts',(-3.73040527620929,-1.,0.385037797882046));
#32776=CARTESIAN_POINT('Ctrl Pts',(-3.73021431755218,-1.,0.385087139001609));
#32777=CARTESIAN_POINT('Ctrl Pts',(-3.73017266276632,-1.,0.385112848332549));
#32778=CARTESIAN_POINT('',(-3.74449296982994,-1.,0.203156094897895));
#32779=CARTESIAN_POINT('Origin',(0.,-1.,0.));
#32780=CARTESIAN_POINT('',(-4.19931119685982,-1.,0.0760622897878236));
#32781=CARTESIAN_POINT('Ctrl Pts',(-3.74449296982994,-1.,0.203156094897895));
#32782=CARTESIAN_POINT('Ctrl Pts',(-3.74453008995129,-1.,0.203188003947965));
#32783=CARTESIAN_POINT('Ctrl Pts',(-3.74471097893961,-1.,0.203266610111264));
#32784=CARTESIAN_POINT('Ctrl Pts',(-3.74535749969262,-1.,0.203375226874331));
#32785=CARTESIAN_POINT('Ctrl Pts',(-3.74703926501843,-1.,0.203484186269314));
#32786=CARTESIAN_POINT('Ctrl Pts',(-3.75054693397716,-1.,0.203550035479097));
#32787=CARTESIAN_POINT('Ctrl Pts',(-3.75585118707924,-1.,0.203530796848403));
#32788=CARTESIAN_POINT('Ctrl Pts',(-3.76242717937273,-1.,0.203414634707646));
#32789=CARTESIAN_POINT('Ctrl Pts',(-3.76992071595267,-1.,0.203192390045337));
#32790=CARTESIAN_POINT('Ctrl Pts',(-3.77793553476879,-1.,0.202854729699196));
#32791=CARTESIAN_POINT('Ctrl Pts',(-3.78609175019317,-1.,0.202394260512193));
#32792=CARTESIAN_POINT('Ctrl Pts',(-3.79408354187274,-1.,0.201807533800799));
#32793=CARTESIAN_POINT('Ctrl Pts',(-3.80175247447171,-1.,0.201097756307252));
#32794=CARTESIAN_POINT('Ctrl Pts',(-3.80909529318501,-1.,0.20027467943329));
#32795=CARTESIAN_POINT('Ctrl Pts',(-3.81620203429702,-1.,0.199351525297396));
#32796=CARTESIAN_POINT('Ctrl Pts',(-3.82321127348981,-1.,0.19834261690047));
#32797=CARTESIAN_POINT('Ctrl Pts',(-3.83026221776488,-1.,0.197260935827375));
#32798=CARTESIAN_POINT('Ctrl Pts',(-3.83743910616265,-1.,0.196115198971889));
#32799=CARTESIAN_POINT('Ctrl Pts',(-3.84475203347052,-1.,0.194909009460254));
#32800=CARTESIAN_POINT('Ctrl Pts',(-3.85216762264019,-1.,0.193642806777747));
#32801=CARTESIAN_POINT('Ctrl Pts',(-3.85962774407652,-1.,0.192315153044979));
#32802=CARTESIAN_POINT('Ctrl Pts',(-3.8670715862477,-1.,0.190924190418613));
#32803=CARTESIAN_POINT('Ctrl Pts',(-3.87445976418377,-1.,0.189469253358254));
#32804=CARTESIAN_POINT('Ctrl Pts',(-3.88178563496187,-1.,0.187951632512663));
#32805=CARTESIAN_POINT('Ctrl Pts',(-3.88906196725817,-1.,0.186373724985263));
#32806=CARTESIAN_POINT('Ctrl Pts',(-3.89631300742633,-1.,0.184738537728035));
#32807=CARTESIAN_POINT('Ctrl Pts',(-3.90356488555138,-1.,0.183049081993193));
#32808=CARTESIAN_POINT('Ctrl Pts',(-3.91083557557193,-1.,0.181307740731796));
#32809=CARTESIAN_POINT('Ctrl Pts',(-3.91812876180948,-1.,0.179515885822894));
#32810=CARTESIAN_POINT('Ctrl Pts',(-3.92543942697672,-1.,0.177674246152328));
#32811=CARTESIAN_POINT('Ctrl Pts',(-3.93275726771049,-1.,0.175783136893872));
#32812=CARTESIAN_POINT('Ctrl Pts',(-3.94007083096214,-1.,0.173842734974607));
#32813=CARTESIAN_POINT('Ctrl Pts',(-3.94737164900861,-1.,0.171853355369233));
#32814=CARTESIAN_POINT('Ctrl Pts',(-3.95465744665263,-1.,0.16981566637413));
#32815=CARTESIAN_POINT('Ctrl Pts',(-3.96192990160296,-1.,0.167730547023312));
#32816=CARTESIAN_POINT('Ctrl Pts',(-3.9691931362141,-1.,0.165598992851097));
#32817=CARTESIAN_POINT('Ctrl Pts',(-3.97645194630944,-1.,0.163422004609999));
#32818=CARTESIAN_POINT('Ctrl Pts',(-3.98371010319866,-1.,0.161200482186087));
#32819=CARTESIAN_POINT('Ctrl Pts',(-3.99096873945862,-1.,0.158935123982796));
#32820=CARTESIAN_POINT('Ctrl Pts',(-3.99822717425869,-1.,0.156626481393735));
#32821=CARTESIAN_POINT('Ctrl Pts',(-4.00548360245297,-1.,0.15427500487231));
#32822=CARTESIAN_POINT('Ctrl Pts',(-4.01273584234684,-1.,0.151881094022909));
#32823=CARTESIAN_POINT('Ctrl Pts',(-4.01998203715588,-1.,0.149445144968707));
#32824=CARTESIAN_POINT('Ctrl Pts',(-4.02722143147048,-1.,0.146967602878998));
#32825=CARTESIAN_POINT('Ctrl Pts',(-4.03445411510403,-1.,0.144448947038352));
#32826=CARTESIAN_POINT('Ctrl Pts',(-4.04168069633842,-1.,0.141889671485508));
#32827=CARTESIAN_POINT('Ctrl Pts',(-4.04890199238056,-1.,0.139290267180059));
#32828=CARTESIAN_POINT('Ctrl Pts',(-4.05611873400122,-1.,0.136651205046111));
#32829=CARTESIAN_POINT('Ctrl Pts',(-4.06333121018476,-1.,0.133972916144225));
#32830=CARTESIAN_POINT('Ctrl Pts',(-4.07053931528579,-1.,0.131255793548914));
#32831=CARTESIAN_POINT('Ctrl Pts',(-4.07774270738809,-1.,0.128500200484814));
#32832=CARTESIAN_POINT('Ctrl Pts',(-4.08494093372315,-1.,0.125706476822529));
#32833=CARTESIAN_POINT('Ctrl Pts',(-4.09213355850836,-1.,0.122874946249119));
#32834=CARTESIAN_POINT('Ctrl Pts',(-4.09932031767243,-1.,0.120005924388162));
#32835=CARTESIAN_POINT('Ctrl Pts',(-4.10650113382187,-1.,0.117099722731704));
#32836=CARTESIAN_POINT('Ctrl Pts',(-4.11367603925313,-1.,0.114156649609601));
#32837=CARTESIAN_POINT('Ctrl Pts',(-4.12084512502444,-1.,0.111177012683377));
#32838=CARTESIAN_POINT('Ctrl Pts',(-4.12800848371386,-1.,0.10816112052835));
#32839=CARTESIAN_POINT('Ctrl Pts',(-4.13516614458396,-1.,0.105109286538864));
#32840=CARTESIAN_POINT('Ctrl Pts',(-4.14231804938737,-1.,0.102021826577454));
#32841=CARTESIAN_POINT('Ctrl Pts',(-4.1494640891762,-1.,0.0988990478899811));
#32842=CARTESIAN_POINT('Ctrl Pts',(-4.15660412653006,-1.,0.0957412403297067));
#32843=CARTESIAN_POINT('Ctrl Pts',(-4.16373802265942,-1.,0.092548667216769));
#32844=CARTESIAN_POINT('Ctrl Pts',(-4.17086566491823,-1.,0.0893215560850327));
#32845=CARTESIAN_POINT('Ctrl Pts',(-4.17798698669991,-1.,0.0860600915552515));
#32846=CARTESIAN_POINT('Ctrl Pts',(-4.1851019532944,-1.,0.082764416438951));
#32847=CARTESIAN_POINT('Ctrl Pts',(-4.19078883322483,-1.,0.0801005887117603));
#32848=CARTESIAN_POINT('Ctrl Pts',(-4.19505112860624,-1.,0.0780873956244402));
#32849=CARTESIAN_POINT('Ctrl Pts',(-4.19789138621624,-1.,0.0767384596142195));
#32850=CARTESIAN_POINT('Ctrl Pts',(-4.19931119685982,-1.,0.0760622897878236));
#32851=CARTESIAN_POINT('',(-4.19931119685982,-1.,-0.0760622897878246));
#32852=CARTESIAN_POINT('',(-4.19931119685982,-1.,0.0760622897878236));
#32853=CARTESIAN_POINT('',(-3.74449296983004,-1.,-0.203156094896101));
#32854=CARTESIAN_POINT('Ctrl Pts',(-4.19931119685982,-1.,-0.0760622897878246));
#32855=CARTESIAN_POINT('Ctrl Pts',(-4.1978913862118,-1.,-0.0767384596141464));
#32856=CARTESIAN_POINT('Ctrl Pts',(-4.19505112859416,-1.,-0.0780873956242397));
#32857=CARTESIAN_POINT('Ctrl Pts',(-4.19078883320504,-1.,-0.080100588711432));
#32858=CARTESIAN_POINT('Ctrl Pts',(-4.18510195327123,-1.,-0.0827644164385679));
#32859=CARTESIAN_POINT('Ctrl Pts',(-4.17798698668094,-1.,-0.0860600915549397));
#32860=CARTESIAN_POINT('Ctrl Pts',(-4.17086566490794,-1.,-0.0893215560848649));
#32861=CARTESIAN_POINT('Ctrl Pts',(-4.16373802265839,-1.,-0.0925486672167531));
#32862=CARTESIAN_POINT('Ctrl Pts',(-4.15660412653577,-1.,-0.0957412403298007));
#32863=CARTESIAN_POINT('Ctrl Pts',(-4.14946408918485,-1.,-0.0988990478901226));
#32864=CARTESIAN_POINT('Ctrl Pts',(-4.14231804939538,-1.,-0.102021826577584));
#32865=CARTESIAN_POINT('Ctrl Pts',(-4.13516614458895,-1.,-0.105109286538945));
#32866=CARTESIAN_POINT('Ctrl Pts',(-4.12800848371504,-1.,-0.108161120528369));
#32867=CARTESIAN_POINT('Ctrl Pts',(-4.1208451250225,-1.,-0.111177012683347));
#32868=CARTESIAN_POINT('Ctrl Pts',(-4.11367603924961,-1.,-0.114156649609546));
#32869=CARTESIAN_POINT('Ctrl Pts',(-4.10650113381833,-1.,-0.117099722731648));
#32870=CARTESIAN_POINT('Ctrl Pts',(-4.09932031767002,-1.,-0.120005924388124));
#32871=CARTESIAN_POINT('Ctrl Pts',(-4.09213355850756,-1.,-0.122874946249107));
#32872=CARTESIAN_POINT('Ctrl Pts',(-4.08494093372377,-1.,-0.12570647682254));
#32873=CARTESIAN_POINT('Ctrl Pts',(-4.07774270738954,-1.,-0.128500200484838));
#32874=CARTESIAN_POINT('Ctrl Pts',(-4.0705393152874,-1.,-0.13125579354894));
#32875=CARTESIAN_POINT('Ctrl Pts',(-4.06333121018596,-1.,-0.133972916144245));
#32876=CARTESIAN_POINT('Ctrl Pts',(-4.05611873400172,-1.,-0.136651205046119));
#32877=CARTESIAN_POINT('Ctrl Pts',(-4.04890199238036,-1.,-0.139290267180057));
#32878=CARTESIAN_POINT('Ctrl Pts',(-4.04168069633781,-1.,-0.1418896714855));
#32879=CARTESIAN_POINT('Ctrl Pts',(-4.03445411510333,-1.,-0.144448947038345));
#32880=CARTESIAN_POINT('Ctrl Pts',(-4.02722143146994,-1.,-0.146967602878994));
#32881=CARTESIAN_POINT('Ctrl Pts',(-4.01998203715564,-1.,-0.149445144968707));
#32882=CARTESIAN_POINT('Ctrl Pts',(-4.01273584234689,-1.,-0.151881094022911));
#32883=CARTESIAN_POINT('Ctrl Pts',(-4.00548360245319,-1.,-0.154275004872311));
#32884=CARTESIAN_POINT('Ctrl Pts',(-3.99822717425893,-1.,-0.156626481393734));
#32885=CARTESIAN_POINT('Ctrl Pts',(-3.99096873945878,-1.,-0.158935123982793));
#32886=CARTESIAN_POINT('Ctrl Pts',(-3.98371010319872,-1.,-0.161200482186085));
#32887=CARTESIAN_POINT('Ctrl Pts',(-3.97645194630943,-1.,-0.163422004609999));
#32888=CARTESIAN_POINT('Ctrl Pts',(-3.96919313621407,-1.,-0.165598992851102));
#32889=CARTESIAN_POINT('Ctrl Pts',(-3.96192990160296,-1.,-0.167730547023319));
#32890=CARTESIAN_POINT('Ctrl Pts',(-3.95465744665268,-1.,-0.169815666374139));
#32891=CARTESIAN_POINT('Ctrl Pts',(-3.94737164900868,-1.,-0.17185335536924));
#32892=CARTESIAN_POINT('Ctrl Pts',(-3.94007083096217,-1.,-0.17384273497461));
#32893=CARTESIAN_POINT('Ctrl Pts',(-3.93275726771042,-1.,-0.175783136893868));
#32894=CARTESIAN_POINT('Ctrl Pts',(-3.92543942697655,-1.,-0.177674246152317));
#32895=CARTESIAN_POINT('Ctrl Pts',(-3.91812876180926,-1.,-0.179515885822882));
#32896=CARTESIAN_POINT('Ctrl Pts',(-3.91083557557175,-1.,-0.181307740731786));
#32897=CARTESIAN_POINT('Ctrl Pts',(-3.90356488555132,-1.,-0.183049081993191));
#32898=CARTESIAN_POINT('Ctrl Pts',(-3.89631300742646,-1.,-0.184738537728043));
#32899=CARTESIAN_POINT('Ctrl Pts',(-3.88906196725848,-1.,-0.18637372498528));
#32900=CARTESIAN_POINT('Ctrl Pts',(-3.88178563496228,-1.,-0.187951632512685));
#32901=CARTESIAN_POINT('Ctrl Pts',(-3.87445976418412,-1.,-0.189469253358272));
#32902=CARTESIAN_POINT('Ctrl Pts',(-3.86707158624783,-1.,-0.19092419041862));
#32903=CARTESIAN_POINT('Ctrl Pts',(-3.85962774407633,-1.,-0.192315153044971));
#32904=CARTESIAN_POINT('Ctrl Pts',(-3.85216762263966,-1.,-0.193642806777723));
#32905=CARTESIAN_POINT('Ctrl Pts',(-3.84475203346977,-1.,-0.194909009460221));
#32906=CARTESIAN_POINT('Ctrl Pts',(-3.83743910616195,-1.,-0.196115198971859));
#32907=CARTESIAN_POINT('Ctrl Pts',(-3.83026221776456,-1.,-0.197260935827361));
#32908=CARTESIAN_POINT('Ctrl Pts',(-3.82321127349016,-1.,-0.198342616900486));
#32909=CARTESIAN_POINT('Ctrl Pts',(-3.81620203429815,-1.,-0.199351525297447));
#32910=CARTESIAN_POINT('Ctrl Pts',(-3.80909529318669,-1.,-0.200274679433364));
#32911=CARTESIAN_POINT('Ctrl Pts',(-3.80175247447337,-1.,-0.201097756307326));
#32912=CARTESIAN_POINT('Ctrl Pts',(-3.7940835418736,-1.,-0.201807533800837));
#32913=CARTESIAN_POINT('Ctrl Pts',(-3.78609175019242,-1.,-0.20239426051216));
#32914=CARTESIAN_POINT('Ctrl Pts',(-3.77793553476614,-1.,-0.202854729699081));
#32915=CARTESIAN_POINT('Ctrl Pts',(-3.7699207159487,-1.,-0.203192390045164));
#32916=CARTESIAN_POINT('Ctrl Pts',(-3.76242717936885,-1.,-0.203414634707478));
#32917=CARTESIAN_POINT('Ctrl Pts',(-3.75585118707734,-1.,-0.203530796848322));
#32918=CARTESIAN_POINT('Ctrl Pts',(-3.75054693397875,-1.,-0.203550035479166));
#32919=CARTESIAN_POINT('Ctrl Pts',(-3.74703926501752,-1.,-0.203484186269415));
#32920=CARTESIAN_POINT('Ctrl Pts',(-3.74535749969115,-1.,-0.203375226874121));
#32921=CARTESIAN_POINT('Ctrl Pts',(-3.74471097893845,-1.,-0.203266610110531));
#32922=CARTESIAN_POINT('Ctrl Pts',(-3.74453008995092,-1.,-0.203188003946657));
#32923=CARTESIAN_POINT('Ctrl Pts',(-3.74449296983004,-1.,-0.203156094896101));
#32924=CARTESIAN_POINT('',(-3.73017266276651,-1.,-0.385112848330762));
#32925=CARTESIAN_POINT('Origin',(0.,-1.,0.));
#32926=CARTESIAN_POINT('',(-4.15950947128175,-1.,-0.581791163835815));
#32927=CARTESIAN_POINT('Ctrl Pts',(-3.73017266276651,-1.,-0.385112848330762));
#32928=CARTESIAN_POINT('Ctrl Pts',(-3.73021431755274,-1.,-0.385087139000374));
#32929=CARTESIAN_POINT('Ctrl Pts',(-3.73040527621055,-1.,-0.385037797881504));
#32930=CARTESIAN_POINT('Ctrl Pts',(-3.73106082862548,-1.,-0.385031656499164));
#32931=CARTESIAN_POINT('Ctrl Pts',(-3.73273893363406,-1.,-0.385187124634206));
#32932=CARTESIAN_POINT('Ctrl Pts',(-3.73621371845318,-1.,-0.385670806454566));
#32933=CARTESIAN_POINT('Ctrl Pts',(-3.74144965781276,-1.,-0.386519576222251));
#32934=CARTESIAN_POINT('Ctrl Pts',(-3.74792651696654,-1.,-0.387663020050836));
#32935=CARTESIAN_POINT('Ctrl Pts',(-3.75529302895152,-1.,-0.389054775898702));
#32936=CARTESIAN_POINT('Ctrl Pts',(-3.76315635033257,-1.,-0.39064207297956));
#32937=CARTESIAN_POINT('Ctrl Pts',(-3.77114011595967,-1.,-0.392372786223432));
#32938=CARTESIAN_POINT('Ctrl Pts',(-3.77894173114283,-1.,-0.394202481011499));
#32939=CARTESIAN_POINT('Ctrl Pts',(-3.78640521279313,-1.,-0.396103205334841));
#32940=CARTESIAN_POINT('Ctrl Pts',(-3.7935288716329,-1.,-0.398064818683969));
#32941=CARTESIAN_POINT('Ctrl Pts',(-3.80040370384546,-1.,-0.4000883465046));
#32942=CARTESIAN_POINT('Ctrl Pts',(-3.80716881962728,-1.,-0.402181320148436));
#32943=CARTESIAN_POINT('Ctrl Pts',(-3.81396374287793,-1.,-0.404352694628273));
#32944=CARTESIAN_POINT('Ctrl Pts',(-3.8208730391381,-1.,-0.406607038258985));
#32945=CARTESIAN_POINT('Ctrl Pts',(-3.82790724256471,-1.,-0.40894237144746));
#32946=CARTESIAN_POINT('Ctrl Pts',(-3.83503345578698,-1.,-0.411353038798518));
#32947=CARTESIAN_POINT('Ctrl Pts',(-3.84219403994762,-1.,-0.413831367016748));
#32948=CARTESIAN_POINT('Ctrl Pts',(-3.84932864157497,-1.,-0.416369678052907));
#32949=CARTESIAN_POINT('Ctrl Pts',(-3.85639825647996,-1.,-0.418962468086773));
#32950=CARTESIAN_POINT('Ctrl Pts',(-3.86339652542709,-1.,-0.421607423177534));
#32951=CARTESIAN_POINT('Ctrl Pts',(-3.87033643487851,-1.,-0.424304173195111));
#32952=CARTESIAN_POINT('Ctrl Pts',(-3.87724240306597,-1.,-0.427053541173457));
#32953=CARTESIAN_POINT('Ctrl Pts',(-3.88414070943341,-1.,-0.429856640579741));
#32954=CARTESIAN_POINT('Ctrl Pts',(-3.89104947940611,-1.,-0.432713929544458));
#32955=CARTESIAN_POINT('Ctrl Pts',(-3.89797256655462,-1.,-0.435624629433527));
#32956=CARTESIAN_POINT('Ctrl Pts',(-3.90490512938563,-1.,-0.438587235458249));
#32957=CARTESIAN_POINT('Ctrl Pts',(-3.91183704069153,-1.,-0.441599824524054));
#32958=CARTESIAN_POINT('Ctrl Pts',(-3.91875701610719,-1.,-0.444660430230591));
#32959=CARTESIAN_POINT('Ctrl Pts',(-3.92565674143416,-1.,-0.447767416837292));
#32960=CARTESIAN_POINT('Ctrl Pts',(-3.93253407403123,-1.,-0.450919768356348));
#32961=CARTESIAN_POINT('Ctrl Pts',(-3.93939080846298,-1.,-0.454116879027584));
#32962=CARTESIAN_POINT('Ctrl Pts',(-3.94623117206678,-1.,-0.457358410451683));
#32963=CARTESIAN_POINT('Ctrl Pts',(-3.95306005817364,-1.,-0.460644124429121));
#32964=CARTESIAN_POINT('Ctrl Pts',(-3.95988133243538,-1.,-0.463973722115733));
#32965=CARTESIAN_POINT('Ctrl Pts',(-3.9666962227393,-1.,-0.467346690880643));
#32966=CARTESIAN_POINT('Ctrl Pts',(-3.97350414289392,-1.,-0.470762379613439));
#32967=CARTESIAN_POINT('Ctrl Pts',(-3.98030338044409,-1.,-0.47422006101951));
#32968=CARTESIAN_POINT('Ctrl Pts',(-3.98709184306738,-1.,-0.477718999122027));
#32969=CARTESIAN_POINT('Ctrl Pts',(-3.99386775880679,-1.,-0.481258512209675));
#32970=CARTESIAN_POINT('Ctrl Pts',(-4.00063045119288,-1.,-0.484838042421835));
#32971=CARTESIAN_POINT('Ctrl Pts',(-4.0073800839099,-1.,-0.488457130424633));
#32972=CARTESIAN_POINT('Ctrl Pts',(-4.01411733503546,-1.,-0.492115383418018));
#32973=CARTESIAN_POINT('Ctrl Pts',(-4.02084308851832,-1.,-0.495812444326251));
#32974=CARTESIAN_POINT('Ctrl Pts',(-4.02755813980101,-1.,-0.499547962340821));
#32975=CARTESIAN_POINT('Ctrl Pts',(-4.03426284174272,-1.,-0.503321556915346));
#32976=CARTESIAN_POINT('Ctrl Pts',(-4.04095715148915,-1.,-0.507132823288136));
#32977=CARTESIAN_POINT('Ctrl Pts',(-4.04764078815447,-1.,-0.51098134921897));
#32978=CARTESIAN_POINT('Ctrl Pts',(-4.05431335771199,-1.,-0.514866728193017));
#32979=CARTESIAN_POINT('Ctrl Pts',(-4.06097448038013,-1.,-0.518788572336923));
#32980=CARTESIAN_POINT('Ctrl Pts',(-4.06762394471314,-1.,-0.522746528603107));
#32981=CARTESIAN_POINT('Ctrl Pts',(-4.07426172299847,-1.,-0.526740277227498));
#32982=CARTESIAN_POINT('Ctrl Pts',(-4.08088789536836,-1.,-0.530769518728571));
#32983=CARTESIAN_POINT('Ctrl Pts',(-4.08750259988885,-1.,-0.534833963477273));
#32984=CARTESIAN_POINT('Ctrl Pts',(-4.09410597627,-1.,-0.538933321179756));
#32985=CARTESIAN_POINT('Ctrl Pts',(-4.10069810243979,-1.,-0.543067286877757));
#32986=CARTESIAN_POINT('Ctrl Pts',(-4.10727897027977,-1.,-0.547235539485637));
#32987=CARTESIAN_POINT('Ctrl Pts',(-4.11384852024721,-1.,-0.551437758497032));
#32988=CARTESIAN_POINT('Ctrl Pts',(-4.12040666195664,-1.,-0.555673636129977));
#32989=CARTESIAN_POINT('Ctrl Pts',(-4.12695329951961,-1.,-0.559942890594773));
#32990=CARTESIAN_POINT('Ctrl Pts',(-4.13348835727104,-1.,-0.564245279537148));
#32991=CARTESIAN_POINT('Ctrl Pts',(-4.14001179830547,-1.,-0.568580610189774));
#32992=CARTESIAN_POINT('Ctrl Pts',(-4.14652361068081,-1.,-0.572948736069522));
#32993=CARTESIAN_POINT('Ctrl Pts',(-4.151723761217,-1.,-0.576469391676688));
#32994=CARTESIAN_POINT('Ctrl Pts',(-4.15561864788576,-1.,-0.579124568914235));
#32995=CARTESIAN_POINT('Ctrl Pts',(-4.1582129171283,-1.,-0.580901211463535));
#32996=CARTESIAN_POINT('Ctrl Pts',(-4.15950947128175,-1.,-0.581791163835815));
#32997=CARTESIAN_POINT('',(-4.13571194405636,-1.,-0.73204283740062));
#32998=CARTESIAN_POINT('',(-4.15950947128175,-1.,-0.581791163835815));
#32999=CARTESIAN_POINT('',(-3.66661143271685,-1.,-0.786422660831985));
#33000=CARTESIAN_POINT('Ctrl Pts',(-4.13571194405636,-1.,-0.73204283740062));
#33001=CARTESIAN_POINT('Ctrl Pts',(-4.1342038373684,-1.,-0.732488575135159));
#33002=CARTESIAN_POINT('Ctrl Pts',(-4.13118752795207,-1.,-0.733376589323546));
#33003=CARTESIAN_POINT('Ctrl Pts',(-4.12666277570844,-1.,-0.734698226764092));
#33004=CARTESIAN_POINT('Ctrl Pts',(-4.120629196238,-1.,-0.736439634331345));
#33005=CARTESIAN_POINT('Ctrl Pts',(-4.11308626951927,-1.,-0.738581708225844));
#33006=CARTESIAN_POINT('Ctrl Pts',(-4.10554241757547,-1.,-0.740688998553377));
#33007=CARTESIAN_POINT('Ctrl Pts',(-4.09799769702611,-1.,-0.742761369689841));
#33008=CARTESIAN_POINT('Ctrl Pts',(-4.09045220253573,-1.,-0.7447986497065));
#33009=CARTESIAN_POINT('Ctrl Pts',(-4.08290608095642,-1.,-0.746800631492315));
#33010=CARTESIAN_POINT('Ctrl Pts',(-4.07535951056152,-1.,-0.748767076680557));
#33011=CARTESIAN_POINT('Ctrl Pts',(-4.06781267242378,-1.,-0.750697720484036));
#33012=CARTESIAN_POINT('Ctrl Pts',(-4.06026572221515,-1.,-0.752592276483072));
#33013=CARTESIAN_POINT('Ctrl Pts',(-4.05271876687915,-1.,-0.754450441816078));
#33014=CARTESIAN_POINT('Ctrl Pts',(-4.04517182653997,-1.,-0.756271902369581));
#33015=CARTESIAN_POINT('Ctrl Pts',(-4.03762485803119,-1.,-0.758056338884944));
#33016=CARTESIAN_POINT('Ctrl Pts',(-4.03007781954412,-1.,-0.759803433243752));
#33017=CARTESIAN_POINT('Ctrl Pts',(-4.02253072741268,-1.,-0.761512875859804));
#33018=CARTESIAN_POINT('Ctrl Pts',(-4.01498370680496,-1.,-0.763184371182935));
#33019=CARTESIAN_POINT('Ctrl Pts',(-4.00743706791509,-1.,-0.764817648785197));
#33020=CARTESIAN_POINT('Ctrl Pts',(-3.99989129179622,-1.,-0.766412457136064));
#33021=CARTESIAN_POINT('Ctrl Pts',(-3.9923468788101,-1.,-0.767968531377915));
#33022=CARTESIAN_POINT('Ctrl Pts',(-3.98480422348451,-1.,-0.769485566245544));
#33023=CARTESIAN_POINT('Ctrl Pts',(-3.97726349165488,-1.,-0.770963190030471));
#33024=CARTESIAN_POINT('Ctrl Pts',(-3.96972446532772,-1.,-0.772400931772136));
#33025=CARTESIAN_POINT('Ctrl Pts',(-3.96218649639807,-1.,-0.773798212026565));
#33026=CARTESIAN_POINT('Ctrl Pts',(-3.9546488545231,-1.,-0.775154418039351));
#33027=CARTESIAN_POINT('Ctrl Pts',(-3.94711101619447,-1.,-0.776468966697921));
#33028=CARTESIAN_POINT('Ctrl Pts',(-3.93957296768103,-1.,-0.777741370568558));
#33029=CARTESIAN_POINT('Ctrl Pts',(-3.93203552473174,-1.,-0.778971308134821));
#33030=CARTESIAN_POINT('Ctrl Pts',(-3.92450058323823,-1.,-0.780158678615542));
#33031=CARTESIAN_POINT('Ctrl Pts',(-3.91697036054676,-1.,-0.781303428618366));
#33032=CARTESIAN_POINT('Ctrl Pts',(-3.90944671004542,-1.,-0.782405395622764));
#33033=CARTESIAN_POINT('Ctrl Pts',(-3.9019303904397,-1.,-0.783464141529081));
#33034=CARTESIAN_POINT('Ctrl Pts',(-3.89442039235103,-1.,-0.784478799358336));
#33035=CARTESIAN_POINT('Ctrl Pts',(-3.88691313167398,-1.,-0.78544789034073));
#33036=CARTESIAN_POINT('Ctrl Pts',(-3.8794040281819,-1.,-0.786369675812608));
#33037=CARTESIAN_POINT('Ctrl Pts',(-3.87188916600912,-1.,-0.787242527617999));
#33038=CARTESIAN_POINT('Ctrl Pts',(-3.86436702561345,-1.,-0.788065315093777));
#33039=CARTESIAN_POINT('Ctrl Pts',(-3.85683995872529,-1.,-0.788837734090672));
#33040=CARTESIAN_POINT('Ctrl Pts',(-3.84931637808894,-1.,-0.789560798155582));
#33041=CARTESIAN_POINT('Ctrl Pts',(-3.84180762342454,-1.,-0.790236124191242));
#33042=CARTESIAN_POINT('Ctrl Pts',(-3.83432392054786,-1.,-0.790865012705301));
#33043=CARTESIAN_POINT('Ctrl Pts',(-3.82687033899792,-1.,-0.791447528662369));
#33044=CARTESIAN_POINT('Ctrl Pts',(-3.81944345442249,-1.,-0.791981740718635));
#33045=CARTESIAN_POINT('Ctrl Pts',(-3.81202588694756,-1.,-0.792462483517634));
#33046=CARTESIAN_POINT('Ctrl Pts',(-3.80459229925637,-1.,-0.792882695234778));
#33047=CARTESIAN_POINT('Ctrl Pts',(-3.79711921389897,-1.,-0.793235612973273));
#33048=CARTESIAN_POINT('Ctrl Pts',(-3.78959439439235,-1.,-0.793516871680993));
#33049=CARTESIAN_POINT('Ctrl Pts',(-3.78202460377598,-1.,-0.7937262357813));
#33050=CARTESIAN_POINT('Ctrl Pts',(-3.77444863801212,-1.,-0.793870523787408));
#33051=CARTESIAN_POINT('Ctrl Pts',(-3.76692626931111,-1.,-0.793961083688991));
#33052=CARTESIAN_POINT('Ctrl Pts',(-3.75951468666257,-1.,-0.794008429134907));
#33053=CARTESIAN_POINT('Ctrl Pts',(-3.75224692493864,-1.,-0.794017347371377));
#33054=CARTESIAN_POINT('Ctrl Pts',(-3.74511357728861,-1.,-0.793982700459952));
#33055=CARTESIAN_POINT('Ctrl Pts',(-3.73803280541687,-1.,-0.793882700937017));
#33056=CARTESIAN_POINT('Ctrl Pts',(-3.73086914695805,-1.,-0.793682750269684));
#33057=CARTESIAN_POINT('Ctrl Pts',(-3.72348797293734,-1.,-0.793347023784205));
#33058=CARTESIAN_POINT('Ctrl Pts',(-3.71580242396124,-1.,-0.792848377370287));
#33059=CARTESIAN_POINT('Ctrl Pts',(-3.70781724021806,-1.,-0.792177688845818));
#33060=CARTESIAN_POINT('Ctrl Pts',(-3.69968940808721,-1.,-0.79135657569598));
#33061=CARTESIAN_POINT('Ctrl Pts',(-3.69172044327364,-1.,-0.790436284988787));
#33062=CARTESIAN_POINT('Ctrl Pts',(-3.68428439783905,-1.,-0.789483546064387));
#33063=CARTESIAN_POINT('Ctrl Pts',(-3.67777119516252,-1.,-0.788569566220285));
#33064=CARTESIAN_POINT('Ctrl Pts',(-3.67252923663655,-1.,-0.787758799995742));
#33065=CARTESIAN_POINT('Ctrl Pts',(-3.66907505398677,-1.,-0.787145041181545));
#33066=CARTESIAN_POINT('Ctrl Pts',(-3.66743103898702,-1.,-0.786774337198062));
#33067=CARTESIAN_POINT('Ctrl Pts',(-3.66680946938292,-1.,-0.786565919558984));
#33068=CARTESIAN_POINT('Ctrl Pts',(-3.6666431041522,-1.,-0.786459983895432));
#33069=CARTESIAN_POINT('Ctrl Pts',(-3.66661143271685,-1.,-0.786422660831985));
#33070=CARTESIAN_POINT('',(-3.62400312501245,-1.,-0.963899035117249));
#33071=CARTESIAN_POINT('Origin',(0.,-1.,0.));
#33072=CARTESIAN_POINT('',(-4.01728681790024,-1.,-1.22531898815164));
#33073=CARTESIAN_POINT('Ctrl Pts',(-3.62400312501245,-1.,-0.963899035117249));
#33074=CARTESIAN_POINT('Ctrl Pts',(-3.6240482887845,-1.,-0.963880158555582));
#33075=CARTESIAN_POINT('Ctrl Pts',(-3.62424461507588,-1.,-0.963861297423241));
#33076=CARTESIAN_POINT('Ctrl Pts',(-3.62489305727662,-1.,-0.963957782642843));
#33077=CARTESIAN_POINT('Ctrl Pts',(-3.62652618145335,-1.,-0.964373850166457));
#33078=CARTESIAN_POINT('Ctrl Pts',(-3.62988252139846,-1.,-0.965395153165293));
#33079=CARTESIAN_POINT('Ctrl Pts',(-3.63492122081143,-1.,-0.967052554541385));
#33080=CARTESIAN_POINT('Ctrl Pts',(-3.64113946505766,-1.,-0.969195124675865));
#33081=CARTESIAN_POINT('Ctrl Pts',(-3.64819756447455,-1.,-0.971722122061341));
#33082=CARTESIAN_POINT('Ctrl Pts',(-3.65571576735126,-1.,-0.974519971354848));
#33083=CARTESIAN_POINT('Ctrl Pts',(-3.66333049637475,-1.,-0.977478312751618));
#33084=CARTESIAN_POINT('Ctrl Pts',(-3.67074983340361,-1.,-0.980505922458267));
#33085=CARTESIAN_POINT('Ctrl Pts',(-3.67782408841715,-1.,-0.983550791470419));
#33086=CARTESIAN_POINT('Ctrl Pts',(-3.68455317926068,-1.,-0.986602639863837));
#33087=CARTESIAN_POINT('Ctrl Pts',(-3.69102682138846,-1.,-0.989676715398558));
#33088=CARTESIAN_POINT('Ctrl Pts',(-3.69738123415662,-1.,-0.99280221833201));
#33089=CARTESIAN_POINT('Ctrl Pts',(-3.70375282282138,-1.,-0.996009819772518));
#33090=CARTESIAN_POINT('Ctrl Pts',(-3.71022439713938,-1.,-0.99931726075653));
#33091=CARTESIAN_POINT('Ctrl Pts',(-3.71680667125118,-1.,-1.00272423396822));
#33092=CARTESIAN_POINT('Ctrl Pts',(-3.72346803750595,-1.,-1.0062200073571));
#33093=CARTESIAN_POINT('Ctrl Pts',(-3.73015276704426,-1.,-1.00978798539496));
#33094=CARTESIAN_POINT('Ctrl Pts',(-3.73680245055734,-1.,-1.01341114319903));
#33095=CARTESIAN_POINT('Ctrl Pts',(-3.74337942504959,-1.,-1.01707794311079));
#33096=CARTESIAN_POINT('Ctrl Pts',(-3.74987777155834,-1.,-1.02078510487428));
#33097=CARTESIAN_POINT('Ctrl Pts',(-3.75631037456194,-1.,-1.0245342944466));
#33098=CARTESIAN_POINT('Ctrl Pts',(-3.76270122291232,-1.,-1.02833014458181));
#33099=CARTESIAN_POINT('Ctrl Pts',(-3.76907609832522,-1.,-1.0321778660492));
#33100=CARTESIAN_POINT('Ctrl Pts',(-3.77545283140445,-1.,-1.03608074678013));
#33101=CARTESIAN_POINT('Ctrl Pts',(-3.78183535008192,-1.,-1.04003862055804));
#33102=CARTESIAN_POINT('Ctrl Pts',(-3.78821910787195,-1.,-1.04404924374426));
#33103=CARTESIAN_POINT('Ctrl Pts',(-3.79459440308793,-1.,-1.04810913267641));
#33104=CARTESIAN_POINT('Ctrl Pts',(-3.80095039790678,-1.,-1.05221457990015));
#33105=CARTESIAN_POINT('Ctrl Pts',(-3.80727913637784,-1.,-1.05636266918643));
#33106=CARTESIAN_POINT('Ctrl Pts',(-3.81357866117485,-1.,-1.06055206187298));
#33107=CARTESIAN_POINT('Ctrl Pts',(-3.81985083953012,-1.,-1.06478244038931));
#33108=CARTESIAN_POINT('Ctrl Pts',(-3.82609989967278,-1.,-1.0690541318036));
#33109=CARTESIAN_POINT('Ctrl Pts',(-3.83233071195145,-1.,-1.0733676663346));
#33110=CARTESIAN_POINT('Ctrl Pts',(-3.83854714117486,-1.,-1.07772335353856));
#33111=CARTESIAN_POINT('Ctrl Pts',(-3.84475048030615,-1.,-1.08212087917986));
#33112=CARTESIAN_POINT('Ctrl Pts',(-3.8509402522269,-1.,-1.08655950846377));
#33113=CARTESIAN_POINT('Ctrl Pts',(-3.85711487933911,-1.,-1.09103825516288));
#33114=CARTESIAN_POINT('Ctrl Pts',(-3.86327241021242,-1.,-1.09555606505012));
#33115=CARTESIAN_POINT('Ctrl Pts',(-3.86941120134872,-1.,-1.10011198761202));
#33116=CARTESIAN_POINT('Ctrl Pts',(-3.87553067187566,-1.,-1.10470536603303));
#33117=CARTESIAN_POINT('Ctrl Pts',(-3.88163105531791,-1.,-1.10933577224029));
#33118=CARTESIAN_POINT('Ctrl Pts',(-3.88771308285229,-1.,-1.11400292434447));
#33119=CARTESIAN_POINT('Ctrl Pts',(-3.89377768340362,-1.,-1.11870660794609));
#33120=CARTESIAN_POINT('Ctrl Pts',(-3.89982569749978,-1.,-1.12344660099029));
#33121=CARTESIAN_POINT('Ctrl Pts',(-3.90585753318622,-1.,-1.12822258281518));
#33122=CARTESIAN_POINT('Ctrl Pts',(-3.91187321145495,-1.,-1.13303414693849));
#33123=CARTESIAN_POINT('Ctrl Pts',(-3.91787251936688,-1.,-1.13788084225511));
#33124=CARTESIAN_POINT('Ctrl Pts',(-3.92385513133937,-1.,-1.14276220561575));
#33125=CARTESIAN_POINT('Ctrl Pts',(-3.92982073294334,-1.,-1.14767779451147));
#33126=CARTESIAN_POINT('Ctrl Pts',(-3.9357691705651,-1.,-1.1526272271639));
#33127=CARTESIAN_POINT('Ctrl Pts',(-3.94170046685542,-1.,-1.1576101834106));
#33128=CARTESIAN_POINT('Ctrl Pts',(-3.9476147478092,-1.,-1.16262637999261));
#33129=CARTESIAN_POINT('Ctrl Pts',(-3.95351219510062,-1.,-1.16767555244495));
#33130=CARTESIAN_POINT('Ctrl Pts',(-3.95939299213164,-1.,-1.17275743590327));
#33131=CARTESIAN_POINT('Ctrl Pts',(-3.96525726357682,-1.,-1.17787174135445));
#33132=CARTESIAN_POINT('Ctrl Pts',(-3.9711050516465,-1.,-1.18301815039596));
#33133=CARTESIAN_POINT('Ctrl Pts',(-3.97693634766926,-1.,-1.18819633715285));
#33134=CARTESIAN_POINT('Ctrl Pts',(-3.98275111052015,-1.,-1.19340598349307));
#33135=CARTESIAN_POINT('Ctrl Pts',(-3.98854928957287,-1.,-1.19864679609596));
#33136=CARTESIAN_POINT('Ctrl Pts',(-3.99433084800649,-1.,-1.2039185237544));
#33137=CARTESIAN_POINT('Ctrl Pts',(-4.00009577952534,-1.,-1.20922097030107));
#33138=CARTESIAN_POINT('Ctrl Pts',(-4.00584409524937,-1.,-1.21455398918813));
#33139=CARTESIAN_POINT('Ctrl Pts',(-4.01042947142681,-1.,-1.21884478244983));
#33140=CARTESIAN_POINT('Ctrl Pts',(-4.01386104434674,-1.,-1.22207656456199));
#33141=CARTESIAN_POINT('Ctrl Pts',(-4.0161454457032,-1.,-1.22423716681447));
#33142=CARTESIAN_POINT('Ctrl Pts',(-4.01728681790024,-1.,-1.22531898815164));
#33143=CARTESIAN_POINT('',(-3.97027773754922,-1.,-1.36999806084572));
#33144=CARTESIAN_POINT('',(-4.01728681790024,-1.,-1.22531898815164));
#33145=CARTESIAN_POINT('',(-3.4984457533445,-1.,-1.35032489087101));
#33146=CARTESIAN_POINT('Ctrl Pts',(-3.97027773754922,-1.,-1.36999806084572));
#33147=CARTESIAN_POINT('Ctrl Pts',(-3.9687184694131,-1.,-1.37020239094614));
#33148=CARTESIAN_POINT('Ctrl Pts',(-3.96560037974645,-1.,-1.37060761745635));
#33149=CARTESIAN_POINT('Ctrl Pts',(-3.96092458506535,-1.,-1.3712051561502));
#33150=CARTESIAN_POINT('Ctrl Pts',(-3.95469287280914,-1.,-1.37198126432386));
#33151=CARTESIAN_POINT('Ctrl Pts',(-3.94690771785133,-1.,-1.37291699202807));
#33152=CARTESIAN_POINT('Ctrl Pts',(-3.93912709040818,-1.,-1.37381821967165));
#33153=CARTESIAN_POINT('Ctrl Pts',(-3.93135106761844,-1.,-1.37468482215751));
#33154=CARTESIAN_POINT('Ctrl Pts',(-3.92357976987672,-1.,-1.37551664448242));
#33155=CARTESIAN_POINT('Ctrl Pts',(-3.91581337462644,-1.,-1.37631350505797));
#33156=CARTESIAN_POINT('Ctrl Pts',(-3.90805209523486,-1.,-1.3770751963402));
#33157=CARTESIAN_POINT('Ctrl Pts',(-3.90029615196727,-1.,-1.37780148512792));
#33158=CARTESIAN_POINT('Ctrl Pts',(-3.89254574338496,-1.,-1.3784921128802));
#33159=CARTESIAN_POINT('Ctrl Pts',(-3.88480102249277,-1.,-1.37914679719383));
#33160=CARTESIAN_POINT('Ctrl Pts',(-3.87706205830532,-1.,-1.37976523097073));
#33161=CARTESIAN_POINT('Ctrl Pts',(-3.86932885813068,-1.,-1.38034709213014));
#33162=CARTESIAN_POINT('Ctrl Pts',(-3.86160143043959,-1.,-1.38089205992989));
#33163=CARTESIAN_POINT('Ctrl Pts',(-3.85387983979481,-1.,-1.38139983115049));
#33164=CARTESIAN_POINT('Ctrl Pts',(-3.84616425605764,-1.,-1.38187013346109));
#33165=CARTESIAN_POINT('Ctrl Pts',(-3.83845502790746,-1.,-1.38230274828821));
#33166=CARTESIAN_POINT('Ctrl Pts',(-3.8307526698229,-1.,-1.38269750245138));
#33167=CARTESIAN_POINT('Ctrl Pts',(-3.82305771743829,-1.,-1.38305421262763));
#33168=CARTESIAN_POINT('Ctrl Pts',(-3.81537060817811,-1.,-1.38337263902782));
#33169=CARTESIAN_POINT('Ctrl Pts',(-3.80769156398411,-1.,-1.3836524404622));
#33170=CARTESIAN_POINT('Ctrl Pts',(-3.80002044322111,-1.,-1.38389311766682));
#33171=CARTESIAN_POINT('Ctrl Pts',(-3.79235669640841,-1.,-1.38409399694566));
#33172=CARTESIAN_POINT('Ctrl Pts',(-3.78469969805082,-1.,-1.38425435883756));
#33173=CARTESIAN_POINT('Ctrl Pts',(-3.77704902230418,-1.,-1.38437354551428));
#33174=CARTESIAN_POINT('Ctrl Pts',(-3.76940473185779,-1.,-1.38445107339518));
#33175=CARTESIAN_POINT('Ctrl Pts',(-3.76176768271367,-1.,-1.3844867525335));
#33176=CARTESIAN_POINT('Ctrl Pts',(-3.7541397631875,-1.,-1.38448077997163));
#33177=CARTESIAN_POINT('Ctrl Pts',(-3.74652317167876,-1.,-1.38443344984394));
#33178=CARTESIAN_POINT('Ctrl Pts',(-3.73891976418104,-1.,-1.38434489156458));
#33179=CARTESIAN_POINT('Ctrl Pts',(-3.73133035859282,-1.,-1.38421479111531));
#33180=CARTESIAN_POINT('Ctrl Pts',(-3.72375409358803,-1.,-1.3840421342895));
#33181=CARTESIAN_POINT('Ctrl Pts',(-3.7161876605181,-1.,-1.38382489984586));
#33182=CARTESIAN_POINT('Ctrl Pts',(-3.70862680753347,-1.,-1.38356065402124));
#33183=CARTESIAN_POINT('Ctrl Pts',(-3.701067921679,-1.,-1.38324717612865));
#33184=CARTESIAN_POINT('Ctrl Pts',(-3.69350967899526,-1.,-1.3828831117165));
#33185=CARTESIAN_POINT('Ctrl Pts',(-3.68595444983837,-1.,-1.38246852827182));
#33186=CARTESIAN_POINT('Ctrl Pts',(-3.67841038482414,-1.,-1.3820057429062));
#33187=CARTESIAN_POINT('Ctrl Pts',(-3.67088843112262,-1.,-1.38149812653868));
#33188=CARTESIAN_POINT('Ctrl Pts',(-3.66339848520857,-1.,-1.38094856333552));
#33189=CARTESIAN_POINT('Ctrl Pts',(-3.6559455440439,-1.,-1.38035791051212));
#33190=CARTESIAN_POINT('Ctrl Pts',(-3.64852652756456,-1.,-1.37972372481603));
#33191=CARTESIAN_POINT('Ctrl Pts',(-3.64112507791141,-1.,-1.37903818567359));
#33192=CARTESIAN_POINT('Ctrl Pts',(-3.63371727442486,-1.,-1.37829035457339));
#33193=CARTESIAN_POINT('Ctrl Pts',(-3.62628098665145,-1.,-1.37746987919881));
#33194=CARTESIAN_POINT('Ctrl Pts',(-3.6188048116042,-1.,-1.37657053403107));
#33195=CARTESIAN_POINT('Ctrl Pts',(-3.61129546591064,-1.,-1.37559314436634));
#33196=CARTESIAN_POINT('Ctrl Pts',(-3.60379020123988,-1.,-1.37455051379623));
#33197=CARTESIAN_POINT('Ctrl Pts',(-3.59634627869048,-1.,-1.37346320103157));
#33198=CARTESIAN_POINT('Ctrl Pts',(-3.58901853846365,-1.,-1.37235053660976));
#33199=CARTESIAN_POINT('Ctrl Pts',(-3.58183885982715,-1.,-1.37122241663062));
#33200=CARTESIAN_POINT('Ctrl Pts',(-3.57479875549486,-1.,-1.37007229485659));
#33201=CARTESIAN_POINT('Ctrl Pts',(-3.5678208030466,-1.,-1.36886584973389));
#33202=CARTESIAN_POINT('Ctrl Pts',(-3.56077662028649,-1.,-1.36754771771233));
#33203=CARTESIAN_POINT('Ctrl Pts',(-3.55353883995949,-1.,-1.3660614545677));
#33204=CARTESIAN_POINT('Ctrl Pts',(-3.54602591832973,-1.,-1.36436666257597));
#33205=CARTESIAN_POINT('Ctrl Pts',(-3.53824396424961,-1.,-1.36245507339307));
#33206=CARTESIAN_POINT('Ctrl Pts',(-3.530344649616,-1.,-1.36037259643734));
#33207=CARTESIAN_POINT('Ctrl Pts',(-3.52261776116748,-1.,-1.35821701528836));
#33208=CARTESIAN_POINT('Ctrl Pts',(-3.51542230699556,-1.,-1.35611275237152));
#33209=CARTESIAN_POINT('Ctrl Pts',(-3.50913227059999,-1.,-1.35419113575956));
#33210=CARTESIAN_POINT('Ctrl Pts',(-3.50408168106261,-1.,-1.35257032843486));
#33211=CARTESIAN_POINT('Ctrl Pts',(-3.5007660381649,-1.,-1.35142377279517));
#33212=CARTESIAN_POINT('Ctrl Pts',(-3.49920025459723,-1.,-1.35080045218587));
#33213=CARTESIAN_POINT('Ctrl Pts',(-3.49861894124827,-1.,-1.35049736560527));
#33214=CARTESIAN_POINT('Ctrl Pts',(-3.49847119623846,-1.,-1.35036670892966));
#33215=CARTESIAN_POINT('Ctrl Pts',(-3.4984457533445,-1.,-1.35032489087101));
#33216=CARTESIAN_POINT('',(-3.42859860294378,-1.,-1.51895082866166));
#33217=CARTESIAN_POINT('Origin',(0.,-1.,0.));
#33218=CARTESIAN_POINT('',(-3.77614523045147,-1.,-1.83867539237861));
#33219=CARTESIAN_POINT('Ctrl Pts',(-3.42859860294378,-1.,-1.51895082866166));
#33220=CARTESIAN_POINT('Ctrl Pts',(-3.42864616361967,-1.,-1.51893924967231));
#33221=CARTESIAN_POINT('Ctrl Pts',(-3.42884302333978,-1.,-1.51895133295017));
#33222=CARTESIAN_POINT('Ctrl Pts',(-3.42946838852728,-1.,-1.51914806898539));
#33223=CARTESIAN_POINT('Ctrl Pts',(-3.43101631893491,-1.,-1.5198144909343));
#33224=CARTESIAN_POINT('Ctrl Pts',(-3.43417156977749,-1.,-1.52134826724227));
#33225=CARTESIAN_POINT('Ctrl Pts',(-3.43888895974182,-1.,-1.52377348950429));
#33226=CARTESIAN_POINT('Ctrl Pts',(-3.44469547527,-1.,-1.52686242875717));
#33227=CARTESIAN_POINT('Ctrl Pts',(-3.45127136828667,-1.,-1.530462444618));
#33228=CARTESIAN_POINT('Ctrl Pts',(-3.45825932955273,-1.,-1.53440195378902));
#33229=CARTESIAN_POINT('Ctrl Pts',(-3.46531752207222,-1.,-1.53851507915533));
#33230=CARTESIAN_POINT('Ctrl Pts',(-3.47217189224576,-1.,-1.54266605398152));
#33231=CARTESIAN_POINT('Ctrl Pts',(-3.47868272898599,-1.,-1.54678009290206));
#33232=CARTESIAN_POINT('Ctrl Pts',(-3.48485155928414,-1.,-1.55084702970382));
#33233=CARTESIAN_POINT('Ctrl Pts',(-3.49076460877317,-1.,-1.5548959590107));
#33234=CARTESIAN_POINT('Ctrl Pts',(-3.49655185179623,-1.,-1.55897703097859));
#33235=CARTESIAN_POINT('Ctrl Pts',(-3.50234321621607,-1.,-1.56314187758689));
#33236=CARTESIAN_POINT('Ctrl Pts',(-3.50821771695427,-1.,-1.56742097575041));
#33237=CARTESIAN_POINT('Ctrl Pts',(-3.51418598431733,-1.,-1.57181569799774));
#33238=CARTESIAN_POINT('Ctrl Pts',(-3.52021847865961,-1.,-1.5763104998818));
#33239=CARTESIAN_POINT('Ctrl Pts',(-3.52626275334899,-1.,-1.58088027227856));
#33240=CARTESIAN_POINT('Ctrl Pts',(-3.53226378147068,-1.,-1.58549906268083));
#33241=CARTESIAN_POINT('Ctrl Pts',(-3.53818616861045,-1.,-1.59014958368725));
#33242=CARTESIAN_POINT('Ctrl Pts',(-3.544024581823,-1.,-1.5948276694975));
#33243=CARTESIAN_POINT('Ctrl Pts',(-3.54979148634426,-1.,-1.59953698113444));
#33244=CARTESIAN_POINT('Ctrl Pts',(-3.55550985096117,-1.,-1.60428584699848));
#33245=CARTESIAN_POINT('Ctrl Pts',(-3.56120432482986,-1.,-1.60908344685459));
#33246=CARTESIAN_POINT('Ctrl Pts',(-3.56689200468404,-1.,-1.61393581747522));
#33247=CARTESIAN_POINT('Ctrl Pts',(-3.57257679609826,-1.,-1.61884340915412));
#33248=CARTESIAN_POINT('Ctrl Pts',(-3.57825455954405,-1.,-1.62380329464851));
#33249=CARTESIAN_POINT('Ctrl Pts',(-3.5839162577435,-1.,-1.62881051550748));
#33250=CARTESIAN_POINT('Ctrl Pts',(-3.58955176627876,-1.,-1.63385971451259));
#33251=CARTESIAN_POINT('Ctrl Pts',(-3.59515368334887,-1.,-1.63894676675349));
#33252=CARTESIAN_POINT('Ctrl Pts',(-3.6007202851384,-1.,-1.6440700438558));
#33253=CARTESIAN_POINT('Ctrl Pts',(-3.60625346556992,-1.,-1.64922952425833));
#33254=CARTESIAN_POINT('Ctrl Pts',(-3.61175734965129,-1.,-1.65442619244327));
#33255=CARTESIAN_POINT('Ctrl Pts',(-3.61723666482457,-1.,-1.65966133399186));
#33256=CARTESIAN_POINT('Ctrl Pts',(-3.62269517989104,-1.,-1.66493585923853));
#33257=CARTESIAN_POINT('Ctrl Pts',(-3.62813422105257,-1.,-1.67024966008037));
#33258=CARTESIAN_POINT('Ctrl Pts',(-3.63355343201211,-1.,-1.67560193613145));
#33259=CARTESIAN_POINT('Ctrl Pts',(-3.63895140887443,-1.,-1.68099146651577));
#33260=CARTESIAN_POINT('Ctrl Pts',(-3.64432638915199,-1.,-1.68641690471455));
#33261=CARTESIAN_POINT('Ctrl Pts',(-3.64967689827393,-1.,-1.691877054817));
#33262=CARTESIAN_POINT('Ctrl Pts',(-3.65500246526798,-1.,-1.69737117722558));
#33263=CARTESIAN_POINT('Ctrl Pts',(-3.6603033877491,-1.,-1.70289888566904));
#33264=CARTESIAN_POINT('Ctrl Pts',(-3.6655804319893,-1.,-1.70846001610983));
#33265=CARTESIAN_POINT('Ctrl Pts',(-3.67083454901629,-1.,-1.71405450210392));
#33266=CARTESIAN_POINT('Ctrl Pts',(-3.67606660374665,-1.,-1.71968225581787));
#33267=CARTESIAN_POINT('Ctrl Pts',(-3.68127704936472,-1.,-1.72534302437003));
#33268=CARTESIAN_POINT('Ctrl Pts',(-3.68646597019188,-1.,-1.73103640956647));
#33269=CARTESIAN_POINT('Ctrl Pts',(-3.69163322647906,-1.,-1.73676193254493));
#33270=CARTESIAN_POINT('Ctrl Pts',(-3.6967785691046,-1.,-1.74251908492589));
#33271=CARTESIAN_POINT('Ctrl Pts',(-3.70190175673422,-1.,-1.74830738046092));
#33272=CARTESIAN_POINT('Ctrl Pts',(-3.70700269736876,-1.,-1.75412641804148));
#33273=CARTESIAN_POINT('Ctrl Pts',(-3.71208146346454,-1.,-1.75997588499021));
#33274=CARTESIAN_POINT('Ctrl Pts',(-3.71713822377675,-1.,-1.76585552124549));
#33275=CARTESIAN_POINT('Ctrl Pts',(-3.72217319911429,-1.,-1.77176509401846));
#33276=CARTESIAN_POINT('Ctrl Pts',(-3.72718661205504,-1.,-1.77770437039606));
#33277=CARTESIAN_POINT('Ctrl Pts',(-3.73217863095022,-1.,-1.78367308442682));
#33278=CARTESIAN_POINT('Ctrl Pts',(-3.73714934729962,-1.,-1.78967092823139));
#33279=CARTESIAN_POINT('Ctrl Pts',(-3.74209880351667,-1.,-1.79569757859041));
#33280=CARTESIAN_POINT('Ctrl Pts',(-3.74702700874954,-1.,-1.80175271485519));
#33281=CARTESIAN_POINT('Ctrl Pts',(-3.75193395888069,-1.,-1.80783603939662));
#33282=CARTESIAN_POINT('Ctrl Pts',(-3.75681965683995,-1.,-1.81394729834032));
#33283=CARTESIAN_POINT('Ctrl Pts',(-3.76168412709652,-1.,-1.82008629694924));
#33284=CARTESIAN_POINT('Ctrl Pts',(-3.76652740355856,-1.,-1.82625289221933));
#33285=CARTESIAN_POINT('Ctrl Pts',(-3.77038509819777,-1.,-1.83120816956515));
#33286=CARTESIAN_POINT('Ctrl Pts',(-3.77326886065484,-1.,-1.83493697935064));
#33287=CARTESIAN_POINT('Ctrl Pts',(-3.77518714458232,-1.,-1.83742834010821));
#33288=CARTESIAN_POINT('Ctrl Pts',(-3.77614523045147,-1.,-1.83867539237861));
#33289=CARTESIAN_POINT('',(-3.70708211654725,-1.,-1.97421938526992));
#33290=CARTESIAN_POINT('',(-3.77614523045147,-1.,-1.83867539237861));
#33291=CARTESIAN_POINT('',(-3.24413672884902,-1.,-1.88097764062542));
#33292=CARTESIAN_POINT('Ctrl Pts',(-3.70708211654725,-1.,-1.97421938526992));
#33293=CARTESIAN_POINT('Ctrl Pts',(-3.7055100813194,-1.,-1.974177276451));
#33294=CARTESIAN_POINT('Ctrl Pts',(-3.70236698911837,-1.,-1.97408973726149));
#33295=CARTESIAN_POINT('Ctrl Pts',(-3.69765528558292,-1.,-1.97394846382288));
#33296=CARTESIAN_POINT('Ctrl Pts',(-3.69137888597855,-1.,-1.97374016224397));
#33297=CARTESIAN_POINT('Ctrl Pts',(-3.68354319913416,-1.,-1.9734465030363));
#33298=CARTESIAN_POINT('Ctrl Pts',(-3.67571738106175,-1.,-1.97311947678035));
#33299=CARTESIAN_POINT('Ctrl Pts',(-3.66790152751984,-1.,-1.9727589719863));
#33300=CARTESIAN_POINT('Ctrl Pts',(-3.66009578166865,-1.,-1.97236485439317));
#33301=CARTESIAN_POINT('Ctrl Pts',(-3.65230034717364,-1.,-1.97193697240645));
#33302=CARTESIAN_POINT('Ctrl Pts',(-3.64451546724221,-1.,-1.97147515441539));
#33303=CARTESIAN_POINT('Ctrl Pts',(-3.63674139590853,-1.,-1.97097920454698));
#33304=CARTESIAN_POINT('Ctrl Pts',(-3.62897836973397,-1.,-1.97044889850518));
#33305=CARTESIAN_POINT('Ctrl Pts',(-3.62122658401722,-1.,-1.96988398129888));
#33306=CARTESIAN_POINT('Ctrl Pts',(-3.61348615496393,-1.,-1.96928416040712));
#33307=CARTESIAN_POINT('Ctrl Pts',(-3.60575714017676,-1.,-1.96864911885775));
#33308=CARTESIAN_POINT('Ctrl Pts',(-3.59803959819725,-1.,-1.96797854118257));
#33309=CARTESIAN_POINT('Ctrl Pts',(-3.5903336402273,-1.,-1.96727213799507));
#33310=CARTESIAN_POINT('Ctrl Pts',(-3.58263947663884,-1.,-1.9665296668894));
#33311=CARTESIAN_POINT('Ctrl Pts',(-3.57495748601088,-1.,-1.96575096652857));
#33312=CARTESIAN_POINT('Ctrl Pts',(-3.56728820357933,-1.,-1.96493594634643));
#33313=CARTESIAN_POINT('Ctrl Pts',(-3.55963218706201,-1.,-1.96408450906868));
#33314=CARTESIAN_POINT('Ctrl Pts',(-3.55198990600929,-1.,-1.96319648628667));
#33315=CARTESIAN_POINT('Ctrl Pts',(-3.54436163300425,-1.,-1.96227157573058));
#33316=CARTESIAN_POINT('Ctrl Pts',(-3.53674730625759,-1.,-1.96130926212661));
#33317=CARTESIAN_POINT('Ctrl Pts',(-3.52914648844289,-1.,-1.96030879411534));
#33318=CARTESIAN_POINT('Ctrl Pts',(-3.52155867431438,-1.,-1.95926936324436));
#33319=CARTESIAN_POINT('Ctrl Pts',(-3.51398354617772,-1.,-1.95819025316768));
#33320=CARTESIAN_POINT('Ctrl Pts',(-3.50642124159913,-1.,-1.95707099606513));
#33321=CARTESIAN_POINT('Ctrl Pts',(-3.49887263575602,-1.,-1.9559115382367));
#33322=CARTESIAN_POINT('Ctrl Pts',(-3.49133956289154,-1.,-1.95471236969653));
#33323=CARTESIAN_POINT('Ctrl Pts',(-3.48382414832648,-1.,-1.95347412486316));
#33324=CARTESIAN_POINT('Ctrl Pts',(-3.47632820495926,-1.,-1.95219722189878));
#33325=CARTESIAN_POINT('Ctrl Pts',(-3.4688525897419,-1.,-1.95088147859876));
#33326=CARTESIAN_POINT('Ctrl Pts',(-3.46139661060959,-1.,-1.94952575850196));
#33327=CARTESIAN_POINT('Ctrl Pts',(-3.45395731584051,-1.,-1.94812754766524));
#33328=CARTESIAN_POINT('Ctrl Pts',(-3.44653088665685,-1.,-1.94668377715332));
#33329=CARTESIAN_POINT('Ctrl Pts',(-3.43911410197693,-1.,-1.94519168842883));
#33330=CARTESIAN_POINT('Ctrl Pts',(-3.43170586602436,-1.,-1.94364973660285));
#33331=CARTESIAN_POINT('Ctrl Pts',(-3.42430850941497,-1.,-1.94205835913692));
#33332=CARTESIAN_POINT('Ctrl Pts',(-3.41692971994082,-1.,-1.94042111965237));
#33333=CARTESIAN_POINT('Ctrl Pts',(-3.40957978266622,-1.,-1.93874306008132));
#33334=CARTESIAN_POINT('Ctrl Pts',(-3.40226802104093,-1.,-1.93702857723089));
#33335=CARTESIAN_POINT('Ctrl Pts',(-3.39499923640789,-1.,-1.93527929945982));
#33336=CARTESIAN_POINT('Ctrl Pts',(-3.38777076883267,-1.,-1.93349233176794));
#33337=CARTESIAN_POINT('Ctrl Pts',(-3.38056768525577,-1.,-1.93165739093292));
#33338=CARTESIAN_POINT('Ctrl Pts',(-3.37336807068078,-1.,-1.92975993109897));
#33339=CARTESIAN_POINT('Ctrl Pts',(-3.36615168657597,-1.,-1.92778626543803));
#33340=CARTESIAN_POINT('Ctrl Pts',(-3.35890824422976,-1.,-1.92572846125763));
#33341=CARTESIAN_POINT('Ctrl Pts',(-3.35164424847206,-1.,-1.92358838440518));
#33342=CARTESIAN_POINT('Ctrl Pts',(-3.34439448941915,-1.,-1.92138450828378));
#33343=CARTESIAN_POINT('Ctrl Pts',(-3.33721230709948,-1.,-1.91914609610173));
#33344=CARTESIAN_POINT('Ctrl Pts',(-3.33014884257812,-1.,-1.91690081930297));
#33345=CARTESIAN_POINT('Ctrl Pts',(-3.32323403454507,-1.,-1.91466343916612));
#33346=CARTESIAN_POINT('Ctrl Pts',(-3.31646052426395,-1.,-1.91242616234459));
#33347=CARTESIAN_POINT('Ctrl Pts',(-3.30975721158694,-1.,-1.91014297830502));
#33348=CARTESIAN_POINT('Ctrl Pts',(-3.30300595568341,-1.,-1.90773912171424));
#33349=CARTESIAN_POINT('Ctrl Pts',(-3.29608978722258,-1.,-1.9051389186417));
#33350=CARTESIAN_POINT('Ctrl Pts',(-3.28893448600364,-1.,-1.9022897124757));
#33351=CARTESIAN_POINT('Ctrl Pts',(-3.28154737912287,-1.,-1.89918429230424));
#33352=CARTESIAN_POINT('Ctrl Pts',(-3.27407108932908,-1.,-1.89589172903662));
#33353=CARTESIAN_POINT('Ctrl Pts',(-3.2667765388833,-1.,-1.89255393500769));
#33354=CARTESIAN_POINT('Ctrl Pts',(-3.2599988519361,-1.,-1.88934996203508));
#33355=CARTESIAN_POINT('Ctrl Pts',(-3.25408686339298,-1.,-1.88646802523372));
#33356=CARTESIAN_POINT('Ctrl Pts',(-3.24935200512055,-1.,-1.88407708646435));
#33357=CARTESIAN_POINT('Ctrl Pts',(-3.24625654410705,-1.,-1.88242596600422));
#33358=CARTESIAN_POINT('Ctrl Pts',(-3.24480754675942,-1.,-1.88156537699118));
#33359=CARTESIAN_POINT('Ctrl Pts',(-3.24428080352952,-1.,-1.88117508446657));
#33360=CARTESIAN_POINT('Ctrl Pts',(-3.24415531671311,-1.,-1.88102292397987));
#33361=CARTESIAN_POINT('Ctrl Pts',(-3.24413672884902,-1.,-1.88097764062542));
#33362=CARTESIAN_POINT('',(-3.14877060440425,-1.,-2.03660101169564));
#33363=CARTESIAN_POINT('Origin',(0.,-1.,0.));
#33364=CARTESIAN_POINT('',(-3.44202241512147,-1.,-2.40675750623143));
#33365=CARTESIAN_POINT('Ctrl Pts',(-3.14877060440425,-1.,-2.03660101169564));
#33366=CARTESIAN_POINT('Ctrl Pts',(-3.1488193908823,-1.,-2.03659701539175));
#33367=CARTESIAN_POINT('Ctrl Pts',(-3.14901193669147,-1.,-2.03663974554941));
#33368=CARTESIAN_POINT('Ctrl Pts',(-3.14959882629936,-1.,-2.03693188810614));
#33369=CARTESIAN_POINT('Ctrl Pts',(-3.15102344775396,-1.,-2.03783225496023));
#33370=CARTESIAN_POINT('Ctrl Pts',(-3.1538999167466,-1.,-2.03984073791432));
#33371=CARTESIAN_POINT('Ctrl Pts',(-3.15817983946525,-1.,-2.04297406404132));
#33372=CARTESIAN_POINT('Ctrl Pts',(-3.16343165059235,-1.,-2.0469333124766));
#33373=CARTESIAN_POINT('Ctrl Pts',(-3.16936341689859,-1.,-2.05151770247452));
#33374=CARTESIAN_POINT('Ctrl Pts',(-3.17564906975592,-1.,-2.05650186773279));
#33375=CARTESIAN_POINT('Ctrl Pts',(-3.18197692964677,-1.,-2.06166849827143));
#33376=CARTESIAN_POINT('Ctrl Pts',(-3.18809755562297,-1.,-2.06684062744065));
#33377=CARTESIAN_POINT('Ctrl Pts',(-3.19388465568113,-1.,-2.07192253497765));
#33378=CARTESIAN_POINT('Ctrl Pts',(-3.19934132835879,-1.,-2.0769044187063));
#33379=CARTESIAN_POINT('Ctrl Pts',(-3.20454818630635,-1.,-2.08182850370816));
#33380=CARTESIAN_POINT('Ctrl Pts',(-3.20962575845433,-1.,-2.08676465517435));
#33381=CARTESIAN_POINT('Ctrl Pts',(-3.2146942960168,-1.,-2.0917841946046));
#33382=CARTESIAN_POINT('Ctrl Pts',(-3.21982707347067,-1.,-2.09692958434933));
#33383=CARTESIAN_POINT('Ctrl Pts',(-3.22503437553496,-1.,-2.10220384298533));
#33384=CARTESIAN_POINT('Ctrl Pts',(-3.23028945793334,-1.,-2.1075869964248));
#33385=CARTESIAN_POINT('Ctrl Pts',(-3.23554444767115,-1.,-2.11304604021784));
#33386=CARTESIAN_POINT('Ctrl Pts',(-3.24074905517282,-1.,-2.11854673326972));
#33387=CARTESIAN_POINT('Ctrl Pts',(-3.24587102613347,-1.,-2.12406646410943));
#33388=CARTESIAN_POINT('Ctrl Pts',(-3.25090574493994,-1.,-2.1296002839681));
#33389=CARTESIAN_POINT('Ctrl Pts',(-3.25586495065027,-1.,-2.13515375878786));
#33390=CARTESIAN_POINT('Ctrl Pts',(-3.26077002641868,-1.,-2.14073870754257));
#33391=CARTESIAN_POINT('Ctrl Pts',(-3.26564388189764,-1.,-2.14636805295663));
#33392=CARTESIAN_POINT('Ctrl Pts',(-3.27050245897244,-1.,-2.15205043199818));
#33393=CARTESIAN_POINT('Ctrl Pts',(-3.27534954469206,-1.,-2.15778690038359));
#33394=CARTESIAN_POINT('Ctrl Pts',(-3.28018150841414,-1.,-2.16357391934434));
#33395=CARTESIAN_POINT('Ctrl Pts',(-3.2849901997973,-1.,-2.16940517773459));
#33396=CARTESIAN_POINT('Ctrl Pts',(-3.28976645712566,-1.,-2.17527380048422));
#33397=CARTESIAN_POINT('Ctrl Pts',(-3.29450361500484,-1.,-2.18117455557062));
#33398=CARTESIAN_POINT('Ctrl Pts',(-3.29920022557635,-1.,-2.18710556500325));
#33399=CARTESIAN_POINT('Ctrl Pts',(-3.30385816281831,-1.,-2.19306710376112));
#33400=CARTESIAN_POINT('Ctrl Pts',(-3.30848134694596,-1.,-2.19906078949924));
#33401=CARTESIAN_POINT('Ctrl Pts',(-3.3130742460895,-1.,-2.20508863150608));
#33402=CARTESIAN_POINT('Ctrl Pts',(-3.31764044024231,-1.,-2.21115211847872));
#33403=CARTESIAN_POINT('Ctrl Pts',(-3.32218125618955,-1.,-2.21725135110889));
#33404=CARTESIAN_POINT('Ctrl Pts',(-3.32669646722871,-1.,-2.22338548312758));
#33405=CARTESIAN_POINT('Ctrl Pts',(-3.33118487773593,-1.,-2.22955308907221));
#33406=CARTESIAN_POINT('Ctrl Pts',(-3.33564495756478,-1.,-2.2357525632881));
#33407=CARTESIAN_POINT('Ctrl Pts',(-3.34007543738044,-1.,-2.24198249391437));
#33408=CARTESIAN_POINT('Ctrl Pts',(-3.34447596770768,-1.,-2.24824207678288));
#33409=CARTESIAN_POINT('Ctrl Pts',(-3.34884690292342,-1.,-2.25453097693524));
#33410=CARTESIAN_POINT('Ctrl Pts',(-3.35318902552676,-1.,-2.26084915222484));
#33411=CARTESIAN_POINT('Ctrl Pts',(-3.35750328523077,-1.,-2.26719668579921));
#33412=CARTESIAN_POINT('Ctrl Pts',(-3.36179055004369,-1.,-2.27357362620902));
#33413=CARTESIAN_POINT('Ctrl Pts',(-3.36605130712978,-1.,-2.27997979457968));
#33414=CARTESIAN_POINT('Ctrl Pts',(-3.37028570206357,-1.,-2.28641481081045));
#33415=CARTESIAN_POINT('Ctrl Pts',(-3.37449367172707,-1.,-2.2928781800731));
#33416=CARTESIAN_POINT('Ctrl Pts',(-3.37867504959382,-1.,-2.29936936127588));
#33417=CARTESIAN_POINT('Ctrl Pts',(-3.38282967336676,-1.,-2.30588783640389));
#33418=CARTESIAN_POINT('Ctrl Pts',(-3.38695751492659,-1.,-2.31243319489505));
#33419=CARTESIAN_POINT('Ctrl Pts',(-3.39105869475112,-1.,-2.31900513925627));
#33420=CARTESIAN_POINT('Ctrl Pts',(-3.39513342020045,-1.,-2.32560343902683));
#33421=CARTESIAN_POINT('Ctrl Pts',(-3.39918194578115,-1.,-2.33222789882601));
#33422=CARTESIAN_POINT('Ctrl Pts',(-3.40320452776646,-1.,-2.33887832342715));
#33423=CARTESIAN_POINT('Ctrl Pts',(-3.40720137403888,-1.,-2.34555447648901));
#33424=CARTESIAN_POINT('Ctrl Pts',(-3.41117262313464,-1.,-2.35225606823649));
#33425=CARTESIAN_POINT('Ctrl Pts',(-3.4151183675076,-1.,-2.35898278606449));
#33426=CARTESIAN_POINT('Ctrl Pts',(-3.41903866635384,-1.,-2.36573431470314));
#33427=CARTESIAN_POINT('Ctrl Pts',(-3.42293356216595,-1.,-2.37251035954351));
#33428=CARTESIAN_POINT('Ctrl Pts',(-3.42680309755241,-1.,-2.37931067029517));
#33429=CARTESIAN_POINT('Ctrl Pts',(-3.43064732714472,-1.,-2.38613505844641));
#33430=CARTESIAN_POINT('Ctrl Pts',(-3.43446630680436,-1.,-2.39298338805823));
#33431=CARTESIAN_POINT('Ctrl Pts',(-3.43750133066036,-1.,-2.39848113411429));
#33432=CARTESIAN_POINT('Ctrl Pts',(-3.43976627485223,-1.,-2.40261515590099));
#33433=CARTESIAN_POINT('Ctrl Pts',(-3.44127120683402,-1.,-2.40537592959345));
#33434=CARTESIAN_POINT('Ctrl Pts',(-3.44202241512147,-1.,-2.40675750623143));
#33435=CARTESIAN_POINT('',(-3.35260583073571,-1.,-2.52982887637028));
#33436=CARTESIAN_POINT('',(-3.44202241512147,-1.,-2.40675750623143));
#33437=CARTESIAN_POINT('',(-2.90994629141676,-1.,-2.36531447826073));
#33438=CARTESIAN_POINT('Ctrl Pts',(-3.35260583073571,-1.,-2.52982887637028));
#33439=CARTESIAN_POINT('Ctrl Pts',(-3.35105973714071,-1.,-2.5295413654909));
#33440=CARTESIAN_POINT('Ctrl Pts',(-3.34796903576663,-1.,-2.52896321610703));
#33441=CARTESIAN_POINT('Ctrl Pts',(-3.34333744115511,-1.,-2.52808660915689));
#33442=CARTESIAN_POINT('Ctrl Pts',(-3.33717089999103,-1.,-2.52689902690158));
#33443=CARTESIAN_POINT('Ctrl Pts',(-3.32947762187533,-1.,-2.52538321164634));
#33444=CARTESIAN_POINT('Ctrl Pts',(-3.32179931078699,-1.,-2.5238359839626));
#33445=CARTESIAN_POINT('Ctrl Pts',(-3.31413607874645,-1.,-2.52225724871313));
#33446=CARTESIAN_POINT('Ctrl Pts',(-3.30648808815442,-1.,-2.52064689568511));
#33447=CARTESIAN_POINT('Ctrl Pts',(-3.29885556388352,-1.,-2.51900480701069));
#33448=CARTESIAN_POINT('Ctrl Pts',(-3.2912387729927,-1.,-2.51733085123797));
#33449=CARTESIAN_POINT('Ctrl Pts',(-3.28363799702982,-1.,-2.51562487464514));
#33450=CARTESIAN_POINT('Ctrl Pts',(-3.27605350473142,-1.,-2.513886692704));
#33451=CARTESIAN_POINT('Ctrl Pts',(-3.26848552888115,-1.,-2.51211608411423));
#33452=CARTESIAN_POINT('Ctrl Pts',(-3.26093423001434,-1.,-2.51031277813486));
#33453=CARTESIAN_POINT('Ctrl Pts',(-3.25339971460982,-1.,-2.50847647070723));
#33454=CARTESIAN_POINT('Ctrl Pts',(-3.24588208983849,-1.,-2.506606859405));
#33455=CARTESIAN_POINT('Ctrl Pts',(-3.23838151080319,-1.,-2.5047036758003));
#33456=CARTESIAN_POINT('Ctrl Pts',(-3.23089822320646,-1.,-2.50276671338111));
#33457=CARTESIAN_POINT('Ctrl Pts',(-3.22343262620503,-1.,-2.50079587201957));
#33458=CARTESIAN_POINT('Ctrl Pts',(-3.21598526261286,-1.,-2.4987911459939));
#33459=CARTESIAN_POINT('Ctrl Pts',(-3.20855669849836,-1.,-2.4967525264737));
#33460=CARTESIAN_POINT('Ctrl Pts',(-3.20114742397588,-1.,-2.49467992057755));
#33461=CARTESIAN_POINT('Ctrl Pts',(-3.19375775555798,-1.,-2.49257307239848));
#33462=CARTESIAN_POINT('Ctrl Pts',(-3.18638771282266,-1.,-2.49043146334059));
#33463=CARTESIAN_POINT('Ctrl Pts',(-3.17903698136622,-1.,-2.48825428288201));
#33464=CARTESIAN_POINT('Ctrl Pts',(-3.17170518863313,-1.,-2.48604065348587));
#33465=CARTESIAN_POINT('Ctrl Pts',(-3.16439213290161,-1.,-2.48378981792725));
#33466=CARTESIAN_POINT('Ctrl Pts',(-3.15709802322739,-1.,-2.48150133566571));
#33467=CARTESIAN_POINT('Ctrl Pts',(-3.14982373241352,-1.,-2.47917529057029));
#33468=CARTESIAN_POINT('Ctrl Pts',(-3.1425709954655,-1.,-2.47681245356109));
#33469=CARTESIAN_POINT('Ctrl Pts',(-3.13534181229295,-1.,-2.47441378371932));
#33470=CARTESIAN_POINT('Ctrl Pts',(-3.12813790805952,-1.,-2.47197997765871));
#33471=CARTESIAN_POINT('Ctrl Pts',(-3.12096015766983,-1.,-2.46951098947469));
#33472=CARTESIAN_POINT('Ctrl Pts',(-3.11380805536122,-1.,-2.46700558843506));
#33473=CARTESIAN_POINT('Ctrl Pts',(-3.1066790790198,-1.,-2.46446082979646));
#33474=CARTESIAN_POINT('Ctrl Pts',(-3.09956993697052,-1.,-2.46187308501884));
#33475=CARTESIAN_POINT('Ctrl Pts',(-3.09247787931887,-1.,-2.4592391256388));
#33476=CARTESIAN_POINT('Ctrl Pts',(-3.08540206545315,-1.,-2.45655725437039));
#33477=CARTESIAN_POINT('Ctrl Pts',(-3.07834472886139,-1.,-2.4538282678779));
#33478=CARTESIAN_POINT('Ctrl Pts',(-3.07131290521297,-1.,-2.45105688854422));
#33479=CARTESIAN_POINT('Ctrl Pts',(-3.06431596421405,-1.,-2.44824970516544));
#33480=CARTESIAN_POINT('Ctrl Pts',(-3.05736242671506,-1.,-2.44541251892556));
#33481=CARTESIAN_POINT('Ctrl Pts',(-3.05045678021504,-1.,-2.44254768923105));
#33482=CARTESIAN_POINT('Ctrl Pts',(-3.04359685040555,-1.,-2.43965194061857));
#33483=CARTESIAN_POINT('Ctrl Pts',(-3.03676949672821,-1.,-2.43671278042414));
#33484=CARTESIAN_POINT('Ctrl Pts',(-3.02995534946978,-1.,-2.43371241361488));
#33485=CARTESIAN_POINT('Ctrl Pts',(-3.02313656036004,-1.,-2.43063415586637));
#33486=CARTESIAN_POINT('Ctrl Pts',(-3.01630420830504,-1.,-2.42746856264168));
#33487=CARTESIAN_POINT('Ctrl Pts',(-3.00946442616658,-1.,-2.42421849439613));
#33488=CARTESIAN_POINT('Ctrl Pts',(-3.00264868585996,-1.,-2.42090763946779));
#33489=CARTESIAN_POINT('Ctrl Pts',(-2.99590509293503,-1.,-2.41757324500514));
#33490=CARTESIAN_POINT('Ctrl Pts',(-2.98927983005796,-1.,-2.41425064199586));
#33491=CARTESIAN_POINT('Ctrl Pts',(-2.98280015815107,-1.,-2.41095909342571));
#33492=CARTESIAN_POINT('Ctrl Pts',(-2.97646002822422,-1.,-2.40768975073713));
#33493=CARTESIAN_POINT('Ctrl Pts',(-2.9701964131236,-1.,-2.40438604734919));
#33494=CARTESIAN_POINT('Ctrl Pts',(-2.96390432240312,-1.,-2.4009556571164));
#33495=CARTESIAN_POINT('Ctrl Pts',(-2.95748006482942,-1.,-2.39730553974517));
#33496=CARTESIAN_POINT('Ctrl Pts',(-2.95085857128439,-1.,-2.39337207631667));
#33497=CARTESIAN_POINT('Ctrl Pts',(-2.94404820669076,-1.,-2.38914929090759));
#33498=CARTESIAN_POINT('Ctrl Pts',(-2.93717903280391,-1.,-2.38472771516311));
#33499=CARTESIAN_POINT('Ctrl Pts',(-2.93049643640206,-1.,-2.38028989582073));
#33500=CARTESIAN_POINT('Ctrl Pts',(-2.92430340582608,-1.,-2.3760651052403));
#33501=CARTESIAN_POINT('Ctrl Pts',(-2.91891503791411,-1.,-2.37229381109821));
#33502=CARTESIAN_POINT('Ctrl Pts',(-2.9146124988314,-1.,-2.36919161373173));
#33503=CARTESIAN_POINT('Ctrl Pts',(-2.91181344022549,-1.,-2.36707658451664));
#33504=CARTESIAN_POINT('Ctrl Pts',(-2.91051690822156,-1.,-2.36599991765749));
#33505=CARTESIAN_POINT('Ctrl Pts',(-2.91005770527719,-1.,-2.36553202948613));
#33506=CARTESIAN_POINT('Ctrl Pts',(-2.90995756655606,-1.,-2.36536211188453));
#33507=CARTESIAN_POINT('Ctrl Pts',(-2.90994629141676,-1.,-2.36531447826074));
#33508=CARTESIAN_POINT('',(-2.79140942341378,-1.,-2.50410331873042));
#33509=CARTESIAN_POINT('Origin',(0.,-1.,0.));
#33510=CARTESIAN_POINT('',(-3.02314558451372,-1.,-2.91557726271063));
#33511=CARTESIAN_POINT('Ctrl Pts',(-2.79140942341378,-1.,-2.50410331873042));
#33512=CARTESIAN_POINT('Ctrl Pts',(-2.79145823440899,-1.,-2.50410700351426));
#33513=CARTESIAN_POINT('Ctrl Pts',(-2.79164172519039,-1.,-2.50417932839343));
#33514=CARTESIAN_POINT('Ctrl Pts',(-2.79217568804874,-1.,-2.50455968395235));
#33515=CARTESIAN_POINT('Ctrl Pts',(-2.79344192164204,-1.,-2.50567182569153));
#33516=CARTESIAN_POINT('Ctrl Pts',(-2.7959687805717,-1.,-2.50810555977564));
#33517=CARTESIAN_POINT('Ctrl Pts',(-2.79970585014308,-1.,-2.51186983687947));
#33518=CARTESIAN_POINT('Ctrl Pts',(-2.80427363984939,-1.,-2.51660190466067));
#33519=CARTESIAN_POINT('Ctrl Pts',(-2.80941521967234,-1.,-2.52205778589922));
#33520=CARTESIAN_POINT('Ctrl Pts',(-2.8148437904867,-1.,-2.52796388055457));
#33521=CARTESIAN_POINT('Ctrl Pts',(-2.82028550483744,-1.,-2.53405679667463));
#33522=CARTESIAN_POINT('Ctrl Pts',(-2.82552167649157,-1.,-2.54012272520141));
#33523=CARTESIAN_POINT('Ctrl Pts',(-2.83044254225794,-1.,-2.54604736792542));
#33524=CARTESIAN_POINT('Ctrl Pts',(-2.83505269592412,-1.,-2.55182152806964));
#33525=CARTESIAN_POINT('Ctrl Pts',(-2.83942515220699,-1.,-2.55749952145165));
#33526=CARTESIAN_POINT('Ctrl Pts',(-2.84366802680211,-1.,-2.56316920798489));
#33527=CARTESIAN_POINT('Ctrl Pts',(-2.84788893329091,-1.,-2.56891984251743));
#33528=CARTESIAN_POINT('Ctrl Pts',(-2.85215360144483,-1.,-2.57480482727128));
#33529=CARTESIAN_POINT('Ctrl Pts',(-2.85647171715147,-1.,-2.58082875254407));
#33530=CARTESIAN_POINT('Ctrl Pts',(-2.86081999003668,-1.,-2.5869677064356));
#33531=CARTESIAN_POINT('Ctrl Pts',(-2.86515629953528,-1.,-2.59318160184921));
#33532=CARTESIAN_POINT('Ctrl Pts',(-2.86943633170712,-1.,-2.59942875223202));
#33533=CARTESIAN_POINT('Ctrl Pts',(-2.87363176656475,-1.,-2.6056817788128));
#33534=CARTESIAN_POINT('Ctrl Pts',(-2.87773881947885,-1.,-2.61193507170928));
#33535=CARTESIAN_POINT('Ctrl Pts',(-2.88176821427502,-1.,-2.61819596473087));
#33536=CARTESIAN_POINT('Ctrl Pts',(-2.88573922195049,-1.,-2.62447947640253));
#33537=CARTESIAN_POINT('Ctrl Pts',(-2.88967244854243,-1.,-2.63080195420771));
#33538=CARTESIAN_POINT('Ctrl Pts',(-2.89358228854557,-1.,-2.63717442263944));
#33539=CARTESIAN_POINT('Ctrl Pts',(-2.89747231723361,-1.,-2.64359851684146));
#33540=CARTESIAN_POINT('Ctrl Pts',(-2.90133950224879,-1.,-2.65007017365576));
#33541=CARTESIAN_POINT('Ctrl Pts',(-2.90517678087467,-1.,-2.65658188464287));
#33542=CARTESIAN_POINT('Ctrl Pts',(-2.90897617968921,-1.,-2.66312542616808));
#33543=CARTESIAN_POINT('Ctrl Pts',(-2.91273193382876,-1.,-2.66969458792627));
#33544=CARTESIAN_POINT('Ctrl Pts',(-2.91644290704281,-1.,-2.67628728855309));
#33545=CARTESIAN_POINT('Ctrl Pts',(-2.92011090722152,-1.,-2.68290409279689));
#33546=CARTESIAN_POINT('Ctrl Pts',(-2.92373955325876,-1.,-2.68954721165342));
#33547=CARTESIAN_POINT('Ctrl Pts',(-2.92733294395268,-1.,-2.69621932864302));
#33548=CARTESIAN_POINT('Ctrl Pts',(-2.93089438233746,-1.,-2.70292247416881));
#33549=CARTESIAN_POINT('Ctrl Pts',(-2.93442516311168,-1.,-2.70965695523776));
#33550=CARTESIAN_POINT('Ctrl Pts',(-2.93792519474955,-1.,-2.71642190053575));
#33551=CARTESIAN_POINT('Ctrl Pts',(-2.94139351933882,-1.,-2.72321571511322));
#33552=CARTESIAN_POINT('Ctrl Pts',(-2.94482887675139,-1.,-2.73003657371613));
#33553=CARTESIAN_POINT('Ctrl Pts',(-2.94823023414381,-1.,-2.73688288329825));
#33554=CARTESIAN_POINT('Ctrl Pts',(-2.95159737214305,-1.,-2.7437537949221));
#33555=CARTESIAN_POINT('Ctrl Pts',(-2.95493069316211,-1.,-2.75064903318996));
#33556=CARTESIAN_POINT('Ctrl Pts',(-2.9582309766594,-1.,-2.75756867888393));
#33557=CARTESIAN_POINT('Ctrl Pts',(-2.96149914764832,-1.,-2.76451296269571));
#33558=CARTESIAN_POINT('Ctrl Pts',(-2.96473605585548,-1.,-2.77148206836464));
#33559=CARTESIAN_POINT('Ctrl Pts',(-2.9679422104295,-1.,-2.77847589542767));
#33560=CARTESIAN_POINT('Ctrl Pts',(-2.97111781461349,-1.,-2.78549409123657));
#33561=CARTESIAN_POINT('Ctrl Pts',(-2.97426288347475,-1.,-2.79253615718147));
#33562=CARTESIAN_POINT('Ctrl Pts',(-2.97737733718242,-1.,-2.79960153278186));
#33563=CARTESIAN_POINT('Ctrl Pts',(-2.98046109647299,-1.,-2.80668968101162));
#33564=CARTESIAN_POINT('Ctrl Pts',(-2.9835141977994,-1.,-2.81380019196454));
#33565=CARTESIAN_POINT('Ctrl Pts',(-2.98653680669434,-1.,-2.82093279065704));
#33566=CARTESIAN_POINT('Ctrl Pts',(-2.98952916401699,-1.,-2.82808728190402));
#33567=CARTESIAN_POINT('Ctrl Pts',(-2.99249155170479,-1.,-2.83526351254383));
#33568=CARTESIAN_POINT('Ctrl Pts',(-2.995424253416,-1.,-2.84246132984334));
#33569=CARTESIAN_POINT('Ctrl Pts',(-2.99832751144566,-1.,-2.84968053289104));
#33570=CARTESIAN_POINT('Ctrl Pts',(-3.0012015079552,-1.,-2.85692085715129));
#33571=CARTESIAN_POINT('Ctrl Pts',(-3.00404638316245,-1.,-2.86418200833065));
#33572=CARTESIAN_POINT('Ctrl Pts',(-3.00686224485374,-1.,-2.87146368430104));
#33573=CARTESIAN_POINT('Ctrl Pts',(-3.0096491810855,-1.,-2.87876560072799));
#33574=CARTESIAN_POINT('Ctrl Pts',(-3.01240727309568,-1.,-2.88608751706796));
#33575=CARTESIAN_POINT('Ctrl Pts',(-3.01513660433291,-1.,-2.8934292556764));
#33576=CARTESIAN_POINT('Ctrl Pts',(-3.01783725123646,-1.,-2.90079069102661));
#33577=CARTESIAN_POINT('Ctrl Pts',(-3.01997487194926,-1.,-2.90669553303902));
#33578=CARTESIAN_POINT('Ctrl Pts',(-3.02156522743299,-1.,-2.91113297349052));
#33579=CARTESIAN_POINT('Ctrl Pts',(-3.02261975104912,-1.,-2.91409518070707));
#33580=CARTESIAN_POINT('Ctrl Pts',(-3.02314558451372,-1.,-2.91557726271063));
#33581=CARTESIAN_POINT('',(-2.91557726271063,-1.,-3.02314558451372));
#33582=CARTESIAN_POINT('',(-3.02314558451372,-1.,-2.91557726271063));
#33583=CARTESIAN_POINT('',(-2.50410331873176,-1.,-2.79140942341258));
#33584=CARTESIAN_POINT('Ctrl Pts',(-2.91557726271063,-1.,-3.02314558451372));
#33585=CARTESIAN_POINT('Ctrl Pts',(-2.91409518070399,-1.,-3.02261975104593));
#33586=CARTESIAN_POINT('Ctrl Pts',(-2.91113297348212,-1.,-3.02156522742431));
#33587=CARTESIAN_POINT('Ctrl Pts',(-2.90669553302526,-1.,-3.01997487193503));
#33588=CARTESIAN_POINT('Ctrl Pts',(-2.9007906910105,-1.,-3.01783725121981));
#33589=CARTESIAN_POINT('Ctrl Pts',(-2.89342925566321,-1.,-3.01513660431928));
#33590=CARTESIAN_POINT('Ctrl Pts',(-2.8860875170608,-1.,-3.01240727308829));
#33591=CARTESIAN_POINT('Ctrl Pts',(-2.87876560072727,-1.,-3.00964918108476));
#33592=CARTESIAN_POINT('Ctrl Pts',(-2.87146368430502,-1.,-3.00686224485784));
#33593=CARTESIAN_POINT('Ctrl Pts',(-2.86418200833667,-1.,-3.00404638316867));
#33594=CARTESIAN_POINT('Ctrl Pts',(-2.85692085715686,-1.,-3.00120150796095));
#33595=CARTESIAN_POINT('Ctrl Pts',(-2.84968053289451,-1.,-2.99832751144925));
#33596=CARTESIAN_POINT('Ctrl Pts',(-2.84246132984415,-1.,-2.99542425341685));
#33597=CARTESIAN_POINT('Ctrl Pts',(-2.83526351254248,-1.,-2.99249155170339));
#33598=CARTESIAN_POINT('Ctrl Pts',(-2.82808728190157,-1.,-2.98952916401446));
#33599=CARTESIAN_POINT('Ctrl Pts',(-2.82093279065457,-1.,-2.9865368066918));
#33600=CARTESIAN_POINT('Ctrl Pts',(-2.81380019196286,-1.,-2.98351419779767));
#33601=CARTESIAN_POINT('Ctrl Pts',(-2.80668968101106,-1.,-2.98046109647241));
#33602=CARTESIAN_POINT('Ctrl Pts',(-2.7996015327823,-1.,-2.97737733718287));
#33603=CARTESIAN_POINT('Ctrl Pts',(-2.79253615718248,-1.,-2.9742628834758));
#33604=CARTESIAN_POINT('Ctrl Pts',(-2.78549409123769,-1.,-2.97111781461465));
#33605=CARTESIAN_POINT('Ctrl Pts',(-2.7784758954285,-1.,-2.96794221043036));
#33606=CARTESIAN_POINT('Ctrl Pts',(-2.77148206836498,-1.,-2.96473605585583));
#33607=CARTESIAN_POINT('Ctrl Pts',(-2.76451296269557,-1.,-2.96149914764818));
#33608=CARTESIAN_POINT('Ctrl Pts',(-2.7575686788835,-1.,-2.95823097665896));
#33609=CARTESIAN_POINT('Ctrl Pts',(-2.75064903318947,-1.,-2.95493069316161));
#33610=CARTESIAN_POINT('Ctrl Pts',(-2.74375379492172,-1.,-2.95159737214266));
#33611=CARTESIAN_POINT('Ctrl Pts',(-2.73688288329808,-1.,-2.94823023414364));
#33612=CARTESIAN_POINT('Ctrl Pts',(-2.73003657371617,-1.,-2.94482887675143));
#33613=CARTESIAN_POINT('Ctrl Pts',(-2.72321571511337,-1.,-2.94139351933897));
#33614=CARTESIAN_POINT('Ctrl Pts',(-2.71642190053592,-1.,-2.93792519474972));
#33615=CARTESIAN_POINT('Ctrl Pts',(-2.70965695523787,-1.,-2.93442516311179));
#33616=CARTESIAN_POINT('Ctrl Pts',(-2.70292247416885,-1.,-2.93089438233749));
#33617=CARTESIAN_POINT('Ctrl Pts',(-2.69621932864301,-1.,-2.92733294395267));
#33618=CARTESIAN_POINT('Ctrl Pts',(-2.68954721165339,-1.,-2.92373955325875));
#33619=CARTESIAN_POINT('Ctrl Pts',(-2.68290409279688,-1.,-2.92011090722152));
#33620=CARTESIAN_POINT('Ctrl Pts',(-2.67628728855312,-1.,-2.91644290704285));
#33621=CARTESIAN_POINT('Ctrl Pts',(-2.66969458792631,-1.,-2.91273193382882));
#33622=CARTESIAN_POINT('Ctrl Pts',(-2.6631254261681,-1.,-2.90897617968923));
#33623=CARTESIAN_POINT('Ctrl Pts',(-2.65658188464282,-1.,-2.90517678087461));
#33624=CARTESIAN_POINT('Ctrl Pts',(-2.65007017365564,-1.,-2.90133950224867));
#33625=CARTESIAN_POINT('Ctrl Pts',(-2.64359851684131,-1.,-2.89747231723345));
#33626=CARTESIAN_POINT('Ctrl Pts',(-2.63717442263932,-1.,-2.89358228854544));
#33627=CARTESIAN_POINT('Ctrl Pts',(-2.63080195420767,-1.,-2.88967244854239));
#33628=CARTESIAN_POINT('Ctrl Pts',(-2.62447947640262,-1.,-2.88573922195059));
#33629=CARTESIAN_POINT('Ctrl Pts',(-2.61819596473108,-1.,-2.88176821427525));
#33630=CARTESIAN_POINT('Ctrl Pts',(-2.61193507170955,-1.,-2.87773881947915));
#33631=CARTESIAN_POINT('Ctrl Pts',(-2.60568177881303,-1.,-2.87363176656501));
#33632=CARTESIAN_POINT('Ctrl Pts',(-2.5994287522321,-1.,-2.86943633170722));
#33633=CARTESIAN_POINT('Ctrl Pts',(-2.59318160184908,-1.,-2.86515629953513));
#33634=CARTESIAN_POINT('Ctrl Pts',(-2.58696770643524,-1.,-2.86081999003629));
#33635=CARTESIAN_POINT('Ctrl Pts',(-2.58082875254357,-1.,-2.85647171715092));
#33636=CARTESIAN_POINT('Ctrl Pts',(-2.57480482727081,-1.,-2.85215360144431));
#33637=CARTESIAN_POINT('Ctrl Pts',(-2.56891984251721,-1.,-2.84788893329067));
#33638=CARTESIAN_POINT('Ctrl Pts',(-2.56316920798513,-1.,-2.84366802680237));
#33639=CARTESIAN_POINT('Ctrl Pts',(-2.55749952145241,-1.,-2.83942515220782));
#33640=CARTESIAN_POINT('Ctrl Pts',(-2.55182152807077,-1.,-2.83505269592536));
#33641=CARTESIAN_POINT('Ctrl Pts',(-2.54604736792655,-1.,-2.83044254225917));
#33642=CARTESIAN_POINT('Ctrl Pts',(-2.54012272520199,-1.,-2.8255216764922));
#33643=CARTESIAN_POINT('Ctrl Pts',(-2.53405679667412,-1.,-2.82028550483689));
#33644=CARTESIAN_POINT('Ctrl Pts',(-2.52796388055278,-1.,-2.81484379048475));
#33645=CARTESIAN_POINT('Ctrl Pts',(-2.52205778589653,-1.,-2.80941521966941));
#33646=CARTESIAN_POINT('Ctrl Pts',(-2.51660190465805,-1.,-2.80427363984653));
#33647=CARTESIAN_POINT('Ctrl Pts',(-2.51186983687818,-1.,-2.79970585014168));
#33648=CARTESIAN_POINT('Ctrl Pts',(-2.50810555977671,-1.,-2.79596878057287));
#33649=CARTESIAN_POINT('Ctrl Pts',(-2.50567182569081,-1.,-2.79344192164147));
#33650=CARTESIAN_POINT('Ctrl Pts',(-2.50455968395146,-1.,-2.79217568804755));
#33651=CARTESIAN_POINT('Ctrl Pts',(-2.50417932839313,-1.,-2.79164172518905));
#33652=CARTESIAN_POINT('Ctrl Pts',(-2.50410700351493,-1.,-2.79145823440781));
#33653=CARTESIAN_POINT('Ctrl Pts',(-2.50410331873176,-1.,-2.79140942341258));
#33654=CARTESIAN_POINT('',(-2.36531447826213,-1.,-2.90994629141562));
#33655=CARTESIAN_POINT('Origin',(0.,-1.,0.));
#33656=CARTESIAN_POINT('',(-2.52982887637028,-1.,-3.35260583073571));
#33657=CARTESIAN_POINT('Ctrl Pts',(-2.36531447826213,-1.,-2.90994629141562));
#33658=CARTESIAN_POINT('Ctrl Pts',(-2.3653621118858,-1.,-2.90995756655558));
#33659=CARTESIAN_POINT('Ctrl Pts',(-2.36553202948741,-1.,-2.9100577052777));
#33660=CARTESIAN_POINT('Ctrl Pts',(-2.36599991765853,-1.,-2.91051690822262));
#33661=CARTESIAN_POINT('Ctrl Pts',(-2.36707658451709,-1.,-2.91181344022628));
#33662=CARTESIAN_POINT('Ctrl Pts',(-2.36919161373074,-1.,-2.91461249883016));
#33663=CARTESIAN_POINT('Ctrl Pts',(-2.37229381109939,-1.,-2.9189150379156));
#33664=CARTESIAN_POINT('Ctrl Pts',(-2.37606510524271,-1.,-2.92430340582912));
#33665=CARTESIAN_POINT('Ctrl Pts',(-2.3802898958232,-1.,-2.93049643640517));
#33666=CARTESIAN_POINT('Ctrl Pts',(-2.38472771516476,-1.,-2.93717903280599));
#33667=CARTESIAN_POINT('Ctrl Pts',(-2.38914929090806,-1.,-2.94404820669135));
#33668=CARTESIAN_POINT('Ctrl Pts',(-2.39337207631613,-1.,-2.95085857128372));
#33669=CARTESIAN_POINT('Ctrl Pts',(-2.39730553974412,-1.,-2.95748006482811));
#33670=CARTESIAN_POINT('Ctrl Pts',(-2.40095565711535,-1.,-2.96390432240181));
#33671=CARTESIAN_POINT('Ctrl Pts',(-2.40438604734848,-1.,-2.97019641312272));
#33672=CARTESIAN_POINT('Ctrl Pts',(-2.40768975073691,-1.,-2.97646002822395));
#33673=CARTESIAN_POINT('Ctrl Pts',(-2.41095909342591,-1.,-2.98280015815132));
#33674=CARTESIAN_POINT('Ctrl Pts',(-2.4142506419963,-1.,-2.98927983005851));
#33675=CARTESIAN_POINT('Ctrl Pts',(-2.4175732450056,-1.,-2.99590509293561));
#33676=CARTESIAN_POINT('Ctrl Pts',(-2.42090763946812,-1.,-3.00264868586038));
#33677=CARTESIAN_POINT('Ctrl Pts',(-2.42421849439625,-1.,-3.00946442616674));
#33678=CARTESIAN_POINT('Ctrl Pts',(-2.4274685626416,-1.,-3.01630420830494));
#33679=CARTESIAN_POINT('Ctrl Pts',(-2.43063415586615,-1.,-3.02313656035977));
#33680=CARTESIAN_POINT('Ctrl Pts',(-2.43371241361462,-1.,-3.02995534946946));
#33681=CARTESIAN_POINT('Ctrl Pts',(-2.43671278042394,-1.,-3.03676949672797));
#33682=CARTESIAN_POINT('Ctrl Pts',(-2.43965194061849,-1.,-3.04359685040545));
#33683=CARTESIAN_POINT('Ctrl Pts',(-2.44254768923109,-1.,-3.05045678021509));
#33684=CARTESIAN_POINT('Ctrl Pts',(-2.44541251892568,-1.,-3.05736242671521));
#33685=CARTESIAN_POINT('Ctrl Pts',(-2.44824970516558,-1.,-3.06431596421422));
#33686=CARTESIAN_POINT('Ctrl Pts',(-2.45105688854432,-1.,-3.0713129052131));
#33687=CARTESIAN_POINT('Ctrl Pts',(-2.45382826787795,-1.,-3.07834472886145));
#33688=CARTESIAN_POINT('Ctrl Pts',(-2.45655725437037,-1.,-3.08540206545313));
#33689=CARTESIAN_POINT('Ctrl Pts',(-2.45923912563875,-1.,-3.09247787931881));
#33690=CARTESIAN_POINT('Ctrl Pts',(-2.4618730850188,-1.,-3.09956993697048));
#33691=CARTESIAN_POINT('Ctrl Pts',(-2.46446082979645,-1.,-3.10667907901981));
#33692=CARTESIAN_POINT('Ctrl Pts',(-2.46700558843507,-1.,-3.11380805536124));
#33693=CARTESIAN_POINT('Ctrl Pts',(-2.4695109894747,-1.,-3.12096015766984));
#33694=CARTESIAN_POINT('Ctrl Pts',(-2.47197997765868,-1.,-3.12813790805948));
#33695=CARTESIAN_POINT('Ctrl Pts',(-2.47441378371923,-1.,-3.13534181229282));
#33696=CARTESIAN_POINT('Ctrl Pts',(-2.47681245356095,-1.,-3.14257099546531));
#33697=CARTESIAN_POINT('Ctrl Pts',(-2.47917529057016,-1.,-3.14982373241335));
#33698=CARTESIAN_POINT('Ctrl Pts',(-2.48150133566568,-1.,-3.15709802322735));
#33699=CARTESIAN_POINT('Ctrl Pts',(-2.48378981792739,-1.,-3.16439213290181));
#33700=CARTESIAN_POINT('Ctrl Pts',(-2.48604065348619,-1.,-3.17170518863357));
#33701=CARTESIAN_POINT('Ctrl Pts',(-2.48825428288243,-1.,-3.17903698136679));
#33702=CARTESIAN_POINT('Ctrl Pts',(-2.49043146334095,-1.,-3.18638771282315));
#33703=CARTESIAN_POINT('Ctrl Pts',(-2.4925730723986,-1.,-3.19375775555814));
#33704=CARTESIAN_POINT('Ctrl Pts',(-2.49467992057726,-1.,-3.20114742397549));
#33705=CARTESIAN_POINT('Ctrl Pts',(-2.49675252647298,-1.,-3.2085566984974));
#33706=CARTESIAN_POINT('Ctrl Pts',(-2.49879114599293,-1.,-3.21598526261157));
#33707=CARTESIAN_POINT('Ctrl Pts',(-2.5007958720187,-1.,-3.22343262620387));
#33708=CARTESIAN_POINT('Ctrl Pts',(-2.50276671338074,-1.,-3.23089822320596));
#33709=CARTESIAN_POINT('Ctrl Pts',(-2.50470367580078,-1.,-3.23838151080383));
#33710=CARTESIAN_POINT('Ctrl Pts',(-2.50660685940645,-1.,-3.24588208984042));
#33711=CARTESIAN_POINT('Ctrl Pts',(-2.50847647070936,-1.,-3.25339971461265));
#33712=CARTESIAN_POINT('Ctrl Pts',(-2.51031277813697,-1.,-3.26093423001716));
#33713=CARTESIAN_POINT('Ctrl Pts',(-2.51211608411539,-1.,-3.26848552888271));
#33714=CARTESIAN_POINT('Ctrl Pts',(-2.51388669270329,-1.,-3.27605350473048));
#33715=CARTESIAN_POINT('Ctrl Pts',(-2.51562487464215,-1.,-3.28363799702583));
#33716=CARTESIAN_POINT('Ctrl Pts',(-2.51733085123316,-1.,-3.2912387729863));
#33717=CARTESIAN_POINT('Ctrl Pts',(-2.51900480700548,-1.,-3.29885556387661));
#33718=CARTESIAN_POINT('Ctrl Pts',(-2.52064689568167,-1.,-3.30648808814986));
#33719=CARTESIAN_POINT('Ctrl Pts',(-2.52225724871375,-1.,-3.31413607874727));
#33720=CARTESIAN_POINT('Ctrl Pts',(-2.52383598396878,-1.,-3.32179931079521));
#33721=CARTESIAN_POINT('Ctrl Pts',(-2.52538321165774,-1.,-3.32947762189049));
#33722=CARTESIAN_POINT('Ctrl Pts',(-2.52689902691551,-1.,-3.33717090000955));
#33723=CARTESIAN_POINT('Ctrl Pts',(-2.52808660916879,-1.,-3.34333744117093));
#33724=CARTESIAN_POINT('Ctrl Pts',(-2.5289632161143,-1.,-3.34796903577628));
#33725=CARTESIAN_POINT('Ctrl Pts',(-2.52954136549357,-1.,-3.35105973714426));
#33726=CARTESIAN_POINT('Ctrl Pts',(-2.52982887637028,-1.,-3.35260583073571));
#33727=CARTESIAN_POINT('',(-2.40675750623143,-1.,-3.44202241512147));
#33728=CARTESIAN_POINT('',(-2.52982887637028,-1.,-3.35260583073571));
#33729=CARTESIAN_POINT('',(-2.03660101169715,-1.,-3.14877060440327));
#33730=CARTESIAN_POINT('Ctrl Pts',(-2.40675750623143,-1.,-3.44202241512147));
#33731=CARTESIAN_POINT('Ctrl Pts',(-2.4053759295909,-1.,-3.44127120683039));
#33732=CARTESIAN_POINT('Ctrl Pts',(-2.40261515589405,-1.,-3.43976627484234));
#33733=CARTESIAN_POINT('Ctrl Pts',(-2.39848113410292,-1.,-3.43750133064416));
#33734=CARTESIAN_POINT('Ctrl Pts',(-2.39298338804493,-1.,-3.4344663067854));
#33735=CARTESIAN_POINT('Ctrl Pts',(-2.38613505843552,-1.,-3.4306473271292));
#33736=CARTESIAN_POINT('Ctrl Pts',(-2.37931067028926,-1.,-3.42680309754399));
#33737=CARTESIAN_POINT('Ctrl Pts',(-2.37251035954292,-1.,-3.42293356216511));
#33738=CARTESIAN_POINT('Ctrl Pts',(-2.36573431470642,-1.,-3.41903866635852));
#33739=CARTESIAN_POINT('Ctrl Pts',(-2.35898278606946,-1.,-3.41511836751469));
#33740=CARTESIAN_POINT('Ctrl Pts',(-2.35225606824109,-1.,-3.41117262314119));
#33741=CARTESIAN_POINT('Ctrl Pts',(-2.34555447649188,-1.,-3.40720137404297));
#33742=CARTESIAN_POINT('Ctrl Pts',(-2.33887832342782,-1.,-3.40320452776743));
#33743=CARTESIAN_POINT('Ctrl Pts',(-2.33222789882489,-1.,-3.39918194577956));
#33744=CARTESIAN_POINT('Ctrl Pts',(-2.3256034390248,-1.,-3.39513342019756));
#33745=CARTESIAN_POINT('Ctrl Pts',(-2.31900513925424,-1.,-3.39105869474822));
#33746=CARTESIAN_POINT('Ctrl Pts',(-2.31243319489367,-1.,-3.38695751492462));
#33747=CARTESIAN_POINT('Ctrl Pts',(-2.30588783640343,-1.,-3.3828296733661));
#33748=CARTESIAN_POINT('Ctrl Pts',(-2.29936936127624,-1.,-3.37867504959433));
#33749=CARTESIAN_POINT('Ctrl Pts',(-2.29287818007393,-1.,-3.37449367172826));
#33750=CARTESIAN_POINT('Ctrl Pts',(-2.28641481081137,-1.,-3.37028570206488));
#33751=CARTESIAN_POINT('Ctrl Pts',(-2.27997979458037,-1.,-3.36605130713076));
#33752=CARTESIAN_POINT('Ctrl Pts',(-2.2735736262093,-1.,-3.36179055004409));
#33753=CARTESIAN_POINT('Ctrl Pts',(-2.2671966857991,-1.,-3.35750328523061));
#33754=CARTESIAN_POINT('Ctrl Pts',(-2.26084915222449,-1.,-3.35318902552626));
#33755=CARTESIAN_POINT('Ctrl Pts',(-2.25453097693483,-1.,-3.34884690292285));
#33756=CARTESIAN_POINT('Ctrl Pts',(-2.24824207678256,-1.,-3.34447596770723));
#33757=CARTESIAN_POINT('Ctrl Pts',(-2.24198249391422,-1.,-3.34007543738025));
#33758=CARTESIAN_POINT('Ctrl Pts',(-2.23575256328812,-1.,-3.33564495756482));
#33759=CARTESIAN_POINT('Ctrl Pts',(-2.22955308907233,-1.,-3.33118487773611));
#33760=CARTESIAN_POINT('Ctrl Pts',(-2.22338548312772,-1.,-3.3266964672289));
#33761=CARTESIAN_POINT('Ctrl Pts',(-2.21725135110898,-1.,-3.32218125618968));
#33762=CARTESIAN_POINT('Ctrl Pts',(-2.21115211847875,-1.,-3.31764044024235));
#33763=CARTESIAN_POINT('Ctrl Pts',(-2.20508863150607,-1.,-3.31307424608949));
#33764=CARTESIAN_POINT('Ctrl Pts',(-2.19906078949923,-1.,-3.30848134694595));
#33765=CARTESIAN_POINT('Ctrl Pts',(-2.19306710376111,-1.,-3.30385816281831));
#33766=CARTESIAN_POINT('Ctrl Pts',(-2.18710556500327,-1.,-3.29920022557639));
#33767=CARTESIAN_POINT('Ctrl Pts',(-2.18117455557065,-1.,-3.2945036150049));
#33768=CARTESIAN_POINT('Ctrl Pts',(-2.17527380048423,-1.,-3.28976645712568));
#33769=CARTESIAN_POINT('Ctrl Pts',(-2.16940517773455,-1.,-3.28499019979724));
#33770=CARTESIAN_POINT('Ctrl Pts',(-2.16357391934425,-1.,-3.280181508414));
#33771=CARTESIAN_POINT('Ctrl Pts',(-2.15778690038347,-1.,-3.27534954469187));
#33772=CARTESIAN_POINT('Ctrl Pts',(-2.15205043199808,-1.,-3.27050245897228));
#33773=CARTESIAN_POINT('Ctrl Pts',(-2.1463680529566,-1.,-3.26564388189759));
#33774=CARTESIAN_POINT('Ctrl Pts',(-2.14073870754264,-1.,-3.26077002641879));
#33775=CARTESIAN_POINT('Ctrl Pts',(-2.13515375878803,-1.,-3.25586495065054));
#33776=CARTESIAN_POINT('Ctrl Pts',(-2.12960028396832,-1.,-3.25090574494028));
#33777=CARTESIAN_POINT('Ctrl Pts',(-2.12406646410962,-1.,-3.24587102613376));
#33778=CARTESIAN_POINT('Ctrl Pts',(-2.11854673326979,-1.,-3.24074905517293));
#33779=CARTESIAN_POINT('Ctrl Pts',(-2.11304604021773,-1.,-3.23554444767099));
#33780=CARTESIAN_POINT('Ctrl Pts',(-2.10758699642451,-1.,-3.23028945793289));
#33781=CARTESIAN_POINT('Ctrl Pts',(-2.10220384298492,-1.,-3.22503437553434));
#33782=CARTESIAN_POINT('Ctrl Pts',(-2.09692958434895,-1.,-3.21982707347009));
#33783=CARTESIAN_POINT('Ctrl Pts',(-2.09178419460443,-1.,-3.21469429601654));
#33784=CARTESIAN_POINT('Ctrl Pts',(-2.08676465517455,-1.,-3.20962575845463));
#33785=CARTESIAN_POINT('Ctrl Pts',(-2.08182850370878,-1.,-3.2045481863073));
#33786=CARTESIAN_POINT('Ctrl Pts',(-2.07690441870722,-1.,-3.19934132836019));
#33787=CARTESIAN_POINT('Ctrl Pts',(-2.07192253497857,-1.,-3.19388465568252));
#33788=CARTESIAN_POINT('Ctrl Pts',(-2.06684062744112,-1.,-3.18809755562368));
#33789=CARTESIAN_POINT('Ctrl Pts',(-2.06166849827101,-1.,-3.18197692964614));
#33790=CARTESIAN_POINT('Ctrl Pts',(-2.05650186773132,-1.,-3.17564906975371));
#33791=CARTESIAN_POINT('Ctrl Pts',(-2.05151770247233,-1.,-3.16936341689527));
#33792=CARTESIAN_POINT('Ctrl Pts',(-2.04693331247446,-1.,-3.16343165058912));
#33793=CARTESIAN_POINT('Ctrl Pts',(-2.04297406404027,-1.,-3.15817983946367));
#33794=CARTESIAN_POINT('Ctrl Pts',(-2.03984073791519,-1.,-3.15389991674792));
#33795=CARTESIAN_POINT('Ctrl Pts',(-2.03783225495961,-1.,-3.15102344775328));
#33796=CARTESIAN_POINT('Ctrl Pts',(-2.03693188810544,-1.,-3.14959882629805));
#33797=CARTESIAN_POINT('Ctrl Pts',(-2.03663974554932,-1.,-3.1490119366901));
#33798=CARTESIAN_POINT('Ctrl Pts',(-2.03659701539259,-1.,-3.14881939088124));
#33799=CARTESIAN_POINT('Ctrl Pts',(-2.03660101169715,-1.,-3.14877060440328));
#33800=CARTESIAN_POINT('',(-1.88097764062697,-1.,-3.24413672884812));
#33801=CARTESIAN_POINT('Origin',(0.,-1.,0.));
#33802=CARTESIAN_POINT('',(-1.97421938526992,-1.,-3.70708211654725));
#33803=CARTESIAN_POINT('Ctrl Pts',(-1.88097764062697,-1.,-3.24413672884812));
#33804=CARTESIAN_POINT('Ctrl Pts',(-1.8810229239812,-1.,-3.24415531671284));
#33805=CARTESIAN_POINT('Ctrl Pts',(-1.88117508446775,-1.,-3.24428080353022));
#33806=CARTESIAN_POINT('Ctrl Pts',(-1.88156537699203,-1.,-3.24480754676064));
#33807=CARTESIAN_POINT('Ctrl Pts',(-1.88242596600454,-1.,-3.2462565441079));
#33808=CARTESIAN_POINT('Ctrl Pts',(-1.88407708646357,-1.,-3.24935200511918));
#33809=CARTESIAN_POINT('Ctrl Pts',(-1.88646802523466,-1.,-3.25408686339463));
#33810=CARTESIAN_POINT('Ctrl Pts',(-1.88934996203698,-1.,-3.25999885193947));
#33811=CARTESIAN_POINT('Ctrl Pts',(-1.89255393500965,-1.,-3.26677653888676));
#33812=CARTESIAN_POINT('Ctrl Pts',(-1.89589172903793,-1.,-3.27407108933139));
#33813=CARTESIAN_POINT('Ctrl Pts',(-1.89918429230462,-1.,-3.28154737912352));
#33814=CARTESIAN_POINT('Ctrl Pts',(-1.90228971247527,-1.,-3.2889344860029));
#33815=CARTESIAN_POINT('Ctrl Pts',(-1.90513891864087,-1.,-3.29608978722113));
#33816=CARTESIAN_POINT('Ctrl Pts',(-1.90773912171341,-1.,-3.30300595568195));
#33817=CARTESIAN_POINT('Ctrl Pts',(-1.91014297830446,-1.,-3.30975721158596));
#33818=CARTESIAN_POINT('Ctrl Pts',(-1.91242616234442,-1.,-3.31646052426364));
#33819=CARTESIAN_POINT('Ctrl Pts',(-1.91466343916628,-1.,-3.32323403454535));
#33820=CARTESIAN_POINT('Ctrl Pts',(-1.91690081930331,-1.,-3.33014884257873));
#33821=CARTESIAN_POINT('Ctrl Pts',(-1.9191460961021,-1.,-3.33721230710012));
#33822=CARTESIAN_POINT('Ctrl Pts',(-1.92138450828404,-1.,-3.34439448941961));
#33823=CARTESIAN_POINT('Ctrl Pts',(-1.92358838440528,-1.,-3.35164424847223));
#33824=CARTESIAN_POINT('Ctrl Pts',(-1.92572846125756,-1.,-3.35890824422965));
#33825=CARTESIAN_POINT('Ctrl Pts',(-1.92778626543786,-1.,-3.36615168657567));
#33826=CARTESIAN_POINT('Ctrl Pts',(-1.92975993109877,-1.,-3.37336807068043));
#33827=CARTESIAN_POINT('Ctrl Pts',(-1.93165739093276,-1.,-3.3805676852555));
#33828=CARTESIAN_POINT('Ctrl Pts',(-1.93349233176788,-1.,-3.38777076883256));
#33829=CARTESIAN_POINT('Ctrl Pts',(-1.93527929945985,-1.,-3.39499923640795));
#33830=CARTESIAN_POINT('Ctrl Pts',(-1.93702857723098,-1.,-3.40226802104109));
#33831=CARTESIAN_POINT('Ctrl Pts',(-1.93874306008143,-1.,-3.40957978266642));
#33832=CARTESIAN_POINT('Ctrl Pts',(-1.94042111965246,-1.,-3.41692971994096));
#33833=CARTESIAN_POINT('Ctrl Pts',(-1.94205835913696,-1.,-3.42430850941503));
#33834=CARTESIAN_POINT('Ctrl Pts',(-1.94364973660284,-1.,-3.43170586602434));
#33835=CARTESIAN_POINT('Ctrl Pts',(-1.94519168842879,-1.,-3.43911410197687));
#33836=CARTESIAN_POINT('Ctrl Pts',(-1.94668377715329,-1.,-3.44653088665681));
#33837=CARTESIAN_POINT('Ctrl Pts',(-1.94812754766524,-1.,-3.45395731584051));
#33838=CARTESIAN_POINT('Ctrl Pts',(-1.94952575850197,-1.,-3.46139661060962));
#33839=CARTESIAN_POINT('Ctrl Pts',(-1.95088147859877,-1.,-3.46885258974191));
#33840=CARTESIAN_POINT('Ctrl Pts',(-1.95219722189876,-1.,-3.47632820495921));
#33841=CARTESIAN_POINT('Ctrl Pts',(-1.95347412486309,-1.,-3.48382414832634));
#33842=CARTESIAN_POINT('Ctrl Pts',(-1.95471236969643,-1.,-3.49133956289133));
#33843=CARTESIAN_POINT('Ctrl Pts',(-1.95591153823661,-1.,-3.49887263575583));
#33844=CARTESIAN_POINT('Ctrl Pts',(-1.95707099606511,-1.,-3.50642124159909));
#33845=CARTESIAN_POINT('Ctrl Pts',(-1.95819025316779,-1.,-3.51398354617794));
#33846=CARTESIAN_POINT('Ctrl Pts',(-1.95926936324461,-1.,-3.52155867431486));
#33847=CARTESIAN_POINT('Ctrl Pts',(-1.96030879411566,-1.,-3.52914648844351));
#33848=CARTESIAN_POINT('Ctrl Pts',(-1.96130926212689,-1.,-3.53674730625813));
#33849=CARTESIAN_POINT('Ctrl Pts',(-1.96227157573067,-1.,-3.54436163300443));
#33850=CARTESIAN_POINT('Ctrl Pts',(-1.96319648628644,-1.,-3.55198990600886));
#33851=CARTESIAN_POINT('Ctrl Pts',(-1.96408450906812,-1.,-3.55963218706096));
#33852=CARTESIAN_POINT('Ctrl Pts',(-1.96493594634567,-1.,-3.56728820357791));
#33853=CARTESIAN_POINT('Ctrl Pts',(-1.96575096652789,-1.,-3.57495748600959));
#33854=CARTESIAN_POINT('Ctrl Pts',(-1.96652966688911,-1.,-3.58263947663829));
#33855=CARTESIAN_POINT('Ctrl Pts',(-1.96727213799544,-1.,-3.59033364022801));
#33856=CARTESIAN_POINT('Ctrl Pts',(-1.96797854118369,-1.,-3.59803959819938));
#33857=CARTESIAN_POINT('Ctrl Pts',(-1.9686491188594,-1.,-3.60575714017989));
#33858=CARTESIAN_POINT('Ctrl Pts',(-1.96928416040877,-1.,-3.61348615496704));
#33859=CARTESIAN_POINT('Ctrl Pts',(-1.96988398129978,-1.,-3.62122658401893));
#33860=CARTESIAN_POINT('Ctrl Pts',(-1.97044889850463,-1.,-3.62897836973293));
#33861=CARTESIAN_POINT('Ctrl Pts',(-1.97097920454464,-1.,-3.63674139590412));
#33862=CARTESIAN_POINT('Ctrl Pts',(-1.97147515441164,-1.,-3.64451546723514));
#33863=CARTESIAN_POINT('Ctrl Pts',(-1.9719369724024,-1.,-3.652300347166));
#33864=CARTESIAN_POINT('Ctrl Pts',(-1.9723648543905,-1.,-3.6600957816636));
#33865=CARTESIAN_POINT('Ctrl Pts',(-1.97275897198678,-1.,-3.66790152752075));
#33866=CARTESIAN_POINT('Ctrl Pts',(-1.97311947678517,-1.,-3.67571738107084));
#33867=CARTESIAN_POINT('Ctrl Pts',(-1.97344650304519,-1.,-3.68354319915092));
#33868=CARTESIAN_POINT('Ctrl Pts',(-1.97374016225483,-1.,-3.69137888599902));
#33869=CARTESIAN_POINT('Ctrl Pts',(-1.97394846383216,-1.,-3.6976552856004));
#33870=CARTESIAN_POINT('Ctrl Pts',(-1.97408973726715,-1.,-3.70236698912904));
#33871=CARTESIAN_POINT('Ctrl Pts',(-1.97417727645308,-1.,-3.70551008132332));
#33872=CARTESIAN_POINT('Ctrl Pts',(-1.97421938526992,-1.,-3.70708211654725));
#33873=CARTESIAN_POINT('',(-1.83867539237861,-1.,-3.77614523045147));
#33874=CARTESIAN_POINT('',(-1.97421938526992,-1.,-3.70708211654725));
#33875=CARTESIAN_POINT('',(-1.5189508286633,-1.,-3.42859860294306));
#33876=CARTESIAN_POINT('Ctrl Pts',(-1.83867539237861,-1.,-3.77614523045147));
#33877=CARTESIAN_POINT('Ctrl Pts',(-1.83742834010626,-1.,-3.77518714457833));
#33878=CARTESIAN_POINT('Ctrl Pts',(-1.83493697934534,-1.,-3.77326886064398));
#33879=CARTESIAN_POINT('Ctrl Pts',(-1.83120816955645,-1.,-3.77038509817999));
#33880=CARTESIAN_POINT('Ctrl Pts',(-1.82625289220915,-1.,-3.76652740353775));
#33881=CARTESIAN_POINT('Ctrl Pts',(-1.82008629694091,-1.,-3.76168412707948));
#33882=CARTESIAN_POINT('Ctrl Pts',(-1.8139472983358,-1.,-3.75681965683071));
#33883=CARTESIAN_POINT('Ctrl Pts',(-1.80783603939617,-1.,-3.75193395887977));
#33884=CARTESIAN_POINT('Ctrl Pts',(-1.8017527148577,-1.,-3.74702700875467));
#33885=CARTESIAN_POINT('Ctrl Pts',(-1.79569757859422,-1.,-3.74209880352445));
#33886=CARTESIAN_POINT('Ctrl Pts',(-1.78967092823491,-1.,-3.73714934730681));
#33887=CARTESIAN_POINT('Ctrl Pts',(-1.78367308442901,-1.,-3.7321786309547));
#33888=CARTESIAN_POINT('Ctrl Pts',(-1.77770437039658,-1.,-3.72718661205609));
#33889=CARTESIAN_POINT('Ctrl Pts',(-1.77176509401761,-1.,-3.72217319911254));
#33890=CARTESIAN_POINT('Ctrl Pts',(-1.76585552124394,-1.,-3.71713822377359));
#33891=CARTESIAN_POINT('Ctrl Pts',(-1.75997588498865,-1.,-3.71208146346136));
#33892=CARTESIAN_POINT('Ctrl Pts',(-1.75412641804042,-1.,-3.70700269736659));
#33893=CARTESIAN_POINT('Ctrl Pts',(-1.74830738046057,-1.,-3.7019017567335));
#33894=CARTESIAN_POINT('Ctrl Pts',(-1.74251908492617,-1.,-3.69677856910517));
#33895=CARTESIAN_POINT('Ctrl Pts',(-1.73676193254557,-1.,-3.69163322648036));
#33896=CARTESIAN_POINT('Ctrl Pts',(-1.73103640956717,-1.,-3.68646597019332));
#33897=CARTESIAN_POINT('Ctrl Pts',(-1.72534302437056,-1.,-3.68127704936579));
#33898=CARTESIAN_POINT('Ctrl Pts',(-1.71968225581808,-1.,-3.67606660374709));
#33899=CARTESIAN_POINT('Ctrl Pts',(-1.71405450210384,-1.,-3.67083454901611));
#33900=CARTESIAN_POINT('Ctrl Pts',(-1.70846001610956,-1.,-3.66558043198876));
#33901=CARTESIAN_POINT('Ctrl Pts',(-1.70289888566873,-1.,-3.66030338774847));
#33902=CARTESIAN_POINT('Ctrl Pts',(-1.69737117722534,-1.,-3.65500246526749));
#33903=CARTESIAN_POINT('Ctrl Pts',(-1.69187705481689,-1.,-3.64967689827371));
#33904=CARTESIAN_POINT('Ctrl Pts',(-1.68641690471457,-1.,-3.64432638915203));
#33905=CARTESIAN_POINT('Ctrl Pts',(-1.68099146651586,-1.,-3.63895140887462));
#33906=CARTESIAN_POINT('Ctrl Pts',(-1.67560193613156,-1.,-3.63355343201232));
#33907=CARTESIAN_POINT('Ctrl Pts',(-1.67024966008045,-1.,-3.62813422105271));
#33908=CARTESIAN_POINT('Ctrl Pts',(-1.66493585923855,-1.,-3.62269517989109));
#33909=CARTESIAN_POINT('Ctrl Pts',(-1.65966133399186,-1.,-3.61723666482456));
#33910=CARTESIAN_POINT('Ctrl Pts',(-1.65442619244325,-1.,-3.61175734965127));
#33911=CARTESIAN_POINT('Ctrl Pts',(-1.64922952425832,-1.,-3.60625346556992));
#33912=CARTESIAN_POINT('Ctrl Pts',(-1.64407004385582,-1.,-3.60072028513845));
#33913=CARTESIAN_POINT('Ctrl Pts',(-1.63894676675352,-1.,-3.59515368334893));
#33914=CARTESIAN_POINT('Ctrl Pts',(-1.6338597145126,-1.,-3.58955176627879));
#33915=CARTESIAN_POINT('Ctrl Pts',(-1.62881051550745,-1.,-3.58391625774343));
#33916=CARTESIAN_POINT('Ctrl Pts',(-1.62380329464844,-1.,-3.5782545595439));
#33917=CARTESIAN_POINT('Ctrl Pts',(-1.61884340915404,-1.,-3.57257679609806));
#33918=CARTESIAN_POINT('Ctrl Pts',(-1.61393581747514,-1.,-3.56689200468387));
#33919=CARTESIAN_POINT('Ctrl Pts',(-1.60908344685457,-1.,-3.5612043248298));
#33920=CARTESIAN_POINT('Ctrl Pts',(-1.60428584699853,-1.,-3.55550985096129));
#33921=CARTESIAN_POINT('Ctrl Pts',(-1.59953698113457,-1.,-3.54979148634454));
#33922=CARTESIAN_POINT('Ctrl Pts',(-1.59482766949766,-1.,-3.54402458182337));
#33923=CARTESIAN_POINT('Ctrl Pts',(-1.59014958368739,-1.,-3.53818616861077));
#33924=CARTESIAN_POINT('Ctrl Pts',(-1.58549906268088,-1.,-3.5322637814708));
#33925=CARTESIAN_POINT('Ctrl Pts',(-1.58088027227848,-1.,-3.52626275334881));
#33926=CARTESIAN_POINT('Ctrl Pts',(-1.57631049988158,-1.,-3.52021847865912));
#33927=CARTESIAN_POINT('Ctrl Pts',(-1.57181569799743,-1.,-3.51418598431665));
#33928=CARTESIAN_POINT('Ctrl Pts',(-1.56742097575012,-1.,-3.50821771695363));
#33929=CARTESIAN_POINT('Ctrl Pts',(-1.56314187758675,-1.,-3.50234321621578));
#33930=CARTESIAN_POINT('Ctrl Pts',(-1.55897703097874,-1.,-3.49655185179655));
#33931=CARTESIAN_POINT('Ctrl Pts',(-1.55489595901116,-1.,-3.4907646087742));
#33932=CARTESIAN_POINT('Ctrl Pts',(-1.55084702970452,-1.,-3.48485155928567));
#33933=CARTESIAN_POINT('Ctrl Pts',(-1.54678009290276,-1.,-3.47868272898751));
#33934=CARTESIAN_POINT('Ctrl Pts',(-1.54266605398187,-1.,-3.47217189224653));
#33935=CARTESIAN_POINT('Ctrl Pts',(-1.53851507915502,-1.,-3.46531752207153));
#33936=CARTESIAN_POINT('Ctrl Pts',(-1.53440195378792,-1.,-3.45825932955032));
#33937=CARTESIAN_POINT('Ctrl Pts',(-1.53046244461635,-1.,-3.45127136828305));
#33938=CARTESIAN_POINT('Ctrl Pts',(-1.52686242875556,-1.,-3.44469547526647));
#33939=CARTESIAN_POINT('Ctrl Pts',(-1.5237734895035,-1.,-3.4388889597401));
#33940=CARTESIAN_POINT('Ctrl Pts',(-1.52134826724293,-1.,-3.43417156977893));
#33941=CARTESIAN_POINT('Ctrl Pts',(-1.5198144909338,-1.,-3.43101631893414));
#33942=CARTESIAN_POINT('Ctrl Pts',(-1.51914806898491,-1.,-3.42946838852587));
#33943=CARTESIAN_POINT('Ctrl Pts',(-1.5189513329503,-1.,-3.42884302333841));
#33944=CARTESIAN_POINT('Ctrl Pts',(-1.51893924967331,-1.,-3.42864616361875));
#33945=CARTESIAN_POINT('Ctrl Pts',(-1.5189508286633,-1.,-3.42859860294306));
#33946=CARTESIAN_POINT('',(-1.35032489087269,-1.,-3.49844575334386));
#33947=CARTESIAN_POINT('Origin',(0.,-1.,0.));
#33948=CARTESIAN_POINT('',(-1.36999806084572,-1.,-3.97027773754922));
#33949=CARTESIAN_POINT('Ctrl Pts',(-1.35032489087269,-1.,-3.49844575334386));
#33950=CARTESIAN_POINT('Ctrl Pts',(-1.35036670893102,-1.,-3.49847119623841));
#33951=CARTESIAN_POINT('Ctrl Pts',(-1.35049736560633,-1.,-3.49861894124915));
#33952=CARTESIAN_POINT('Ctrl Pts',(-1.35080045218652,-1.,-3.49920025459856));
#33953=CARTESIAN_POINT('Ctrl Pts',(-1.35142377279535,-1.,-3.5007660381658));
#33954=CARTESIAN_POINT('Ctrl Pts',(-1.3525703284343,-1.,-3.50408168106113));
#33955=CARTESIAN_POINT('Ctrl Pts',(-1.35419113576022,-1.,-3.50913227060177));
#33956=CARTESIAN_POINT('Ctrl Pts',(-1.35611275237288,-1.,-3.51542230699919));
#33957=CARTESIAN_POINT('Ctrl Pts',(-1.35821701528975,-1.,-3.52261776117121));
#33958=CARTESIAN_POINT('Ctrl Pts',(-1.36037259643827,-1.,-3.53034464961849));
#33959=CARTESIAN_POINT('Ctrl Pts',(-1.36245507339334,-1.,-3.53824396425032));
#33960=CARTESIAN_POINT('Ctrl Pts',(-1.36436666257567,-1.,-3.54602591832893));
#33961=CARTESIAN_POINT('Ctrl Pts',(-1.36606145456711,-1.,-3.55353883995793));
#33962=CARTESIAN_POINT('Ctrl Pts',(-1.36754771771174,-1.,-3.56077662028492));
#33963=CARTESIAN_POINT('Ctrl Pts',(-1.36886584973349,-1.,-3.56782080304554));
#33964=CARTESIAN_POINT('Ctrl Pts',(-1.37007229485646,-1.,-3.57479875549453));
#33965=CARTESIAN_POINT('Ctrl Pts',(-1.37122241663073,-1.,-3.58183885982745));
#33966=CARTESIAN_POINT('Ctrl Pts',(-1.37235053661,-1.,-3.5890185384643));
#33967=CARTESIAN_POINT('Ctrl Pts',(-1.37346320103184,-1.,-3.59634627869117));
#33968=CARTESIAN_POINT('Ctrl Pts',(-1.37455051379642,-1.,-3.60379020124038));
#33969=CARTESIAN_POINT('Ctrl Pts',(-1.37559314436641,-1.,-3.61129546591082));
#33970=CARTESIAN_POINT('Ctrl Pts',(-1.37657053403102,-1.,-3.61880481160408));
#33971=CARTESIAN_POINT('Ctrl Pts',(-1.37746987919868,-1.,-3.62628098665112));
#33972=CARTESIAN_POINT('Ctrl Pts',(-1.37829035457324,-1.,-3.63371727442448));
#33973=CARTESIAN_POINT('Ctrl Pts',(-1.37903818567347,-1.,-3.64112507791112));
#33974=CARTESIAN_POINT('Ctrl Pts',(-1.37972372481598,-1.,-3.64852652756444));
#33975=CARTESIAN_POINT('Ctrl Pts',(-1.38035791051215,-1.,-3.65594554404396));
#33976=CARTESIAN_POINT('Ctrl Pts',(-1.38094856333558,-1.,-3.66339848520874));
#33977=CARTESIAN_POINT('Ctrl Pts',(-1.38149812653876,-1.,-3.67088843112282));
#33978=CARTESIAN_POINT('Ctrl Pts',(-1.38200574290626,-1.,-3.6784103848243));
#33979=CARTESIAN_POINT('Ctrl Pts',(-1.38246852827185,-1.,-3.68595444983844));
#33980=CARTESIAN_POINT('Ctrl Pts',(-1.38288311171649,-1.,-3.69350967899523));
#33981=CARTESIAN_POINT('Ctrl Pts',(-1.38324717612862,-1.,-3.70106792167894));
#33982=CARTESIAN_POINT('Ctrl Pts',(-1.38356065402122,-1.,-3.70862680753343));
#33983=CARTESIAN_POINT('Ctrl Pts',(-1.38382489984585,-1.,-3.7161876605181));
#33984=CARTESIAN_POINT('Ctrl Pts',(-1.3840421342895,-1.,-3.72375409358805));
#33985=CARTESIAN_POINT('Ctrl Pts',(-1.38421479111531,-1.,-3.73133035859283));
#33986=CARTESIAN_POINT('Ctrl Pts',(-1.38434489156456,-1.,-3.73891976418099));
#33987=CARTESIAN_POINT('Ctrl Pts',(-1.38443344984389,-1.,-3.7465231716786));
#33988=CARTESIAN_POINT('Ctrl Pts',(-1.38448077997155,-1.,-3.75413976318727));
#33989=CARTESIAN_POINT('Ctrl Pts',(-1.38448675253343,-1.,-3.76176768271347));
#33990=CARTESIAN_POINT('Ctrl Pts',(-1.38445107339517,-1.,-3.76940473185775));
#33991=CARTESIAN_POINT('Ctrl Pts',(-1.38437354551435,-1.,-3.77704902230441));
#33992=CARTESIAN_POINT('Ctrl Pts',(-1.38425435883773,-1.,-3.78469969805134));
#33993=CARTESIAN_POINT('Ctrl Pts',(-1.38409399694589,-1.,-3.79235669640907));
#33994=CARTESIAN_POINT('Ctrl Pts',(-1.38389311766701,-1.,-3.80002044322169));
#33995=CARTESIAN_POINT('Ctrl Pts',(-1.38365244046226,-1.,-3.80769156398429));
#33996=CARTESIAN_POINT('Ctrl Pts',(-1.38337263902766,-1.,-3.81537060817765));
#33997=CARTESIAN_POINT('Ctrl Pts',(-1.38305421262724,-1.,-3.82305771743715));
#33998=CARTESIAN_POINT('Ctrl Pts',(-1.38269750245086,-1.,-3.83075266982138));
#33999=CARTESIAN_POINT('Ctrl Pts',(-1.38230274828774,-1.,-3.83845502790609));
#34000=CARTESIAN_POINT('Ctrl Pts',(-1.38187013346089,-1.,-3.84616425605705));
#34001=CARTESIAN_POINT('Ctrl Pts',(-1.38139983115075,-1.,-3.85387983979557));
#34002=CARTESIAN_POINT('Ctrl Pts',(-1.38089205993067,-1.,-3.86160143044187));
#34003=CARTESIAN_POINT('Ctrl Pts',(-1.38034709213129,-1.,-3.86932885813403));
#34004=CARTESIAN_POINT('Ctrl Pts',(-1.37976523097187,-1.,-3.87706205830865));
#34005=CARTESIAN_POINT('Ctrl Pts',(-1.37914679719446,-1.,-3.88480102249461));
#34006=CARTESIAN_POINT('Ctrl Pts',(-1.37849211287981,-1.,-3.89254574338385));
#34007=CARTESIAN_POINT('Ctrl Pts',(-1.3778014851263,-1.,-3.90029615196255));
#34008=CARTESIAN_POINT('Ctrl Pts',(-1.3770751963376,-1.,-3.90805209522729));
#34009=CARTESIAN_POINT('Ctrl Pts',(-1.37631350505516,-1.,-3.91581337461825));
#34010=CARTESIAN_POINT('Ctrl Pts',(-1.37551664448057,-1.,-3.92357976987132));
#34011=CARTESIAN_POINT('Ctrl Pts',(-1.37468482215784,-1.,-3.93135106761941));
#34012=CARTESIAN_POINT('Ctrl Pts',(-1.37381821967499,-1.,-3.93912709041791));
#34013=CARTESIAN_POINT('Ctrl Pts',(-1.37291699203423,-1.,-3.94690771786926));
#34014=CARTESIAN_POINT('Ctrl Pts',(-1.37198126433139,-1.,-3.95469287283105));
#34015=CARTESIAN_POINT('Ctrl Pts',(-1.37120515615663,-1.,-3.96092458508407));
#34016=CARTESIAN_POINT('Ctrl Pts',(-1.37060761746027,-1.,-3.96560037975788));
#34017=CARTESIAN_POINT('Ctrl Pts',(-1.37020239094758,-1.,-3.9687184694173));
#34018=CARTESIAN_POINT('Ctrl Pts',(-1.36999806084572,-1.,-3.97027773754922));
#34019=CARTESIAN_POINT('',(-1.22531898815164,-1.,-4.01728681790024));
#34020=CARTESIAN_POINT('',(-1.36999806084572,-1.,-3.97027773754922));
#34021=CARTESIAN_POINT('',(-0.963899035118986,-1.,-3.62400312501199));
#34022=CARTESIAN_POINT('Ctrl Pts',(-1.22531898815164,-1.,-4.01728681790024));
#34023=CARTESIAN_POINT('Ctrl Pts',(-1.22423716681317,-1.,-4.01614544569895));
#34024=CARTESIAN_POINT('Ctrl Pts',(-1.22207656455845,-1.,-4.01386104433519));
#34025=CARTESIAN_POINT('Ctrl Pts',(-1.21884478244403,-1.,-4.01042947140789));
#34026=CARTESIAN_POINT('Ctrl Pts',(-1.21455398918133,-1.,-4.00584409522722));
#34027=CARTESIAN_POINT('Ctrl Pts',(-1.20922097029551,-1.,-4.00009577950721));
#34028=CARTESIAN_POINT('Ctrl Pts',(-1.20391852375139,-1.,-3.99433084799666));
#34029=CARTESIAN_POINT('Ctrl Pts',(-1.19864679609566,-1.,-3.98854928957189));
#34030=CARTESIAN_POINT('Ctrl Pts',(-1.19340598349475,-1.,-3.98275111052561));
#34031=CARTESIAN_POINT('Ctrl Pts',(-1.18819633715539,-1.,-3.97693634767754));
#34032=CARTESIAN_POINT('Ctrl Pts',(-1.18301815039831,-1.,-3.97110505165415));
#34033=CARTESIAN_POINT('Ctrl Pts',(-1.17787174135592,-1.,-3.96525726358159));
#34034=CARTESIAN_POINT('Ctrl Pts',(-1.17275743590361,-1.,-3.95939299213276));
#34035=CARTESIAN_POINT('Ctrl Pts',(-1.16767555244438,-1.,-3.95351219509876));
#34036=CARTESIAN_POINT('Ctrl Pts',(-1.16262637999157,-1.,-3.94761474780583));
#34037=CARTESIAN_POINT('Ctrl Pts',(-1.15761018340956,-1.,-3.94170046685203));
#34038=CARTESIAN_POINT('Ctrl Pts',(-1.1526272271632,-1.,-3.9357691705628));
#34039=CARTESIAN_POINT('Ctrl Pts',(-1.14767779451123,-1.,-3.92982073294257));
#34040=CARTESIAN_POINT('Ctrl Pts',(-1.14276220561593,-1.,-3.92385513133997));
#34041=CARTESIAN_POINT('Ctrl Pts',(-1.13788084225554,-1.,-3.91787251936827));
#34042=CARTESIAN_POINT('Ctrl Pts',(-1.13303414693896,-1.,-3.91187321145649));
#34043=CARTESIAN_POINT('Ctrl Pts',(-1.12822258281553,-1.,-3.90585753318737));
#34044=CARTESIAN_POINT('Ctrl Pts',(-1.12344660099043,-1.,-3.89982569750025));
#34045=CARTESIAN_POINT('Ctrl Pts',(-1.11870660794603,-1.,-3.89377768340344));
#34046=CARTESIAN_POINT('Ctrl Pts',(-1.11400292434429,-1.,-3.88771308285171));
#34047=CARTESIAN_POINT('Ctrl Pts',(-1.10933577224008,-1.,-3.88163105531724));
#34048=CARTESIAN_POINT('Ctrl Pts',(-1.10470536603287,-1.,-3.87553067187514));
#34049=CARTESIAN_POINT('Ctrl Pts',(-1.10011198761195,-1.,-3.86941120134849));
#34050=CARTESIAN_POINT('Ctrl Pts',(-1.09555606505013,-1.,-3.86327241021247));
#34051=CARTESIAN_POINT('Ctrl Pts',(-1.09103825516294,-1.,-3.85711487933931));
#34052=CARTESIAN_POINT('Ctrl Pts',(-1.08655950846384,-1.,-3.85094025222713));
#34053=CARTESIAN_POINT('Ctrl Pts',(-1.08212087917991,-1.,-3.8447504803063));
#34054=CARTESIAN_POINT('Ctrl Pts',(-1.07772335353858,-1.,-3.83854714117491));
#34055=CARTESIAN_POINT('Ctrl Pts',(-1.07336766633459,-1.,-3.83233071195144));
#34056=CARTESIAN_POINT('Ctrl Pts',(-1.06905413180359,-1.,-3.82609989967276));
#34057=CARTESIAN_POINT('Ctrl Pts',(-1.0647824403893,-1.,-3.81985083953012));
#34058=CARTESIAN_POINT('Ctrl Pts',(-1.06055206187299,-1.,-3.8135786611749));
#34059=CARTESIAN_POINT('Ctrl Pts',(-1.05636266918644,-1.,-3.80727913637791));
#34060=CARTESIAN_POINT('Ctrl Pts',(-1.05221457990016,-1.,-3.80095039790681));
#34061=CARTESIAN_POINT('Ctrl Pts',(-1.04810913267639,-1.,-3.79459440308786));
#34062=CARTESIAN_POINT('Ctrl Pts',(-1.04404924374422,-1.,-3.78821910787179));
#34063=CARTESIAN_POINT('Ctrl Pts',(-1.04003862055798,-1.,-3.7818353500817));
#34064=CARTESIAN_POINT('Ctrl Pts',(-1.03608074678008,-1.,-3.77545283140427));
#34065=CARTESIAN_POINT('Ctrl Pts',(-1.03217786604919,-1.,-3.76907609832516));
#34066=CARTESIAN_POINT('Ctrl Pts',(-1.02833014458184,-1.,-3.76270122291245));
#34067=CARTESIAN_POINT('Ctrl Pts',(-1.02453429444668,-1.,-3.75631037456224));
#34068=CARTESIAN_POINT('Ctrl Pts',(-1.02078510487439,-1.,-3.74987777155873));
#34069=CARTESIAN_POINT('Ctrl Pts',(-1.01707794311088,-1.,-3.74337942504993));
#34070=CARTESIAN_POINT('Ctrl Pts',(-1.01341114319906,-1.,-3.73680245055747));
#34071=CARTESIAN_POINT('Ctrl Pts',(-1.00978798539491,-1.,-3.73015276704407));
#34072=CARTESIAN_POINT('Ctrl Pts',(-1.00622000735696,-1.,-3.72346803750544));
#34073=CARTESIAN_POINT('Ctrl Pts',(-1.00272423396802,-1.,-3.71680667125047));
#34074=CARTESIAN_POINT('Ctrl Pts',(-0.999317260756344,-1.,-3.7102243971387));
#34075=CARTESIAN_POINT('Ctrl Pts',(-0.996009819772432,-1.,-3.70375282282107));
#34076=CARTESIAN_POINT('Ctrl Pts',(-0.992802218332104,-1.,-3.69738123415696));
#34077=CARTESIAN_POINT('Ctrl Pts',(-0.989676715398858,-1.,-3.69102682138955));
#34078=CARTESIAN_POINT('Ctrl Pts',(-0.986602639864286,-1.,-3.6845531792623));
#34079=CARTESIAN_POINT('Ctrl Pts',(-0.983550791470864,-1.,-3.67782408841876));
#34080=CARTESIAN_POINT('Ctrl Pts',(-0.980505922458494,-1.,-3.67074983340444));
#34081=CARTESIAN_POINT('Ctrl Pts',(-0.977478312751416,-1.,-3.66333049637403));
#34082=CARTESIAN_POINT('Ctrl Pts',(-0.974519971354139,-1.,-3.6557157673487));
#34083=CARTESIAN_POINT('Ctrl Pts',(-0.971722122060277,-1.,-3.64819756447072));
#34084=CARTESIAN_POINT('Ctrl Pts',(-0.969195124674829,-1.,-3.64113946505393));
#34085=CARTESIAN_POINT('Ctrl Pts',(-0.967052554540877,-1.,-3.6349212208096));
#34086=CARTESIAN_POINT('Ctrl Pts',(-0.965395153165716,-1.,-3.62988252139998));
#34087=CARTESIAN_POINT('Ctrl Pts',(-0.964373850166081,-1.,-3.62652618145252));
#34088=CARTESIAN_POINT('Ctrl Pts',(-0.963957782642589,-1.,-3.62489305727516));
#34089=CARTESIAN_POINT('Ctrl Pts',(-0.963861297423579,-1.,-3.62424461507455));
#34090=CARTESIAN_POINT('Ctrl Pts',(-0.963880158556713,-1.,-3.62404828878374));
#34091=CARTESIAN_POINT('Ctrl Pts',(-0.963899035118986,-1.,-3.62400312501199));
#34092=CARTESIAN_POINT('',(-0.786422660833743,-1.,-3.66661143271648));
#34093=CARTESIAN_POINT('Origin',(0.,-1.,0.));
#34094=CARTESIAN_POINT('',(-0.732042837400619,-1.,-4.13571194405636));
#34095=CARTESIAN_POINT('Ctrl Pts',(-0.786422660833743,-1.,-3.66661143271648));
#34096=CARTESIAN_POINT('Ctrl Pts',(-0.786459983896781,-1.,-3.66664310415236));
#34097=CARTESIAN_POINT('Ctrl Pts',(-0.78656591955989,-1.,-3.66680946938396));
#34098=CARTESIAN_POINT('Ctrl Pts',(-0.786774337198499,-1.,-3.66743103898844));
#34099=CARTESIAN_POINT('Ctrl Pts',(-0.787145041181589,-1.,-3.66907505398769));
#34100=CARTESIAN_POINT('Ctrl Pts',(-0.787758799995426,-1.,-3.672529236635));
#34101=CARTESIAN_POINT('Ctrl Pts',(-0.788569566220662,-1.,-3.67777119516438));
#34102=CARTESIAN_POINT('Ctrl Pts',(-0.789483546065158,-1.,-3.68428439784285));
#34103=CARTESIAN_POINT('Ctrl Pts',(-0.79043628498958,-1.,-3.69172044327754));
#34104=CARTESIAN_POINT('Ctrl Pts',(-0.791356575696509,-1.,-3.69968940808982));
#34105=CARTESIAN_POINT('Ctrl Pts',(-0.792177688845968,-1.,-3.70781724021879));
#34106=CARTESIAN_POINT('Ctrl Pts',(-0.792848377370115,-1.,-3.7158024239604));
#34107=CARTESIAN_POINT('Ctrl Pts',(-0.79334702378387,-1.,-3.7234879729357));
#34108=CARTESIAN_POINT('Ctrl Pts',(-0.793682750269347,-1.,-3.7308691469564));
#34109=CARTESIAN_POINT('Ctrl Pts',(-0.79388270093679,-1.,-3.73803280541576));
#34110=CARTESIAN_POINT('Ctrl Pts',(-0.79398270045988,-1.,-3.74511357728827));
#34111=CARTESIAN_POINT('Ctrl Pts',(-0.794017347371441,-1.,-3.75224692493895));
#34112=CARTESIAN_POINT('Ctrl Pts',(-0.794008429135047,-1.,-3.75951468666325));
#34113=CARTESIAN_POINT('Ctrl Pts',(-0.793961083689141,-1.,-3.76692626931184));
#34114=CARTESIAN_POINT('Ctrl Pts',(-0.793870523787515,-1.,-3.77444863801264));
#34115=CARTESIAN_POINT('Ctrl Pts',(-0.793726235781339,-1.,-3.78202460377617));
#34116=CARTESIAN_POINT('Ctrl Pts',(-0.793516871680966,-1.,-3.78959439439222));
#34117=CARTESIAN_POINT('Ctrl Pts',(-0.7932356129732,-1.,-3.79711921389862));
#34118=CARTESIAN_POINT('Ctrl Pts',(-0.792882695234693,-1.,-3.80459229925598));
#34119=CARTESIAN_POINT('Ctrl Pts',(-0.792462483517568,-1.,-3.81202588694726));
#34120=CARTESIAN_POINT('Ctrl Pts',(-0.791981740718606,-1.,-3.81944345442237));
#34121=CARTESIAN_POINT('Ctrl Pts',(-0.791447528662381,-1.,-3.82687033899799));
#34122=CARTESIAN_POINT('Ctrl Pts',(-0.79086501270534,-1.,-3.83432392054804));
#34123=CARTESIAN_POINT('Ctrl Pts',(-0.790236124191289,-1.,-3.84180762342476));
#34124=CARTESIAN_POINT('Ctrl Pts',(-0.789560798155619,-1.,-3.8493163780891));
#34125=CARTESIAN_POINT('Ctrl Pts',(-0.788837734090688,-1.,-3.85683995872536));
#34126=CARTESIAN_POINT('Ctrl Pts',(-0.788065315093771,-1.,-3.86436702561342));
#34127=CARTESIAN_POINT('Ctrl Pts',(-0.78724252761798,-1.,-3.87188916600905));
#34128=CARTESIAN_POINT('Ctrl Pts',(-0.786369675812592,-1.,-3.87940402818186));
#34129=CARTESIAN_POINT('Ctrl Pts',(-0.785447890340723,-1.,-3.88691313167399));
#34130=CARTESIAN_POINT('Ctrl Pts',(-0.784478799358336,-1.,-3.89442039235105));
#34131=CARTESIAN_POINT('Ctrl Pts',(-0.783464141529082,-1.,-3.90193039043971));
#34132=CARTESIAN_POINT('Ctrl Pts',(-0.782405395622759,-1.,-3.90944671004536));
#34133=CARTESIAN_POINT('Ctrl Pts',(-0.781303428618344,-1.,-3.9169703605466));
#34134=CARTESIAN_POINT('Ctrl Pts',(-0.780158678615507,-1.,-3.92450058323799));
#34135=CARTESIAN_POINT('Ctrl Pts',(-0.778971308134786,-1.,-3.93203552473153));
#34136=CARTESIAN_POINT('Ctrl Pts',(-0.77774137056855,-1.,-3.93957296768098));
#34137=CARTESIAN_POINT('Ctrl Pts',(-0.77646896669796,-1.,-3.94711101619471));
#34138=CARTESIAN_POINT('Ctrl Pts',(-0.775154418039441,-1.,-3.95464885452364));
#34139=CARTESIAN_POINT('Ctrl Pts',(-0.773798212026683,-1.,-3.96218649639876));
#34140=CARTESIAN_POINT('Ctrl Pts',(-0.772400931772239,-1.,-3.96972446532832));
#34141=CARTESIAN_POINT('Ctrl Pts',(-0.770963190030504,-1.,-3.97726349165507));
#34142=CARTESIAN_POINT('Ctrl Pts',(-0.769485566245459,-1.,-3.98480422348403));
#34143=CARTESIAN_POINT('Ctrl Pts',(-0.767968531377708,-1.,-3.99234687880892));
#34144=CARTESIAN_POINT('Ctrl Pts',(-0.766412457135786,-1.,-3.99989129179464));
#34145=CARTESIAN_POINT('Ctrl Pts',(-0.764817648784946,-1.,-4.00743706791366));
#34146=CARTESIAN_POINT('Ctrl Pts',(-0.763184371182827,-1.,-4.01498370680434));
#34147=CARTESIAN_POINT('Ctrl Pts',(-0.761512875859942,-1.,-4.02253072741347));
#34148=CARTESIAN_POINT('Ctrl Pts',(-0.759803433244166,-1.,-4.0300778195465));
#34149=CARTESIAN_POINT('Ctrl Pts',(-0.758056338885554,-1.,-4.03762485803468));
#34150=CARTESIAN_POINT('Ctrl Pts',(-0.756271902370187,-1.,-4.04517182654344));
#34151=CARTESIAN_POINT('Ctrl Pts',(-0.754450441816412,-1.,-4.05271876688106));
#34152=CARTESIAN_POINT('Ctrl Pts',(-0.752592276482869,-1.,-4.06026572221399));
#34153=CARTESIAN_POINT('Ctrl Pts',(-0.750697720483176,-1.,-4.06781267241886));
#34154=CARTESIAN_POINT('Ctrl Pts',(-0.748767076679177,-1.,-4.07535951055363));
#34155=CARTESIAN_POINT('Ctrl Pts',(-0.746800631490822,-1.,-4.08290608094789));
#34156=CARTESIAN_POINT('Ctrl Pts',(-0.744798649705514,-1.,-4.09045220253011));
#34157=CARTESIAN_POINT('Ctrl Pts',(-0.742761369690018,-1.,-4.09799769702712));
#34158=CARTESIAN_POINT('Ctrl Pts',(-0.740688998555152,-1.,-4.1055424175856));
#34159=CARTESIAN_POINT('Ctrl Pts',(-0.738581708229119,-1.,-4.11308626953795));
#34160=CARTESIAN_POINT('Ctrl Pts',(-0.736439634335347,-1.,-4.12062919626082));
#34161=CARTESIAN_POINT('Ctrl Pts',(-0.734698226767512,-1.,-4.12666277572794));
#34162=CARTESIAN_POINT('Ctrl Pts',(-0.733376589325634,-1.,-4.13118752796397));
#34163=CARTESIAN_POINT('Ctrl Pts',(-0.732488575135926,-1.,-4.13420383737278));
#34164=CARTESIAN_POINT('Ctrl Pts',(-0.732042837400619,-1.,-4.13571194405636));
#34165=CARTESIAN_POINT('',(-0.581791163835814,-1.,-4.15950947128175));
#34166=CARTESIAN_POINT('',(-0.732042837400619,-1.,-4.13571194405636));
#34167=CARTESIAN_POINT('',(-0.385112848332549,-1.,-3.73017266276632));
#34168=CARTESIAN_POINT('Ctrl Pts',(-0.581791163835814,-1.,-4.15950947128175));
#34169=CARTESIAN_POINT('Ctrl Pts',(-0.580901211462913,-1.,-4.15821291712391));
#34170=CARTESIAN_POINT('Ctrl Pts',(-0.579124568912543,-1.,-4.15561864787379));
#34171=CARTESIAN_POINT('Ctrl Pts',(-0.576469391673917,-1.,-4.1517237611974));
#34172=CARTESIAN_POINT('Ctrl Pts',(-0.572948736066277,-1.,-4.14652361065787));
#34173=CARTESIAN_POINT('Ctrl Pts',(-0.568580610187116,-1.,-4.14001179828669));
#34174=CARTESIAN_POINT('Ctrl Pts',(-0.564245279535705,-1.,-4.13348835726086));
#34175=CARTESIAN_POINT('Ctrl Pts',(-0.559942890594628,-1.,-4.12695329951859));
#34176=CARTESIAN_POINT('Ctrl Pts',(-0.555673636130778,-1.,-4.1204066619623));
#34177=CARTESIAN_POINT('Ctrl Pts',(-0.551437758498247,-1.,-4.11384852025578));
#34178=CARTESIAN_POINT('Ctrl Pts',(-0.54723553948676,-1.,-4.1072789702877));
#34179=CARTESIAN_POINT('Ctrl Pts',(-0.543067286878457,-1.,-4.10069810244473));
#34180=CARTESIAN_POINT('Ctrl Pts',(-0.538933321179921,-1.,-4.09410597627116));
#34181=CARTESIAN_POINT('Ctrl Pts',(-0.534833963476999,-1.,-4.08750259988693));
#34182=CARTESIAN_POINT('Ctrl Pts',(-0.530769518728075,-1.,-4.08088789536488));
#34183=CARTESIAN_POINT('Ctrl Pts',(-0.526740277227,-1.,-4.07426172299496));
#34184=CARTESIAN_POINT('Ctrl Pts',(-0.522746528602768,-1.,-4.06762394471075));
#34185=CARTESIAN_POINT('Ctrl Pts',(-0.51878857233681,-1.,-4.06097448037934));
#34186=CARTESIAN_POINT('Ctrl Pts',(-0.514866728193104,-1.,-4.05431335771261));
#34187=CARTESIAN_POINT('Ctrl Pts',(-0.510981349219174,-1.,-4.04764078815591));
#34188=CARTESIAN_POINT('Ctrl Pts',(-0.507132823288362,-1.,-4.04095715149074));
#34189=CARTESIAN_POINT('Ctrl Pts',(-0.503321556915514,-1.,-4.0342628417439));
#34190=CARTESIAN_POINT('Ctrl Pts',(-0.49954796234089,-1.,-4.0275581398015));
#34191=CARTESIAN_POINT('Ctrl Pts',(-0.495812444326223,-1.,-4.02084308851813));
#34192=CARTESIAN_POINT('Ctrl Pts',(-0.492115383417931,-1.,-4.01411733503486));
#34193=CARTESIAN_POINT('Ctrl Pts',(-0.488457130424531,-1.,-4.0073800839092));
#34194=CARTESIAN_POINT('Ctrl Pts',(-0.484838042421754,-1.,-4.00063045119234));
#34195=CARTESIAN_POINT('Ctrl Pts',(-0.481258512209638,-1.,-3.99386775880655));
#34196=CARTESIAN_POINT('Ctrl Pts',(-0.477718999122033,-1.,-3.98709184306743));
#34197=CARTESIAN_POINT('Ctrl Pts',(-0.474220061019542,-1.,-3.9803033804443));
#34198=CARTESIAN_POINT('Ctrl Pts',(-0.470762379613477,-1.,-3.97350414289415));
#34199=CARTESIAN_POINT('Ctrl Pts',(-0.467346690880672,-1.,-3.96669622273946));
#34200=CARTESIAN_POINT('Ctrl Pts',(-0.463973722115744,-1.,-3.95988133243543));
#34201=CARTESIAN_POINT('Ctrl Pts',(-0.460644124429119,-1.,-3.95306005817363));
#34202=CARTESIAN_POINT('Ctrl Pts',(-0.457358410451674,-1.,-3.94623117206675));
#34203=CARTESIAN_POINT('Ctrl Pts',(-0.454116879027576,-1.,-3.93939080846298));
#34204=CARTESIAN_POINT('Ctrl Pts',(-0.450919768356347,-1.,-3.93253407403128));
#34205=CARTESIAN_POINT('Ctrl Pts',(-0.447767416837297,-1.,-3.92565674143424));
#34206=CARTESIAN_POINT('Ctrl Pts',(-0.444660430230593,-1.,-3.91875701610721));
#34207=CARTESIAN_POINT('Ctrl Pts',(-0.441599824524047,-1.,-3.91183704069146));
#34208=CARTESIAN_POINT('Ctrl Pts',(-0.438587235458233,-1.,-3.90490512938546));
#34209=CARTESIAN_POINT('Ctrl Pts',(-0.435624629433506,-1.,-3.8979725665544));
#34210=CARTESIAN_POINT('Ctrl Pts',(-0.432713929544439,-1.,-3.89104947940592));
#34211=CARTESIAN_POINT('Ctrl Pts',(-0.429856640579734,-1.,-3.88414070943334));
#34212=CARTESIAN_POINT('Ctrl Pts',(-0.427053541173469,-1.,-3.87724240306609));
#34213=CARTESIAN_POINT('Ctrl Pts',(-0.424304173195142,-1.,-3.87033643487882));
#34214=CARTESIAN_POINT('Ctrl Pts',(-0.421607423177576,-1.,-3.86339652542749));
#34215=CARTESIAN_POINT('Ctrl Pts',(-0.41896246808681,-1.,-3.85639825648031));
#34216=CARTESIAN_POINT('Ctrl Pts',(-0.41636967805292,-1.,-3.8493286415751));
#34217=CARTESIAN_POINT('Ctrl Pts',(-0.413831367016727,-1.,-3.84219403994742));
#34218=CARTESIAN_POINT('Ctrl Pts',(-0.41135303879846,-1.,-3.83503345578645));
#34219=CARTESIAN_POINT('Ctrl Pts',(-0.408942371447377,-1.,-3.82790724256397));
#34220=CARTESIAN_POINT('Ctrl Pts',(-0.406607038258906,-1.,-3.82087303913741));
#34221=CARTESIAN_POINT('Ctrl Pts',(-0.404352694628236,-1.,-3.81396374287762));
#34222=CARTESIAN_POINT('Ctrl Pts',(-0.402181320148475,-1.,-3.80716881962763));
#34223=CARTESIAN_POINT('Ctrl Pts',(-0.400088346504727,-1.,-3.80040370384659));
#34224=CARTESIAN_POINT('Ctrl Pts',(-0.398064818684158,-1.,-3.79352887163457));
#34225=CARTESIAN_POINT('Ctrl Pts',(-0.396103205335029,-1.,-3.78640521279479));
#34226=CARTESIAN_POINT('Ctrl Pts',(-0.394202481011595,-1.,-3.77894173114368));
#34227=CARTESIAN_POINT('Ctrl Pts',(-0.392372786223347,-1.,-3.77114011595892));
#34228=CARTESIAN_POINT('Ctrl Pts',(-0.390642072979259,-1.,-3.76315635032993));
#34229=CARTESIAN_POINT('Ctrl Pts',(-0.389054775898251,-1.,-3.75529302894757));
#34230=CARTESIAN_POINT('Ctrl Pts',(-0.387663020050396,-1.,-3.74792651696269));
#34231=CARTESIAN_POINT('Ctrl Pts',(-0.386519576222035,-1.,-3.74144965781088));
#34232=CARTESIAN_POINT('Ctrl Pts',(-0.385670806454744,-1.,-3.73621371845475));
#34233=CARTESIAN_POINT('Ctrl Pts',(-0.385187124633965,-1.,-3.73273893363318));
#34234=CARTESIAN_POINT('Ctrl Pts',(-0.385031656499141,-1.,-3.73106082862399));
#34235=CARTESIAN_POINT('Ctrl Pts',(-0.385037797882046,-1.,-3.73040527620929));
#34236=CARTESIAN_POINT('Ctrl Pts',(-0.385087139001609,-1.,-3.73021431755218));
#34237=CARTESIAN_POINT('Ctrl Pts',(-0.385112848332549,-1.,-3.73017266276632));
#34238=CARTESIAN_POINT('',(-0.203156094897896,-1.,-3.74449296982994));
#34239=CARTESIAN_POINT('Origin',(0.,-1.,0.));
#34240=CARTESIAN_POINT('',(-0.0760622897878238,-1.,-4.19931119685982));
#34241=CARTESIAN_POINT('Ctrl Pts',(-0.203156094897896,-1.,-3.74449296982994));
#34242=CARTESIAN_POINT('Ctrl Pts',(-0.203188003947965,-1.,-3.74453008995129));
#34243=CARTESIAN_POINT('Ctrl Pts',(-0.203266610111264,-1.,-3.74471097893961));
#34244=CARTESIAN_POINT('Ctrl Pts',(-0.203375226874331,-1.,-3.74535749969262));
#34245=CARTESIAN_POINT('Ctrl Pts',(-0.203484186269315,-1.,-3.74703926501843));
#34246=CARTESIAN_POINT('Ctrl Pts',(-0.203550035479097,-1.,-3.75054693397716));
#34247=CARTESIAN_POINT('Ctrl Pts',(-0.203530796848404,-1.,-3.75585118707924));
#34248=CARTESIAN_POINT('Ctrl Pts',(-0.203414634707646,-1.,-3.76242717937273));
#34249=CARTESIAN_POINT('Ctrl Pts',(-0.203192390045337,-1.,-3.76992071595267));
#34250=CARTESIAN_POINT('Ctrl Pts',(-0.202854729699197,-1.,-3.77793553476879));
#34251=CARTESIAN_POINT('Ctrl Pts',(-0.202394260512193,-1.,-3.78609175019317));
#34252=CARTESIAN_POINT('Ctrl Pts',(-0.201807533800799,-1.,-3.79408354187274));
#34253=CARTESIAN_POINT('Ctrl Pts',(-0.201097756307252,-1.,-3.80175247447171));
#34254=CARTESIAN_POINT('Ctrl Pts',(-0.20027467943329,-1.,-3.80909529318501));
#34255=CARTESIAN_POINT('Ctrl Pts',(-0.199351525297396,-1.,-3.81620203429702));
#34256=CARTESIAN_POINT('Ctrl Pts',(-0.19834261690047,-1.,-3.82321127348981));
#34257=CARTESIAN_POINT('Ctrl Pts',(-0.197260935827375,-1.,-3.83026221776488));
#34258=CARTESIAN_POINT('Ctrl Pts',(-0.19611519897189,-1.,-3.83743910616265));
#34259=CARTESIAN_POINT('Ctrl Pts',(-0.194909009460255,-1.,-3.84475203347052));
#34260=CARTESIAN_POINT('Ctrl Pts',(-0.193642806777748,-1.,-3.85216762264019));
#34261=CARTESIAN_POINT('Ctrl Pts',(-0.19231515304498,-1.,-3.85962774407652));
#34262=CARTESIAN_POINT('Ctrl Pts',(-0.190924190418613,-1.,-3.8670715862477));
#34263=CARTESIAN_POINT('Ctrl Pts',(-0.189469253358254,-1.,-3.87445976418377));
#34264=CARTESIAN_POINT('Ctrl Pts',(-0.187951632512663,-1.,-3.88178563496187));
#34265=CARTESIAN_POINT('Ctrl Pts',(-0.186373724985263,-1.,-3.88906196725817));
#34266=CARTESIAN_POINT('Ctrl Pts',(-0.184738537728035,-1.,-3.89631300742633));
#34267=CARTESIAN_POINT('Ctrl Pts',(-0.183049081993193,-1.,-3.90356488555138));
#34268=CARTESIAN_POINT('Ctrl Pts',(-0.181307740731796,-1.,-3.91083557557193));
#34269=CARTESIAN_POINT('Ctrl Pts',(-0.179515885822895,-1.,-3.91812876180948));
#34270=CARTESIAN_POINT('Ctrl Pts',(-0.177674246152328,-1.,-3.92543942697672));
#34271=CARTESIAN_POINT('Ctrl Pts',(-0.175783136893873,-1.,-3.93275726771049));
#34272=CARTESIAN_POINT('Ctrl Pts',(-0.173842734974607,-1.,-3.94007083096214));
#34273=CARTESIAN_POINT('Ctrl Pts',(-0.171853355369233,-1.,-3.94737164900861));
#34274=CARTESIAN_POINT('Ctrl Pts',(-0.16981566637413,-1.,-3.95465744665263));
#34275=CARTESIAN_POINT('Ctrl Pts',(-0.167730547023312,-1.,-3.96192990160296));
#34276=CARTESIAN_POINT('Ctrl Pts',(-0.165598992851098,-1.,-3.9691931362141));
#34277=CARTESIAN_POINT('Ctrl Pts',(-0.163422004609999,-1.,-3.97645194630944));
#34278=CARTESIAN_POINT('Ctrl Pts',(-0.161200482186088,-1.,-3.98371010319866));
#34279=CARTESIAN_POINT('Ctrl Pts',(-0.158935123982796,-1.,-3.99096873945862));
#34280=CARTESIAN_POINT('Ctrl Pts',(-0.156626481393736,-1.,-3.99822717425869));
#34281=CARTESIAN_POINT('Ctrl Pts',(-0.15427500487231,-1.,-4.00548360245297));
#34282=CARTESIAN_POINT('Ctrl Pts',(-0.151881094022909,-1.,-4.01273584234684));
#34283=CARTESIAN_POINT('Ctrl Pts',(-0.149445144968708,-1.,-4.01998203715588));
#34284=CARTESIAN_POINT('Ctrl Pts',(-0.146967602878999,-1.,-4.02722143147048));
#34285=CARTESIAN_POINT('Ctrl Pts',(-0.144448947038352,-1.,-4.03445411510403));
#34286=CARTESIAN_POINT('Ctrl Pts',(-0.141889671485508,-1.,-4.04168069633842));
#34287=CARTESIAN_POINT('Ctrl Pts',(-0.13929026718006,-1.,-4.04890199238056));
#34288=CARTESIAN_POINT('Ctrl Pts',(-0.136651205046111,-1.,-4.05611873400122));
#34289=CARTESIAN_POINT('Ctrl Pts',(-0.133972916144225,-1.,-4.06333121018476));
#34290=CARTESIAN_POINT('Ctrl Pts',(-0.131255793548914,-1.,-4.07053931528579));
#34291=CARTESIAN_POINT('Ctrl Pts',(-0.128500200484814,-1.,-4.07774270738809));
#34292=CARTESIAN_POINT('Ctrl Pts',(-0.125706476822529,-1.,-4.08494093372315));
#34293=CARTESIAN_POINT('Ctrl Pts',(-0.122874946249119,-1.,-4.09213355850836));
#34294=CARTESIAN_POINT('Ctrl Pts',(-0.120005924388162,-1.,-4.09932031767243));
#34295=CARTESIAN_POINT('Ctrl Pts',(-0.117099722731705,-1.,-4.10650113382187));
#34296=CARTESIAN_POINT('Ctrl Pts',(-0.114156649609602,-1.,-4.11367603925313));
#34297=CARTESIAN_POINT('Ctrl Pts',(-0.111177012683377,-1.,-4.12084512502444));
#34298=CARTESIAN_POINT('Ctrl Pts',(-0.10816112052835,-1.,-4.12800848371386));
#34299=CARTESIAN_POINT('Ctrl Pts',(-0.105109286538864,-1.,-4.13516614458396));
#34300=CARTESIAN_POINT('Ctrl Pts',(-0.102021826577454,-1.,-4.14231804938737));
#34301=CARTESIAN_POINT('Ctrl Pts',(-0.0988990478899814,-1.,-4.1494640891762));
#34302=CARTESIAN_POINT('Ctrl Pts',(-0.095741240329707,-1.,-4.15660412653006));
#34303=CARTESIAN_POINT('Ctrl Pts',(-0.0925486672167692,-1.,-4.16373802265942));
#34304=CARTESIAN_POINT('Ctrl Pts',(-0.089321556085033,-1.,-4.17086566491823));
#34305=CARTESIAN_POINT('Ctrl Pts',(-0.0860600915552517,-1.,-4.17798698669991));
#34306=CARTESIAN_POINT('Ctrl Pts',(-0.0827644164389512,-1.,-4.1851019532944));
#34307=CARTESIAN_POINT('Ctrl Pts',(-0.0801005887117605,-1.,-4.19078883322483));
#34308=CARTESIAN_POINT('Ctrl Pts',(-0.0780873956244405,-1.,-4.19505112860624));
#34309=CARTESIAN_POINT('Ctrl Pts',(-0.0767384596142197,-1.,-4.19789138621624));
#34310=CARTESIAN_POINT('Ctrl Pts',(-0.0760622897878238,-1.,-4.19931119685982));
#34311=CARTESIAN_POINT('',(0.0760622897878244,-1.,-4.19931119685982));
#34312=CARTESIAN_POINT('',(-0.0760622897878238,-1.,-4.19931119685982));
#34313=CARTESIAN_POINT('',(0.2031560948961,-1.,-3.74449296983004));
#34314=CARTESIAN_POINT('Ctrl Pts',(0.0760622897878244,-1.,-4.19931119685982));
#34315=CARTESIAN_POINT('Ctrl Pts',(0.0767384596141462,-1.,-4.1978913862118));
#34316=CARTESIAN_POINT('Ctrl Pts',(0.0780873956242395,-1.,-4.19505112859416));
#34317=CARTESIAN_POINT('Ctrl Pts',(0.0801005887114317,-1.,-4.19078883320504));
#34318=CARTESIAN_POINT('Ctrl Pts',(0.0827644164385676,-1.,-4.18510195327123));
#34319=CARTESIAN_POINT('Ctrl Pts',(0.0860600915549394,-1.,-4.17798698668094));
#34320=CARTESIAN_POINT('Ctrl Pts',(0.0893215560848647,-1.,-4.17086566490794));
#34321=CARTESIAN_POINT('Ctrl Pts',(0.0925486672167528,-1.,-4.16373802265839));
#34322=CARTESIAN_POINT('Ctrl Pts',(0.0957412403298004,-1.,-4.15660412653577));
#34323=CARTESIAN_POINT('Ctrl Pts',(0.0988990478901223,-1.,-4.14946408918485));
#34324=CARTESIAN_POINT('Ctrl Pts',(0.102021826577584,-1.,-4.14231804939538));
#34325=CARTESIAN_POINT('Ctrl Pts',(0.105109286538945,-1.,-4.13516614458895));
#34326=CARTESIAN_POINT('Ctrl Pts',(0.108161120528369,-1.,-4.12800848371504));
#34327=CARTESIAN_POINT('Ctrl Pts',(0.111177012683346,-1.,-4.1208451250225));
#34328=CARTESIAN_POINT('Ctrl Pts',(0.114156649609545,-1.,-4.11367603924961));
#34329=CARTESIAN_POINT('Ctrl Pts',(0.117099722731648,-1.,-4.10650113381833));
#34330=CARTESIAN_POINT('Ctrl Pts',(0.120005924388124,-1.,-4.09932031767002));
#34331=CARTESIAN_POINT('Ctrl Pts',(0.122874946249107,-1.,-4.09213355850756));
#34332=CARTESIAN_POINT('Ctrl Pts',(0.12570647682254,-1.,-4.08494093372377));
#34333=CARTESIAN_POINT('Ctrl Pts',(0.128500200484837,-1.,-4.07774270738954));
#34334=CARTESIAN_POINT('Ctrl Pts',(0.13125579354894,-1.,-4.0705393152874));
#34335=CARTESIAN_POINT('Ctrl Pts',(0.133972916144245,-1.,-4.06333121018596));
#34336=CARTESIAN_POINT('Ctrl Pts',(0.136651205046119,-1.,-4.05611873400172));
#34337=CARTESIAN_POINT('Ctrl Pts',(0.139290267180057,-1.,-4.04890199238036));
#34338=CARTESIAN_POINT('Ctrl Pts',(0.1418896714855,-1.,-4.04168069633781));
#34339=CARTESIAN_POINT('Ctrl Pts',(0.144448947038344,-1.,-4.03445411510333));
#34340=CARTESIAN_POINT('Ctrl Pts',(0.146967602878994,-1.,-4.02722143146994));
#34341=CARTESIAN_POINT('Ctrl Pts',(0.149445144968707,-1.,-4.01998203715564));
#34342=CARTESIAN_POINT('Ctrl Pts',(0.15188109402291,-1.,-4.01273584234689));
#34343=CARTESIAN_POINT('Ctrl Pts',(0.15427500487231,-1.,-4.00548360245319));
#34344=CARTESIAN_POINT('Ctrl Pts',(0.156626481393734,-1.,-3.99822717425893));
#34345=CARTESIAN_POINT('Ctrl Pts',(0.158935123982793,-1.,-3.99096873945878));
#34346=CARTESIAN_POINT('Ctrl Pts',(0.161200482186084,-1.,-3.98371010319872));
#34347=CARTESIAN_POINT('Ctrl Pts',(0.163422004609999,-1.,-3.97645194630943));
#34348=CARTESIAN_POINT('Ctrl Pts',(0.165598992851102,-1.,-3.96919313621407));
#34349=CARTESIAN_POINT('Ctrl Pts',(0.167730547023319,-1.,-3.96192990160296));
#34350=CARTESIAN_POINT('Ctrl Pts',(0.169815666374139,-1.,-3.95465744665268));
#34351=CARTESIAN_POINT('Ctrl Pts',(0.17185335536924,-1.,-3.94737164900868));
#34352=CARTESIAN_POINT('Ctrl Pts',(0.173842734974609,-1.,-3.94007083096217));
#34353=CARTESIAN_POINT('Ctrl Pts',(0.175783136893868,-1.,-3.93275726771042));
#34354=CARTESIAN_POINT('Ctrl Pts',(0.177674246152317,-1.,-3.92543942697655));
#34355=CARTESIAN_POINT('Ctrl Pts',(0.179515885822881,-1.,-3.91812876180926));
#34356=CARTESIAN_POINT('Ctrl Pts',(0.181307740731785,-1.,-3.91083557557175));
#34357=CARTESIAN_POINT('Ctrl Pts',(0.18304908199319,-1.,-3.90356488555132));
#34358=CARTESIAN_POINT('Ctrl Pts',(0.184738537728043,-1.,-3.89631300742646));
#34359=CARTESIAN_POINT('Ctrl Pts',(0.18637372498528,-1.,-3.88906196725848));
#34360=CARTESIAN_POINT('Ctrl Pts',(0.187951632512685,-1.,-3.88178563496228));
#34361=CARTESIAN_POINT('Ctrl Pts',(0.189469253358272,-1.,-3.87445976418412));
#34362=CARTESIAN_POINT('Ctrl Pts',(0.19092419041862,-1.,-3.86707158624783));
#34363=CARTESIAN_POINT('Ctrl Pts',(0.19231515304497,-1.,-3.85962774407633));
#34364=CARTESIAN_POINT('Ctrl Pts',(0.193642806777723,-1.,-3.85216762263966));
#34365=CARTESIAN_POINT('Ctrl Pts',(0.19490900946022,-1.,-3.84475203346977));
#34366=CARTESIAN_POINT('Ctrl Pts',(0.196115198971859,-1.,-3.83743910616195));
#34367=CARTESIAN_POINT('Ctrl Pts',(0.197260935827361,-1.,-3.83026221776456));
#34368=CARTESIAN_POINT('Ctrl Pts',(0.198342616900486,-1.,-3.82321127349016));
#34369=CARTESIAN_POINT('Ctrl Pts',(0.199351525297447,-1.,-3.81620203429815));
#34370=CARTESIAN_POINT('Ctrl Pts',(0.200274679433364,-1.,-3.80909529318669));
#34371=CARTESIAN_POINT('Ctrl Pts',(0.201097756307326,-1.,-3.80175247447337));
#34372=CARTESIAN_POINT('Ctrl Pts',(0.201807533800837,-1.,-3.7940835418736));
#34373=CARTESIAN_POINT('Ctrl Pts',(0.20239426051216,-1.,-3.78609175019242));
#34374=CARTESIAN_POINT('Ctrl Pts',(0.202854729699081,-1.,-3.77793553476614));
#34375=CARTESIAN_POINT('Ctrl Pts',(0.203192390045164,-1.,-3.7699207159487));
#34376=CARTESIAN_POINT('Ctrl Pts',(0.203414634707478,-1.,-3.76242717936885));
#34377=CARTESIAN_POINT('Ctrl Pts',(0.203530796848321,-1.,-3.75585118707734));
#34378=CARTESIAN_POINT('Ctrl Pts',(0.203550035479166,-1.,-3.75054693397875));
#34379=CARTESIAN_POINT('Ctrl Pts',(0.203484186269415,-1.,-3.74703926501752));
#34380=CARTESIAN_POINT('Ctrl Pts',(0.203375226874121,-1.,-3.74535749969115));
#34381=CARTESIAN_POINT('Ctrl Pts',(0.203266610110531,-1.,-3.74471097893845));
#34382=CARTESIAN_POINT('Ctrl Pts',(0.203188003946657,-1.,-3.74453008995092));
#34383=CARTESIAN_POINT('Ctrl Pts',(0.2031560948961,-1.,-3.74449296983004));
#34384=CARTESIAN_POINT('',(0.385112848330761,-1.,-3.73017266276651));
#34385=CARTESIAN_POINT('Origin',(0.,-1.,0.));
#34386=CARTESIAN_POINT('',(0.581791163835815,-1.,-4.15950947128175));
#34387=CARTESIAN_POINT('Ctrl Pts',(0.385112848330761,-1.,-3.73017266276651));
#34388=CARTESIAN_POINT('Ctrl Pts',(0.385087139000374,-1.,-3.73021431755274));
#34389=CARTESIAN_POINT('Ctrl Pts',(0.385037797881504,-1.,-3.73040527621055));
#34390=CARTESIAN_POINT('Ctrl Pts',(0.385031656499164,-1.,-3.73106082862548));
#34391=CARTESIAN_POINT('Ctrl Pts',(0.385187124634206,-1.,-3.73273893363406));
#34392=CARTESIAN_POINT('Ctrl Pts',(0.385670806454565,-1.,-3.73621371845318));
#34393=CARTESIAN_POINT('Ctrl Pts',(0.386519576222251,-1.,-3.74144965781276));
#34394=CARTESIAN_POINT('Ctrl Pts',(0.387663020050836,-1.,-3.74792651696654));
#34395=CARTESIAN_POINT('Ctrl Pts',(0.389054775898701,-1.,-3.75529302895152));
#34396=CARTESIAN_POINT('Ctrl Pts',(0.390642072979559,-1.,-3.76315635033257));
#34397=CARTESIAN_POINT('Ctrl Pts',(0.392372786223432,-1.,-3.77114011595967));
#34398=CARTESIAN_POINT('Ctrl Pts',(0.394202481011499,-1.,-3.77894173114283));
#34399=CARTESIAN_POINT('Ctrl Pts',(0.39610320533484,-1.,-3.78640521279313));
#34400=CARTESIAN_POINT('Ctrl Pts',(0.398064818683969,-1.,-3.7935288716329));
#34401=CARTESIAN_POINT('Ctrl Pts',(0.4000883465046,-1.,-3.80040370384546));
#34402=CARTESIAN_POINT('Ctrl Pts',(0.402181320148435,-1.,-3.80716881962728));
#34403=CARTESIAN_POINT('Ctrl Pts',(0.404352694628273,-1.,-3.81396374287793));
#34404=CARTESIAN_POINT('Ctrl Pts',(0.406607038258985,-1.,-3.8208730391381));
#34405=CARTESIAN_POINT('Ctrl Pts',(0.408942371447459,-1.,-3.82790724256471));
#34406=CARTESIAN_POINT('Ctrl Pts',(0.411353038798518,-1.,-3.83503345578698));
#34407=CARTESIAN_POINT('Ctrl Pts',(0.413831367016748,-1.,-3.84219403994762));
#34408=CARTESIAN_POINT('Ctrl Pts',(0.416369678052906,-1.,-3.84932864157497));
#34409=CARTESIAN_POINT('Ctrl Pts',(0.418962468086773,-1.,-3.85639825647996));
#34410=CARTESIAN_POINT('Ctrl Pts',(0.421607423177534,-1.,-3.86339652542709));
#34411=CARTESIAN_POINT('Ctrl Pts',(0.42430417319511,-1.,-3.87033643487851));
#34412=CARTESIAN_POINT('Ctrl Pts',(0.427053541173457,-1.,-3.87724240306597));
#34413=CARTESIAN_POINT('Ctrl Pts',(0.429856640579741,-1.,-3.88414070943341));
#34414=CARTESIAN_POINT('Ctrl Pts',(0.432713929544458,-1.,-3.89104947940611));
#34415=CARTESIAN_POINT('Ctrl Pts',(0.435624629433527,-1.,-3.89797256655462));
#34416=CARTESIAN_POINT('Ctrl Pts',(0.438587235458249,-1.,-3.90490512938563));
#34417=CARTESIAN_POINT('Ctrl Pts',(0.441599824524054,-1.,-3.91183704069153));
#34418=CARTESIAN_POINT('Ctrl Pts',(0.44466043023059,-1.,-3.91875701610719));
#34419=CARTESIAN_POINT('Ctrl Pts',(0.447767416837292,-1.,-3.92565674143416));
#34420=CARTESIAN_POINT('Ctrl Pts',(0.450919768356348,-1.,-3.93253407403123));
#34421=CARTESIAN_POINT('Ctrl Pts',(0.454116879027584,-1.,-3.93939080846298));
#34422=CARTESIAN_POINT('Ctrl Pts',(0.457358410451682,-1.,-3.94623117206678));
#34423=CARTESIAN_POINT('Ctrl Pts',(0.460644124429121,-1.,-3.95306005817364));
#34424=CARTESIAN_POINT('Ctrl Pts',(0.463973722115733,-1.,-3.95988133243538));
#34425=CARTESIAN_POINT('Ctrl Pts',(0.467346690880643,-1.,-3.9666962227393));
#34426=CARTESIAN_POINT('Ctrl Pts',(0.470762379613439,-1.,-3.97350414289392));
#34427=CARTESIAN_POINT('Ctrl Pts',(0.474220061019509,-1.,-3.98030338044409));
#34428=CARTESIAN_POINT('Ctrl Pts',(0.477718999122027,-1.,-3.98709184306738));
#34429=CARTESIAN_POINT('Ctrl Pts',(0.481258512209675,-1.,-3.99386775880679));
#34430=CARTESIAN_POINT('Ctrl Pts',(0.484838042421834,-1.,-4.00063045119288));
#34431=CARTESIAN_POINT('Ctrl Pts',(0.488457130424633,-1.,-4.0073800839099));
#34432=CARTESIAN_POINT('Ctrl Pts',(0.492115383418018,-1.,-4.01411733503546));
#34433=CARTESIAN_POINT('Ctrl Pts',(0.495812444326251,-1.,-4.02084308851832));
#34434=CARTESIAN_POINT('Ctrl Pts',(0.499547962340821,-1.,-4.02755813980101));
#34435=CARTESIAN_POINT('Ctrl Pts',(0.503321556915346,-1.,-4.03426284174272));
#34436=CARTESIAN_POINT('Ctrl Pts',(0.507132823288136,-1.,-4.04095715148915));
#34437=CARTESIAN_POINT('Ctrl Pts',(0.51098134921897,-1.,-4.04764078815447));
#34438=CARTESIAN_POINT('Ctrl Pts',(0.514866728193016,-1.,-4.05431335771199));
#34439=CARTESIAN_POINT('Ctrl Pts',(0.518788572336923,-1.,-4.06097448038013));
#34440=CARTESIAN_POINT('Ctrl Pts',(0.522746528603107,-1.,-4.06762394471314));
#34441=CARTESIAN_POINT('Ctrl Pts',(0.526740277227498,-1.,-4.07426172299847));
#34442=CARTESIAN_POINT('Ctrl Pts',(0.53076951872857,-1.,-4.08088789536836));
#34443=CARTESIAN_POINT('Ctrl Pts',(0.534833963477273,-1.,-4.08750259988885));
#34444=CARTESIAN_POINT('Ctrl Pts',(0.538933321179755,-1.,-4.09410597627));
#34445=CARTESIAN_POINT('Ctrl Pts',(0.543067286877757,-1.,-4.10069810243979));
#34446=CARTESIAN_POINT('Ctrl Pts',(0.547235539485636,-1.,-4.10727897027977));
#34447=CARTESIAN_POINT('Ctrl Pts',(0.551437758497032,-1.,-4.11384852024721));
#34448=CARTESIAN_POINT('Ctrl Pts',(0.555673636129977,-1.,-4.12040666195664));
#34449=CARTESIAN_POINT('Ctrl Pts',(0.559942890594773,-1.,-4.12695329951961));
#34450=CARTESIAN_POINT('Ctrl Pts',(0.564245279537148,-1.,-4.13348835727104));
#34451=CARTESIAN_POINT('Ctrl Pts',(0.568580610189774,-1.,-4.14001179830547));
#34452=CARTESIAN_POINT('Ctrl Pts',(0.572948736069522,-1.,-4.14652361068081));
#34453=CARTESIAN_POINT('Ctrl Pts',(0.576469391676688,-1.,-4.151723761217));
#34454=CARTESIAN_POINT('Ctrl Pts',(0.579124568914235,-1.,-4.15561864788576));
#34455=CARTESIAN_POINT('Ctrl Pts',(0.580901211463535,-1.,-4.1582129171283));
#34456=CARTESIAN_POINT('Ctrl Pts',(0.581791163835815,-1.,-4.15950947128175));
#34457=CARTESIAN_POINT('',(0.73204283740062,-1.,-4.13571194405636));
#34458=CARTESIAN_POINT('',(0.581791163835815,-1.,-4.15950947128175));
#34459=CARTESIAN_POINT('',(0.786422660831985,-1.,-3.66661143271685));
#34460=CARTESIAN_POINT('Ctrl Pts',(0.73204283740062,-1.,-4.13571194405636));
#34461=CARTESIAN_POINT('Ctrl Pts',(0.732488575135159,-1.,-4.1342038373684));
#34462=CARTESIAN_POINT('Ctrl Pts',(0.733376589323546,-1.,-4.13118752795207));
#34463=CARTESIAN_POINT('Ctrl Pts',(0.734698226764092,-1.,-4.12666277570844));
#34464=CARTESIAN_POINT('Ctrl Pts',(0.736439634331344,-1.,-4.120629196238));
#34465=CARTESIAN_POINT('Ctrl Pts',(0.738581708225843,-1.,-4.11308626951927));
#34466=CARTESIAN_POINT('Ctrl Pts',(0.740688998553376,-1.,-4.10554241757547));
#34467=CARTESIAN_POINT('Ctrl Pts',(0.742761369689841,-1.,-4.09799769702611));
#34468=CARTESIAN_POINT('Ctrl Pts',(0.7447986497065,-1.,-4.09045220253573));
#34469=CARTESIAN_POINT('Ctrl Pts',(0.746800631492315,-1.,-4.08290608095642));
#34470=CARTESIAN_POINT('Ctrl Pts',(0.748767076680557,-1.,-4.07535951056152));
#34471=CARTESIAN_POINT('Ctrl Pts',(0.750697720484036,-1.,-4.06781267242378));
#34472=CARTESIAN_POINT('Ctrl Pts',(0.752592276483072,-1.,-4.06026572221515));
#34473=CARTESIAN_POINT('Ctrl Pts',(0.754450441816078,-1.,-4.05271876687915));
#34474=CARTESIAN_POINT('Ctrl Pts',(0.75627190236958,-1.,-4.04517182653997));
#34475=CARTESIAN_POINT('Ctrl Pts',(0.758056338884944,-1.,-4.03762485803119));
#34476=CARTESIAN_POINT('Ctrl Pts',(0.759803433243751,-1.,-4.03007781954412));
#34477=CARTESIAN_POINT('Ctrl Pts',(0.761512875859804,-1.,-4.02253072741268));
#34478=CARTESIAN_POINT('Ctrl Pts',(0.763184371182935,-1.,-4.01498370680496));
#34479=CARTESIAN_POINT('Ctrl Pts',(0.764817648785197,-1.,-4.00743706791509));
#34480=CARTESIAN_POINT('Ctrl Pts',(0.766412457136063,-1.,-3.99989129179622));
#34481=CARTESIAN_POINT('Ctrl Pts',(0.767968531377914,-1.,-3.9923468788101));
#34482=CARTESIAN_POINT('Ctrl Pts',(0.769485566245544,-1.,-3.98480422348451));
#34483=CARTESIAN_POINT('Ctrl Pts',(0.77096319003047,-1.,-3.97726349165488));
#34484=CARTESIAN_POINT('Ctrl Pts',(0.772400931772136,-1.,-3.96972446532772));
#34485=CARTESIAN_POINT('Ctrl Pts',(0.773798212026565,-1.,-3.96218649639807));
#34486=CARTESIAN_POINT('Ctrl Pts',(0.775154418039351,-1.,-3.9546488545231));
#34487=CARTESIAN_POINT('Ctrl Pts',(0.776468966697921,-1.,-3.94711101619447));
#34488=CARTESIAN_POINT('Ctrl Pts',(0.777741370568558,-1.,-3.93957296768103));
#34489=CARTESIAN_POINT('Ctrl Pts',(0.77897130813482,-1.,-3.93203552473174));
#34490=CARTESIAN_POINT('Ctrl Pts',(0.780158678615542,-1.,-3.92450058323823));
#34491=CARTESIAN_POINT('Ctrl Pts',(0.781303428618366,-1.,-3.91697036054676));
#34492=CARTESIAN_POINT('Ctrl Pts',(0.782405395622764,-1.,-3.90944671004542));
#34493=CARTESIAN_POINT('Ctrl Pts',(0.783464141529081,-1.,-3.9019303904397));
#34494=CARTESIAN_POINT('Ctrl Pts',(0.784478799358336,-1.,-3.89442039235103));
#34495=CARTESIAN_POINT('Ctrl Pts',(0.78544789034073,-1.,-3.88691313167398));
#34496=CARTESIAN_POINT('Ctrl Pts',(0.786369675812608,-1.,-3.8794040281819));
#34497=CARTESIAN_POINT('Ctrl Pts',(0.787242527617999,-1.,-3.87188916600912));
#34498=CARTESIAN_POINT('Ctrl Pts',(0.788065315093777,-1.,-3.86436702561345));
#34499=CARTESIAN_POINT('Ctrl Pts',(0.788837734090671,-1.,-3.85683995872529));
#34500=CARTESIAN_POINT('Ctrl Pts',(0.789560798155582,-1.,-3.84931637808894));
#34501=CARTESIAN_POINT('Ctrl Pts',(0.790236124191242,-1.,-3.84180762342454));
#34502=CARTESIAN_POINT('Ctrl Pts',(0.7908650127053,-1.,-3.83432392054786));
#34503=CARTESIAN_POINT('Ctrl Pts',(0.791447528662369,-1.,-3.82687033899792));
#34504=CARTESIAN_POINT('Ctrl Pts',(0.791981740718634,-1.,-3.81944345442249));
#34505=CARTESIAN_POINT('Ctrl Pts',(0.792462483517634,-1.,-3.81202588694756));
#34506=CARTESIAN_POINT('Ctrl Pts',(0.792882695234777,-1.,-3.80459229925637));
#34507=CARTESIAN_POINT('Ctrl Pts',(0.793235612973273,-1.,-3.79711921389897));
#34508=CARTESIAN_POINT('Ctrl Pts',(0.793516871680993,-1.,-3.78959439439235));
#34509=CARTESIAN_POINT('Ctrl Pts',(0.7937262357813,-1.,-3.78202460377598));
#34510=CARTESIAN_POINT('Ctrl Pts',(0.793870523787407,-1.,-3.77444863801212));
#34511=CARTESIAN_POINT('Ctrl Pts',(0.793961083688991,-1.,-3.76692626931111));
#34512=CARTESIAN_POINT('Ctrl Pts',(0.794008429134907,-1.,-3.75951468666257));
#34513=CARTESIAN_POINT('Ctrl Pts',(0.794017347371377,-1.,-3.75224692493864));
#34514=CARTESIAN_POINT('Ctrl Pts',(0.793982700459951,-1.,-3.74511357728861));
#34515=CARTESIAN_POINT('Ctrl Pts',(0.793882700937016,-1.,-3.73803280541687));
#34516=CARTESIAN_POINT('Ctrl Pts',(0.793682750269684,-1.,-3.73086914695805));
#34517=CARTESIAN_POINT('Ctrl Pts',(0.793347023784204,-1.,-3.72348797293734));
#34518=CARTESIAN_POINT('Ctrl Pts',(0.792848377370287,-1.,-3.71580242396124));
#34519=CARTESIAN_POINT('Ctrl Pts',(0.792177688845817,-1.,-3.70781724021806));
#34520=CARTESIAN_POINT('Ctrl Pts',(0.79135657569598,-1.,-3.69968940808721));
#34521=CARTESIAN_POINT('Ctrl Pts',(0.790436284988787,-1.,-3.69172044327364));
#34522=CARTESIAN_POINT('Ctrl Pts',(0.789483546064386,-1.,-3.68428439783905));
#34523=CARTESIAN_POINT('Ctrl Pts',(0.788569566220285,-1.,-3.67777119516252));
#34524=CARTESIAN_POINT('Ctrl Pts',(0.787758799995742,-1.,-3.67252923663655));
#34525=CARTESIAN_POINT('Ctrl Pts',(0.787145041181545,-1.,-3.66907505398677));
#34526=CARTESIAN_POINT('Ctrl Pts',(0.786774337198062,-1.,-3.66743103898702));
#34527=CARTESIAN_POINT('Ctrl Pts',(0.786565919558984,-1.,-3.66680946938292));
#34528=CARTESIAN_POINT('Ctrl Pts',(0.786459983895431,-1.,-3.6666431041522));
#34529=CARTESIAN_POINT('Ctrl Pts',(0.786422660831985,-1.,-3.66661143271685));
#34530=CARTESIAN_POINT('',(0.963899035117249,-1.,-3.62400312501245));
#34531=CARTESIAN_POINT('Origin',(0.,-1.,0.));
#34532=CARTESIAN_POINT('',(1.22531898815164,-1.,-4.01728681790024));
#34533=CARTESIAN_POINT('Ctrl Pts',(0.963899035117249,-1.,-3.62400312501245));
#34534=CARTESIAN_POINT('Ctrl Pts',(0.963880158555582,-1.,-3.6240482887845));
#34535=CARTESIAN_POINT('Ctrl Pts',(0.963861297423241,-1.,-3.62424461507588));
#34536=CARTESIAN_POINT('Ctrl Pts',(0.963957782642843,-1.,-3.62489305727662));
#34537=CARTESIAN_POINT('Ctrl Pts',(0.964373850166457,-1.,-3.62652618145335));
#34538=CARTESIAN_POINT('Ctrl Pts',(0.965395153165293,-1.,-3.62988252139846));
#34539=CARTESIAN_POINT('Ctrl Pts',(0.967052554541385,-1.,-3.63492122081143));
#34540=CARTESIAN_POINT('Ctrl Pts',(0.969195124675865,-1.,-3.64113946505766));
#34541=CARTESIAN_POINT('Ctrl Pts',(0.971722122061341,-1.,-3.64819756447455));
#34542=CARTESIAN_POINT('Ctrl Pts',(0.974519971354848,-1.,-3.65571576735126));
#34543=CARTESIAN_POINT('Ctrl Pts',(0.977478312751618,-1.,-3.66333049637475));
#34544=CARTESIAN_POINT('Ctrl Pts',(0.980505922458267,-1.,-3.67074983340361));
#34545=CARTESIAN_POINT('Ctrl Pts',(0.983550791470419,-1.,-3.67782408841715));
#34546=CARTESIAN_POINT('Ctrl Pts',(0.986602639863837,-1.,-3.68455317926068));
#34547=CARTESIAN_POINT('Ctrl Pts',(0.989676715398558,-1.,-3.69102682138847));
#34548=CARTESIAN_POINT('Ctrl Pts',(0.99280221833201,-1.,-3.69738123415662));
#34549=CARTESIAN_POINT('Ctrl Pts',(0.996009819772518,-1.,-3.70375282282138));
#34550=CARTESIAN_POINT('Ctrl Pts',(0.99931726075653,-1.,-3.71022439713938));
#34551=CARTESIAN_POINT('Ctrl Pts',(1.00272423396822,-1.,-3.71680667125119));
#34552=CARTESIAN_POINT('Ctrl Pts',(1.0062200073571,-1.,-3.72346803750596));
#34553=CARTESIAN_POINT('Ctrl Pts',(1.00978798539496,-1.,-3.73015276704426));
#34554=CARTESIAN_POINT('Ctrl Pts',(1.01341114319903,-1.,-3.73680245055734));
#34555=CARTESIAN_POINT('Ctrl Pts',(1.01707794311079,-1.,-3.74337942504959));
#34556=CARTESIAN_POINT('Ctrl Pts',(1.02078510487428,-1.,-3.74987777155834));
#34557=CARTESIAN_POINT('Ctrl Pts',(1.0245342944466,-1.,-3.75631037456194));
#34558=CARTESIAN_POINT('Ctrl Pts',(1.02833014458181,-1.,-3.76270122291232));
#34559=CARTESIAN_POINT('Ctrl Pts',(1.0321778660492,-1.,-3.76907609832522));
#34560=CARTESIAN_POINT('Ctrl Pts',(1.03608074678013,-1.,-3.77545283140445));
#34561=CARTESIAN_POINT('Ctrl Pts',(1.04003862055804,-1.,-3.78183535008192));
#34562=CARTESIAN_POINT('Ctrl Pts',(1.04404924374426,-1.,-3.78821910787195));
#34563=CARTESIAN_POINT('Ctrl Pts',(1.04810913267641,-1.,-3.79459440308793));
#34564=CARTESIAN_POINT('Ctrl Pts',(1.05221457990015,-1.,-3.80095039790678));
#34565=CARTESIAN_POINT('Ctrl Pts',(1.05636266918643,-1.,-3.80727913637784));
#34566=CARTESIAN_POINT('Ctrl Pts',(1.06055206187298,-1.,-3.81357866117485));
#34567=CARTESIAN_POINT('Ctrl Pts',(1.06478244038931,-1.,-3.81985083953012));
#34568=CARTESIAN_POINT('Ctrl Pts',(1.0690541318036,-1.,-3.82609989967278));
#34569=CARTESIAN_POINT('Ctrl Pts',(1.0733676663346,-1.,-3.83233071195145));
#34570=CARTESIAN_POINT('Ctrl Pts',(1.07772335353856,-1.,-3.83854714117486));
#34571=CARTESIAN_POINT('Ctrl Pts',(1.08212087917986,-1.,-3.84475048030615));
#34572=CARTESIAN_POINT('Ctrl Pts',(1.08655950846377,-1.,-3.85094025222691));
#34573=CARTESIAN_POINT('Ctrl Pts',(1.09103825516288,-1.,-3.85711487933911));
#34574=CARTESIAN_POINT('Ctrl Pts',(1.09555606505012,-1.,-3.86327241021242));
#34575=CARTESIAN_POINT('Ctrl Pts',(1.10011198761202,-1.,-3.86941120134872));
#34576=CARTESIAN_POINT('Ctrl Pts',(1.10470536603303,-1.,-3.87553067187566));
#34577=CARTESIAN_POINT('Ctrl Pts',(1.10933577224029,-1.,-3.88163105531791));
#34578=CARTESIAN_POINT('Ctrl Pts',(1.11400292434447,-1.,-3.88771308285229));
#34579=CARTESIAN_POINT('Ctrl Pts',(1.11870660794609,-1.,-3.89377768340362));
#34580=CARTESIAN_POINT('Ctrl Pts',(1.12344660099029,-1.,-3.89982569749978));
#34581=CARTESIAN_POINT('Ctrl Pts',(1.12822258281518,-1.,-3.90585753318622));
#34582=CARTESIAN_POINT('Ctrl Pts',(1.13303414693849,-1.,-3.91187321145495));
#34583=CARTESIAN_POINT('Ctrl Pts',(1.13788084225511,-1.,-3.91787251936688));
#34584=CARTESIAN_POINT('Ctrl Pts',(1.14276220561575,-1.,-3.92385513133937));
#34585=CARTESIAN_POINT('Ctrl Pts',(1.14767779451147,-1.,-3.92982073294334));
#34586=CARTESIAN_POINT('Ctrl Pts',(1.1526272271639,-1.,-3.9357691705651));
#34587=CARTESIAN_POINT('Ctrl Pts',(1.1576101834106,-1.,-3.94170046685542));
#34588=CARTESIAN_POINT('Ctrl Pts',(1.16262637999261,-1.,-3.9476147478092));
#34589=CARTESIAN_POINT('Ctrl Pts',(1.16767555244495,-1.,-3.95351219510062));
#34590=CARTESIAN_POINT('Ctrl Pts',(1.17275743590327,-1.,-3.95939299213164));
#34591=CARTESIAN_POINT('Ctrl Pts',(1.17787174135445,-1.,-3.96525726357682));
#34592=CARTESIAN_POINT('Ctrl Pts',(1.18301815039596,-1.,-3.9711050516465));
#34593=CARTESIAN_POINT('Ctrl Pts',(1.18819633715285,-1.,-3.97693634766926));
#34594=CARTESIAN_POINT('Ctrl Pts',(1.19340598349307,-1.,-3.98275111052015));
#34595=CARTESIAN_POINT('Ctrl Pts',(1.19864679609596,-1.,-3.98854928957287));
#34596=CARTESIAN_POINT('Ctrl Pts',(1.2039185237544,-1.,-3.99433084800649));
#34597=CARTESIAN_POINT('Ctrl Pts',(1.20922097030107,-1.,-4.00009577952534));
#34598=CARTESIAN_POINT('Ctrl Pts',(1.21455398918813,-1.,-4.00584409524937));
#34599=CARTESIAN_POINT('Ctrl Pts',(1.21884478244983,-1.,-4.01042947142681));
#34600=CARTESIAN_POINT('Ctrl Pts',(1.22207656456199,-1.,-4.01386104434674));
#34601=CARTESIAN_POINT('Ctrl Pts',(1.22423716681447,-1.,-4.0161454457032));
#34602=CARTESIAN_POINT('Ctrl Pts',(1.22531898815164,-1.,-4.01728681790024));
#34603=CARTESIAN_POINT('',(1.36999806084572,-1.,-3.97027773754922));
#34604=CARTESIAN_POINT('',(1.22531898815164,-1.,-4.01728681790024));
#34605=CARTESIAN_POINT('',(1.35032489087101,-1.,-3.4984457533445));
#34606=CARTESIAN_POINT('Ctrl Pts',(1.36999806084572,-1.,-3.97027773754922));
#34607=CARTESIAN_POINT('Ctrl Pts',(1.37020239094614,-1.,-3.9687184694131));
#34608=CARTESIAN_POINT('Ctrl Pts',(1.37060761745635,-1.,-3.96560037974645));
#34609=CARTESIAN_POINT('Ctrl Pts',(1.3712051561502,-1.,-3.96092458506535));
#34610=CARTESIAN_POINT('Ctrl Pts',(1.37198126432386,-1.,-3.95469287280914));
#34611=CARTESIAN_POINT('Ctrl Pts',(1.37291699202807,-1.,-3.94690771785133));
#34612=CARTESIAN_POINT('Ctrl Pts',(1.37381821967165,-1.,-3.93912709040818));
#34613=CARTESIAN_POINT('Ctrl Pts',(1.37468482215751,-1.,-3.93135106761844));
#34614=CARTESIAN_POINT('Ctrl Pts',(1.37551664448242,-1.,-3.92357976987672));
#34615=CARTESIAN_POINT('Ctrl Pts',(1.37631350505797,-1.,-3.91581337462644));
#34616=CARTESIAN_POINT('Ctrl Pts',(1.3770751963402,-1.,-3.90805209523486));
#34617=CARTESIAN_POINT('Ctrl Pts',(1.37780148512792,-1.,-3.90029615196727));
#34618=CARTESIAN_POINT('Ctrl Pts',(1.3784921128802,-1.,-3.89254574338496));
#34619=CARTESIAN_POINT('Ctrl Pts',(1.37914679719383,-1.,-3.88480102249278));
#34620=CARTESIAN_POINT('Ctrl Pts',(1.37976523097073,-1.,-3.87706205830532));
#34621=CARTESIAN_POINT('Ctrl Pts',(1.38034709213014,-1.,-3.86932885813068));
#34622=CARTESIAN_POINT('Ctrl Pts',(1.38089205992989,-1.,-3.86160143043959));
#34623=CARTESIAN_POINT('Ctrl Pts',(1.38139983115049,-1.,-3.85387983979481));
#34624=CARTESIAN_POINT('Ctrl Pts',(1.38187013346109,-1.,-3.84616425605764));
#34625=CARTESIAN_POINT('Ctrl Pts',(1.38230274828821,-1.,-3.83845502790746));
#34626=CARTESIAN_POINT('Ctrl Pts',(1.38269750245138,-1.,-3.8307526698229));
#34627=CARTESIAN_POINT('Ctrl Pts',(1.38305421262763,-1.,-3.82305771743829));
#34628=CARTESIAN_POINT('Ctrl Pts',(1.38337263902782,-1.,-3.81537060817811));
#34629=CARTESIAN_POINT('Ctrl Pts',(1.3836524404622,-1.,-3.80769156398411));
#34630=CARTESIAN_POINT('Ctrl Pts',(1.38389311766682,-1.,-3.80002044322111));
#34631=CARTESIAN_POINT('Ctrl Pts',(1.38409399694566,-1.,-3.79235669640841));
#34632=CARTESIAN_POINT('Ctrl Pts',(1.38425435883756,-1.,-3.78469969805082));
#34633=CARTESIAN_POINT('Ctrl Pts',(1.38437354551428,-1.,-3.77704902230418));
#34634=CARTESIAN_POINT('Ctrl Pts',(1.38445107339518,-1.,-3.76940473185779));
#34635=CARTESIAN_POINT('Ctrl Pts',(1.3844867525335,-1.,-3.76176768271367));
#34636=CARTESIAN_POINT('Ctrl Pts',(1.38448077997163,-1.,-3.7541397631875));
#34637=CARTESIAN_POINT('Ctrl Pts',(1.38443344984394,-1.,-3.74652317167876));
#34638=CARTESIAN_POINT('Ctrl Pts',(1.38434489156458,-1.,-3.73891976418104));
#34639=CARTESIAN_POINT('Ctrl Pts',(1.38421479111531,-1.,-3.73133035859282));
#34640=CARTESIAN_POINT('Ctrl Pts',(1.3840421342895,-1.,-3.72375409358803));
#34641=CARTESIAN_POINT('Ctrl Pts',(1.38382489984586,-1.,-3.7161876605181));
#34642=CARTESIAN_POINT('Ctrl Pts',(1.38356065402124,-1.,-3.70862680753347));
#34643=CARTESIAN_POINT('Ctrl Pts',(1.38324717612865,-1.,-3.701067921679));
#34644=CARTESIAN_POINT('Ctrl Pts',(1.3828831117165,-1.,-3.69350967899526));
#34645=CARTESIAN_POINT('Ctrl Pts',(1.38246852827182,-1.,-3.68595444983838));
#34646=CARTESIAN_POINT('Ctrl Pts',(1.3820057429062,-1.,-3.67841038482414));
#34647=CARTESIAN_POINT('Ctrl Pts',(1.38149812653868,-1.,-3.67088843112262));
#34648=CARTESIAN_POINT('Ctrl Pts',(1.38094856333552,-1.,-3.66339848520857));
#34649=CARTESIAN_POINT('Ctrl Pts',(1.38035791051212,-1.,-3.6559455440439));
#34650=CARTESIAN_POINT('Ctrl Pts',(1.37972372481603,-1.,-3.64852652756456));
#34651=CARTESIAN_POINT('Ctrl Pts',(1.37903818567359,-1.,-3.64112507791141));
#34652=CARTESIAN_POINT('Ctrl Pts',(1.37829035457339,-1.,-3.63371727442486));
#34653=CARTESIAN_POINT('Ctrl Pts',(1.37746987919881,-1.,-3.62628098665145));
#34654=CARTESIAN_POINT('Ctrl Pts',(1.37657053403107,-1.,-3.61880481160421));
#34655=CARTESIAN_POINT('Ctrl Pts',(1.37559314436634,-1.,-3.61129546591064));
#34656=CARTESIAN_POINT('Ctrl Pts',(1.37455051379623,-1.,-3.60379020123988));
#34657=CARTESIAN_POINT('Ctrl Pts',(1.37346320103157,-1.,-3.59634627869048));
#34658=CARTESIAN_POINT('Ctrl Pts',(1.37235053660976,-1.,-3.58901853846365));
#34659=CARTESIAN_POINT('Ctrl Pts',(1.37122241663062,-1.,-3.58183885982715));
#34660=CARTESIAN_POINT('Ctrl Pts',(1.37007229485659,-1.,-3.57479875549486));
#34661=CARTESIAN_POINT('Ctrl Pts',(1.36886584973389,-1.,-3.5678208030466));
#34662=CARTESIAN_POINT('Ctrl Pts',(1.36754771771233,-1.,-3.56077662028649));
#34663=CARTESIAN_POINT('Ctrl Pts',(1.3660614545677,-1.,-3.55353883995949));
#34664=CARTESIAN_POINT('Ctrl Pts',(1.36436666257597,-1.,-3.54602591832973));
#34665=CARTESIAN_POINT('Ctrl Pts',(1.36245507339307,-1.,-3.53824396424961));
#34666=CARTESIAN_POINT('Ctrl Pts',(1.36037259643734,-1.,-3.530344649616));
#34667=CARTESIAN_POINT('Ctrl Pts',(1.35821701528836,-1.,-3.52261776116748));
#34668=CARTESIAN_POINT('Ctrl Pts',(1.35611275237152,-1.,-3.51542230699556));
#34669=CARTESIAN_POINT('Ctrl Pts',(1.35419113575956,-1.,-3.50913227059999));
#34670=CARTESIAN_POINT('Ctrl Pts',(1.35257032843486,-1.,-3.50408168106261));
#34671=CARTESIAN_POINT('Ctrl Pts',(1.35142377279517,-1.,-3.5007660381649));
#34672=CARTESIAN_POINT('Ctrl Pts',(1.35080045218586,-1.,-3.49920025459723));
#34673=CARTESIAN_POINT('Ctrl Pts',(1.35049736560527,-1.,-3.49861894124827));
#34674=CARTESIAN_POINT('Ctrl Pts',(1.35036670892966,-1.,-3.49847119623846));
#34675=CARTESIAN_POINT('Ctrl Pts',(1.35032489087101,-1.,-3.4984457533445));
#34676=CARTESIAN_POINT('',(1.51895082866166,-1.,-3.42859860294378));
#34677=CARTESIAN_POINT('Origin',(0.,-1.,0.));
#34678=CARTESIAN_POINT('',(1.83867539237861,-1.,-3.77614523045147));
#34679=CARTESIAN_POINT('Ctrl Pts',(1.51895082866166,-1.,-3.42859860294378));
#34680=CARTESIAN_POINT('Ctrl Pts',(1.51893924967231,-1.,-3.42864616361967));
#34681=CARTESIAN_POINT('Ctrl Pts',(1.51895133295017,-1.,-3.42884302333978));
#34682=CARTESIAN_POINT('Ctrl Pts',(1.51914806898539,-1.,-3.42946838852728));
#34683=CARTESIAN_POINT('Ctrl Pts',(1.5198144909343,-1.,-3.43101631893491));
#34684=CARTESIAN_POINT('Ctrl Pts',(1.52134826724227,-1.,-3.43417156977749));
#34685=CARTESIAN_POINT('Ctrl Pts',(1.52377348950429,-1.,-3.43888895974182));
#34686=CARTESIAN_POINT('Ctrl Pts',(1.52686242875717,-1.,-3.44469547527));
#34687=CARTESIAN_POINT('Ctrl Pts',(1.530462444618,-1.,-3.45127136828667));
#34688=CARTESIAN_POINT('Ctrl Pts',(1.53440195378902,-1.,-3.45825932955273));
#34689=CARTESIAN_POINT('Ctrl Pts',(1.53851507915533,-1.,-3.46531752207222));
#34690=CARTESIAN_POINT('Ctrl Pts',(1.54266605398152,-1.,-3.47217189224576));
#34691=CARTESIAN_POINT('Ctrl Pts',(1.54678009290206,-1.,-3.47868272898599));
#34692=CARTESIAN_POINT('Ctrl Pts',(1.55084702970382,-1.,-3.48485155928414));
#34693=CARTESIAN_POINT('Ctrl Pts',(1.5548959590107,-1.,-3.49076460877317));
#34694=CARTESIAN_POINT('Ctrl Pts',(1.55897703097859,-1.,-3.49655185179623));
#34695=CARTESIAN_POINT('Ctrl Pts',(1.56314187758689,-1.,-3.50234321621607));
#34696=CARTESIAN_POINT('Ctrl Pts',(1.56742097575041,-1.,-3.50821771695427));
#34697=CARTESIAN_POINT('Ctrl Pts',(1.57181569799774,-1.,-3.51418598431733));
#34698=CARTESIAN_POINT('Ctrl Pts',(1.5763104998818,-1.,-3.52021847865961));
#34699=CARTESIAN_POINT('Ctrl Pts',(1.58088027227856,-1.,-3.52626275334899));
#34700=CARTESIAN_POINT('Ctrl Pts',(1.58549906268083,-1.,-3.53226378147068));
#34701=CARTESIAN_POINT('Ctrl Pts',(1.59014958368725,-1.,-3.53818616861045));
#34702=CARTESIAN_POINT('Ctrl Pts',(1.5948276694975,-1.,-3.544024581823));
#34703=CARTESIAN_POINT('Ctrl Pts',(1.59953698113444,-1.,-3.54979148634426));
#34704=CARTESIAN_POINT('Ctrl Pts',(1.60428584699848,-1.,-3.55550985096117));
#34705=CARTESIAN_POINT('Ctrl Pts',(1.60908344685459,-1.,-3.56120432482986));
#34706=CARTESIAN_POINT('Ctrl Pts',(1.61393581747522,-1.,-3.56689200468404));
#34707=CARTESIAN_POINT('Ctrl Pts',(1.61884340915412,-1.,-3.57257679609826));
#34708=CARTESIAN_POINT('Ctrl Pts',(1.62380329464851,-1.,-3.57825455954405));
#34709=CARTESIAN_POINT('Ctrl Pts',(1.62881051550748,-1.,-3.5839162577435));
#34710=CARTESIAN_POINT('Ctrl Pts',(1.63385971451259,-1.,-3.58955176627876));
#34711=CARTESIAN_POINT('Ctrl Pts',(1.63894676675349,-1.,-3.59515368334887));
#34712=CARTESIAN_POINT('Ctrl Pts',(1.6440700438558,-1.,-3.6007202851384));
#34713=CARTESIAN_POINT('Ctrl Pts',(1.64922952425833,-1.,-3.60625346556992));
#34714=CARTESIAN_POINT('Ctrl Pts',(1.65442619244327,-1.,-3.61175734965129));
#34715=CARTESIAN_POINT('Ctrl Pts',(1.65966133399186,-1.,-3.61723666482457));
#34716=CARTESIAN_POINT('Ctrl Pts',(1.66493585923853,-1.,-3.62269517989104));
#34717=CARTESIAN_POINT('Ctrl Pts',(1.67024966008037,-1.,-3.62813422105257));
#34718=CARTESIAN_POINT('Ctrl Pts',(1.67560193613145,-1.,-3.63355343201211));
#34719=CARTESIAN_POINT('Ctrl Pts',(1.68099146651577,-1.,-3.63895140887443));
#34720=CARTESIAN_POINT('Ctrl Pts',(1.68641690471455,-1.,-3.64432638915199));
#34721=CARTESIAN_POINT('Ctrl Pts',(1.691877054817,-1.,-3.64967689827393));
#34722=CARTESIAN_POINT('Ctrl Pts',(1.69737117722558,-1.,-3.65500246526798));
#34723=CARTESIAN_POINT('Ctrl Pts',(1.70289888566904,-1.,-3.6603033877491));
#34724=CARTESIAN_POINT('Ctrl Pts',(1.70846001610983,-1.,-3.6655804319893));
#34725=CARTESIAN_POINT('Ctrl Pts',(1.71405450210392,-1.,-3.67083454901629));
#34726=CARTESIAN_POINT('Ctrl Pts',(1.71968225581787,-1.,-3.67606660374665));
#34727=CARTESIAN_POINT('Ctrl Pts',(1.72534302437003,-1.,-3.68127704936472));
#34728=CARTESIAN_POINT('Ctrl Pts',(1.73103640956647,-1.,-3.68646597019188));
#34729=CARTESIAN_POINT('Ctrl Pts',(1.73676193254493,-1.,-3.69163322647906));
#34730=CARTESIAN_POINT('Ctrl Pts',(1.74251908492589,-1.,-3.6967785691046));
#34731=CARTESIAN_POINT('Ctrl Pts',(1.74830738046092,-1.,-3.70190175673422));
#34732=CARTESIAN_POINT('Ctrl Pts',(1.75412641804148,-1.,-3.70700269736876));
#34733=CARTESIAN_POINT('Ctrl Pts',(1.75997588499021,-1.,-3.71208146346455));
#34734=CARTESIAN_POINT('Ctrl Pts',(1.76585552124549,-1.,-3.71713822377676));
#34735=CARTESIAN_POINT('Ctrl Pts',(1.77176509401846,-1.,-3.72217319911429));
#34736=CARTESIAN_POINT('Ctrl Pts',(1.77770437039606,-1.,-3.72718661205504));
#34737=CARTESIAN_POINT('Ctrl Pts',(1.78367308442682,-1.,-3.73217863095022));
#34738=CARTESIAN_POINT('Ctrl Pts',(1.78967092823139,-1.,-3.73714934729962));
#34739=CARTESIAN_POINT('Ctrl Pts',(1.79569757859041,-1.,-3.74209880351667));
#34740=CARTESIAN_POINT('Ctrl Pts',(1.80175271485519,-1.,-3.74702700874954));
#34741=CARTESIAN_POINT('Ctrl Pts',(1.80783603939662,-1.,-3.75193395888069));
#34742=CARTESIAN_POINT('Ctrl Pts',(1.81394729834032,-1.,-3.75681965683995));
#34743=CARTESIAN_POINT('Ctrl Pts',(1.82008629694924,-1.,-3.76168412709652));
#34744=CARTESIAN_POINT('Ctrl Pts',(1.82625289221933,-1.,-3.76652740355856));
#34745=CARTESIAN_POINT('Ctrl Pts',(1.83120816956515,-1.,-3.77038509819777));
#34746=CARTESIAN_POINT('Ctrl Pts',(1.83493697935064,-1.,-3.77326886065484));
#34747=CARTESIAN_POINT('Ctrl Pts',(1.83742834010821,-1.,-3.77518714458232));
#34748=CARTESIAN_POINT('Ctrl Pts',(1.83867539237861,-1.,-3.77614523045147));
#34749=CARTESIAN_POINT('',(1.97421938526992,-1.,-3.70708211654725));
#34750=CARTESIAN_POINT('',(1.83867539237861,-1.,-3.77614523045147));
#34751=CARTESIAN_POINT('',(1.88097764062541,-1.,-3.24413672884902));
#34752=CARTESIAN_POINT('Ctrl Pts',(1.97421938526992,-1.,-3.70708211654725));
#34753=CARTESIAN_POINT('Ctrl Pts',(1.974177276451,-1.,-3.7055100813194));
#34754=CARTESIAN_POINT('Ctrl Pts',(1.97408973726149,-1.,-3.70236698911837));
#34755=CARTESIAN_POINT('Ctrl Pts',(1.97394846382288,-1.,-3.69765528558292));
#34756=CARTESIAN_POINT('Ctrl Pts',(1.97374016224397,-1.,-3.69137888597855));
#34757=CARTESIAN_POINT('Ctrl Pts',(1.9734465030363,-1.,-3.68354319913416));
#34758=CARTESIAN_POINT('Ctrl Pts',(1.97311947678035,-1.,-3.67571738106175));
#34759=CARTESIAN_POINT('Ctrl Pts',(1.9727589719863,-1.,-3.66790152751984));
#34760=CARTESIAN_POINT('Ctrl Pts',(1.97236485439317,-1.,-3.66009578166865));
#34761=CARTESIAN_POINT('Ctrl Pts',(1.97193697240645,-1.,-3.65230034717364));
#34762=CARTESIAN_POINT('Ctrl Pts',(1.97147515441539,-1.,-3.64451546724222));
#34763=CARTESIAN_POINT('Ctrl Pts',(1.97097920454698,-1.,-3.63674139590853));
#34764=CARTESIAN_POINT('Ctrl Pts',(1.97044889850518,-1.,-3.62897836973397));
#34765=CARTESIAN_POINT('Ctrl Pts',(1.96988398129888,-1.,-3.62122658401722));
#34766=CARTESIAN_POINT('Ctrl Pts',(1.96928416040712,-1.,-3.61348615496393));
#34767=CARTESIAN_POINT('Ctrl Pts',(1.96864911885775,-1.,-3.60575714017676));
#34768=CARTESIAN_POINT('Ctrl Pts',(1.96797854118257,-1.,-3.59803959819725));
#34769=CARTESIAN_POINT('Ctrl Pts',(1.96727213799507,-1.,-3.5903336402273));
#34770=CARTESIAN_POINT('Ctrl Pts',(1.9665296668894,-1.,-3.58263947663884));
#34771=CARTESIAN_POINT('Ctrl Pts',(1.96575096652857,-1.,-3.57495748601088));
#34772=CARTESIAN_POINT('Ctrl Pts',(1.96493594634643,-1.,-3.56728820357933));
#34773=CARTESIAN_POINT('Ctrl Pts',(1.96408450906868,-1.,-3.55963218706201));
#34774=CARTESIAN_POINT('Ctrl Pts',(1.96319648628667,-1.,-3.55198990600929));
#34775=CARTESIAN_POINT('Ctrl Pts',(1.96227157573058,-1.,-3.54436163300425));
#34776=CARTESIAN_POINT('Ctrl Pts',(1.96130926212661,-1.,-3.53674730625759));
#34777=CARTESIAN_POINT('Ctrl Pts',(1.96030879411534,-1.,-3.52914648844289));
#34778=CARTESIAN_POINT('Ctrl Pts',(1.95926936324436,-1.,-3.52155867431438));
#34779=CARTESIAN_POINT('Ctrl Pts',(1.95819025316768,-1.,-3.51398354617773));
#34780=CARTESIAN_POINT('Ctrl Pts',(1.95707099606513,-1.,-3.50642124159913));
#34781=CARTESIAN_POINT('Ctrl Pts',(1.9559115382367,-1.,-3.49887263575602));
#34782=CARTESIAN_POINT('Ctrl Pts',(1.95471236969653,-1.,-3.49133956289154));
#34783=CARTESIAN_POINT('Ctrl Pts',(1.95347412486316,-1.,-3.48382414832649));
#34784=CARTESIAN_POINT('Ctrl Pts',(1.95219722189878,-1.,-3.47632820495926));
#34785=CARTESIAN_POINT('Ctrl Pts',(1.95088147859876,-1.,-3.4688525897419));
#34786=CARTESIAN_POINT('Ctrl Pts',(1.94952575850196,-1.,-3.46139661060959));
#34787=CARTESIAN_POINT('Ctrl Pts',(1.94812754766524,-1.,-3.45395731584051));
#34788=CARTESIAN_POINT('Ctrl Pts',(1.94668377715332,-1.,-3.44653088665685));
#34789=CARTESIAN_POINT('Ctrl Pts',(1.94519168842883,-1.,-3.43911410197693));
#34790=CARTESIAN_POINT('Ctrl Pts',(1.94364973660285,-1.,-3.43170586602436));
#34791=CARTESIAN_POINT('Ctrl Pts',(1.94205835913692,-1.,-3.42430850941497));
#34792=CARTESIAN_POINT('Ctrl Pts',(1.94042111965237,-1.,-3.41692971994082));
#34793=CARTESIAN_POINT('Ctrl Pts',(1.93874306008132,-1.,-3.40957978266623));
#34794=CARTESIAN_POINT('Ctrl Pts',(1.93702857723089,-1.,-3.40226802104093));
#34795=CARTESIAN_POINT('Ctrl Pts',(1.93527929945982,-1.,-3.39499923640789));
#34796=CARTESIAN_POINT('Ctrl Pts',(1.93349233176794,-1.,-3.38777076883267));
#34797=CARTESIAN_POINT('Ctrl Pts',(1.93165739093292,-1.,-3.38056768525577));
#34798=CARTESIAN_POINT('Ctrl Pts',(1.92975993109897,-1.,-3.37336807068078));
#34799=CARTESIAN_POINT('Ctrl Pts',(1.92778626543803,-1.,-3.36615168657597));
#34800=CARTESIAN_POINT('Ctrl Pts',(1.92572846125763,-1.,-3.35890824422976));
#34801=CARTESIAN_POINT('Ctrl Pts',(1.92358838440518,-1.,-3.35164424847207));
#34802=CARTESIAN_POINT('Ctrl Pts',(1.92138450828378,-1.,-3.34439448941915));
#34803=CARTESIAN_POINT('Ctrl Pts',(1.91914609610173,-1.,-3.33721230709948));
#34804=CARTESIAN_POINT('Ctrl Pts',(1.91690081930297,-1.,-3.33014884257812));
#34805=CARTESIAN_POINT('Ctrl Pts',(1.91466343916612,-1.,-3.32323403454507));
#34806=CARTESIAN_POINT('Ctrl Pts',(1.91242616234459,-1.,-3.31646052426395));
#34807=CARTESIAN_POINT('Ctrl Pts',(1.91014297830502,-1.,-3.30975721158694));
#34808=CARTESIAN_POINT('Ctrl Pts',(1.90773912171424,-1.,-3.30300595568341));
#34809=CARTESIAN_POINT('Ctrl Pts',(1.9051389186417,-1.,-3.29608978722258));
#34810=CARTESIAN_POINT('Ctrl Pts',(1.9022897124757,-1.,-3.28893448600364));
#34811=CARTESIAN_POINT('Ctrl Pts',(1.89918429230424,-1.,-3.28154737912287));
#34812=CARTESIAN_POINT('Ctrl Pts',(1.89589172903662,-1.,-3.27407108932908));
#34813=CARTESIAN_POINT('Ctrl Pts',(1.89255393500769,-1.,-3.2667765388833));
#34814=CARTESIAN_POINT('Ctrl Pts',(1.88934996203508,-1.,-3.2599988519361));
#34815=CARTESIAN_POINT('Ctrl Pts',(1.88646802523372,-1.,-3.25408686339298));
#34816=CARTESIAN_POINT('Ctrl Pts',(1.88407708646435,-1.,-3.24935200512055));
#34817=CARTESIAN_POINT('Ctrl Pts',(1.88242596600422,-1.,-3.24625654410705));
#34818=CARTESIAN_POINT('Ctrl Pts',(1.88156537699118,-1.,-3.24480754675942));
#34819=CARTESIAN_POINT('Ctrl Pts',(1.88117508446657,-1.,-3.24428080352952));
#34820=CARTESIAN_POINT('Ctrl Pts',(1.88102292397987,-1.,-3.24415531671311));
#34821=CARTESIAN_POINT('Ctrl Pts',(1.88097764062541,-1.,-3.24413672884902));
#34822=CARTESIAN_POINT('',(2.03660101169564,-1.,-3.14877060440425));
#34823=CARTESIAN_POINT('Origin',(0.,-1.,0.));
#34824=CARTESIAN_POINT('',(2.40675750623143,-1.,-3.44202241512147));
#34825=CARTESIAN_POINT('Ctrl Pts',(2.03660101169564,-1.,-3.14877060440425));
#34826=CARTESIAN_POINT('Ctrl Pts',(2.03659701539175,-1.,-3.1488193908823));
#34827=CARTESIAN_POINT('Ctrl Pts',(2.03663974554941,-1.,-3.14901193669147));
#34828=CARTESIAN_POINT('Ctrl Pts',(2.03693188810614,-1.,-3.14959882629936));
#34829=CARTESIAN_POINT('Ctrl Pts',(2.03783225496023,-1.,-3.15102344775396));
#34830=CARTESIAN_POINT('Ctrl Pts',(2.03984073791432,-1.,-3.1538999167466));
#34831=CARTESIAN_POINT('Ctrl Pts',(2.04297406404132,-1.,-3.15817983946525));
#34832=CARTESIAN_POINT('Ctrl Pts',(2.0469333124766,-1.,-3.16343165059235));
#34833=CARTESIAN_POINT('Ctrl Pts',(2.05151770247452,-1.,-3.16936341689859));
#34834=CARTESIAN_POINT('Ctrl Pts',(2.05650186773279,-1.,-3.17564906975592));
#34835=CARTESIAN_POINT('Ctrl Pts',(2.06166849827143,-1.,-3.18197692964677));
#34836=CARTESIAN_POINT('Ctrl Pts',(2.06684062744065,-1.,-3.18809755562297));
#34837=CARTESIAN_POINT('Ctrl Pts',(2.07192253497765,-1.,-3.19388465568113));
#34838=CARTESIAN_POINT('Ctrl Pts',(2.0769044187063,-1.,-3.19934132835879));
#34839=CARTESIAN_POINT('Ctrl Pts',(2.08182850370816,-1.,-3.20454818630635));
#34840=CARTESIAN_POINT('Ctrl Pts',(2.08676465517435,-1.,-3.20962575845433));
#34841=CARTESIAN_POINT('Ctrl Pts',(2.0917841946046,-1.,-3.2146942960168));
#34842=CARTESIAN_POINT('Ctrl Pts',(2.09692958434933,-1.,-3.21982707347067));
#34843=CARTESIAN_POINT('Ctrl Pts',(2.10220384298533,-1.,-3.22503437553496));
#34844=CARTESIAN_POINT('Ctrl Pts',(2.1075869964248,-1.,-3.23028945793334));
#34845=CARTESIAN_POINT('Ctrl Pts',(2.11304604021784,-1.,-3.23554444767115));
#34846=CARTESIAN_POINT('Ctrl Pts',(2.11854673326972,-1.,-3.24074905517282));
#34847=CARTESIAN_POINT('Ctrl Pts',(2.12406646410943,-1.,-3.24587102613347));
#34848=CARTESIAN_POINT('Ctrl Pts',(2.1296002839681,-1.,-3.25090574493994));
#34849=CARTESIAN_POINT('Ctrl Pts',(2.13515375878786,-1.,-3.25586495065027));
#34850=CARTESIAN_POINT('Ctrl Pts',(2.14073870754257,-1.,-3.26077002641868));
#34851=CARTESIAN_POINT('Ctrl Pts',(2.14636805295663,-1.,-3.26564388189764));
#34852=CARTESIAN_POINT('Ctrl Pts',(2.15205043199818,-1.,-3.27050245897244));
#34853=CARTESIAN_POINT('Ctrl Pts',(2.15778690038359,-1.,-3.27534954469206));
#34854=CARTESIAN_POINT('Ctrl Pts',(2.16357391934434,-1.,-3.28018150841414));
#34855=CARTESIAN_POINT('Ctrl Pts',(2.16940517773459,-1.,-3.2849901997973));
#34856=CARTESIAN_POINT('Ctrl Pts',(2.17527380048422,-1.,-3.28976645712566));
#34857=CARTESIAN_POINT('Ctrl Pts',(2.18117455557062,-1.,-3.29450361500484));
#34858=CARTESIAN_POINT('Ctrl Pts',(2.18710556500325,-1.,-3.29920022557635));
#34859=CARTESIAN_POINT('Ctrl Pts',(2.19306710376112,-1.,-3.30385816281831));
#34860=CARTESIAN_POINT('Ctrl Pts',(2.19906078949924,-1.,-3.30848134694597));
#34861=CARTESIAN_POINT('Ctrl Pts',(2.20508863150608,-1.,-3.3130742460895));
#34862=CARTESIAN_POINT('Ctrl Pts',(2.21115211847872,-1.,-3.31764044024231));
#34863=CARTESIAN_POINT('Ctrl Pts',(2.21725135110889,-1.,-3.32218125618955));
#34864=CARTESIAN_POINT('Ctrl Pts',(2.22338548312758,-1.,-3.32669646722871));
#34865=CARTESIAN_POINT('Ctrl Pts',(2.22955308907221,-1.,-3.33118487773593));
#34866=CARTESIAN_POINT('Ctrl Pts',(2.23575256328809,-1.,-3.33564495756478));
#34867=CARTESIAN_POINT('Ctrl Pts',(2.24198249391437,-1.,-3.34007543738044));
#34868=CARTESIAN_POINT('Ctrl Pts',(2.24824207678287,-1.,-3.34447596770768));
#34869=CARTESIAN_POINT('Ctrl Pts',(2.25453097693524,-1.,-3.34884690292342));
#34870=CARTESIAN_POINT('Ctrl Pts',(2.26084915222484,-1.,-3.35318902552676));
#34871=CARTESIAN_POINT('Ctrl Pts',(2.26719668579921,-1.,-3.35750328523077));
#34872=CARTESIAN_POINT('Ctrl Pts',(2.27357362620902,-1.,-3.36179055004369));
#34873=CARTESIAN_POINT('Ctrl Pts',(2.27997979457968,-1.,-3.36605130712978));
#34874=CARTESIAN_POINT('Ctrl Pts',(2.28641481081045,-1.,-3.37028570206357));
#34875=CARTESIAN_POINT('Ctrl Pts',(2.2928781800731,-1.,-3.37449367172707));
#34876=CARTESIAN_POINT('Ctrl Pts',(2.29936936127588,-1.,-3.37867504959382));
#34877=CARTESIAN_POINT('Ctrl Pts',(2.30588783640389,-1.,-3.38282967336676));
#34878=CARTESIAN_POINT('Ctrl Pts',(2.31243319489505,-1.,-3.38695751492659));
#34879=CARTESIAN_POINT('Ctrl Pts',(2.31900513925627,-1.,-3.39105869475112));
#34880=CARTESIAN_POINT('Ctrl Pts',(2.32560343902683,-1.,-3.39513342020045));
#34881=CARTESIAN_POINT('Ctrl Pts',(2.33222789882601,-1.,-3.39918194578115));
#34882=CARTESIAN_POINT('Ctrl Pts',(2.33887832342715,-1.,-3.40320452776646));
#34883=CARTESIAN_POINT('Ctrl Pts',(2.34555447648901,-1.,-3.40720137403888));
#34884=CARTESIAN_POINT('Ctrl Pts',(2.35225606823649,-1.,-3.41117262313464));
#34885=CARTESIAN_POINT('Ctrl Pts',(2.35898278606449,-1.,-3.4151183675076));
#34886=CARTESIAN_POINT('Ctrl Pts',(2.36573431470313,-1.,-3.41903866635384));
#34887=CARTESIAN_POINT('Ctrl Pts',(2.37251035954351,-1.,-3.42293356216595));
#34888=CARTESIAN_POINT('Ctrl Pts',(2.37931067029517,-1.,-3.42680309755241));
#34889=CARTESIAN_POINT('Ctrl Pts',(2.38613505844641,-1.,-3.43064732714472));
#34890=CARTESIAN_POINT('Ctrl Pts',(2.39298338805823,-1.,-3.43446630680436));
#34891=CARTESIAN_POINT('Ctrl Pts',(2.39848113411428,-1.,-3.43750133066037));
#34892=CARTESIAN_POINT('Ctrl Pts',(2.40261515590099,-1.,-3.43976627485223));
#34893=CARTESIAN_POINT('Ctrl Pts',(2.40537592959345,-1.,-3.44127120683402));
#34894=CARTESIAN_POINT('Ctrl Pts',(2.40675750623143,-1.,-3.44202241512147));
#34895=CARTESIAN_POINT('',(2.52982887637028,-1.,-3.35260583073571));
#34896=CARTESIAN_POINT('',(2.40675750623143,-1.,-3.44202241512147));
#34897=CARTESIAN_POINT('',(2.36531447826073,-1.,-2.90994629141676));
#34898=CARTESIAN_POINT('Ctrl Pts',(2.52982887637028,-1.,-3.35260583073571));
#34899=CARTESIAN_POINT('Ctrl Pts',(2.5295413654909,-1.,-3.35105973714072));
#34900=CARTESIAN_POINT('Ctrl Pts',(2.52896321610703,-1.,-3.34796903576663));
#34901=CARTESIAN_POINT('Ctrl Pts',(2.52808660915689,-1.,-3.34333744115511));
#34902=CARTESIAN_POINT('Ctrl Pts',(2.52689902690158,-1.,-3.33717089999103));
#34903=CARTESIAN_POINT('Ctrl Pts',(2.52538321164634,-1.,-3.32947762187533));
#34904=CARTESIAN_POINT('Ctrl Pts',(2.5238359839626,-1.,-3.32179931078699));
#34905=CARTESIAN_POINT('Ctrl Pts',(2.52225724871313,-1.,-3.31413607874645));
#34906=CARTESIAN_POINT('Ctrl Pts',(2.52064689568511,-1.,-3.30648808815443));
#34907=CARTESIAN_POINT('Ctrl Pts',(2.51900480701068,-1.,-3.29885556388353));
#34908=CARTESIAN_POINT('Ctrl Pts',(2.51733085123797,-1.,-3.2912387729927));
#34909=CARTESIAN_POINT('Ctrl Pts',(2.51562487464514,-1.,-3.28363799702982));
#34910=CARTESIAN_POINT('Ctrl Pts',(2.513886692704,-1.,-3.27605350473142));
#34911=CARTESIAN_POINT('Ctrl Pts',(2.51211608411423,-1.,-3.26848552888116));
#34912=CARTESIAN_POINT('Ctrl Pts',(2.51031277813486,-1.,-3.26093423001434));
#34913=CARTESIAN_POINT('Ctrl Pts',(2.50847647070723,-1.,-3.25339971460982));
#34914=CARTESIAN_POINT('Ctrl Pts',(2.506606859405,-1.,-3.24588208983849));
#34915=CARTESIAN_POINT('Ctrl Pts',(2.5047036758003,-1.,-3.23838151080319));
#34916=CARTESIAN_POINT('Ctrl Pts',(2.50276671338111,-1.,-3.23089822320646));
#34917=CARTESIAN_POINT('Ctrl Pts',(2.50079587201957,-1.,-3.22343262620503));
#34918=CARTESIAN_POINT('Ctrl Pts',(2.4987911459939,-1.,-3.21598526261286));
#34919=CARTESIAN_POINT('Ctrl Pts',(2.4967525264737,-1.,-3.20855669849836));
#34920=CARTESIAN_POINT('Ctrl Pts',(2.49467992057755,-1.,-3.20114742397588));
#34921=CARTESIAN_POINT('Ctrl Pts',(2.49257307239848,-1.,-3.19375775555798));
#34922=CARTESIAN_POINT('Ctrl Pts',(2.49043146334059,-1.,-3.18638771282266));
#34923=CARTESIAN_POINT('Ctrl Pts',(2.48825428288201,-1.,-3.17903698136622));
#34924=CARTESIAN_POINT('Ctrl Pts',(2.48604065348587,-1.,-3.17170518863313));
#34925=CARTESIAN_POINT('Ctrl Pts',(2.48378981792725,-1.,-3.16439213290161));
#34926=CARTESIAN_POINT('Ctrl Pts',(2.48150133566571,-1.,-3.15709802322739));
#34927=CARTESIAN_POINT('Ctrl Pts',(2.47917529057029,-1.,-3.14982373241352));
#34928=CARTESIAN_POINT('Ctrl Pts',(2.47681245356109,-1.,-3.1425709954655));
#34929=CARTESIAN_POINT('Ctrl Pts',(2.47441378371932,-1.,-3.13534181229295));
#34930=CARTESIAN_POINT('Ctrl Pts',(2.47197997765871,-1.,-3.12813790805952));
#34931=CARTESIAN_POINT('Ctrl Pts',(2.46951098947469,-1.,-3.12096015766983));
#34932=CARTESIAN_POINT('Ctrl Pts',(2.46700558843506,-1.,-3.11380805536122));
#34933=CARTESIAN_POINT('Ctrl Pts',(2.46446082979646,-1.,-3.1066790790198));
#34934=CARTESIAN_POINT('Ctrl Pts',(2.46187308501884,-1.,-3.09956993697052));
#34935=CARTESIAN_POINT('Ctrl Pts',(2.4592391256388,-1.,-3.09247787931887));
#34936=CARTESIAN_POINT('Ctrl Pts',(2.45655725437039,-1.,-3.08540206545315));
#34937=CARTESIAN_POINT('Ctrl Pts',(2.4538282678779,-1.,-3.07834472886139));
#34938=CARTESIAN_POINT('Ctrl Pts',(2.45105688854422,-1.,-3.07131290521297));
#34939=CARTESIAN_POINT('Ctrl Pts',(2.44824970516543,-1.,-3.06431596421405));
#34940=CARTESIAN_POINT('Ctrl Pts',(2.44541251892556,-1.,-3.05736242671506));
#34941=CARTESIAN_POINT('Ctrl Pts',(2.44254768923105,-1.,-3.05045678021504));
#34942=CARTESIAN_POINT('Ctrl Pts',(2.43965194061857,-1.,-3.04359685040555));
#34943=CARTESIAN_POINT('Ctrl Pts',(2.43671278042414,-1.,-3.03676949672822));
#34944=CARTESIAN_POINT('Ctrl Pts',(2.43371241361488,-1.,-3.02995534946978));
#34945=CARTESIAN_POINT('Ctrl Pts',(2.43063415586637,-1.,-3.02313656036004));
#34946=CARTESIAN_POINT('Ctrl Pts',(2.42746856264168,-1.,-3.01630420830504));
#34947=CARTESIAN_POINT('Ctrl Pts',(2.42421849439613,-1.,-3.00946442616659));
#34948=CARTESIAN_POINT('Ctrl Pts',(2.42090763946779,-1.,-3.00264868585996));
#34949=CARTESIAN_POINT('Ctrl Pts',(2.41757324500514,-1.,-2.99590509293503));
#34950=CARTESIAN_POINT('Ctrl Pts',(2.41425064199586,-1.,-2.98927983005796));
#34951=CARTESIAN_POINT('Ctrl Pts',(2.41095909342571,-1.,-2.98280015815107));
#34952=CARTESIAN_POINT('Ctrl Pts',(2.40768975073713,-1.,-2.97646002822422));
#34953=CARTESIAN_POINT('Ctrl Pts',(2.40438604734919,-1.,-2.9701964131236));
#34954=CARTESIAN_POINT('Ctrl Pts',(2.4009556571164,-1.,-2.96390432240312));
#34955=CARTESIAN_POINT('Ctrl Pts',(2.39730553974516,-1.,-2.95748006482942));
#34956=CARTESIAN_POINT('Ctrl Pts',(2.39337207631667,-1.,-2.95085857128439));
#34957=CARTESIAN_POINT('Ctrl Pts',(2.38914929090759,-1.,-2.94404820669076));
#34958=CARTESIAN_POINT('Ctrl Pts',(2.38472771516311,-1.,-2.93717903280391));
#34959=CARTESIAN_POINT('Ctrl Pts',(2.38028989582073,-1.,-2.93049643640206));
#34960=CARTESIAN_POINT('Ctrl Pts',(2.3760651052403,-1.,-2.92430340582608));
#34961=CARTESIAN_POINT('Ctrl Pts',(2.37229381109821,-1.,-2.91891503791411));
#34962=CARTESIAN_POINT('Ctrl Pts',(2.36919161373173,-1.,-2.9146124988314));
#34963=CARTESIAN_POINT('Ctrl Pts',(2.36707658451664,-1.,-2.91181344022549));
#34964=CARTESIAN_POINT('Ctrl Pts',(2.36599991765749,-1.,-2.91051690822156));
#34965=CARTESIAN_POINT('Ctrl Pts',(2.36553202948613,-1.,-2.91005770527719));
#34966=CARTESIAN_POINT('Ctrl Pts',(2.36536211188453,-1.,-2.90995756655606));
#34967=CARTESIAN_POINT('Ctrl Pts',(2.36531447826073,-1.,-2.90994629141676));
#34968=CARTESIAN_POINT('',(2.50410331873042,-1.,-2.79140942341378));
#34969=CARTESIAN_POINT('Origin',(0.,-1.,0.));
#34970=CARTESIAN_POINT('',(2.91557726271063,-1.,-3.02314558451372));
#34971=CARTESIAN_POINT('Ctrl Pts',(2.50410331873042,-1.,-2.79140942341378));
#34972=CARTESIAN_POINT('Ctrl Pts',(2.50410700351426,-1.,-2.79145823440899));
#34973=CARTESIAN_POINT('Ctrl Pts',(2.50417932839343,-1.,-2.79164172519039));
#34974=CARTESIAN_POINT('Ctrl Pts',(2.50455968395235,-1.,-2.79217568804874));
#34975=CARTESIAN_POINT('Ctrl Pts',(2.50567182569153,-1.,-2.79344192164204));
#34976=CARTESIAN_POINT('Ctrl Pts',(2.50810555977564,-1.,-2.7959687805717));
#34977=CARTESIAN_POINT('Ctrl Pts',(2.51186983687947,-1.,-2.79970585014308));
#34978=CARTESIAN_POINT('Ctrl Pts',(2.51660190466067,-1.,-2.80427363984939));
#34979=CARTESIAN_POINT('Ctrl Pts',(2.52205778589922,-1.,-2.80941521967234));
#34980=CARTESIAN_POINT('Ctrl Pts',(2.52796388055457,-1.,-2.8148437904867));
#34981=CARTESIAN_POINT('Ctrl Pts',(2.53405679667463,-1.,-2.82028550483744));
#34982=CARTESIAN_POINT('Ctrl Pts',(2.54012272520141,-1.,-2.82552167649157));
#34983=CARTESIAN_POINT('Ctrl Pts',(2.54604736792542,-1.,-2.83044254225794));
#34984=CARTESIAN_POINT('Ctrl Pts',(2.55182152806964,-1.,-2.83505269592412));
#34985=CARTESIAN_POINT('Ctrl Pts',(2.55749952145165,-1.,-2.83942515220699));
#34986=CARTESIAN_POINT('Ctrl Pts',(2.56316920798489,-1.,-2.84366802680211));
#34987=CARTESIAN_POINT('Ctrl Pts',(2.56891984251743,-1.,-2.84788893329091));
#34988=CARTESIAN_POINT('Ctrl Pts',(2.57480482727128,-1.,-2.85215360144483));
#34989=CARTESIAN_POINT('Ctrl Pts',(2.58082875254407,-1.,-2.85647171715147));
#34990=CARTESIAN_POINT('Ctrl Pts',(2.5869677064356,-1.,-2.86081999003668));
#34991=CARTESIAN_POINT('Ctrl Pts',(2.59318160184921,-1.,-2.86515629953528));
#34992=CARTESIAN_POINT('Ctrl Pts',(2.59942875223202,-1.,-2.86943633170712));
#34993=CARTESIAN_POINT('Ctrl Pts',(2.6056817788128,-1.,-2.87363176656475));
#34994=CARTESIAN_POINT('Ctrl Pts',(2.61193507170928,-1.,-2.87773881947885));
#34995=CARTESIAN_POINT('Ctrl Pts',(2.61819596473087,-1.,-2.88176821427502));
#34996=CARTESIAN_POINT('Ctrl Pts',(2.62447947640253,-1.,-2.88573922195049));
#34997=CARTESIAN_POINT('Ctrl Pts',(2.63080195420771,-1.,-2.88967244854243));
#34998=CARTESIAN_POINT('Ctrl Pts',(2.63717442263944,-1.,-2.89358228854557));
#34999=CARTESIAN_POINT('Ctrl Pts',(2.64359851684146,-1.,-2.89747231723361));
#35000=CARTESIAN_POINT('Ctrl Pts',(2.65007017365576,-1.,-2.90133950224879));
#35001=CARTESIAN_POINT('Ctrl Pts',(2.65658188464287,-1.,-2.90517678087467));
#35002=CARTESIAN_POINT('Ctrl Pts',(2.66312542616808,-1.,-2.90897617968921));
#35003=CARTESIAN_POINT('Ctrl Pts',(2.66969458792627,-1.,-2.91273193382876));
#35004=CARTESIAN_POINT('Ctrl Pts',(2.67628728855309,-1.,-2.91644290704281));
#35005=CARTESIAN_POINT('Ctrl Pts',(2.68290409279689,-1.,-2.92011090722152));
#35006=CARTESIAN_POINT('Ctrl Pts',(2.68954721165342,-1.,-2.92373955325876));
#35007=CARTESIAN_POINT('Ctrl Pts',(2.69621932864302,-1.,-2.92733294395268));
#35008=CARTESIAN_POINT('Ctrl Pts',(2.70292247416881,-1.,-2.93089438233746));
#35009=CARTESIAN_POINT('Ctrl Pts',(2.70965695523776,-1.,-2.93442516311168));
#35010=CARTESIAN_POINT('Ctrl Pts',(2.71642190053575,-1.,-2.93792519474955));
#35011=CARTESIAN_POINT('Ctrl Pts',(2.72321571511322,-1.,-2.94139351933882));
#35012=CARTESIAN_POINT('Ctrl Pts',(2.73003657371613,-1.,-2.94482887675139));
#35013=CARTESIAN_POINT('Ctrl Pts',(2.73688288329825,-1.,-2.94823023414381));
#35014=CARTESIAN_POINT('Ctrl Pts',(2.7437537949221,-1.,-2.95159737214305));
#35015=CARTESIAN_POINT('Ctrl Pts',(2.75064903318996,-1.,-2.95493069316211));
#35016=CARTESIAN_POINT('Ctrl Pts',(2.75756867888393,-1.,-2.9582309766594));
#35017=CARTESIAN_POINT('Ctrl Pts',(2.76451296269571,-1.,-2.96149914764832));
#35018=CARTESIAN_POINT('Ctrl Pts',(2.77148206836464,-1.,-2.96473605585548));
#35019=CARTESIAN_POINT('Ctrl Pts',(2.77847589542767,-1.,-2.9679422104295));
#35020=CARTESIAN_POINT('Ctrl Pts',(2.78549409123657,-1.,-2.97111781461349));
#35021=CARTESIAN_POINT('Ctrl Pts',(2.79253615718147,-1.,-2.97426288347475));
#35022=CARTESIAN_POINT('Ctrl Pts',(2.79960153278186,-1.,-2.97737733718242));
#35023=CARTESIAN_POINT('Ctrl Pts',(2.80668968101162,-1.,-2.98046109647299));
#35024=CARTESIAN_POINT('Ctrl Pts',(2.81380019196454,-1.,-2.9835141977994));
#35025=CARTESIAN_POINT('Ctrl Pts',(2.82093279065704,-1.,-2.98653680669434));
#35026=CARTESIAN_POINT('Ctrl Pts',(2.82808728190402,-1.,-2.98952916401699));
#35027=CARTESIAN_POINT('Ctrl Pts',(2.83526351254383,-1.,-2.99249155170479));
#35028=CARTESIAN_POINT('Ctrl Pts',(2.84246132984334,-1.,-2.995424253416));
#35029=CARTESIAN_POINT('Ctrl Pts',(2.84968053289104,-1.,-2.99832751144566));
#35030=CARTESIAN_POINT('Ctrl Pts',(2.85692085715129,-1.,-3.0012015079552));
#35031=CARTESIAN_POINT('Ctrl Pts',(2.86418200833065,-1.,-3.00404638316245));
#35032=CARTESIAN_POINT('Ctrl Pts',(2.87146368430104,-1.,-3.00686224485374));
#35033=CARTESIAN_POINT('Ctrl Pts',(2.87876560072799,-1.,-3.0096491810855));
#35034=CARTESIAN_POINT('Ctrl Pts',(2.88608751706796,-1.,-3.01240727309568));
#35035=CARTESIAN_POINT('Ctrl Pts',(2.8934292556764,-1.,-3.01513660433291));
#35036=CARTESIAN_POINT('Ctrl Pts',(2.90079069102661,-1.,-3.01783725123646));
#35037=CARTESIAN_POINT('Ctrl Pts',(2.90669553303902,-1.,-3.01997487194926));
#35038=CARTESIAN_POINT('Ctrl Pts',(2.91113297349052,-1.,-3.02156522743299));
#35039=CARTESIAN_POINT('Ctrl Pts',(2.91409518070707,-1.,-3.02261975104912));
#35040=CARTESIAN_POINT('Ctrl Pts',(2.91557726271063,-1.,-3.02314558451372));
#35041=CARTESIAN_POINT('',(3.02314558451372,-1.,-2.91557726271063));
#35042=CARTESIAN_POINT('',(2.91557726271063,-1.,-3.02314558451372));
#35043=CARTESIAN_POINT('',(2.79140942341258,-1.,-2.50410331873176));
#35044=CARTESIAN_POINT('Ctrl Pts',(3.02314558451372,-1.,-2.91557726271063));
#35045=CARTESIAN_POINT('Ctrl Pts',(3.02261975104593,-1.,-2.91409518070399));
#35046=CARTESIAN_POINT('Ctrl Pts',(3.02156522742431,-1.,-2.91113297348212));
#35047=CARTESIAN_POINT('Ctrl Pts',(3.01997487193503,-1.,-2.90669553302526));
#35048=CARTESIAN_POINT('Ctrl Pts',(3.01783725121981,-1.,-2.9007906910105));
#35049=CARTESIAN_POINT('Ctrl Pts',(3.01513660431928,-1.,-2.89342925566321));
#35050=CARTESIAN_POINT('Ctrl Pts',(3.01240727308829,-1.,-2.8860875170608));
#35051=CARTESIAN_POINT('Ctrl Pts',(3.00964918108476,-1.,-2.87876560072727));
#35052=CARTESIAN_POINT('Ctrl Pts',(3.00686224485784,-1.,-2.87146368430502));
#35053=CARTESIAN_POINT('Ctrl Pts',(3.00404638316867,-1.,-2.86418200833667));
#35054=CARTESIAN_POINT('Ctrl Pts',(3.00120150796095,-1.,-2.85692085715686));
#35055=CARTESIAN_POINT('Ctrl Pts',(2.99832751144925,-1.,-2.84968053289451));
#35056=CARTESIAN_POINT('Ctrl Pts',(2.99542425341685,-1.,-2.84246132984415));
#35057=CARTESIAN_POINT('Ctrl Pts',(2.99249155170339,-1.,-2.83526351254248));
#35058=CARTESIAN_POINT('Ctrl Pts',(2.98952916401446,-1.,-2.82808728190157));
#35059=CARTESIAN_POINT('Ctrl Pts',(2.9865368066918,-1.,-2.82093279065457));
#35060=CARTESIAN_POINT('Ctrl Pts',(2.98351419779767,-1.,-2.81380019196286));
#35061=CARTESIAN_POINT('Ctrl Pts',(2.98046109647241,-1.,-2.80668968101106));
#35062=CARTESIAN_POINT('Ctrl Pts',(2.97737733718287,-1.,-2.7996015327823));
#35063=CARTESIAN_POINT('Ctrl Pts',(2.9742628834758,-1.,-2.79253615718248));
#35064=CARTESIAN_POINT('Ctrl Pts',(2.97111781461465,-1.,-2.78549409123769));
#35065=CARTESIAN_POINT('Ctrl Pts',(2.96794221043036,-1.,-2.7784758954285));
#35066=CARTESIAN_POINT('Ctrl Pts',(2.96473605585583,-1.,-2.77148206836498));
#35067=CARTESIAN_POINT('Ctrl Pts',(2.96149914764818,-1.,-2.76451296269557));
#35068=CARTESIAN_POINT('Ctrl Pts',(2.95823097665896,-1.,-2.7575686788835));
#35069=CARTESIAN_POINT('Ctrl Pts',(2.95493069316161,-1.,-2.75064903318947));
#35070=CARTESIAN_POINT('Ctrl Pts',(2.95159737214266,-1.,-2.74375379492172));
#35071=CARTESIAN_POINT('Ctrl Pts',(2.94823023414364,-1.,-2.73688288329808));
#35072=CARTESIAN_POINT('Ctrl Pts',(2.94482887675143,-1.,-2.73003657371617));
#35073=CARTESIAN_POINT('Ctrl Pts',(2.94139351933897,-1.,-2.72321571511337));
#35074=CARTESIAN_POINT('Ctrl Pts',(2.93792519474972,-1.,-2.71642190053592));
#35075=CARTESIAN_POINT('Ctrl Pts',(2.93442516311179,-1.,-2.70965695523787));
#35076=CARTESIAN_POINT('Ctrl Pts',(2.93089438233749,-1.,-2.70292247416885));
#35077=CARTESIAN_POINT('Ctrl Pts',(2.92733294395267,-1.,-2.69621932864301));
#35078=CARTESIAN_POINT('Ctrl Pts',(2.92373955325875,-1.,-2.68954721165339));
#35079=CARTESIAN_POINT('Ctrl Pts',(2.92011090722152,-1.,-2.68290409279688));
#35080=CARTESIAN_POINT('Ctrl Pts',(2.91644290704285,-1.,-2.67628728855312));
#35081=CARTESIAN_POINT('Ctrl Pts',(2.91273193382882,-1.,-2.66969458792631));
#35082=CARTESIAN_POINT('Ctrl Pts',(2.90897617968923,-1.,-2.6631254261681));
#35083=CARTESIAN_POINT('Ctrl Pts',(2.90517678087461,-1.,-2.65658188464282));
#35084=CARTESIAN_POINT('Ctrl Pts',(2.90133950224867,-1.,-2.65007017365564));
#35085=CARTESIAN_POINT('Ctrl Pts',(2.89747231723345,-1.,-2.64359851684131));
#35086=CARTESIAN_POINT('Ctrl Pts',(2.89358228854544,-1.,-2.63717442263932));
#35087=CARTESIAN_POINT('Ctrl Pts',(2.88967244854239,-1.,-2.63080195420767));
#35088=CARTESIAN_POINT('Ctrl Pts',(2.88573922195059,-1.,-2.62447947640262));
#35089=CARTESIAN_POINT('Ctrl Pts',(2.88176821427525,-1.,-2.61819596473108));
#35090=CARTESIAN_POINT('Ctrl Pts',(2.87773881947915,-1.,-2.61193507170955));
#35091=CARTESIAN_POINT('Ctrl Pts',(2.87363176656501,-1.,-2.60568177881303));
#35092=CARTESIAN_POINT('Ctrl Pts',(2.86943633170722,-1.,-2.5994287522321));
#35093=CARTESIAN_POINT('Ctrl Pts',(2.86515629953513,-1.,-2.59318160184908));
#35094=CARTESIAN_POINT('Ctrl Pts',(2.86081999003629,-1.,-2.58696770643524));
#35095=CARTESIAN_POINT('Ctrl Pts',(2.85647171715092,-1.,-2.58082875254357));
#35096=CARTESIAN_POINT('Ctrl Pts',(2.85215360144431,-1.,-2.57480482727081));
#35097=CARTESIAN_POINT('Ctrl Pts',(2.84788893329067,-1.,-2.56891984251721));
#35098=CARTESIAN_POINT('Ctrl Pts',(2.84366802680237,-1.,-2.56316920798513));
#35099=CARTESIAN_POINT('Ctrl Pts',(2.83942515220782,-1.,-2.55749952145241));
#35100=CARTESIAN_POINT('Ctrl Pts',(2.83505269592536,-1.,-2.55182152807077));
#35101=CARTESIAN_POINT('Ctrl Pts',(2.83044254225917,-1.,-2.54604736792655));
#35102=CARTESIAN_POINT('Ctrl Pts',(2.8255216764922,-1.,-2.54012272520199));
#35103=CARTESIAN_POINT('Ctrl Pts',(2.82028550483689,-1.,-2.53405679667412));
#35104=CARTESIAN_POINT('Ctrl Pts',(2.81484379048475,-1.,-2.52796388055278));
#35105=CARTESIAN_POINT('Ctrl Pts',(2.80941521966941,-1.,-2.52205778589653));
#35106=CARTESIAN_POINT('Ctrl Pts',(2.80427363984653,-1.,-2.51660190465805));
#35107=CARTESIAN_POINT('Ctrl Pts',(2.79970585014168,-1.,-2.51186983687818));
#35108=CARTESIAN_POINT('Ctrl Pts',(2.79596878057287,-1.,-2.50810555977671));
#35109=CARTESIAN_POINT('Ctrl Pts',(2.79344192164147,-1.,-2.50567182569081));
#35110=CARTESIAN_POINT('Ctrl Pts',(2.79217568804755,-1.,-2.50455968395146));
#35111=CARTESIAN_POINT('Ctrl Pts',(2.79164172518905,-1.,-2.50417932839313));
#35112=CARTESIAN_POINT('Ctrl Pts',(2.79145823440781,-1.,-2.50410700351493));
#35113=CARTESIAN_POINT('Ctrl Pts',(2.79140942341258,-1.,-2.50410331873176));
#35114=CARTESIAN_POINT('',(2.90994629141562,-1.,-2.36531447826213));
#35115=CARTESIAN_POINT('Origin',(0.,-1.,0.));
#35116=CARTESIAN_POINT('',(3.35260583073571,-1.,-2.52982887637028));
#35117=CARTESIAN_POINT('Ctrl Pts',(2.90994629141562,-1.,-2.36531447826213));
#35118=CARTESIAN_POINT('Ctrl Pts',(2.90995756655558,-1.,-2.3653621118858));
#35119=CARTESIAN_POINT('Ctrl Pts',(2.9100577052777,-1.,-2.36553202948741));
#35120=CARTESIAN_POINT('Ctrl Pts',(2.91051690822262,-1.,-2.36599991765853));
#35121=CARTESIAN_POINT('Ctrl Pts',(2.91181344022628,-1.,-2.36707658451709));
#35122=CARTESIAN_POINT('Ctrl Pts',(2.91461249883016,-1.,-2.36919161373074));
#35123=CARTESIAN_POINT('Ctrl Pts',(2.9189150379156,-1.,-2.37229381109939));
#35124=CARTESIAN_POINT('Ctrl Pts',(2.92430340582912,-1.,-2.37606510524271));
#35125=CARTESIAN_POINT('Ctrl Pts',(2.93049643640517,-1.,-2.3802898958232));
#35126=CARTESIAN_POINT('Ctrl Pts',(2.93717903280599,-1.,-2.38472771516476));
#35127=CARTESIAN_POINT('Ctrl Pts',(2.94404820669135,-1.,-2.38914929090806));
#35128=CARTESIAN_POINT('Ctrl Pts',(2.95085857128372,-1.,-2.39337207631613));
#35129=CARTESIAN_POINT('Ctrl Pts',(2.95748006482811,-1.,-2.39730553974412));
#35130=CARTESIAN_POINT('Ctrl Pts',(2.9639043224018,-1.,-2.40095565711535));
#35131=CARTESIAN_POINT('Ctrl Pts',(2.97019641312272,-1.,-2.40438604734848));
#35132=CARTESIAN_POINT('Ctrl Pts',(2.97646002822395,-1.,-2.40768975073691));
#35133=CARTESIAN_POINT('Ctrl Pts',(2.98280015815132,-1.,-2.41095909342591));
#35134=CARTESIAN_POINT('Ctrl Pts',(2.98927983005851,-1.,-2.4142506419963));
#35135=CARTESIAN_POINT('Ctrl Pts',(2.99590509293561,-1.,-2.4175732450056));
#35136=CARTESIAN_POINT('Ctrl Pts',(3.00264868586038,-1.,-2.42090763946812));
#35137=CARTESIAN_POINT('Ctrl Pts',(3.00946442616674,-1.,-2.42421849439625));
#35138=CARTESIAN_POINT('Ctrl Pts',(3.01630420830493,-1.,-2.4274685626416));
#35139=CARTESIAN_POINT('Ctrl Pts',(3.02313656035977,-1.,-2.43063415586615));
#35140=CARTESIAN_POINT('Ctrl Pts',(3.02995534946946,-1.,-2.43371241361462));
#35141=CARTESIAN_POINT('Ctrl Pts',(3.03676949672797,-1.,-2.43671278042394));
#35142=CARTESIAN_POINT('Ctrl Pts',(3.04359685040545,-1.,-2.43965194061849));
#35143=CARTESIAN_POINT('Ctrl Pts',(3.05045678021509,-1.,-2.44254768923109));
#35144=CARTESIAN_POINT('Ctrl Pts',(3.05736242671521,-1.,-2.44541251892568));
#35145=CARTESIAN_POINT('Ctrl Pts',(3.06431596421422,-1.,-2.44824970516558));
#35146=CARTESIAN_POINT('Ctrl Pts',(3.0713129052131,-1.,-2.45105688854432));
#35147=CARTESIAN_POINT('Ctrl Pts',(3.07834472886145,-1.,-2.45382826787795));
#35148=CARTESIAN_POINT('Ctrl Pts',(3.08540206545313,-1.,-2.45655725437037));
#35149=CARTESIAN_POINT('Ctrl Pts',(3.09247787931881,-1.,-2.45923912563875));
#35150=CARTESIAN_POINT('Ctrl Pts',(3.09956993697048,-1.,-2.4618730850188));
#35151=CARTESIAN_POINT('Ctrl Pts',(3.10667907901981,-1.,-2.46446082979645));
#35152=CARTESIAN_POINT('Ctrl Pts',(3.11380805536124,-1.,-2.46700558843507));
#35153=CARTESIAN_POINT('Ctrl Pts',(3.12096015766984,-1.,-2.4695109894747));
#35154=CARTESIAN_POINT('Ctrl Pts',(3.12813790805948,-1.,-2.47197997765868));
#35155=CARTESIAN_POINT('Ctrl Pts',(3.13534181229282,-1.,-2.47441378371923));
#35156=CARTESIAN_POINT('Ctrl Pts',(3.14257099546531,-1.,-2.47681245356095));
#35157=CARTESIAN_POINT('Ctrl Pts',(3.14982373241335,-1.,-2.47917529057016));
#35158=CARTESIAN_POINT('Ctrl Pts',(3.15709802322735,-1.,-2.48150133566568));
#35159=CARTESIAN_POINT('Ctrl Pts',(3.16439213290181,-1.,-2.48378981792739));
#35160=CARTESIAN_POINT('Ctrl Pts',(3.17170518863357,-1.,-2.48604065348619));
#35161=CARTESIAN_POINT('Ctrl Pts',(3.17903698136678,-1.,-2.48825428288243));
#35162=CARTESIAN_POINT('Ctrl Pts',(3.18638771282315,-1.,-2.49043146334095));
#35163=CARTESIAN_POINT('Ctrl Pts',(3.19375775555814,-1.,-2.4925730723986));
#35164=CARTESIAN_POINT('Ctrl Pts',(3.20114742397549,-1.,-2.49467992057726));
#35165=CARTESIAN_POINT('Ctrl Pts',(3.2085566984974,-1.,-2.49675252647298));
#35166=CARTESIAN_POINT('Ctrl Pts',(3.21598526261157,-1.,-2.49879114599293));
#35167=CARTESIAN_POINT('Ctrl Pts',(3.22343262620387,-1.,-2.5007958720187));
#35168=CARTESIAN_POINT('Ctrl Pts',(3.23089822320596,-1.,-2.50276671338074));
#35169=CARTESIAN_POINT('Ctrl Pts',(3.23838151080383,-1.,-2.50470367580078));
#35170=CARTESIAN_POINT('Ctrl Pts',(3.24588208984042,-1.,-2.50660685940645));
#35171=CARTESIAN_POINT('Ctrl Pts',(3.25339971461265,-1.,-2.50847647070936));
#35172=CARTESIAN_POINT('Ctrl Pts',(3.26093423001716,-1.,-2.51031277813697));
#35173=CARTESIAN_POINT('Ctrl Pts',(3.26848552888271,-1.,-2.51211608411539));
#35174=CARTESIAN_POINT('Ctrl Pts',(3.27605350473048,-1.,-2.51388669270329));
#35175=CARTESIAN_POINT('Ctrl Pts',(3.28363799702583,-1.,-2.51562487464215));
#35176=CARTESIAN_POINT('Ctrl Pts',(3.2912387729863,-1.,-2.51733085123316));
#35177=CARTESIAN_POINT('Ctrl Pts',(3.29885556387661,-1.,-2.51900480700548));
#35178=CARTESIAN_POINT('Ctrl Pts',(3.30648808814986,-1.,-2.52064689568167));
#35179=CARTESIAN_POINT('Ctrl Pts',(3.31413607874727,-1.,-2.52225724871375));
#35180=CARTESIAN_POINT('Ctrl Pts',(3.32179931079521,-1.,-2.52383598396878));
#35181=CARTESIAN_POINT('Ctrl Pts',(3.32947762189049,-1.,-2.52538321165774));
#35182=CARTESIAN_POINT('Ctrl Pts',(3.33717090000955,-1.,-2.52689902691551));
#35183=CARTESIAN_POINT('Ctrl Pts',(3.34333744117093,-1.,-2.52808660916879));
#35184=CARTESIAN_POINT('Ctrl Pts',(3.34796903577628,-1.,-2.5289632161143));
#35185=CARTESIAN_POINT('Ctrl Pts',(3.35105973714426,-1.,-2.52954136549357));
#35186=CARTESIAN_POINT('Ctrl Pts',(3.35260583073571,-1.,-2.52982887637028));
#35187=CARTESIAN_POINT('',(3.44202241512147,-1.,-2.40675750623143));
#35188=CARTESIAN_POINT('',(3.35260583073571,-1.,-2.52982887637028));
#35189=CARTESIAN_POINT('',(3.14877060440327,-1.,-2.03660101169714));
#35190=CARTESIAN_POINT('Ctrl Pts',(3.44202241512147,-1.,-2.40675750623143));
#35191=CARTESIAN_POINT('Ctrl Pts',(3.44127120683039,-1.,-2.4053759295909));
#35192=CARTESIAN_POINT('Ctrl Pts',(3.43976627484234,-1.,-2.40261515589405));
#35193=CARTESIAN_POINT('Ctrl Pts',(3.43750133064416,-1.,-2.39848113410292));
#35194=CARTESIAN_POINT('Ctrl Pts',(3.4344663067854,-1.,-2.39298338804493));
#35195=CARTESIAN_POINT('Ctrl Pts',(3.43064732712919,-1.,-2.38613505843552));
#35196=CARTESIAN_POINT('Ctrl Pts',(3.42680309754399,-1.,-2.37931067028926));
#35197=CARTESIAN_POINT('Ctrl Pts',(3.42293356216511,-1.,-2.37251035954292));
#35198=CARTESIAN_POINT('Ctrl Pts',(3.41903866635852,-1.,-2.36573431470642));
#35199=CARTESIAN_POINT('Ctrl Pts',(3.41511836751469,-1.,-2.35898278606946));
#35200=CARTESIAN_POINT('Ctrl Pts',(3.41117262314119,-1.,-2.35225606824109));
#35201=CARTESIAN_POINT('Ctrl Pts',(3.40720137404297,-1.,-2.34555447649188));
#35202=CARTESIAN_POINT('Ctrl Pts',(3.40320452776743,-1.,-2.33887832342782));
#35203=CARTESIAN_POINT('Ctrl Pts',(3.39918194577956,-1.,-2.33222789882489));
#35204=CARTESIAN_POINT('Ctrl Pts',(3.39513342019756,-1.,-2.3256034390248));
#35205=CARTESIAN_POINT('Ctrl Pts',(3.39105869474822,-1.,-2.31900513925424));
#35206=CARTESIAN_POINT('Ctrl Pts',(3.38695751492462,-1.,-2.31243319489367));
#35207=CARTESIAN_POINT('Ctrl Pts',(3.3828296733661,-1.,-2.30588783640343));
#35208=CARTESIAN_POINT('Ctrl Pts',(3.37867504959433,-1.,-2.29936936127624));
#35209=CARTESIAN_POINT('Ctrl Pts',(3.37449367172826,-1.,-2.29287818007393));
#35210=CARTESIAN_POINT('Ctrl Pts',(3.37028570206488,-1.,-2.28641481081137));
#35211=CARTESIAN_POINT('Ctrl Pts',(3.36605130713076,-1.,-2.27997979458037));
#35212=CARTESIAN_POINT('Ctrl Pts',(3.36179055004409,-1.,-2.2735736262093));
#35213=CARTESIAN_POINT('Ctrl Pts',(3.35750328523061,-1.,-2.2671966857991));
#35214=CARTESIAN_POINT('Ctrl Pts',(3.35318902552626,-1.,-2.26084915222449));
#35215=CARTESIAN_POINT('Ctrl Pts',(3.34884690292285,-1.,-2.25453097693483));
#35216=CARTESIAN_POINT('Ctrl Pts',(3.34447596770723,-1.,-2.24824207678256));
#35217=CARTESIAN_POINT('Ctrl Pts',(3.34007543738025,-1.,-2.24198249391422));
#35218=CARTESIAN_POINT('Ctrl Pts',(3.33564495756481,-1.,-2.23575256328812));
#35219=CARTESIAN_POINT('Ctrl Pts',(3.33118487773611,-1.,-2.22955308907233));
#35220=CARTESIAN_POINT('Ctrl Pts',(3.3266964672289,-1.,-2.22338548312772));
#35221=CARTESIAN_POINT('Ctrl Pts',(3.32218125618968,-1.,-2.21725135110898));
#35222=CARTESIAN_POINT('Ctrl Pts',(3.31764044024235,-1.,-2.21115211847875));
#35223=CARTESIAN_POINT('Ctrl Pts',(3.31307424608949,-1.,-2.20508863150607));
#35224=CARTESIAN_POINT('Ctrl Pts',(3.30848134694595,-1.,-2.19906078949923));
#35225=CARTESIAN_POINT('Ctrl Pts',(3.30385816281831,-1.,-2.19306710376111));
#35226=CARTESIAN_POINT('Ctrl Pts',(3.29920022557639,-1.,-2.18710556500327));
#35227=CARTESIAN_POINT('Ctrl Pts',(3.2945036150049,-1.,-2.18117455557065));
#35228=CARTESIAN_POINT('Ctrl Pts',(3.28976645712568,-1.,-2.17527380048423));
#35229=CARTESIAN_POINT('Ctrl Pts',(3.28499019979724,-1.,-2.16940517773455));
#35230=CARTESIAN_POINT('Ctrl Pts',(3.280181508414,-1.,-2.16357391934425));
#35231=CARTESIAN_POINT('Ctrl Pts',(3.27534954469187,-1.,-2.15778690038347));
#35232=CARTESIAN_POINT('Ctrl Pts',(3.27050245897228,-1.,-2.15205043199808));
#35233=CARTESIAN_POINT('Ctrl Pts',(3.26564388189759,-1.,-2.1463680529566));
#35234=CARTESIAN_POINT('Ctrl Pts',(3.26077002641879,-1.,-2.14073870754264));
#35235=CARTESIAN_POINT('Ctrl Pts',(3.25586495065054,-1.,-2.13515375878803));
#35236=CARTESIAN_POINT('Ctrl Pts',(3.25090574494028,-1.,-2.12960028396832));
#35237=CARTESIAN_POINT('Ctrl Pts',(3.24587102613376,-1.,-2.12406646410962));
#35238=CARTESIAN_POINT('Ctrl Pts',(3.24074905517293,-1.,-2.11854673326979));
#35239=CARTESIAN_POINT('Ctrl Pts',(3.23554444767099,-1.,-2.11304604021773));
#35240=CARTESIAN_POINT('Ctrl Pts',(3.23028945793289,-1.,-2.10758699642451));
#35241=CARTESIAN_POINT('Ctrl Pts',(3.22503437553434,-1.,-2.10220384298492));
#35242=CARTESIAN_POINT('Ctrl Pts',(3.21982707347009,-1.,-2.09692958434895));
#35243=CARTESIAN_POINT('Ctrl Pts',(3.21469429601654,-1.,-2.09178419460443));
#35244=CARTESIAN_POINT('Ctrl Pts',(3.20962575845463,-1.,-2.08676465517455));
#35245=CARTESIAN_POINT('Ctrl Pts',(3.2045481863073,-1.,-2.08182850370878));
#35246=CARTESIAN_POINT('Ctrl Pts',(3.19934132836019,-1.,-2.07690441870722));
#35247=CARTESIAN_POINT('Ctrl Pts',(3.19388465568252,-1.,-2.07192253497857));
#35248=CARTESIAN_POINT('Ctrl Pts',(3.18809755562368,-1.,-2.06684062744112));
#35249=CARTESIAN_POINT('Ctrl Pts',(3.18197692964614,-1.,-2.06166849827101));
#35250=CARTESIAN_POINT('Ctrl Pts',(3.17564906975371,-1.,-2.05650186773132));
#35251=CARTESIAN_POINT('Ctrl Pts',(3.16936341689527,-1.,-2.05151770247233));
#35252=CARTESIAN_POINT('Ctrl Pts',(3.16343165058912,-1.,-2.04693331247446));
#35253=CARTESIAN_POINT('Ctrl Pts',(3.15817983946367,-1.,-2.04297406404027));
#35254=CARTESIAN_POINT('Ctrl Pts',(3.15389991674792,-1.,-2.03984073791519));
#35255=CARTESIAN_POINT('Ctrl Pts',(3.15102344775328,-1.,-2.03783225495961));
#35256=CARTESIAN_POINT('Ctrl Pts',(3.14959882629805,-1.,-2.03693188810545));
#35257=CARTESIAN_POINT('Ctrl Pts',(3.1490119366901,-1.,-2.03663974554932));
#35258=CARTESIAN_POINT('Ctrl Pts',(3.14881939088124,-1.,-2.03659701539259));
#35259=CARTESIAN_POINT('Ctrl Pts',(3.14877060440327,-1.,-2.03660101169714));
#35260=CARTESIAN_POINT('',(3.24413672884812,-1.,-1.88097764062697));
#35261=CARTESIAN_POINT('Origin',(0.,-1.,0.));
#35262=CARTESIAN_POINT('',(3.70708211654725,-1.,-1.97421938526992));
#35263=CARTESIAN_POINT('Ctrl Pts',(3.24413672884812,-1.,-1.88097764062697));
#35264=CARTESIAN_POINT('Ctrl Pts',(3.24415531671284,-1.,-1.8810229239812));
#35265=CARTESIAN_POINT('Ctrl Pts',(3.24428080353022,-1.,-1.88117508446775));
#35266=CARTESIAN_POINT('Ctrl Pts',(3.24480754676064,-1.,-1.88156537699203));
#35267=CARTESIAN_POINT('Ctrl Pts',(3.2462565441079,-1.,-1.88242596600454));
#35268=CARTESIAN_POINT('Ctrl Pts',(3.24935200511918,-1.,-1.88407708646357));
#35269=CARTESIAN_POINT('Ctrl Pts',(3.25408686339463,-1.,-1.88646802523466));
#35270=CARTESIAN_POINT('Ctrl Pts',(3.25999885193947,-1.,-1.88934996203698));
#35271=CARTESIAN_POINT('Ctrl Pts',(3.26677653888676,-1.,-1.89255393500965));
#35272=CARTESIAN_POINT('Ctrl Pts',(3.27407108933139,-1.,-1.89589172903793));
#35273=CARTESIAN_POINT('Ctrl Pts',(3.28154737912352,-1.,-1.89918429230462));
#35274=CARTESIAN_POINT('Ctrl Pts',(3.2889344860029,-1.,-1.90228971247527));
#35275=CARTESIAN_POINT('Ctrl Pts',(3.29608978722113,-1.,-1.90513891864087));
#35276=CARTESIAN_POINT('Ctrl Pts',(3.30300595568195,-1.,-1.90773912171341));
#35277=CARTESIAN_POINT('Ctrl Pts',(3.30975721158596,-1.,-1.91014297830446));
#35278=CARTESIAN_POINT('Ctrl Pts',(3.31646052426364,-1.,-1.91242616234442));
#35279=CARTESIAN_POINT('Ctrl Pts',(3.32323403454535,-1.,-1.91466343916628));
#35280=CARTESIAN_POINT('Ctrl Pts',(3.33014884257873,-1.,-1.91690081930332));
#35281=CARTESIAN_POINT('Ctrl Pts',(3.33721230710012,-1.,-1.9191460961021));
#35282=CARTESIAN_POINT('Ctrl Pts',(3.34439448941961,-1.,-1.92138450828404));
#35283=CARTESIAN_POINT('Ctrl Pts',(3.35164424847223,-1.,-1.92358838440528));
#35284=CARTESIAN_POINT('Ctrl Pts',(3.35890824422965,-1.,-1.92572846125756));
#35285=CARTESIAN_POINT('Ctrl Pts',(3.36615168657567,-1.,-1.92778626543786));
#35286=CARTESIAN_POINT('Ctrl Pts',(3.37336807068043,-1.,-1.92975993109877));
#35287=CARTESIAN_POINT('Ctrl Pts',(3.3805676852555,-1.,-1.93165739093276));
#35288=CARTESIAN_POINT('Ctrl Pts',(3.38777076883256,-1.,-1.93349233176788));
#35289=CARTESIAN_POINT('Ctrl Pts',(3.39499923640795,-1.,-1.93527929945985));
#35290=CARTESIAN_POINT('Ctrl Pts',(3.40226802104109,-1.,-1.93702857723098));
#35291=CARTESIAN_POINT('Ctrl Pts',(3.40957978266642,-1.,-1.93874306008143));
#35292=CARTESIAN_POINT('Ctrl Pts',(3.41692971994096,-1.,-1.94042111965246));
#35293=CARTESIAN_POINT('Ctrl Pts',(3.42430850941503,-1.,-1.94205835913696));
#35294=CARTESIAN_POINT('Ctrl Pts',(3.43170586602434,-1.,-1.94364973660284));
#35295=CARTESIAN_POINT('Ctrl Pts',(3.43911410197687,-1.,-1.94519168842879));
#35296=CARTESIAN_POINT('Ctrl Pts',(3.44653088665681,-1.,-1.94668377715329));
#35297=CARTESIAN_POINT('Ctrl Pts',(3.45395731584051,-1.,-1.94812754766524));
#35298=CARTESIAN_POINT('Ctrl Pts',(3.46139661060962,-1.,-1.94952575850197));
#35299=CARTESIAN_POINT('Ctrl Pts',(3.46885258974191,-1.,-1.95088147859877));
#35300=CARTESIAN_POINT('Ctrl Pts',(3.47632820495921,-1.,-1.95219722189876));
#35301=CARTESIAN_POINT('Ctrl Pts',(3.48382414832634,-1.,-1.95347412486309));
#35302=CARTESIAN_POINT('Ctrl Pts',(3.49133956289133,-1.,-1.95471236969643));
#35303=CARTESIAN_POINT('Ctrl Pts',(3.49887263575583,-1.,-1.95591153823661));
#35304=CARTESIAN_POINT('Ctrl Pts',(3.50642124159909,-1.,-1.95707099606511));
#35305=CARTESIAN_POINT('Ctrl Pts',(3.51398354617794,-1.,-1.95819025316779));
#35306=CARTESIAN_POINT('Ctrl Pts',(3.52155867431486,-1.,-1.95926936324461));
#35307=CARTESIAN_POINT('Ctrl Pts',(3.52914648844351,-1.,-1.96030879411566));
#35308=CARTESIAN_POINT('Ctrl Pts',(3.53674730625813,-1.,-1.96130926212689));
#35309=CARTESIAN_POINT('Ctrl Pts',(3.54436163300443,-1.,-1.96227157573067));
#35310=CARTESIAN_POINT('Ctrl Pts',(3.55198990600886,-1.,-1.96319648628644));
#35311=CARTESIAN_POINT('Ctrl Pts',(3.55963218706096,-1.,-1.96408450906812));
#35312=CARTESIAN_POINT('Ctrl Pts',(3.56728820357791,-1.,-1.96493594634567));
#35313=CARTESIAN_POINT('Ctrl Pts',(3.57495748600959,-1.,-1.96575096652789));
#35314=CARTESIAN_POINT('Ctrl Pts',(3.58263947663829,-1.,-1.96652966688911));
#35315=CARTESIAN_POINT('Ctrl Pts',(3.59033364022801,-1.,-1.96727213799544));
#35316=CARTESIAN_POINT('Ctrl Pts',(3.59803959819938,-1.,-1.96797854118369));
#35317=CARTESIAN_POINT('Ctrl Pts',(3.60575714017989,-1.,-1.9686491188594));
#35318=CARTESIAN_POINT('Ctrl Pts',(3.61348615496704,-1.,-1.96928416040877));
#35319=CARTESIAN_POINT('Ctrl Pts',(3.62122658401893,-1.,-1.96988398129978));
#35320=CARTESIAN_POINT('Ctrl Pts',(3.62897836973293,-1.,-1.97044889850463));
#35321=CARTESIAN_POINT('Ctrl Pts',(3.63674139590412,-1.,-1.97097920454464));
#35322=CARTESIAN_POINT('Ctrl Pts',(3.64451546723514,-1.,-1.97147515441164));
#35323=CARTESIAN_POINT('Ctrl Pts',(3.652300347166,-1.,-1.9719369724024));
#35324=CARTESIAN_POINT('Ctrl Pts',(3.6600957816636,-1.,-1.9723648543905));
#35325=CARTESIAN_POINT('Ctrl Pts',(3.66790152752075,-1.,-1.97275897198678));
#35326=CARTESIAN_POINT('Ctrl Pts',(3.67571738107084,-1.,-1.97311947678517));
#35327=CARTESIAN_POINT('Ctrl Pts',(3.68354319915092,-1.,-1.97344650304519));
#35328=CARTESIAN_POINT('Ctrl Pts',(3.69137888599902,-1.,-1.97374016225483));
#35329=CARTESIAN_POINT('Ctrl Pts',(3.6976552856004,-1.,-1.97394846383216));
#35330=CARTESIAN_POINT('Ctrl Pts',(3.70236698912904,-1.,-1.97408973726715));
#35331=CARTESIAN_POINT('Ctrl Pts',(3.70551008132332,-1.,-1.97417727645308));
#35332=CARTESIAN_POINT('Ctrl Pts',(3.70708211654725,-1.,-1.97421938526992));
#35333=CARTESIAN_POINT('',(3.77614523045147,-1.,-1.83867539237861));
#35334=CARTESIAN_POINT('',(3.70708211654725,-1.,-1.97421938526992));
#35335=CARTESIAN_POINT('',(3.42859860294305,-1.,-1.5189508286633));
#35336=CARTESIAN_POINT('Ctrl Pts',(3.77614523045147,-1.,-1.83867539237861));
#35337=CARTESIAN_POINT('Ctrl Pts',(3.77518714457833,-1.,-1.83742834010626));
#35338=CARTESIAN_POINT('Ctrl Pts',(3.77326886064398,-1.,-1.83493697934534));
#35339=CARTESIAN_POINT('Ctrl Pts',(3.77038509817999,-1.,-1.83120816955646));
#35340=CARTESIAN_POINT('Ctrl Pts',(3.76652740353775,-1.,-1.82625289220915));
#35341=CARTESIAN_POINT('Ctrl Pts',(3.76168412707948,-1.,-1.82008629694091));
#35342=CARTESIAN_POINT('Ctrl Pts',(3.75681965683071,-1.,-1.8139472983358));
#35343=CARTESIAN_POINT('Ctrl Pts',(3.75193395887977,-1.,-1.80783603939617));
#35344=CARTESIAN_POINT('Ctrl Pts',(3.74702700875467,-1.,-1.8017527148577));
#35345=CARTESIAN_POINT('Ctrl Pts',(3.74209880352445,-1.,-1.79569757859422));
#35346=CARTESIAN_POINT('Ctrl Pts',(3.73714934730681,-1.,-1.78967092823491));
#35347=CARTESIAN_POINT('Ctrl Pts',(3.7321786309547,-1.,-1.78367308442901));
#35348=CARTESIAN_POINT('Ctrl Pts',(3.72718661205609,-1.,-1.77770437039658));
#35349=CARTESIAN_POINT('Ctrl Pts',(3.72217319911254,-1.,-1.77176509401761));
#35350=CARTESIAN_POINT('Ctrl Pts',(3.71713822377359,-1.,-1.76585552124394));
#35351=CARTESIAN_POINT('Ctrl Pts',(3.71208146346136,-1.,-1.75997588498865));
#35352=CARTESIAN_POINT('Ctrl Pts',(3.70700269736659,-1.,-1.75412641804042));
#35353=CARTESIAN_POINT('Ctrl Pts',(3.7019017567335,-1.,-1.74830738046057));
#35354=CARTESIAN_POINT('Ctrl Pts',(3.69677856910517,-1.,-1.74251908492617));
#35355=CARTESIAN_POINT('Ctrl Pts',(3.69163322648036,-1.,-1.73676193254557));
#35356=CARTESIAN_POINT('Ctrl Pts',(3.68646597019332,-1.,-1.73103640956717));
#35357=CARTESIAN_POINT('Ctrl Pts',(3.68127704936579,-1.,-1.72534302437056));
#35358=CARTESIAN_POINT('Ctrl Pts',(3.67606660374709,-1.,-1.71968225581808));
#35359=CARTESIAN_POINT('Ctrl Pts',(3.67083454901611,-1.,-1.71405450210384));
#35360=CARTESIAN_POINT('Ctrl Pts',(3.66558043198876,-1.,-1.70846001610956));
#35361=CARTESIAN_POINT('Ctrl Pts',(3.66030338774847,-1.,-1.70289888566873));
#35362=CARTESIAN_POINT('Ctrl Pts',(3.65500246526749,-1.,-1.69737117722534));
#35363=CARTESIAN_POINT('Ctrl Pts',(3.64967689827371,-1.,-1.69187705481689));
#35364=CARTESIAN_POINT('Ctrl Pts',(3.64432638915203,-1.,-1.68641690471457));
#35365=CARTESIAN_POINT('Ctrl Pts',(3.63895140887462,-1.,-1.68099146651586));
#35366=CARTESIAN_POINT('Ctrl Pts',(3.63355343201232,-1.,-1.67560193613156));
#35367=CARTESIAN_POINT('Ctrl Pts',(3.62813422105271,-1.,-1.67024966008045));
#35368=CARTESIAN_POINT('Ctrl Pts',(3.62269517989109,-1.,-1.66493585923855));
#35369=CARTESIAN_POINT('Ctrl Pts',(3.61723666482456,-1.,-1.65966133399186));
#35370=CARTESIAN_POINT('Ctrl Pts',(3.61175734965127,-1.,-1.65442619244325));
#35371=CARTESIAN_POINT('Ctrl Pts',(3.60625346556992,-1.,-1.64922952425832));
#35372=CARTESIAN_POINT('Ctrl Pts',(3.60072028513845,-1.,-1.64407004385582));
#35373=CARTESIAN_POINT('Ctrl Pts',(3.59515368334893,-1.,-1.63894676675352));
#35374=CARTESIAN_POINT('Ctrl Pts',(3.58955176627879,-1.,-1.6338597145126));
#35375=CARTESIAN_POINT('Ctrl Pts',(3.58391625774343,-1.,-1.62881051550745));
#35376=CARTESIAN_POINT('Ctrl Pts',(3.5782545595439,-1.,-1.62380329464844));
#35377=CARTESIAN_POINT('Ctrl Pts',(3.57257679609806,-1.,-1.61884340915404));
#35378=CARTESIAN_POINT('Ctrl Pts',(3.56689200468387,-1.,-1.61393581747514));
#35379=CARTESIAN_POINT('Ctrl Pts',(3.5612043248298,-1.,-1.60908344685457));
#35380=CARTESIAN_POINT('Ctrl Pts',(3.55550985096129,-1.,-1.60428584699853));
#35381=CARTESIAN_POINT('Ctrl Pts',(3.54979148634454,-1.,-1.59953698113457));
#35382=CARTESIAN_POINT('Ctrl Pts',(3.54402458182337,-1.,-1.59482766949766));
#35383=CARTESIAN_POINT('Ctrl Pts',(3.53818616861077,-1.,-1.59014958368739));
#35384=CARTESIAN_POINT('Ctrl Pts',(3.5322637814708,-1.,-1.58549906268088));
#35385=CARTESIAN_POINT('Ctrl Pts',(3.52626275334881,-1.,-1.58088027227848));
#35386=CARTESIAN_POINT('Ctrl Pts',(3.52021847865912,-1.,-1.57631049988158));
#35387=CARTESIAN_POINT('Ctrl Pts',(3.51418598431665,-1.,-1.57181569799743));
#35388=CARTESIAN_POINT('Ctrl Pts',(3.50821771695363,-1.,-1.56742097575012));
#35389=CARTESIAN_POINT('Ctrl Pts',(3.50234321621578,-1.,-1.56314187758675));
#35390=CARTESIAN_POINT('Ctrl Pts',(3.49655185179655,-1.,-1.55897703097874));
#35391=CARTESIAN_POINT('Ctrl Pts',(3.4907646087742,-1.,-1.55489595901116));
#35392=CARTESIAN_POINT('Ctrl Pts',(3.48485155928567,-1.,-1.55084702970452));
#35393=CARTESIAN_POINT('Ctrl Pts',(3.47868272898751,-1.,-1.54678009290276));
#35394=CARTESIAN_POINT('Ctrl Pts',(3.47217189224653,-1.,-1.54266605398188));
#35395=CARTESIAN_POINT('Ctrl Pts',(3.46531752207153,-1.,-1.53851507915502));
#35396=CARTESIAN_POINT('Ctrl Pts',(3.45825932955032,-1.,-1.53440195378792));
#35397=CARTESIAN_POINT('Ctrl Pts',(3.45127136828305,-1.,-1.53046244461635));
#35398=CARTESIAN_POINT('Ctrl Pts',(3.44469547526647,-1.,-1.52686242875556));
#35399=CARTESIAN_POINT('Ctrl Pts',(3.4388889597401,-1.,-1.5237734895035));
#35400=CARTESIAN_POINT('Ctrl Pts',(3.43417156977893,-1.,-1.52134826724293));
#35401=CARTESIAN_POINT('Ctrl Pts',(3.43101631893414,-1.,-1.5198144909338));
#35402=CARTESIAN_POINT('Ctrl Pts',(3.42946838852587,-1.,-1.51914806898491));
#35403=CARTESIAN_POINT('Ctrl Pts',(3.42884302333841,-1.,-1.5189513329503));
#35404=CARTESIAN_POINT('Ctrl Pts',(3.42864616361875,-1.,-1.51893924967331));
#35405=CARTESIAN_POINT('Ctrl Pts',(3.42859860294305,-1.,-1.5189508286633));
#35406=CARTESIAN_POINT('',(3.49844575334386,-1.,-1.35032489087269));
#35407=CARTESIAN_POINT('Origin',(0.,-1.,0.));
#35408=CARTESIAN_POINT('',(3.97027773754922,-1.,-1.36999806084572));
#35409=CARTESIAN_POINT('Ctrl Pts',(3.49844575334386,-1.,-1.35032489087269));
#35410=CARTESIAN_POINT('Ctrl Pts',(3.49847119623841,-1.,-1.35036670893102));
#35411=CARTESIAN_POINT('Ctrl Pts',(3.49861894124915,-1.,-1.35049736560633));
#35412=CARTESIAN_POINT('Ctrl Pts',(3.49920025459856,-1.,-1.35080045218652));
#35413=CARTESIAN_POINT('Ctrl Pts',(3.5007660381658,-1.,-1.35142377279535));
#35414=CARTESIAN_POINT('Ctrl Pts',(3.50408168106113,-1.,-1.3525703284343));
#35415=CARTESIAN_POINT('Ctrl Pts',(3.50913227060177,-1.,-1.35419113576022));
#35416=CARTESIAN_POINT('Ctrl Pts',(3.51542230699919,-1.,-1.35611275237288));
#35417=CARTESIAN_POINT('Ctrl Pts',(3.52261776117121,-1.,-1.35821701528975));
#35418=CARTESIAN_POINT('Ctrl Pts',(3.53034464961849,-1.,-1.36037259643827));
#35419=CARTESIAN_POINT('Ctrl Pts',(3.53824396425032,-1.,-1.36245507339334));
#35420=CARTESIAN_POINT('Ctrl Pts',(3.54602591832893,-1.,-1.36436666257568));
#35421=CARTESIAN_POINT('Ctrl Pts',(3.55353883995793,-1.,-1.36606145456711));
#35422=CARTESIAN_POINT('Ctrl Pts',(3.56077662028492,-1.,-1.36754771771174));
#35423=CARTESIAN_POINT('Ctrl Pts',(3.56782080304554,-1.,-1.36886584973349));
#35424=CARTESIAN_POINT('Ctrl Pts',(3.57479875549453,-1.,-1.37007229485646));
#35425=CARTESIAN_POINT('Ctrl Pts',(3.58183885982745,-1.,-1.37122241663073));
#35426=CARTESIAN_POINT('Ctrl Pts',(3.5890185384643,-1.,-1.37235053661));
#35427=CARTESIAN_POINT('Ctrl Pts',(3.59634627869117,-1.,-1.37346320103184));
#35428=CARTESIAN_POINT('Ctrl Pts',(3.60379020124038,-1.,-1.37455051379642));
#35429=CARTESIAN_POINT('Ctrl Pts',(3.61129546591082,-1.,-1.37559314436641));
#35430=CARTESIAN_POINT('Ctrl Pts',(3.61880481160408,-1.,-1.37657053403102));
#35431=CARTESIAN_POINT('Ctrl Pts',(3.62628098665112,-1.,-1.37746987919868));
#35432=CARTESIAN_POINT('Ctrl Pts',(3.63371727442448,-1.,-1.37829035457325));
#35433=CARTESIAN_POINT('Ctrl Pts',(3.64112507791112,-1.,-1.37903818567347));
#35434=CARTESIAN_POINT('Ctrl Pts',(3.64852652756444,-1.,-1.37972372481598));
#35435=CARTESIAN_POINT('Ctrl Pts',(3.65594554404396,-1.,-1.38035791051215));
#35436=CARTESIAN_POINT('Ctrl Pts',(3.66339848520874,-1.,-1.38094856333558));
#35437=CARTESIAN_POINT('Ctrl Pts',(3.67088843112282,-1.,-1.38149812653876));
#35438=CARTESIAN_POINT('Ctrl Pts',(3.6784103848243,-1.,-1.38200574290626));
#35439=CARTESIAN_POINT('Ctrl Pts',(3.68595444983844,-1.,-1.38246852827185));
#35440=CARTESIAN_POINT('Ctrl Pts',(3.69350967899523,-1.,-1.38288311171649));
#35441=CARTESIAN_POINT('Ctrl Pts',(3.70106792167894,-1.,-1.38324717612862));
#35442=CARTESIAN_POINT('Ctrl Pts',(3.70862680753343,-1.,-1.38356065402122));
#35443=CARTESIAN_POINT('Ctrl Pts',(3.7161876605181,-1.,-1.38382489984585));
#35444=CARTESIAN_POINT('Ctrl Pts',(3.72375409358805,-1.,-1.3840421342895));
#35445=CARTESIAN_POINT('Ctrl Pts',(3.73133035859283,-1.,-1.38421479111531));
#35446=CARTESIAN_POINT('Ctrl Pts',(3.73891976418099,-1.,-1.38434489156456));
#35447=CARTESIAN_POINT('Ctrl Pts',(3.7465231716786,-1.,-1.38443344984389));
#35448=CARTESIAN_POINT('Ctrl Pts',(3.75413976318727,-1.,-1.38448077997155));
#35449=CARTESIAN_POINT('Ctrl Pts',(3.76176768271347,-1.,-1.38448675253343));
#35450=CARTESIAN_POINT('Ctrl Pts',(3.76940473185775,-1.,-1.38445107339517));
#35451=CARTESIAN_POINT('Ctrl Pts',(3.77704902230441,-1.,-1.38437354551435));
#35452=CARTESIAN_POINT('Ctrl Pts',(3.78469969805134,-1.,-1.38425435883773));
#35453=CARTESIAN_POINT('Ctrl Pts',(3.79235669640907,-1.,-1.38409399694589));
#35454=CARTESIAN_POINT('Ctrl Pts',(3.80002044322169,-1.,-1.38389311766701));
#35455=CARTESIAN_POINT('Ctrl Pts',(3.80769156398429,-1.,-1.38365244046226));
#35456=CARTESIAN_POINT('Ctrl Pts',(3.81537060817765,-1.,-1.38337263902766));
#35457=CARTESIAN_POINT('Ctrl Pts',(3.82305771743715,-1.,-1.38305421262724));
#35458=CARTESIAN_POINT('Ctrl Pts',(3.83075266982138,-1.,-1.38269750245086));
#35459=CARTESIAN_POINT('Ctrl Pts',(3.83845502790609,-1.,-1.38230274828774));
#35460=CARTESIAN_POINT('Ctrl Pts',(3.84616425605705,-1.,-1.38187013346089));
#35461=CARTESIAN_POINT('Ctrl Pts',(3.85387983979557,-1.,-1.38139983115075));
#35462=CARTESIAN_POINT('Ctrl Pts',(3.86160143044187,-1.,-1.38089205993068));
#35463=CARTESIAN_POINT('Ctrl Pts',(3.86932885813403,-1.,-1.38034709213129));
#35464=CARTESIAN_POINT('Ctrl Pts',(3.87706205830865,-1.,-1.37976523097187));
#35465=CARTESIAN_POINT('Ctrl Pts',(3.88480102249461,-1.,-1.37914679719446));
#35466=CARTESIAN_POINT('Ctrl Pts',(3.89254574338385,-1.,-1.37849211287981));
#35467=CARTESIAN_POINT('Ctrl Pts',(3.90029615196255,-1.,-1.3778014851263));
#35468=CARTESIAN_POINT('Ctrl Pts',(3.90805209522729,-1.,-1.3770751963376));
#35469=CARTESIAN_POINT('Ctrl Pts',(3.91581337461825,-1.,-1.37631350505516));
#35470=CARTESIAN_POINT('Ctrl Pts',(3.92357976987132,-1.,-1.37551664448057));
#35471=CARTESIAN_POINT('Ctrl Pts',(3.93135106761941,-1.,-1.37468482215784));
#35472=CARTESIAN_POINT('Ctrl Pts',(3.93912709041791,-1.,-1.37381821967499));
#35473=CARTESIAN_POINT('Ctrl Pts',(3.94690771786926,-1.,-1.37291699203423));
#35474=CARTESIAN_POINT('Ctrl Pts',(3.95469287283105,-1.,-1.37198126433139));
#35475=CARTESIAN_POINT('Ctrl Pts',(3.96092458508407,-1.,-1.37120515615663));
#35476=CARTESIAN_POINT('Ctrl Pts',(3.96560037975788,-1.,-1.37060761746027));
#35477=CARTESIAN_POINT('Ctrl Pts',(3.9687184694173,-1.,-1.37020239094758));
#35478=CARTESIAN_POINT('Ctrl Pts',(3.97027773754922,-1.,-1.36999806084572));
#35479=CARTESIAN_POINT('',(4.01728681790024,-1.,-1.22531898815164));
#35480=CARTESIAN_POINT('',(3.97027773754922,-1.,-1.36999806084572));
#35481=CARTESIAN_POINT('',(3.62400312501199,-1.,-0.963899035118986));
#35482=CARTESIAN_POINT('Ctrl Pts',(4.01728681790024,-1.,-1.22531898815164));
#35483=CARTESIAN_POINT('Ctrl Pts',(4.01614544569895,-1.,-1.22423716681317));
#35484=CARTESIAN_POINT('Ctrl Pts',(4.01386104433519,-1.,-1.22207656455845));
#35485=CARTESIAN_POINT('Ctrl Pts',(4.01042947140789,-1.,-1.21884478244403));
#35486=CARTESIAN_POINT('Ctrl Pts',(4.00584409522722,-1.,-1.21455398918133));
#35487=CARTESIAN_POINT('Ctrl Pts',(4.00009577950721,-1.,-1.20922097029551));
#35488=CARTESIAN_POINT('Ctrl Pts',(3.99433084799666,-1.,-1.20391852375139));
#35489=CARTESIAN_POINT('Ctrl Pts',(3.98854928957189,-1.,-1.19864679609566));
#35490=CARTESIAN_POINT('Ctrl Pts',(3.98275111052561,-1.,-1.19340598349475));
#35491=CARTESIAN_POINT('Ctrl Pts',(3.97693634767754,-1.,-1.18819633715539));
#35492=CARTESIAN_POINT('Ctrl Pts',(3.97110505165415,-1.,-1.18301815039831));
#35493=CARTESIAN_POINT('Ctrl Pts',(3.96525726358159,-1.,-1.17787174135592));
#35494=CARTESIAN_POINT('Ctrl Pts',(3.95939299213276,-1.,-1.17275743590361));
#35495=CARTESIAN_POINT('Ctrl Pts',(3.95351219509876,-1.,-1.16767555244438));
#35496=CARTESIAN_POINT('Ctrl Pts',(3.94761474780583,-1.,-1.16262637999157));
#35497=CARTESIAN_POINT('Ctrl Pts',(3.94170046685203,-1.,-1.15761018340956));
#35498=CARTESIAN_POINT('Ctrl Pts',(3.9357691705628,-1.,-1.1526272271632));
#35499=CARTESIAN_POINT('Ctrl Pts',(3.92982073294257,-1.,-1.14767779451124));
#35500=CARTESIAN_POINT('Ctrl Pts',(3.92385513133997,-1.,-1.14276220561593));
#35501=CARTESIAN_POINT('Ctrl Pts',(3.91787251936827,-1.,-1.13788084225554));
#35502=CARTESIAN_POINT('Ctrl Pts',(3.91187321145649,-1.,-1.13303414693896));
#35503=CARTESIAN_POINT('Ctrl Pts',(3.90585753318737,-1.,-1.12822258281553));
#35504=CARTESIAN_POINT('Ctrl Pts',(3.89982569750025,-1.,-1.12344660099043));
#35505=CARTESIAN_POINT('Ctrl Pts',(3.89377768340344,-1.,-1.11870660794603));
#35506=CARTESIAN_POINT('Ctrl Pts',(3.88771308285171,-1.,-1.11400292434429));
#35507=CARTESIAN_POINT('Ctrl Pts',(3.88163105531724,-1.,-1.10933577224008));
#35508=CARTESIAN_POINT('Ctrl Pts',(3.87553067187514,-1.,-1.10470536603287));
#35509=CARTESIAN_POINT('Ctrl Pts',(3.86941120134849,-1.,-1.10011198761195));
#35510=CARTESIAN_POINT('Ctrl Pts',(3.86327241021247,-1.,-1.09555606505013));
#35511=CARTESIAN_POINT('Ctrl Pts',(3.85711487933931,-1.,-1.09103825516294));
#35512=CARTESIAN_POINT('Ctrl Pts',(3.85094025222713,-1.,-1.08655950846384));
#35513=CARTESIAN_POINT('Ctrl Pts',(3.8447504803063,-1.,-1.08212087917991));
#35514=CARTESIAN_POINT('Ctrl Pts',(3.83854714117491,-1.,-1.07772335353858));
#35515=CARTESIAN_POINT('Ctrl Pts',(3.83233071195144,-1.,-1.07336766633459));
#35516=CARTESIAN_POINT('Ctrl Pts',(3.82609989967276,-1.,-1.06905413180359));
#35517=CARTESIAN_POINT('Ctrl Pts',(3.81985083953012,-1.,-1.0647824403893));
#35518=CARTESIAN_POINT('Ctrl Pts',(3.8135786611749,-1.,-1.06055206187299));
#35519=CARTESIAN_POINT('Ctrl Pts',(3.80727913637791,-1.,-1.05636266918644));
#35520=CARTESIAN_POINT('Ctrl Pts',(3.80095039790681,-1.,-1.05221457990016));
#35521=CARTESIAN_POINT('Ctrl Pts',(3.79459440308786,-1.,-1.04810913267639));
#35522=CARTESIAN_POINT('Ctrl Pts',(3.78821910787179,-1.,-1.04404924374422));
#35523=CARTESIAN_POINT('Ctrl Pts',(3.7818353500817,-1.,-1.04003862055798));
#35524=CARTESIAN_POINT('Ctrl Pts',(3.77545283140427,-1.,-1.03608074678008));
#35525=CARTESIAN_POINT('Ctrl Pts',(3.76907609832516,-1.,-1.03217786604919));
#35526=CARTESIAN_POINT('Ctrl Pts',(3.76270122291245,-1.,-1.02833014458184));
#35527=CARTESIAN_POINT('Ctrl Pts',(3.75631037456224,-1.,-1.02453429444668));
#35528=CARTESIAN_POINT('Ctrl Pts',(3.74987777155873,-1.,-1.02078510487439));
#35529=CARTESIAN_POINT('Ctrl Pts',(3.74337942504993,-1.,-1.01707794311088));
#35530=CARTESIAN_POINT('Ctrl Pts',(3.73680245055747,-1.,-1.01341114319906));
#35531=CARTESIAN_POINT('Ctrl Pts',(3.73015276704407,-1.,-1.00978798539491));
#35532=CARTESIAN_POINT('Ctrl Pts',(3.72346803750544,-1.,-1.00622000735696));
#35533=CARTESIAN_POINT('Ctrl Pts',(3.71680667125047,-1.,-1.00272423396802));
#35534=CARTESIAN_POINT('Ctrl Pts',(3.7102243971387,-1.,-0.999317260756345));
#35535=CARTESIAN_POINT('Ctrl Pts',(3.70375282282107,-1.,-0.996009819772432));
#35536=CARTESIAN_POINT('Ctrl Pts',(3.69738123415696,-1.,-0.992802218332104));
#35537=CARTESIAN_POINT('Ctrl Pts',(3.69102682138955,-1.,-0.989676715398859));
#35538=CARTESIAN_POINT('Ctrl Pts',(3.6845531792623,-1.,-0.986602639864286));
#35539=CARTESIAN_POINT('Ctrl Pts',(3.67782408841876,-1.,-0.983550791470865));
#35540=CARTESIAN_POINT('Ctrl Pts',(3.67074983340444,-1.,-0.980505922458495));
#35541=CARTESIAN_POINT('Ctrl Pts',(3.66333049637403,-1.,-0.977478312751416));
#35542=CARTESIAN_POINT('Ctrl Pts',(3.6557157673487,-1.,-0.974519971354139));
#35543=CARTESIAN_POINT('Ctrl Pts',(3.64819756447072,-1.,-0.971722122060278));
#35544=CARTESIAN_POINT('Ctrl Pts',(3.64113946505393,-1.,-0.969195124674829));
#35545=CARTESIAN_POINT('Ctrl Pts',(3.6349212208096,-1.,-0.967052554540878));
#35546=CARTESIAN_POINT('Ctrl Pts',(3.62988252139998,-1.,-0.965395153165716));
#35547=CARTESIAN_POINT('Ctrl Pts',(3.62652618145252,-1.,-0.964373850166081));
#35548=CARTESIAN_POINT('Ctrl Pts',(3.62489305727516,-1.,-0.963957782642589));
#35549=CARTESIAN_POINT('Ctrl Pts',(3.62424461507455,-1.,-0.963861297423579));
#35550=CARTESIAN_POINT('Ctrl Pts',(3.62404828878374,-1.,-0.963880158556713));
#35551=CARTESIAN_POINT('Ctrl Pts',(3.62400312501199,-1.,-0.963899035118986));
#35552=CARTESIAN_POINT('',(3.66661143271648,-1.,-0.786422660833743));
#35553=CARTESIAN_POINT('Origin',(0.,-1.,0.));
#35554=CARTESIAN_POINT('',(4.13571194405636,-1.,-0.73204283740062));
#35555=CARTESIAN_POINT('Ctrl Pts',(3.66661143271648,-1.,-0.786422660833743));
#35556=CARTESIAN_POINT('Ctrl Pts',(3.66664310415236,-1.,-0.786459983896781));
#35557=CARTESIAN_POINT('Ctrl Pts',(3.66680946938396,-1.,-0.78656591955989));
#35558=CARTESIAN_POINT('Ctrl Pts',(3.66743103898844,-1.,-0.7867743371985));
#35559=CARTESIAN_POINT('Ctrl Pts',(3.66907505398769,-1.,-0.787145041181589));
#35560=CARTESIAN_POINT('Ctrl Pts',(3.672529236635,-1.,-0.787758799995427));
#35561=CARTESIAN_POINT('Ctrl Pts',(3.67777119516438,-1.,-0.788569566220663));
#35562=CARTESIAN_POINT('Ctrl Pts',(3.68428439784285,-1.,-0.789483546065159));
#35563=CARTESIAN_POINT('Ctrl Pts',(3.69172044327754,-1.,-0.79043628498958));
#35564=CARTESIAN_POINT('Ctrl Pts',(3.69968940808982,-1.,-0.791356575696509));
#35565=CARTESIAN_POINT('Ctrl Pts',(3.70781724021879,-1.,-0.792177688845968));
#35566=CARTESIAN_POINT('Ctrl Pts',(3.7158024239604,-1.,-0.792848377370116));
#35567=CARTESIAN_POINT('Ctrl Pts',(3.7234879729357,-1.,-0.793347023783871));
#35568=CARTESIAN_POINT('Ctrl Pts',(3.7308691469564,-1.,-0.793682750269348));
#35569=CARTESIAN_POINT('Ctrl Pts',(3.73803280541576,-1.,-0.793882700936791));
#35570=CARTESIAN_POINT('Ctrl Pts',(3.74511357728827,-1.,-0.79398270045988));
#35571=CARTESIAN_POINT('Ctrl Pts',(3.75224692493895,-1.,-0.794017347371441));
#35572=CARTESIAN_POINT('Ctrl Pts',(3.75951468666325,-1.,-0.794008429135047));
#35573=CARTESIAN_POINT('Ctrl Pts',(3.76692626931184,-1.,-0.793961083689141));
#35574=CARTESIAN_POINT('Ctrl Pts',(3.77444863801264,-1.,-0.793870523787515));
#35575=CARTESIAN_POINT('Ctrl Pts',(3.78202460377617,-1.,-0.79372623578134));
#35576=CARTESIAN_POINT('Ctrl Pts',(3.78959439439222,-1.,-0.793516871680966));
#35577=CARTESIAN_POINT('Ctrl Pts',(3.79711921389862,-1.,-0.793235612973201));
#35578=CARTESIAN_POINT('Ctrl Pts',(3.80459229925598,-1.,-0.792882695234693));
#35579=CARTESIAN_POINT('Ctrl Pts',(3.81202588694726,-1.,-0.792462483517568));
#35580=CARTESIAN_POINT('Ctrl Pts',(3.81944345442237,-1.,-0.791981740718607));
#35581=CARTESIAN_POINT('Ctrl Pts',(3.82687033899799,-1.,-0.791447528662381));
#35582=CARTESIAN_POINT('Ctrl Pts',(3.83432392054804,-1.,-0.79086501270534));
#35583=CARTESIAN_POINT('Ctrl Pts',(3.84180762342476,-1.,-0.790236124191289));
#35584=CARTESIAN_POINT('Ctrl Pts',(3.8493163780891,-1.,-0.789560798155619));
#35585=CARTESIAN_POINT('Ctrl Pts',(3.85683995872536,-1.,-0.788837734090688));
#35586=CARTESIAN_POINT('Ctrl Pts',(3.86436702561342,-1.,-0.788065315093771));
#35587=CARTESIAN_POINT('Ctrl Pts',(3.87188916600905,-1.,-0.787242527617981));
#35588=CARTESIAN_POINT('Ctrl Pts',(3.87940402818186,-1.,-0.786369675812592));
#35589=CARTESIAN_POINT('Ctrl Pts',(3.88691313167399,-1.,-0.785447890340723));
#35590=CARTESIAN_POINT('Ctrl Pts',(3.89442039235105,-1.,-0.784478799358336));
#35591=CARTESIAN_POINT('Ctrl Pts',(3.90193039043971,-1.,-0.783464141529083));
#35592=CARTESIAN_POINT('Ctrl Pts',(3.90944671004536,-1.,-0.782405395622759));
#35593=CARTESIAN_POINT('Ctrl Pts',(3.9169703605466,-1.,-0.781303428618344));
#35594=CARTESIAN_POINT('Ctrl Pts',(3.92450058323799,-1.,-0.780158678615507));
#35595=CARTESIAN_POINT('Ctrl Pts',(3.93203552473153,-1.,-0.778971308134786));
#35596=CARTESIAN_POINT('Ctrl Pts',(3.93957296768098,-1.,-0.77774137056855));
#35597=CARTESIAN_POINT('Ctrl Pts',(3.94711101619471,-1.,-0.77646896669796));
#35598=CARTESIAN_POINT('Ctrl Pts',(3.95464885452364,-1.,-0.775154418039442));
#35599=CARTESIAN_POINT('Ctrl Pts',(3.96218649639876,-1.,-0.773798212026683));
#35600=CARTESIAN_POINT('Ctrl Pts',(3.96972446532832,-1.,-0.772400931772239));
#35601=CARTESIAN_POINT('Ctrl Pts',(3.97726349165507,-1.,-0.770963190030504));
#35602=CARTESIAN_POINT('Ctrl Pts',(3.98480422348403,-1.,-0.76948556624546));
#35603=CARTESIAN_POINT('Ctrl Pts',(3.99234687880892,-1.,-0.767968531377708));
#35604=CARTESIAN_POINT('Ctrl Pts',(3.99989129179464,-1.,-0.766412457135786));
#35605=CARTESIAN_POINT('Ctrl Pts',(4.00743706791366,-1.,-0.764817648784947));
#35606=CARTESIAN_POINT('Ctrl Pts',(4.01498370680434,-1.,-0.763184371182827));
#35607=CARTESIAN_POINT('Ctrl Pts',(4.02253072741347,-1.,-0.761512875859942));
#35608=CARTESIAN_POINT('Ctrl Pts',(4.0300778195465,-1.,-0.759803433244166));
#35609=CARTESIAN_POINT('Ctrl Pts',(4.03762485803468,-1.,-0.758056338885554));
#35610=CARTESIAN_POINT('Ctrl Pts',(4.04517182654344,-1.,-0.756271902370187));
#35611=CARTESIAN_POINT('Ctrl Pts',(4.05271876688106,-1.,-0.754450441816412));
#35612=CARTESIAN_POINT('Ctrl Pts',(4.06026572221399,-1.,-0.752592276482869));
#35613=CARTESIAN_POINT('Ctrl Pts',(4.06781267241886,-1.,-0.750697720483176));
#35614=CARTESIAN_POINT('Ctrl Pts',(4.07535951055363,-1.,-0.748767076679177));
#35615=CARTESIAN_POINT('Ctrl Pts',(4.08290608094789,-1.,-0.746800631490822));
#35616=CARTESIAN_POINT('Ctrl Pts',(4.09045220253011,-1.,-0.744798649705514));
#35617=CARTESIAN_POINT('Ctrl Pts',(4.09799769702712,-1.,-0.742761369690018));
#35618=CARTESIAN_POINT('Ctrl Pts',(4.1055424175856,-1.,-0.740688998555152));
#35619=CARTESIAN_POINT('Ctrl Pts',(4.11308626953795,-1.,-0.738581708229119));
#35620=CARTESIAN_POINT('Ctrl Pts',(4.12062919626082,-1.,-0.736439634335347));
#35621=CARTESIAN_POINT('Ctrl Pts',(4.12666277572794,-1.,-0.734698226767513));
#35622=CARTESIAN_POINT('Ctrl Pts',(4.13118752796397,-1.,-0.733376589325634));
#35623=CARTESIAN_POINT('Ctrl Pts',(4.13420383737278,-1.,-0.732488575135926));
#35624=CARTESIAN_POINT('Ctrl Pts',(4.13571194405636,-1.,-0.73204283740062));
#35625=CARTESIAN_POINT('',(4.15950947128175,-1.,-0.581791163835815));
#35626=CARTESIAN_POINT('',(4.13571194405636,-1.,-0.73204283740062));
#35627=CARTESIAN_POINT('',(3.73017266276632,-1.,-0.385112848332549));
#35628=CARTESIAN_POINT('Ctrl Pts',(4.15950947128175,-1.,-0.581791163835815));
#35629=CARTESIAN_POINT('Ctrl Pts',(4.15821291712391,-1.,-0.580901211462913));
#35630=CARTESIAN_POINT('Ctrl Pts',(4.15561864787379,-1.,-0.579124568912544));
#35631=CARTESIAN_POINT('Ctrl Pts',(4.1517237611974,-1.,-0.576469391673917));
#35632=CARTESIAN_POINT('Ctrl Pts',(4.14652361065787,-1.,-0.572948736066277));
#35633=CARTESIAN_POINT('Ctrl Pts',(4.14001179828669,-1.,-0.568580610187116));
#35634=CARTESIAN_POINT('Ctrl Pts',(4.13348835726086,-1.,-0.564245279535706));
#35635=CARTESIAN_POINT('Ctrl Pts',(4.12695329951859,-1.,-0.559942890594628));
#35636=CARTESIAN_POINT('Ctrl Pts',(4.1204066619623,-1.,-0.555673636130778));
#35637=CARTESIAN_POINT('Ctrl Pts',(4.11384852025578,-1.,-0.551437758498247));
#35638=CARTESIAN_POINT('Ctrl Pts',(4.1072789702877,-1.,-0.54723553948676));
#35639=CARTESIAN_POINT('Ctrl Pts',(4.10069810244473,-1.,-0.543067286878457));
#35640=CARTESIAN_POINT('Ctrl Pts',(4.09410597627116,-1.,-0.538933321179921));
#35641=CARTESIAN_POINT('Ctrl Pts',(4.08750259988693,-1.,-0.534833963477));
#35642=CARTESIAN_POINT('Ctrl Pts',(4.08088789536488,-1.,-0.530769518728076));
#35643=CARTESIAN_POINT('Ctrl Pts',(4.07426172299496,-1.,-0.526740277227));
#35644=CARTESIAN_POINT('Ctrl Pts',(4.06762394471075,-1.,-0.522746528602768));
#35645=CARTESIAN_POINT('Ctrl Pts',(4.06097448037934,-1.,-0.51878857233681));
#35646=CARTESIAN_POINT('Ctrl Pts',(4.05431335771261,-1.,-0.514866728193104));
#35647=CARTESIAN_POINT('Ctrl Pts',(4.04764078815591,-1.,-0.510981349219174));
#35648=CARTESIAN_POINT('Ctrl Pts',(4.04095715149074,-1.,-0.507132823288362));
#35649=CARTESIAN_POINT('Ctrl Pts',(4.0342628417439,-1.,-0.503321556915514));
#35650=CARTESIAN_POINT('Ctrl Pts',(4.0275581398015,-1.,-0.49954796234089));
#35651=CARTESIAN_POINT('Ctrl Pts',(4.02084308851813,-1.,-0.495812444326223));
#35652=CARTESIAN_POINT('Ctrl Pts',(4.01411733503486,-1.,-0.492115383417931));
#35653=CARTESIAN_POINT('Ctrl Pts',(4.0073800839092,-1.,-0.488457130424531));
#35654=CARTESIAN_POINT('Ctrl Pts',(4.00063045119234,-1.,-0.484838042421754));
#35655=CARTESIAN_POINT('Ctrl Pts',(3.99386775880655,-1.,-0.481258512209638));
#35656=CARTESIAN_POINT('Ctrl Pts',(3.98709184306743,-1.,-0.477718999122033));
#35657=CARTESIAN_POINT('Ctrl Pts',(3.9803033804443,-1.,-0.474220061019542));
#35658=CARTESIAN_POINT('Ctrl Pts',(3.97350414289415,-1.,-0.470762379613478));
#35659=CARTESIAN_POINT('Ctrl Pts',(3.96669622273946,-1.,-0.467346690880672));
#35660=CARTESIAN_POINT('Ctrl Pts',(3.95988133243543,-1.,-0.463973722115745));
#35661=CARTESIAN_POINT('Ctrl Pts',(3.95306005817363,-1.,-0.460644124429119));
#35662=CARTESIAN_POINT('Ctrl Pts',(3.94623117206675,-1.,-0.457358410451674));
#35663=CARTESIAN_POINT('Ctrl Pts',(3.93939080846298,-1.,-0.454116879027576));
#35664=CARTESIAN_POINT('Ctrl Pts',(3.93253407403128,-1.,-0.450919768356347));
#35665=CARTESIAN_POINT('Ctrl Pts',(3.92565674143424,-1.,-0.447767416837297));
#35666=CARTESIAN_POINT('Ctrl Pts',(3.91875701610721,-1.,-0.444660430230593));
#35667=CARTESIAN_POINT('Ctrl Pts',(3.91183704069146,-1.,-0.441599824524048));
#35668=CARTESIAN_POINT('Ctrl Pts',(3.90490512938546,-1.,-0.438587235458234));
#35669=CARTESIAN_POINT('Ctrl Pts',(3.8979725665544,-1.,-0.435624629433506));
#35670=CARTESIAN_POINT('Ctrl Pts',(3.89104947940592,-1.,-0.43271392954444));
#35671=CARTESIAN_POINT('Ctrl Pts',(3.88414070943334,-1.,-0.429856640579734));
#35672=CARTESIAN_POINT('Ctrl Pts',(3.87724240306609,-1.,-0.427053541173469));
#35673=CARTESIAN_POINT('Ctrl Pts',(3.87033643487882,-1.,-0.424304173195143));
#35674=CARTESIAN_POINT('Ctrl Pts',(3.86339652542749,-1.,-0.421607423177576));
#35675=CARTESIAN_POINT('Ctrl Pts',(3.85639825648031,-1.,-0.41896246808681));
#35676=CARTESIAN_POINT('Ctrl Pts',(3.8493286415751,-1.,-0.41636967805292));
#35677=CARTESIAN_POINT('Ctrl Pts',(3.84219403994742,-1.,-0.413831367016727));
#35678=CARTESIAN_POINT('Ctrl Pts',(3.83503345578645,-1.,-0.41135303879846));
#35679=CARTESIAN_POINT('Ctrl Pts',(3.82790724256397,-1.,-0.408942371447377));
#35680=CARTESIAN_POINT('Ctrl Pts',(3.82087303913741,-1.,-0.406607038258907));
#35681=CARTESIAN_POINT('Ctrl Pts',(3.81396374287762,-1.,-0.404352694628237));
#35682=CARTESIAN_POINT('Ctrl Pts',(3.80716881962763,-1.,-0.402181320148475));
#35683=CARTESIAN_POINT('Ctrl Pts',(3.80040370384659,-1.,-0.400088346504727));
#35684=CARTESIAN_POINT('Ctrl Pts',(3.79352887163457,-1.,-0.398064818684159));
#35685=CARTESIAN_POINT('Ctrl Pts',(3.78640521279479,-1.,-0.396103205335029));
#35686=CARTESIAN_POINT('Ctrl Pts',(3.77894173114368,-1.,-0.394202481011595));
#35687=CARTESIAN_POINT('Ctrl Pts',(3.77114011595892,-1.,-0.392372786223347));
#35688=CARTESIAN_POINT('Ctrl Pts',(3.76315635032993,-1.,-0.390642072979259));
#35689=CARTESIAN_POINT('Ctrl Pts',(3.75529302894757,-1.,-0.389054775898251));
#35690=CARTESIAN_POINT('Ctrl Pts',(3.74792651696269,-1.,-0.387663020050396));
#35691=CARTESIAN_POINT('Ctrl Pts',(3.74144965781088,-1.,-0.386519576222036));
#35692=CARTESIAN_POINT('Ctrl Pts',(3.73621371845475,-1.,-0.385670806454744));
#35693=CARTESIAN_POINT('Ctrl Pts',(3.73273893363318,-1.,-0.385187124633965));
#35694=CARTESIAN_POINT('Ctrl Pts',(3.73106082862399,-1.,-0.385031656499142));
#35695=CARTESIAN_POINT('Ctrl Pts',(3.73040527620929,-1.,-0.385037797882046));
#35696=CARTESIAN_POINT('Ctrl Pts',(3.73021431755218,-1.,-0.385087139001609));
#35697=CARTESIAN_POINT('Ctrl Pts',(3.73017266276632,-1.,-0.385112848332549));
#35698=CARTESIAN_POINT('',(3.74449296982994,-1.,-0.203156094897896));
#35699=CARTESIAN_POINT('Origin',(0.,-1.,0.));
#35700=CARTESIAN_POINT('',(4.19931119685982,-1.,-0.0760622897878241));
#35701=CARTESIAN_POINT('Ctrl Pts',(3.74449296982994,-1.,-0.203156094897896));
#35702=CARTESIAN_POINT('Ctrl Pts',(3.74453008995129,-1.,-0.203188003947965));
#35703=CARTESIAN_POINT('Ctrl Pts',(3.74471097893961,-1.,-0.203266610111264));
#35704=CARTESIAN_POINT('Ctrl Pts',(3.74535749969262,-1.,-0.203375226874332));
#35705=CARTESIAN_POINT('Ctrl Pts',(3.74703926501843,-1.,-0.203484186269315));
#35706=CARTESIAN_POINT('Ctrl Pts',(3.75054693397716,-1.,-0.203550035479097));
#35707=CARTESIAN_POINT('Ctrl Pts',(3.75585118707924,-1.,-0.203530796848404));
#35708=CARTESIAN_POINT('Ctrl Pts',(3.76242717937273,-1.,-0.203414634707647));
#35709=CARTESIAN_POINT('Ctrl Pts',(3.76992071595267,-1.,-0.203192390045338));
#35710=CARTESIAN_POINT('Ctrl Pts',(3.77793553476879,-1.,-0.202854729699197));
#35711=CARTESIAN_POINT('Ctrl Pts',(3.78609175019317,-1.,-0.202394260512193));
#35712=CARTESIAN_POINT('Ctrl Pts',(3.79408354187274,-1.,-0.201807533800799));
#35713=CARTESIAN_POINT('Ctrl Pts',(3.80175247447171,-1.,-0.201097756307252));
#35714=CARTESIAN_POINT('Ctrl Pts',(3.80909529318501,-1.,-0.20027467943329));
#35715=CARTESIAN_POINT('Ctrl Pts',(3.81620203429702,-1.,-0.199351525297397));
#35716=CARTESIAN_POINT('Ctrl Pts',(3.82321127348981,-1.,-0.19834261690047));
#35717=CARTESIAN_POINT('Ctrl Pts',(3.83026221776488,-1.,-0.197260935827375));
#35718=CARTESIAN_POINT('Ctrl Pts',(3.83743910616265,-1.,-0.19611519897189));
#35719=CARTESIAN_POINT('Ctrl Pts',(3.84475203347052,-1.,-0.194909009460255));
#35720=CARTESIAN_POINT('Ctrl Pts',(3.85216762264019,-1.,-0.193642806777748));
#35721=CARTESIAN_POINT('Ctrl Pts',(3.85962774407652,-1.,-0.19231515304498));
#35722=CARTESIAN_POINT('Ctrl Pts',(3.8670715862477,-1.,-0.190924190418613));
#35723=CARTESIAN_POINT('Ctrl Pts',(3.87445976418377,-1.,-0.189469253358255));
#35724=CARTESIAN_POINT('Ctrl Pts',(3.88178563496187,-1.,-0.187951632512664));
#35725=CARTESIAN_POINT('Ctrl Pts',(3.88906196725817,-1.,-0.186373724985263));
#35726=CARTESIAN_POINT('Ctrl Pts',(3.89631300742633,-1.,-0.184738537728035));
#35727=CARTESIAN_POINT('Ctrl Pts',(3.90356488555138,-1.,-0.183049081993193));
#35728=CARTESIAN_POINT('Ctrl Pts',(3.91083557557193,-1.,-0.181307740731796));
#35729=CARTESIAN_POINT('Ctrl Pts',(3.91812876180948,-1.,-0.179515885822895));
#35730=CARTESIAN_POINT('Ctrl Pts',(3.92543942697672,-1.,-0.177674246152328));
#35731=CARTESIAN_POINT('Ctrl Pts',(3.93275726771049,-1.,-0.175783136893873));
#35732=CARTESIAN_POINT('Ctrl Pts',(3.94007083096214,-1.,-0.173842734974608));
#35733=CARTESIAN_POINT('Ctrl Pts',(3.94737164900861,-1.,-0.171853355369233));
#35734=CARTESIAN_POINT('Ctrl Pts',(3.95465744665263,-1.,-0.16981566637413));
#35735=CARTESIAN_POINT('Ctrl Pts',(3.96192990160296,-1.,-0.167730547023312));
#35736=CARTESIAN_POINT('Ctrl Pts',(3.9691931362141,-1.,-0.165598992851098));
#35737=CARTESIAN_POINT('Ctrl Pts',(3.97645194630944,-1.,-0.163422004609999));
#35738=CARTESIAN_POINT('Ctrl Pts',(3.98371010319866,-1.,-0.161200482186088));
#35739=CARTESIAN_POINT('Ctrl Pts',(3.99096873945862,-1.,-0.158935123982796));
#35740=CARTESIAN_POINT('Ctrl Pts',(3.99822717425869,-1.,-0.156626481393736));
#35741=CARTESIAN_POINT('Ctrl Pts',(4.00548360245297,-1.,-0.15427500487231));
#35742=CARTESIAN_POINT('Ctrl Pts',(4.01273584234684,-1.,-0.151881094022909));
#35743=CARTESIAN_POINT('Ctrl Pts',(4.01998203715588,-1.,-0.149445144968708));
#35744=CARTESIAN_POINT('Ctrl Pts',(4.02722143147048,-1.,-0.146967602878999));
#35745=CARTESIAN_POINT('Ctrl Pts',(4.03445411510403,-1.,-0.144448947038352));
#35746=CARTESIAN_POINT('Ctrl Pts',(4.04168069633842,-1.,-0.141889671485508));
#35747=CARTESIAN_POINT('Ctrl Pts',(4.04890199238056,-1.,-0.13929026718006));
#35748=CARTESIAN_POINT('Ctrl Pts',(4.05611873400122,-1.,-0.136651205046111));
#35749=CARTESIAN_POINT('Ctrl Pts',(4.06333121018476,-1.,-0.133972916144225));
#35750=CARTESIAN_POINT('Ctrl Pts',(4.07053931528579,-1.,-0.131255793548914));
#35751=CARTESIAN_POINT('Ctrl Pts',(4.07774270738809,-1.,-0.128500200484814));
#35752=CARTESIAN_POINT('Ctrl Pts',(4.08494093372315,-1.,-0.12570647682253));
#35753=CARTESIAN_POINT('Ctrl Pts',(4.09213355850836,-1.,-0.122874946249119));
#35754=CARTESIAN_POINT('Ctrl Pts',(4.09932031767243,-1.,-0.120005924388162));
#35755=CARTESIAN_POINT('Ctrl Pts',(4.10650113382187,-1.,-0.117099722731705));
#35756=CARTESIAN_POINT('Ctrl Pts',(4.11367603925313,-1.,-0.114156649609602));
#35757=CARTESIAN_POINT('Ctrl Pts',(4.12084512502444,-1.,-0.111177012683378));
#35758=CARTESIAN_POINT('Ctrl Pts',(4.12800848371386,-1.,-0.10816112052835));
#35759=CARTESIAN_POINT('Ctrl Pts',(4.13516614458396,-1.,-0.105109286538864));
#35760=CARTESIAN_POINT('Ctrl Pts',(4.14231804938737,-1.,-0.102021826577454));
#35761=CARTESIAN_POINT('Ctrl Pts',(4.1494640891762,-1.,-0.0988990478899816));
#35762=CARTESIAN_POINT('Ctrl Pts',(4.15660412653006,-1.,-0.0957412403297072));
#35763=CARTESIAN_POINT('Ctrl Pts',(4.16373802265942,-1.,-0.0925486672167695));
#35764=CARTESIAN_POINT('Ctrl Pts',(4.17086566491823,-1.,-0.0893215560850332));
#35765=CARTESIAN_POINT('Ctrl Pts',(4.17798698669991,-1.,-0.086060091555252));
#35766=CARTESIAN_POINT('Ctrl Pts',(4.1851019532944,-1.,-0.0827644164389515));
#35767=CARTESIAN_POINT('Ctrl Pts',(4.19078883322483,-1.,-0.0801005887117608));
#35768=CARTESIAN_POINT('Ctrl Pts',(4.19505112860624,-1.,-0.0780873956244407));
#35769=CARTESIAN_POINT('Ctrl Pts',(4.19789138621624,-1.,-0.07673845961422));
#35770=CARTESIAN_POINT('Ctrl Pts',(4.19931119685982,-1.,-0.0760622897878241));
#35771=CARTESIAN_POINT('',(4.19931119685982,-1.,0.0760622897878241));
#35772=CARTESIAN_POINT('',(4.19931119685982,-1.,-0.0760622897878241));
#35773=CARTESIAN_POINT('',(3.74449296983004,-1.,0.2031560948961));
#35774=CARTESIAN_POINT('Ctrl Pts',(4.19931119685982,-1.,0.0760622897878241));
#35775=CARTESIAN_POINT('Ctrl Pts',(4.1978913862118,-1.,0.0767384596141459));
#35776=CARTESIAN_POINT('Ctrl Pts',(4.19505112859416,-1.,0.0780873956242392));
#35777=CARTESIAN_POINT('Ctrl Pts',(4.19078883320504,-1.,0.0801005887114315));
#35778=CARTESIAN_POINT('Ctrl Pts',(4.18510195327123,-1.,0.0827644164385674));
#35779=CARTESIAN_POINT('Ctrl Pts',(4.17798698668094,-1.,0.0860600915549391));
#35780=CARTESIAN_POINT('Ctrl Pts',(4.17086566490794,-1.,0.0893215560848644));
#35781=CARTESIAN_POINT('Ctrl Pts',(4.16373802265839,-1.,0.0925486672167526));
#35782=CARTESIAN_POINT('Ctrl Pts',(4.15660412653577,-1.,0.0957412403298002));
#35783=CARTESIAN_POINT('Ctrl Pts',(4.14946408918485,-1.,0.0988990478901221));
#35784=CARTESIAN_POINT('Ctrl Pts',(4.14231804939538,-1.,0.102021826577583));
#35785=CARTESIAN_POINT('Ctrl Pts',(4.13516614458895,-1.,0.105109286538945));
#35786=CARTESIAN_POINT('Ctrl Pts',(4.12800848371504,-1.,0.108161120528369));
#35787=CARTESIAN_POINT('Ctrl Pts',(4.1208451250225,-1.,0.111177012683346));
#35788=CARTESIAN_POINT('Ctrl Pts',(4.11367603924961,-1.,0.114156649609545));
#35789=CARTESIAN_POINT('Ctrl Pts',(4.10650113381833,-1.,0.117099722731648));
#35790=CARTESIAN_POINT('Ctrl Pts',(4.09932031767002,-1.,0.120005924388124));
#35791=CARTESIAN_POINT('Ctrl Pts',(4.09213355850756,-1.,0.122874946249106));
#35792=CARTESIAN_POINT('Ctrl Pts',(4.08494093372377,-1.,0.125706476822539));
#35793=CARTESIAN_POINT('Ctrl Pts',(4.07774270738954,-1.,0.128500200484837));
#35794=CARTESIAN_POINT('Ctrl Pts',(4.0705393152874,-1.,0.13125579354894));
#35795=CARTESIAN_POINT('Ctrl Pts',(4.06333121018596,-1.,0.133972916144244));
#35796=CARTESIAN_POINT('Ctrl Pts',(4.05611873400172,-1.,0.136651205046119));
#35797=CARTESIAN_POINT('Ctrl Pts',(4.04890199238036,-1.,0.139290267180057));
#35798=CARTESIAN_POINT('Ctrl Pts',(4.04168069633781,-1.,0.1418896714855));
#35799=CARTESIAN_POINT('Ctrl Pts',(4.03445411510333,-1.,0.144448947038344));
#35800=CARTESIAN_POINT('Ctrl Pts',(4.02722143146994,-1.,0.146967602878994));
#35801=CARTESIAN_POINT('Ctrl Pts',(4.01998203715564,-1.,0.149445144968706));
#35802=CARTESIAN_POINT('Ctrl Pts',(4.01273584234689,-1.,0.15188109402291));
#35803=CARTESIAN_POINT('Ctrl Pts',(4.00548360245319,-1.,0.15427500487231));
#35804=CARTESIAN_POINT('Ctrl Pts',(3.99822717425893,-1.,0.156626481393734));
#35805=CARTESIAN_POINT('Ctrl Pts',(3.99096873945878,-1.,0.158935123982793));
#35806=CARTESIAN_POINT('Ctrl Pts',(3.98371010319872,-1.,0.161200482186084));
#35807=CARTESIAN_POINT('Ctrl Pts',(3.97645194630943,-1.,0.163422004609999));
#35808=CARTESIAN_POINT('Ctrl Pts',(3.96919313621407,-1.,0.165598992851102));
#35809=CARTESIAN_POINT('Ctrl Pts',(3.96192990160296,-1.,0.167730547023319));
#35810=CARTESIAN_POINT('Ctrl Pts',(3.95465744665268,-1.,0.169815666374138));
#35811=CARTESIAN_POINT('Ctrl Pts',(3.94737164900868,-1.,0.17185335536924));
#35812=CARTESIAN_POINT('Ctrl Pts',(3.94007083096217,-1.,0.173842734974609));
#35813=CARTESIAN_POINT('Ctrl Pts',(3.93275726771042,-1.,0.175783136893867));
#35814=CARTESIAN_POINT('Ctrl Pts',(3.92543942697655,-1.,0.177674246152317));
#35815=CARTESIAN_POINT('Ctrl Pts',(3.91812876180926,-1.,0.179515885822881));
#35816=CARTESIAN_POINT('Ctrl Pts',(3.91083557557175,-1.,0.181307740731785));
#35817=CARTESIAN_POINT('Ctrl Pts',(3.90356488555132,-1.,0.18304908199319));
#35818=CARTESIAN_POINT('Ctrl Pts',(3.89631300742646,-1.,0.184738537728042));
#35819=CARTESIAN_POINT('Ctrl Pts',(3.88906196725848,-1.,0.18637372498528));
#35820=CARTESIAN_POINT('Ctrl Pts',(3.88178563496228,-1.,0.187951632512684));
#35821=CARTESIAN_POINT('Ctrl Pts',(3.87445976418412,-1.,0.189469253358272));
#35822=CARTESIAN_POINT('Ctrl Pts',(3.86707158624783,-1.,0.190924190418619));
#35823=CARTESIAN_POINT('Ctrl Pts',(3.85962774407633,-1.,0.19231515304497));
#35824=CARTESIAN_POINT('Ctrl Pts',(3.85216762263966,-1.,0.193642806777722));
#35825=CARTESIAN_POINT('Ctrl Pts',(3.84475203346977,-1.,0.19490900946022));
#35826=CARTESIAN_POINT('Ctrl Pts',(3.83743910616195,-1.,0.196115198971858));
#35827=CARTESIAN_POINT('Ctrl Pts',(3.83026221776456,-1.,0.197260935827361));
#35828=CARTESIAN_POINT('Ctrl Pts',(3.82321127349016,-1.,0.198342616900486));
#35829=CARTESIAN_POINT('Ctrl Pts',(3.81620203429815,-1.,0.199351525297447));
#35830=CARTESIAN_POINT('Ctrl Pts',(3.80909529318669,-1.,0.200274679433364));
#35831=CARTESIAN_POINT('Ctrl Pts',(3.80175247447337,-1.,0.201097756307325));
#35832=CARTESIAN_POINT('Ctrl Pts',(3.7940835418736,-1.,0.201807533800837));
#35833=CARTESIAN_POINT('Ctrl Pts',(3.78609175019242,-1.,0.20239426051216));
#35834=CARTESIAN_POINT('Ctrl Pts',(3.77793553476614,-1.,0.20285472969908));
#35835=CARTESIAN_POINT('Ctrl Pts',(3.7699207159487,-1.,0.203192390045164));
#35836=CARTESIAN_POINT('Ctrl Pts',(3.76242717936885,-1.,0.203414634707478));
#35837=CARTESIAN_POINT('Ctrl Pts',(3.75585118707734,-1.,0.203530796848321));
#35838=CARTESIAN_POINT('Ctrl Pts',(3.75054693397875,-1.,0.203550035479166));
#35839=CARTESIAN_POINT('Ctrl Pts',(3.74703926501752,-1.,0.203484186269415));
#35840=CARTESIAN_POINT('Ctrl Pts',(3.74535749969115,-1.,0.203375226874121));
#35841=CARTESIAN_POINT('Ctrl Pts',(3.74471097893845,-1.,0.20326661011053));
#35842=CARTESIAN_POINT('Ctrl Pts',(3.74453008995092,-1.,0.203188003946656));
#35843=CARTESIAN_POINT('Ctrl Pts',(3.74449296983004,-1.,0.2031560948961));
#35844=CARTESIAN_POINT('',(3.73017266276651,-1.,0.385112848330762));
#35845=CARTESIAN_POINT('Origin',(0.,-1.,0.));
#35846=CARTESIAN_POINT('',(4.15950947128175,-1.,0.581791163835816));
#35847=CARTESIAN_POINT('Ctrl Pts',(3.73017266276651,-1.,0.385112848330762));
#35848=CARTESIAN_POINT('Ctrl Pts',(3.73021431755274,-1.,0.385087139000375));
#35849=CARTESIAN_POINT('Ctrl Pts',(3.73040527621055,-1.,0.385037797881504));
#35850=CARTESIAN_POINT('Ctrl Pts',(3.73106082862548,-1.,0.385031656499164));
#35851=CARTESIAN_POINT('Ctrl Pts',(3.73273893363406,-1.,0.385187124634207));
#35852=CARTESIAN_POINT('Ctrl Pts',(3.73621371845318,-1.,0.385670806454566));
#35853=CARTESIAN_POINT('Ctrl Pts',(3.74144965781276,-1.,0.386519576222252));
#35854=CARTESIAN_POINT('Ctrl Pts',(3.74792651696654,-1.,0.387663020050836));
#35855=CARTESIAN_POINT('Ctrl Pts',(3.75529302895152,-1.,0.389054775898702));
#35856=CARTESIAN_POINT('Ctrl Pts',(3.76315635033257,-1.,0.39064207297956));
#35857=CARTESIAN_POINT('Ctrl Pts',(3.77114011595967,-1.,0.392372786223433));
#35858=CARTESIAN_POINT('Ctrl Pts',(3.77894173114283,-1.,0.3942024810115));
#35859=CARTESIAN_POINT('Ctrl Pts',(3.78640521279313,-1.,0.396103205334841));
#35860=CARTESIAN_POINT('Ctrl Pts',(3.7935288716329,-1.,0.39806481868397));
#35861=CARTESIAN_POINT('Ctrl Pts',(3.80040370384546,-1.,0.400088346504601));
#35862=CARTESIAN_POINT('Ctrl Pts',(3.80716881962728,-1.,0.402181320148436));
#35863=CARTESIAN_POINT('Ctrl Pts',(3.81396374287793,-1.,0.404352694628274));
#35864=CARTESIAN_POINT('Ctrl Pts',(3.8208730391381,-1.,0.406607038258986));
#35865=CARTESIAN_POINT('Ctrl Pts',(3.82790724256471,-1.,0.40894237144746));
#35866=CARTESIAN_POINT('Ctrl Pts',(3.83503345578698,-1.,0.411353038798519));
#35867=CARTESIAN_POINT('Ctrl Pts',(3.84219403994762,-1.,0.413831367016748));
#35868=CARTESIAN_POINT('Ctrl Pts',(3.84932864157497,-1.,0.416369678052907));
#35869=CARTESIAN_POINT('Ctrl Pts',(3.85639825647996,-1.,0.418962468086773));
#35870=CARTESIAN_POINT('Ctrl Pts',(3.86339652542709,-1.,0.421607423177534));
#35871=CARTESIAN_POINT('Ctrl Pts',(3.87033643487851,-1.,0.424304173195111));
#35872=CARTESIAN_POINT('Ctrl Pts',(3.87724240306597,-1.,0.427053541173458));
#35873=CARTESIAN_POINT('Ctrl Pts',(3.88414070943341,-1.,0.429856640579741));
#35874=CARTESIAN_POINT('Ctrl Pts',(3.89104947940611,-1.,0.432713929544459));
#35875=CARTESIAN_POINT('Ctrl Pts',(3.89797256655462,-1.,0.435624629433528));
#35876=CARTESIAN_POINT('Ctrl Pts',(3.90490512938563,-1.,0.43858723545825));
#35877=CARTESIAN_POINT('Ctrl Pts',(3.91183704069153,-1.,0.441599824524055));
#35878=CARTESIAN_POINT('Ctrl Pts',(3.91875701610719,-1.,0.444660430230591));
#35879=CARTESIAN_POINT('Ctrl Pts',(3.92565674143416,-1.,0.447767416837293));
#35880=CARTESIAN_POINT('Ctrl Pts',(3.93253407403123,-1.,0.450919768356349));
#35881=CARTESIAN_POINT('Ctrl Pts',(3.93939080846298,-1.,0.454116879027584));
#35882=CARTESIAN_POINT('Ctrl Pts',(3.94623117206678,-1.,0.457358410451683));
#35883=CARTESIAN_POINT('Ctrl Pts',(3.95306005817364,-1.,0.460644124429122));
#35884=CARTESIAN_POINT('Ctrl Pts',(3.95988133243538,-1.,0.463973722115734));
#35885=CARTESIAN_POINT('Ctrl Pts',(3.9666962227393,-1.,0.467346690880644));
#35886=CARTESIAN_POINT('Ctrl Pts',(3.97350414289392,-1.,0.47076237961344));
#35887=CARTESIAN_POINT('Ctrl Pts',(3.98030338044409,-1.,0.47422006101951));
#35888=CARTESIAN_POINT('Ctrl Pts',(3.98709184306738,-1.,0.477718999122028));
#35889=CARTESIAN_POINT('Ctrl Pts',(3.99386775880679,-1.,0.481258512209676));
#35890=CARTESIAN_POINT('Ctrl Pts',(4.00063045119288,-1.,0.484838042421835));
#35891=CARTESIAN_POINT('Ctrl Pts',(4.0073800839099,-1.,0.488457130424634));
#35892=CARTESIAN_POINT('Ctrl Pts',(4.01411733503546,-1.,0.492115383418019));
#35893=CARTESIAN_POINT('Ctrl Pts',(4.02084308851832,-1.,0.495812444326251));
#35894=CARTESIAN_POINT('Ctrl Pts',(4.02755813980101,-1.,0.499547962340822));
#35895=CARTESIAN_POINT('Ctrl Pts',(4.03426284174272,-1.,0.503321556915346));
#35896=CARTESIAN_POINT('Ctrl Pts',(4.04095715148915,-1.,0.507132823288137));
#35897=CARTESIAN_POINT('Ctrl Pts',(4.04764078815447,-1.,0.510981349218971));
#35898=CARTESIAN_POINT('Ctrl Pts',(4.05431335771199,-1.,0.514866728193017));
#35899=CARTESIAN_POINT('Ctrl Pts',(4.06097448038013,-1.,0.518788572336924));
#35900=CARTESIAN_POINT('Ctrl Pts',(4.06762394471314,-1.,0.522746528603108));
#35901=CARTESIAN_POINT('Ctrl Pts',(4.07426172299847,-1.,0.526740277227498));
#35902=CARTESIAN_POINT('Ctrl Pts',(4.08088789536836,-1.,0.530769518728571));
#35903=CARTESIAN_POINT('Ctrl Pts',(4.08750259988885,-1.,0.534833963477273));
#35904=CARTESIAN_POINT('Ctrl Pts',(4.09410597627,-1.,0.538933321179756));
#35905=CARTESIAN_POINT('Ctrl Pts',(4.10069810243979,-1.,0.543067286877758));
#35906=CARTESIAN_POINT('Ctrl Pts',(4.10727897027977,-1.,0.547235539485637));
#35907=CARTESIAN_POINT('Ctrl Pts',(4.11384852024721,-1.,0.551437758497033));
#35908=CARTESIAN_POINT('Ctrl Pts',(4.12040666195664,-1.,0.555673636129978));
#35909=CARTESIAN_POINT('Ctrl Pts',(4.12695329951961,-1.,0.559942890594774));
#35910=CARTESIAN_POINT('Ctrl Pts',(4.13348835727104,-1.,0.564245279537149));
#35911=CARTESIAN_POINT('Ctrl Pts',(4.14001179830547,-1.,0.568580610189775));
#35912=CARTESIAN_POINT('Ctrl Pts',(4.14652361068081,-1.,0.572948736069523));
#35913=CARTESIAN_POINT('Ctrl Pts',(4.151723761217,-1.,0.576469391676689));
#35914=CARTESIAN_POINT('Ctrl Pts',(4.15561864788576,-1.,0.579124568914236));
#35915=CARTESIAN_POINT('Ctrl Pts',(4.1582129171283,-1.,0.580901211463535));
#35916=CARTESIAN_POINT('Ctrl Pts',(4.15950947128175,-1.,0.581791163835816));
#35917=CARTESIAN_POINT('',(4.13571194405636,-1.,0.732042837400621));
#35918=CARTESIAN_POINT('',(4.15950947128175,-1.,0.581791163835816));
#35919=CARTESIAN_POINT('Ctrl Pts',(4.13571194405636,-1.,0.732042837400621));
#35920=CARTESIAN_POINT('Ctrl Pts',(4.1342038373684,-1.,0.73248857513516));
#35921=CARTESIAN_POINT('Ctrl Pts',(4.13118752795207,-1.,0.733376589323547));
#35922=CARTESIAN_POINT('Ctrl Pts',(4.12666277570844,-1.,0.734698226764093));
#35923=CARTESIAN_POINT('Ctrl Pts',(4.120629196238,-1.,0.736439634331345));
#35924=CARTESIAN_POINT('Ctrl Pts',(4.11308626951927,-1.,0.738581708225844));
#35925=CARTESIAN_POINT('Ctrl Pts',(4.10554241757547,-1.,0.740688998553377));
#35926=CARTESIAN_POINT('Ctrl Pts',(4.09799769702611,-1.,0.742761369689842));
#35927=CARTESIAN_POINT('Ctrl Pts',(4.09045220253573,-1.,0.744798649706501));
#35928=CARTESIAN_POINT('Ctrl Pts',(4.08290608095642,-1.,0.746800631492316));
#35929=CARTESIAN_POINT('Ctrl Pts',(4.07535951056152,-1.,0.748767076680558));
#35930=CARTESIAN_POINT('Ctrl Pts',(4.06781267242378,-1.,0.750697720484037));
#35931=CARTESIAN_POINT('Ctrl Pts',(4.06026572221515,-1.,0.752592276483073));
#35932=CARTESIAN_POINT('Ctrl Pts',(4.05271876687915,-1.,0.754450441816078));
#35933=CARTESIAN_POINT('Ctrl Pts',(4.04517182653997,-1.,0.756271902369581));
#35934=CARTESIAN_POINT('Ctrl Pts',(4.03762485803119,-1.,0.758056338884945));
#35935=CARTESIAN_POINT('Ctrl Pts',(4.03007781954412,-1.,0.759803433243752));
#35936=CARTESIAN_POINT('Ctrl Pts',(4.02253072741268,-1.,0.761512875859805));
#35937=CARTESIAN_POINT('Ctrl Pts',(4.01498370680496,-1.,0.763184371182936));
#35938=CARTESIAN_POINT('Ctrl Pts',(4.00743706791509,-1.,0.764817648785198));
#35939=CARTESIAN_POINT('Ctrl Pts',(3.99989129179622,-1.,0.766412457136064));
#35940=CARTESIAN_POINT('Ctrl Pts',(3.9923468788101,-1.,0.767968531377915));
#35941=CARTESIAN_POINT('Ctrl Pts',(3.98480422348451,-1.,0.769485566245545));
#35942=CARTESIAN_POINT('Ctrl Pts',(3.97726349165488,-1.,0.770963190030471));
#35943=CARTESIAN_POINT('Ctrl Pts',(3.96972446532772,-1.,0.772400931772137));
#35944=CARTESIAN_POINT('Ctrl Pts',(3.96218649639807,-1.,0.773798212026566));
#35945=CARTESIAN_POINT('Ctrl Pts',(3.9546488545231,-1.,0.775154418039352));
#35946=CARTESIAN_POINT('Ctrl Pts',(3.94711101619447,-1.,0.776468966697922));
#35947=CARTESIAN_POINT('Ctrl Pts',(3.93957296768103,-1.,0.777741370568559));
#35948=CARTESIAN_POINT('Ctrl Pts',(3.93203552473174,-1.,0.778971308134821));
#35949=CARTESIAN_POINT('Ctrl Pts',(3.92450058323823,-1.,0.780158678615543));
#35950=CARTESIAN_POINT('Ctrl Pts',(3.91697036054676,-1.,0.781303428618367));
#35951=CARTESIAN_POINT('Ctrl Pts',(3.90944671004542,-1.,0.782405395622765));
#35952=CARTESIAN_POINT('Ctrl Pts',(3.9019303904397,-1.,0.783464141529082));
#35953=CARTESIAN_POINT('Ctrl Pts',(3.89442039235103,-1.,0.784478799358337));
#35954=CARTESIAN_POINT('Ctrl Pts',(3.88691313167398,-1.,0.785447890340731));
#35955=CARTESIAN_POINT('Ctrl Pts',(3.8794040281819,-1.,0.786369675812609));
#35956=CARTESIAN_POINT('Ctrl Pts',(3.87188916600912,-1.,0.787242527617999));
#35957=CARTESIAN_POINT('Ctrl Pts',(3.86436702561345,-1.,0.788065315093778));
#35958=CARTESIAN_POINT('Ctrl Pts',(3.85683995872529,-1.,0.788837734090672));
#35959=CARTESIAN_POINT('Ctrl Pts',(3.84931637808894,-1.,0.789560798155583));
#35960=CARTESIAN_POINT('Ctrl Pts',(3.84180762342454,-1.,0.790236124191243));
#35961=CARTESIAN_POINT('Ctrl Pts',(3.83432392054786,-1.,0.790865012705301));
#35962=CARTESIAN_POINT('Ctrl Pts',(3.82687033899792,-1.,0.791447528662369));
#35963=CARTESIAN_POINT('Ctrl Pts',(3.81944345442249,-1.,0.791981740718635));
#35964=CARTESIAN_POINT('Ctrl Pts',(3.81202588694756,-1.,0.792462483517635));
#35965=CARTESIAN_POINT('Ctrl Pts',(3.80459229925637,-1.,0.792882695234778));
#35966=CARTESIAN_POINT('Ctrl Pts',(3.79711921389897,-1.,0.793235612973274));
#35967=CARTESIAN_POINT('Ctrl Pts',(3.78959439439235,-1.,0.793516871680994));
#35968=CARTESIAN_POINT('Ctrl Pts',(3.78202460377598,-1.,0.793726235781301));
#35969=CARTESIAN_POINT('Ctrl Pts',(3.77444863801212,-1.,0.793870523787408));
#35970=CARTESIAN_POINT('Ctrl Pts',(3.76692626931111,-1.,0.793961083688992));
#35971=CARTESIAN_POINT('Ctrl Pts',(3.75951468666257,-1.,0.794008429134908));
#35972=CARTESIAN_POINT('Ctrl Pts',(3.75224692493864,-1.,0.794017347371378));
#35973=CARTESIAN_POINT('Ctrl Pts',(3.74511357728861,-1.,0.793982700459952));
#35974=CARTESIAN_POINT('Ctrl Pts',(3.73803280541687,-1.,0.793882700937017));
#35975=CARTESIAN_POINT('Ctrl Pts',(3.73086914695805,-1.,0.793682750269684));
#35976=CARTESIAN_POINT('Ctrl Pts',(3.72348797293734,-1.,0.793347023784205));
#35977=CARTESIAN_POINT('Ctrl Pts',(3.71580242396124,-1.,0.792848377370287));
#35978=CARTESIAN_POINT('Ctrl Pts',(3.70781724021806,-1.,0.792177688845818));
#35979=CARTESIAN_POINT('Ctrl Pts',(3.69968940808721,-1.,0.79135657569598));
#35980=CARTESIAN_POINT('Ctrl Pts',(3.69172044327364,-1.,0.790436284988788));
#35981=CARTESIAN_POINT('Ctrl Pts',(3.68428439783905,-1.,0.789483546064387));
#35982=CARTESIAN_POINT('Ctrl Pts',(3.67777119516252,-1.,0.788569566220286));
#35983=CARTESIAN_POINT('Ctrl Pts',(3.67252923663655,-1.,0.787758799995743));
#35984=CARTESIAN_POINT('Ctrl Pts',(3.66907505398677,-1.,0.787145041181546));
#35985=CARTESIAN_POINT('Ctrl Pts',(3.66743103898702,-1.,0.786774337198063));
#35986=CARTESIAN_POINT('Ctrl Pts',(3.66680946938292,-1.,0.786565919558984));
#35987=CARTESIAN_POINT('Ctrl Pts',(3.6666431041522,-1.,0.786459983895432));
#35988=CARTESIAN_POINT('Ctrl Pts',(3.66661143271685,-1.,0.786422660831985));
#35989=CARTESIAN_POINT('Origin',(0.,-1.,0.));
#35990=CARTESIAN_POINT('Origin',(0.,0.,0.));
#35991=CARTESIAN_POINT('Origin',(0.,2.2,0.));
#35992=CARTESIAN_POINT('Origin',(0.,1.,0.));
#35993=CARTESIAN_POINT('',(-2.,2.2,2.44929359829471E-16));
#35994=CARTESIAN_POINT('Origin',(0.,2.2,0.));
#35995=CARTESIAN_POINT('',(-2.,1.,2.44929359829471E-16));
#35996=CARTESIAN_POINT('',(-2.,1.,2.44929359829471E-16));
#35997=CARTESIAN_POINT('Origin',(0.,1.,0.));
#35998=CARTESIAN_POINT('Origin',(0.,2.2,0.));
#35999=CARTESIAN_POINT('Ctrl Pts',(4.15950947128175,-1.,0.581791163835816));
#36000=CARTESIAN_POINT('Ctrl Pts',(4.15950947128175,1.,0.581791163835816));
#36001=CARTESIAN_POINT('Ctrl Pts',(4.1582129171283,-1.,0.580901211463535));
#36002=CARTESIAN_POINT('Ctrl Pts',(4.1582129171283,1.,0.580901211463535));
#36003=CARTESIAN_POINT('Ctrl Pts',(4.15561864788576,-1.,0.579124568914236));
#36004=CARTESIAN_POINT('Ctrl Pts',(4.15561864788576,1.,0.579124568914236));
#36005=CARTESIAN_POINT('Ctrl Pts',(4.151723761217,-1.,0.576469391676689));
#36006=CARTESIAN_POINT('Ctrl Pts',(4.151723761217,1.,0.576469391676689));
#36007=CARTESIAN_POINT('Ctrl Pts',(4.14652361068081,-1.,0.572948736069523));
#36008=CARTESIAN_POINT('Ctrl Pts',(4.14652361068081,1.,0.572948736069523));
#36009=CARTESIAN_POINT('Ctrl Pts',(4.14001179830547,-1.,0.568580610189775));
#36010=CARTESIAN_POINT('Ctrl Pts',(4.14001179830547,1.,0.568580610189775));
#36011=CARTESIAN_POINT('Ctrl Pts',(4.13348835727104,-1.,0.564245279537149));
#36012=CARTESIAN_POINT('Ctrl Pts',(4.13348835727104,1.,0.564245279537149));
#36013=CARTESIAN_POINT('Ctrl Pts',(4.12695329951961,-1.,0.559942890594774));
#36014=CARTESIAN_POINT('Ctrl Pts',(4.12695329951961,1.,0.559942890594774));
#36015=CARTESIAN_POINT('Ctrl Pts',(4.12040666195664,-1.,0.555673636129978));
#36016=CARTESIAN_POINT('Ctrl Pts',(4.12040666195664,1.,0.555673636129978));
#36017=CARTESIAN_POINT('Ctrl Pts',(4.11384852024721,-1.,0.551437758497033));
#36018=CARTESIAN_POINT('Ctrl Pts',(4.11384852024721,1.,0.551437758497033));
#36019=CARTESIAN_POINT('Ctrl Pts',(4.10727897027977,-1.,0.547235539485637));
#36020=CARTESIAN_POINT('Ctrl Pts',(4.10727897027977,1.,0.547235539485637));
#36021=CARTESIAN_POINT('Ctrl Pts',(4.10069810243979,-1.,0.543067286877758));
#36022=CARTESIAN_POINT('Ctrl Pts',(4.10069810243979,1.,0.543067286877758));
#36023=CARTESIAN_POINT('Ctrl Pts',(4.09410597627,-1.,0.538933321179756));
#36024=CARTESIAN_POINT('Ctrl Pts',(4.09410597627,1.,0.538933321179756));
#36025=CARTESIAN_POINT('Ctrl Pts',(4.08750259988885,-1.,0.534833963477273));
#36026=CARTESIAN_POINT('Ctrl Pts',(4.08750259988885,1.,0.534833963477273));
#36027=CARTESIAN_POINT('Ctrl Pts',(4.08088789536836,-1.,0.530769518728571));
#36028=CARTESIAN_POINT('Ctrl Pts',(4.08088789536836,1.,0.530769518728571));
#36029=CARTESIAN_POINT('Ctrl Pts',(4.07426172299847,-1.,0.526740277227498));
#36030=CARTESIAN_POINT('Ctrl Pts',(4.07426172299847,1.,0.526740277227498));
#36031=CARTESIAN_POINT('Ctrl Pts',(4.06762394471314,-1.,0.522746528603108));
#36032=CARTESIAN_POINT('Ctrl Pts',(4.06762394471314,1.,0.522746528603108));
#36033=CARTESIAN_POINT('Ctrl Pts',(4.06097448038013,-1.,0.518788572336924));
#36034=CARTESIAN_POINT('Ctrl Pts',(4.06097448038013,1.,0.518788572336924));
#36035=CARTESIAN_POINT('Ctrl Pts',(4.05431335771199,-1.,0.514866728193017));
#36036=CARTESIAN_POINT('Ctrl Pts',(4.05431335771199,1.,0.514866728193017));
#36037=CARTESIAN_POINT('Ctrl Pts',(4.04764078815447,-1.,0.510981349218971));
#36038=CARTESIAN_POINT('Ctrl Pts',(4.04764078815447,1.,0.510981349218971));
#36039=CARTESIAN_POINT('Ctrl Pts',(4.04095715148915,-1.,0.507132823288137));
#36040=CARTESIAN_POINT('Ctrl Pts',(4.04095715148915,1.,0.507132823288137));
#36041=CARTESIAN_POINT('Ctrl Pts',(4.03426284174272,-1.,0.503321556915346));
#36042=CARTESIAN_POINT('Ctrl Pts',(4.03426284174272,1.,0.503321556915346));
#36043=CARTESIAN_POINT('Ctrl Pts',(4.02755813980101,-1.,0.499547962340822));
#36044=CARTESIAN_POINT('Ctrl Pts',(4.02755813980101,1.,0.499547962340822));
#36045=CARTESIAN_POINT('Ctrl Pts',(4.02084308851832,-1.,0.495812444326251));
#36046=CARTESIAN_POINT('Ctrl Pts',(4.02084308851832,1.,0.495812444326251));
#36047=CARTESIAN_POINT('Ctrl Pts',(4.01411733503546,-1.,0.492115383418019));
#36048=CARTESIAN_POINT('Ctrl Pts',(4.01411733503546,1.,0.492115383418019));
#36049=CARTESIAN_POINT('Ctrl Pts',(4.0073800839099,-1.,0.488457130424634));
#36050=CARTESIAN_POINT('Ctrl Pts',(4.0073800839099,1.,0.488457130424634));
#36051=CARTESIAN_POINT('Ctrl Pts',(4.00063045119288,-1.,0.484838042421835));
#36052=CARTESIAN_POINT('Ctrl Pts',(4.00063045119288,1.,0.484838042421835));
#36053=CARTESIAN_POINT('Ctrl Pts',(3.99386775880679,-1.,0.481258512209676));
#36054=CARTESIAN_POINT('Ctrl Pts',(3.99386775880679,1.,0.481258512209676));
#36055=CARTESIAN_POINT('Ctrl Pts',(3.98709184306738,-1.,0.477718999122028));
#36056=CARTESIAN_POINT('Ctrl Pts',(3.98709184306738,1.,0.477718999122028));
#36057=CARTESIAN_POINT('Ctrl Pts',(3.98030338044409,-1.,0.47422006101951));
#36058=CARTESIAN_POINT('Ctrl Pts',(3.98030338044409,1.,0.47422006101951));
#36059=CARTESIAN_POINT('Ctrl Pts',(3.97350414289392,-1.,0.47076237961344));
#36060=CARTESIAN_POINT('Ctrl Pts',(3.97350414289392,1.,0.47076237961344));
#36061=CARTESIAN_POINT('Ctrl Pts',(3.9666962227393,-1.,0.467346690880644));
#36062=CARTESIAN_POINT('Ctrl Pts',(3.9666962227393,1.,0.467346690880644));
#36063=CARTESIAN_POINT('Ctrl Pts',(3.95988133243538,-1.,0.463973722115734));
#36064=CARTESIAN_POINT('Ctrl Pts',(3.95988133243538,1.,0.463973722115734));
#36065=CARTESIAN_POINT('Ctrl Pts',(3.95306005817364,-1.,0.460644124429122));
#36066=CARTESIAN_POINT('Ctrl Pts',(3.95306005817364,1.,0.460644124429122));
#36067=CARTESIAN_POINT('Ctrl Pts',(3.94623117206678,-1.,0.457358410451683));
#36068=CARTESIAN_POINT('Ctrl Pts',(3.94623117206678,1.,0.457358410451683));
#36069=CARTESIAN_POINT('Ctrl Pts',(3.93939080846298,-1.,0.454116879027584));
#36070=CARTESIAN_POINT('Ctrl Pts',(3.93939080846298,1.,0.454116879027584));
#36071=CARTESIAN_POINT('Ctrl Pts',(3.93253407403123,-1.,0.450919768356349));
#36072=CARTESIAN_POINT('Ctrl Pts',(3.93253407403123,1.,0.450919768356349));
#36073=CARTESIAN_POINT('Ctrl Pts',(3.92565674143416,-1.,0.447767416837293));
#36074=CARTESIAN_POINT('Ctrl Pts',(3.92565674143416,1.,0.447767416837293));
#36075=CARTESIAN_POINT('Ctrl Pts',(3.91875701610719,-1.,0.444660430230591));
#36076=CARTESIAN_POINT('Ctrl Pts',(3.91875701610719,1.,0.444660430230591));
#36077=CARTESIAN_POINT('Ctrl Pts',(3.91183704069153,-1.,0.441599824524055));
#36078=CARTESIAN_POINT('Ctrl Pts',(3.91183704069153,1.,0.441599824524055));
#36079=CARTESIAN_POINT('Ctrl Pts',(3.90490512938563,-1.,0.43858723545825));
#36080=CARTESIAN_POINT('Ctrl Pts',(3.90490512938563,1.,0.43858723545825));
#36081=CARTESIAN_POINT('Ctrl Pts',(3.89797256655462,-1.,0.435624629433528));
#36082=CARTESIAN_POINT('Ctrl Pts',(3.89797256655462,1.,0.435624629433528));
#36083=CARTESIAN_POINT('Ctrl Pts',(3.89104947940611,-1.,0.432713929544459));
#36084=CARTESIAN_POINT('Ctrl Pts',(3.89104947940611,1.,0.432713929544459));
#36085=CARTESIAN_POINT('Ctrl Pts',(3.88414070943341,-1.,0.429856640579741));
#36086=CARTESIAN_POINT('Ctrl Pts',(3.88414070943341,1.,0.429856640579741));
#36087=CARTESIAN_POINT('Ctrl Pts',(3.87724240306597,-1.,0.427053541173458));
#36088=CARTESIAN_POINT('Ctrl Pts',(3.87724240306597,1.,0.427053541173458));
#36089=CARTESIAN_POINT('Ctrl Pts',(3.87033643487851,-1.,0.424304173195111));
#36090=CARTESIAN_POINT('Ctrl Pts',(3.87033643487851,1.,0.424304173195111));
#36091=CARTESIAN_POINT('Ctrl Pts',(3.86339652542709,-1.,0.421607423177534));
#36092=CARTESIAN_POINT('Ctrl Pts',(3.86339652542709,1.,0.421607423177534));
#36093=CARTESIAN_POINT('Ctrl Pts',(3.85639825647996,-1.,0.418962468086773));
#36094=CARTESIAN_POINT('Ctrl Pts',(3.85639825647996,1.,0.418962468086773));
#36095=CARTESIAN_POINT('Ctrl Pts',(3.84932864157497,-1.,0.416369678052907));
#36096=CARTESIAN_POINT('Ctrl Pts',(3.84932864157497,1.,0.416369678052907));
#36097=CARTESIAN_POINT('Ctrl Pts',(3.84219403994762,-1.,0.413831367016748));
#36098=CARTESIAN_POINT('Ctrl Pts',(3.84219403994762,1.,0.413831367016748));
#36099=CARTESIAN_POINT('Ctrl Pts',(3.83503345578698,-1.,0.411353038798519));
#36100=CARTESIAN_POINT('Ctrl Pts',(3.83503345578698,1.,0.411353038798519));
#36101=CARTESIAN_POINT('Ctrl Pts',(3.82790724256471,-1.,0.40894237144746));
#36102=CARTESIAN_POINT('Ctrl Pts',(3.82790724256471,1.,0.40894237144746));
#36103=CARTESIAN_POINT('Ctrl Pts',(3.8208730391381,-1.,0.406607038258986));
#36104=CARTESIAN_POINT('Ctrl Pts',(3.8208730391381,1.,0.406607038258986));
#36105=CARTESIAN_POINT('Ctrl Pts',(3.81396374287793,-1.,0.404352694628274));
#36106=CARTESIAN_POINT('Ctrl Pts',(3.81396374287793,1.,0.404352694628274));
#36107=CARTESIAN_POINT('Ctrl Pts',(3.80716881962728,-1.,0.402181320148436));
#36108=CARTESIAN_POINT('Ctrl Pts',(3.80716881962728,1.,0.402181320148436));
#36109=CARTESIAN_POINT('Ctrl Pts',(3.80040370384546,-1.,0.400088346504601));
#36110=CARTESIAN_POINT('Ctrl Pts',(3.80040370384546,1.,0.400088346504601));
#36111=CARTESIAN_POINT('Ctrl Pts',(3.7935288716329,-1.,0.39806481868397));
#36112=CARTESIAN_POINT('Ctrl Pts',(3.7935288716329,1.,0.39806481868397));
#36113=CARTESIAN_POINT('Ctrl Pts',(3.78640521279313,-1.,0.396103205334841));
#36114=CARTESIAN_POINT('Ctrl Pts',(3.78640521279313,1.,0.396103205334841));
#36115=CARTESIAN_POINT('Ctrl Pts',(3.77894173114283,-1.,0.3942024810115));
#36116=CARTESIAN_POINT('Ctrl Pts',(3.77894173114283,1.,0.3942024810115));
#36117=CARTESIAN_POINT('Ctrl Pts',(3.77114011595967,-1.,0.392372786223433));
#36118=CARTESIAN_POINT('Ctrl Pts',(3.77114011595967,1.,0.392372786223433));
#36119=CARTESIAN_POINT('Ctrl Pts',(3.76315635033257,-1.,0.39064207297956));
#36120=CARTESIAN_POINT('Ctrl Pts',(3.76315635033257,1.,0.39064207297956));
#36121=CARTESIAN_POINT('Ctrl Pts',(3.75529302895152,-1.,0.389054775898702));
#36122=CARTESIAN_POINT('Ctrl Pts',(3.75529302895152,1.,0.389054775898702));
#36123=CARTESIAN_POINT('Ctrl Pts',(3.74792651696654,-1.,0.387663020050836));
#36124=CARTESIAN_POINT('Ctrl Pts',(3.74792651696654,1.,0.387663020050836));
#36125=CARTESIAN_POINT('Ctrl Pts',(3.74144965781276,-1.,0.386519576222252));
#36126=CARTESIAN_POINT('Ctrl Pts',(3.74144965781276,1.,0.386519576222252));
#36127=CARTESIAN_POINT('Ctrl Pts',(3.73621371845318,-1.,0.385670806454566));
#36128=CARTESIAN_POINT('Ctrl Pts',(3.73621371845318,1.,0.385670806454566));
#36129=CARTESIAN_POINT('Ctrl Pts',(3.73245705638843,-1.,0.385147887988952));
#36130=CARTESIAN_POINT('Ctrl Pts',(3.73245705638843,1.,0.385147887988952));
#36131=CARTESIAN_POINT('Ctrl Pts',(3.73072465900175,-1.,0.385001870183213));
#36132=CARTESIAN_POINT('Ctrl Pts',(3.73072465900175,1.,0.385001870183213));
#36133=CARTESIAN_POINT('Ctrl Pts',(3.73015851028356,-1.,0.385047711603463));
#36134=CARTESIAN_POINT('Ctrl Pts',(3.73015851028356,1.,0.385047711603463));
#36135=CARTESIAN_POINT('Ctrl Pts',(3.73010668803042,-1.,0.385147278814643));
#36136=CARTESIAN_POINT('Ctrl Pts',(3.73010668803042,1.,0.385147278814643));
#36137=CARTESIAN_POINT('Ctrl Pts',(3.73016218570874,-1.,0.38521431477633));
#36138=CARTESIAN_POINT('Ctrl Pts',(3.73016218570874,1.,0.38521431477633));
#36139=CARTESIAN_POINT('',(3.73017266276651,1.,0.385112848330762));
#36140=CARTESIAN_POINT('Ctrl Pts',(3.73017266276651,1.,0.385112848330762));
#36141=CARTESIAN_POINT('Ctrl Pts',(3.73017266276651,0.666666666666667,0.385112848330762));
#36142=CARTESIAN_POINT('Ctrl Pts',(3.73017266276651,0.333333333333333,0.385112848330762));
#36143=CARTESIAN_POINT('Ctrl Pts',(3.73017266276651,-0.333333333333333,
0.385112848330762));
#36144=CARTESIAN_POINT('Ctrl Pts',(3.73017266276651,-0.666666666666667,
0.385112848330763));
#36145=CARTESIAN_POINT('Ctrl Pts',(3.73017266276651,-1.,0.385112848330763));
#36146=CARTESIAN_POINT('',(4.15950947128175,1.,0.581791163835816));
#36147=CARTESIAN_POINT('Ctrl Pts',(4.15950947128175,1.,0.581791163835816));
#36148=CARTESIAN_POINT('Ctrl Pts',(4.1582129171283,1.,0.580901211463535));
#36149=CARTESIAN_POINT('Ctrl Pts',(4.15561864788576,1.,0.579124568914236));
#36150=CARTESIAN_POINT('Ctrl Pts',(4.151723761217,1.,0.576469391676689));
#36151=CARTESIAN_POINT('Ctrl Pts',(4.14652361068081,1.,0.572948736069523));
#36152=CARTESIAN_POINT('Ctrl Pts',(4.14001179830547,1.,0.568580610189775));
#36153=CARTESIAN_POINT('Ctrl Pts',(4.13348835727104,1.,0.564245279537149));
#36154=CARTESIAN_POINT('Ctrl Pts',(4.12695329951961,1.,0.559942890594774));
#36155=CARTESIAN_POINT('Ctrl Pts',(4.12040666195664,1.,0.555673636129978));
#36156=CARTESIAN_POINT('Ctrl Pts',(4.11384852024721,1.,0.551437758497033));
#36157=CARTESIAN_POINT('Ctrl Pts',(4.10727897027977,1.,0.547235539485637));
#36158=CARTESIAN_POINT('Ctrl Pts',(4.10069810243979,1.,0.543067286877758));
#36159=CARTESIAN_POINT('Ctrl Pts',(4.09410597627,1.,0.538933321179756));
#36160=CARTESIAN_POINT('Ctrl Pts',(4.08750259988885,1.,0.534833963477273));
#36161=CARTESIAN_POINT('Ctrl Pts',(4.08088789536836,1.,0.530769518728571));
#36162=CARTESIAN_POINT('Ctrl Pts',(4.07426172299847,1.,0.526740277227498));
#36163=CARTESIAN_POINT('Ctrl Pts',(4.06762394471314,1.,0.522746528603108));
#36164=CARTESIAN_POINT('Ctrl Pts',(4.06097448038013,1.,0.518788572336924));
#36165=CARTESIAN_POINT('Ctrl Pts',(4.05431335771199,1.,0.514866728193017));
#36166=CARTESIAN_POINT('Ctrl Pts',(4.04764078815447,1.,0.510981349218971));
#36167=CARTESIAN_POINT('Ctrl Pts',(4.04095715148915,1.,0.507132823288137));
#36168=CARTESIAN_POINT('Ctrl Pts',(4.03426284174272,1.,0.503321556915346));
#36169=CARTESIAN_POINT('Ctrl Pts',(4.02755813980101,1.,0.499547962340822));
#36170=CARTESIAN_POINT('Ctrl Pts',(4.02084308851832,1.,0.495812444326251));
#36171=CARTESIAN_POINT('Ctrl Pts',(4.01411733503546,1.,0.492115383418019));
#36172=CARTESIAN_POINT('Ctrl Pts',(4.0073800839099,1.,0.488457130424634));
#36173=CARTESIAN_POINT('Ctrl Pts',(4.00063045119288,1.,0.484838042421835));
#36174=CARTESIAN_POINT('Ctrl Pts',(3.99386775880679,1.,0.481258512209676));
#36175=CARTESIAN_POINT('Ctrl Pts',(3.98709184306738,1.,0.477718999122028));
#36176=CARTESIAN_POINT('Ctrl Pts',(3.98030338044409,1.,0.47422006101951));
#36177=CARTESIAN_POINT('Ctrl Pts',(3.97350414289392,1.,0.47076237961344));
#36178=CARTESIAN_POINT('Ctrl Pts',(3.9666962227393,1.,0.467346690880644));
#36179=CARTESIAN_POINT('Ctrl Pts',(3.95988133243538,1.,0.463973722115734));
#36180=CARTESIAN_POINT('Ctrl Pts',(3.95306005817364,1.,0.460644124429122));
#36181=CARTESIAN_POINT('Ctrl Pts',(3.94623117206678,1.,0.457358410451683));
#36182=CARTESIAN_POINT('Ctrl Pts',(3.93939080846298,1.,0.454116879027584));
#36183=CARTESIAN_POINT('Ctrl Pts',(3.93253407403123,1.,0.450919768356349));
#36184=CARTESIAN_POINT('Ctrl Pts',(3.92565674143416,1.,0.447767416837293));
#36185=CARTESIAN_POINT('Ctrl Pts',(3.91875701610719,1.,0.444660430230591));
#36186=CARTESIAN_POINT('Ctrl Pts',(3.91183704069153,1.,0.441599824524055));
#36187=CARTESIAN_POINT('Ctrl Pts',(3.90490512938563,1.,0.43858723545825));
#36188=CARTESIAN_POINT('Ctrl Pts',(3.89797256655462,1.,0.435624629433528));
#36189=CARTESIAN_POINT('Ctrl Pts',(3.89104947940611,1.,0.432713929544459));
#36190=CARTESIAN_POINT('Ctrl Pts',(3.88414070943341,1.,0.429856640579741));
#36191=CARTESIAN_POINT('Ctrl Pts',(3.87724240306597,1.,0.427053541173458));
#36192=CARTESIAN_POINT('Ctrl Pts',(3.87033643487851,1.,0.424304173195111));
#36193=CARTESIAN_POINT('Ctrl Pts',(3.86339652542709,1.,0.421607423177534));
#36194=CARTESIAN_POINT('Ctrl Pts',(3.85639825647996,1.,0.418962468086773));
#36195=CARTESIAN_POINT('Ctrl Pts',(3.84932864157497,1.,0.416369678052907));
#36196=CARTESIAN_POINT('Ctrl Pts',(3.84219403994762,1.,0.413831367016748));
#36197=CARTESIAN_POINT('Ctrl Pts',(3.83503345578698,1.,0.411353038798519));
#36198=CARTESIAN_POINT('Ctrl Pts',(3.82790724256471,1.,0.40894237144746));
#36199=CARTESIAN_POINT('Ctrl Pts',(3.8208730391381,1.,0.406607038258986));
#36200=CARTESIAN_POINT('Ctrl Pts',(3.81396374287793,1.,0.404352694628274));
#36201=CARTESIAN_POINT('Ctrl Pts',(3.80716881962728,1.,0.402181320148436));
#36202=CARTESIAN_POINT('Ctrl Pts',(3.80040370384546,1.,0.400088346504601));
#36203=CARTESIAN_POINT('Ctrl Pts',(3.7935288716329,1.,0.39806481868397));
#36204=CARTESIAN_POINT('Ctrl Pts',(3.78640521279313,1.,0.396103205334841));
#36205=CARTESIAN_POINT('Ctrl Pts',(3.77894173114283,1.,0.3942024810115));
#36206=CARTESIAN_POINT('Ctrl Pts',(3.77114011595967,1.,0.392372786223433));
#36207=CARTESIAN_POINT('Ctrl Pts',(3.76315635033257,1.,0.39064207297956));
#36208=CARTESIAN_POINT('Ctrl Pts',(3.75529302895152,1.,0.389054775898702));
#36209=CARTESIAN_POINT('Ctrl Pts',(3.74792651696654,1.,0.387663020050836));
#36210=CARTESIAN_POINT('Ctrl Pts',(3.74144965781276,1.,0.386519576222252));
#36211=CARTESIAN_POINT('Ctrl Pts',(3.73621371845318,1.,0.385670806454566));
#36212=CARTESIAN_POINT('Ctrl Pts',(3.73273893363406,1.,0.385187124634207));
#36213=CARTESIAN_POINT('Ctrl Pts',(3.73106082862548,1.,0.385031656499164));
#36214=CARTESIAN_POINT('Ctrl Pts',(3.73040527621055,1.,0.385037797881504));
#36215=CARTESIAN_POINT('Ctrl Pts',(3.73021431755274,1.,0.385087139000375));
#36216=CARTESIAN_POINT('Ctrl Pts',(3.73017266276651,1.,0.385112848330762));
#36217=CARTESIAN_POINT('',(4.15950947128175,0.,0.581791163835816));
#36218=CARTESIAN_POINT('Ctrl Pts',(3.66663282329846,-1.,0.7863229229206));
#36219=CARTESIAN_POINT('Ctrl Pts',(3.66663282329846,1.,0.7863229229206));
#36220=CARTESIAN_POINT('Ctrl Pts',(3.66655932661986,-1.,0.786369528183326));
#36221=CARTESIAN_POINT('Ctrl Pts',(3.66655932661986,1.,0.786369528183326));
#36222=CARTESIAN_POINT('Ctrl Pts',(3.66657784455334,-1.,0.786480236185697));
#36223=CARTESIAN_POINT('Ctrl Pts',(3.66657784455334,1.,0.786480236185697));
#36224=CARTESIAN_POINT('Ctrl Pts',(3.66710211820482,-1.,0.786698783542764));
#36225=CARTESIAN_POINT('Ctrl Pts',(3.66710211820482,1.,0.786698783542764));
#36226=CARTESIAN_POINT('Ctrl Pts',(3.66879484801113,-1.,0.787095252590501));
#36227=CARTESIAN_POINT('Ctrl Pts',(3.66879484801113,1.,0.787095252590501));
#36228=CARTESIAN_POINT('Ctrl Pts',(3.67252923663655,-1.,0.787758799995743));
#36229=CARTESIAN_POINT('Ctrl Pts',(3.67252923663655,1.,0.787758799995743));
#36230=CARTESIAN_POINT('Ctrl Pts',(3.67777119516252,-1.,0.788569566220286));
#36231=CARTESIAN_POINT('Ctrl Pts',(3.67777119516252,1.,0.788569566220286));
#36232=CARTESIAN_POINT('Ctrl Pts',(3.68428439783905,-1.,0.789483546064387));
#36233=CARTESIAN_POINT('Ctrl Pts',(3.68428439783905,1.,0.789483546064387));
#36234=CARTESIAN_POINT('Ctrl Pts',(3.69172044327364,-1.,0.790436284988788));
#36235=CARTESIAN_POINT('Ctrl Pts',(3.69172044327364,1.,0.790436284988788));
#36236=CARTESIAN_POINT('Ctrl Pts',(3.69968940808721,-1.,0.79135657569598));
#36237=CARTESIAN_POINT('Ctrl Pts',(3.69968940808721,1.,0.79135657569598));
#36238=CARTESIAN_POINT('Ctrl Pts',(3.70781724021806,-1.,0.792177688845818));
#36239=CARTESIAN_POINT('Ctrl Pts',(3.70781724021806,1.,0.792177688845818));
#36240=CARTESIAN_POINT('Ctrl Pts',(3.71580242396124,-1.,0.792848377370287));
#36241=CARTESIAN_POINT('Ctrl Pts',(3.71580242396124,1.,0.792848377370287));
#36242=CARTESIAN_POINT('Ctrl Pts',(3.72348797293734,-1.,0.793347023784205));
#36243=CARTESIAN_POINT('Ctrl Pts',(3.72348797293734,1.,0.793347023784205));
#36244=CARTESIAN_POINT('Ctrl Pts',(3.73086914695805,-1.,0.793682750269684));
#36245=CARTESIAN_POINT('Ctrl Pts',(3.73086914695805,1.,0.793682750269684));
#36246=CARTESIAN_POINT('Ctrl Pts',(3.73803280541687,-1.,0.793882700937017));
#36247=CARTESIAN_POINT('Ctrl Pts',(3.73803280541687,1.,0.793882700937017));
#36248=CARTESIAN_POINT('Ctrl Pts',(3.74511357728861,-1.,0.793982700459952));
#36249=CARTESIAN_POINT('Ctrl Pts',(3.74511357728861,1.,0.793982700459952));
#36250=CARTESIAN_POINT('Ctrl Pts',(3.75224692493864,-1.,0.794017347371378));
#36251=CARTESIAN_POINT('Ctrl Pts',(3.75224692493864,1.,0.794017347371378));
#36252=CARTESIAN_POINT('Ctrl Pts',(3.75951468666257,-1.,0.794008429134908));
#36253=CARTESIAN_POINT('Ctrl Pts',(3.75951468666257,1.,0.794008429134908));
#36254=CARTESIAN_POINT('Ctrl Pts',(3.76692626931111,-1.,0.793961083688992));
#36255=CARTESIAN_POINT('Ctrl Pts',(3.76692626931111,1.,0.793961083688992));
#36256=CARTESIAN_POINT('Ctrl Pts',(3.77444863801212,-1.,0.793870523787408));
#36257=CARTESIAN_POINT('Ctrl Pts',(3.77444863801212,1.,0.793870523787408));
#36258=CARTESIAN_POINT('Ctrl Pts',(3.78202460377598,-1.,0.793726235781301));
#36259=CARTESIAN_POINT('Ctrl Pts',(3.78202460377598,1.,0.793726235781301));
#36260=CARTESIAN_POINT('Ctrl Pts',(3.78959439439235,-1.,0.793516871680994));
#36261=CARTESIAN_POINT('Ctrl Pts',(3.78959439439235,1.,0.793516871680994));
#36262=CARTESIAN_POINT('Ctrl Pts',(3.79711921389897,-1.,0.793235612973274));
#36263=CARTESIAN_POINT('Ctrl Pts',(3.79711921389897,1.,0.793235612973274));
#36264=CARTESIAN_POINT('Ctrl Pts',(3.80459229925637,-1.,0.792882695234778));
#36265=CARTESIAN_POINT('Ctrl Pts',(3.80459229925637,1.,0.792882695234778));
#36266=CARTESIAN_POINT('Ctrl Pts',(3.81202588694756,-1.,0.792462483517635));
#36267=CARTESIAN_POINT('Ctrl Pts',(3.81202588694756,1.,0.792462483517635));
#36268=CARTESIAN_POINT('Ctrl Pts',(3.81944345442249,-1.,0.791981740718635));
#36269=CARTESIAN_POINT('Ctrl Pts',(3.81944345442249,1.,0.791981740718635));
#36270=CARTESIAN_POINT('Ctrl Pts',(3.82687033899792,-1.,0.791447528662369));
#36271=CARTESIAN_POINT('Ctrl Pts',(3.82687033899792,1.,0.791447528662369));
#36272=CARTESIAN_POINT('Ctrl Pts',(3.83432392054786,-1.,0.790865012705301));
#36273=CARTESIAN_POINT('Ctrl Pts',(3.83432392054786,1.,0.790865012705301));
#36274=CARTESIAN_POINT('Ctrl Pts',(3.84180762342454,-1.,0.790236124191243));
#36275=CARTESIAN_POINT('Ctrl Pts',(3.84180762342454,1.,0.790236124191243));
#36276=CARTESIAN_POINT('Ctrl Pts',(3.84931637808894,-1.,0.789560798155583));
#36277=CARTESIAN_POINT('Ctrl Pts',(3.84931637808894,1.,0.789560798155583));
#36278=CARTESIAN_POINT('Ctrl Pts',(3.85683995872529,-1.,0.788837734090672));
#36279=CARTESIAN_POINT('Ctrl Pts',(3.85683995872529,1.,0.788837734090672));
#36280=CARTESIAN_POINT('Ctrl Pts',(3.86436702561345,-1.,0.788065315093778));
#36281=CARTESIAN_POINT('Ctrl Pts',(3.86436702561345,1.,0.788065315093778));
#36282=CARTESIAN_POINT('Ctrl Pts',(3.87188916600912,-1.,0.787242527617999));
#36283=CARTESIAN_POINT('Ctrl Pts',(3.87188916600912,1.,0.787242527617999));
#36284=CARTESIAN_POINT('Ctrl Pts',(3.8794040281819,-1.,0.786369675812609));
#36285=CARTESIAN_POINT('Ctrl Pts',(3.8794040281819,1.,0.786369675812609));
#36286=CARTESIAN_POINT('Ctrl Pts',(3.88691313167398,-1.,0.785447890340731));
#36287=CARTESIAN_POINT('Ctrl Pts',(3.88691313167398,1.,0.785447890340731));
#36288=CARTESIAN_POINT('Ctrl Pts',(3.89442039235103,-1.,0.784478799358337));
#36289=CARTESIAN_POINT('Ctrl Pts',(3.89442039235103,1.,0.784478799358337));
#36290=CARTESIAN_POINT('Ctrl Pts',(3.9019303904397,-1.,0.783464141529082));
#36291=CARTESIAN_POINT('Ctrl Pts',(3.9019303904397,1.,0.783464141529082));
#36292=CARTESIAN_POINT('Ctrl Pts',(3.90944671004542,-1.,0.782405395622765));
#36293=CARTESIAN_POINT('Ctrl Pts',(3.90944671004542,1.,0.782405395622765));
#36294=CARTESIAN_POINT('Ctrl Pts',(3.91697036054676,-1.,0.781303428618367));
#36295=CARTESIAN_POINT('Ctrl Pts',(3.91697036054676,1.,0.781303428618367));
#36296=CARTESIAN_POINT('Ctrl Pts',(3.92450058323823,-1.,0.780158678615543));
#36297=CARTESIAN_POINT('Ctrl Pts',(3.92450058323823,1.,0.780158678615543));
#36298=CARTESIAN_POINT('Ctrl Pts',(3.93203552473174,-1.,0.778971308134821));
#36299=CARTESIAN_POINT('Ctrl Pts',(3.93203552473174,1.,0.778971308134821));
#36300=CARTESIAN_POINT('Ctrl Pts',(3.93957296768103,-1.,0.777741370568559));
#36301=CARTESIAN_POINT('Ctrl Pts',(3.93957296768103,1.,0.777741370568559));
#36302=CARTESIAN_POINT('Ctrl Pts',(3.94711101619447,-1.,0.776468966697922));
#36303=CARTESIAN_POINT('Ctrl Pts',(3.94711101619447,1.,0.776468966697922));
#36304=CARTESIAN_POINT('Ctrl Pts',(3.9546488545231,-1.,0.775154418039352));
#36305=CARTESIAN_POINT('Ctrl Pts',(3.9546488545231,1.,0.775154418039352));
#36306=CARTESIAN_POINT('Ctrl Pts',(3.96218649639807,-1.,0.773798212026566));
#36307=CARTESIAN_POINT('Ctrl Pts',(3.96218649639807,1.,0.773798212026566));
#36308=CARTESIAN_POINT('Ctrl Pts',(3.96972446532772,-1.,0.772400931772137));
#36309=CARTESIAN_POINT('Ctrl Pts',(3.96972446532772,1.,0.772400931772137));
#36310=CARTESIAN_POINT('Ctrl Pts',(3.97726349165488,-1.,0.770963190030471));
#36311=CARTESIAN_POINT('Ctrl Pts',(3.97726349165488,1.,0.770963190030471));
#36312=CARTESIAN_POINT('Ctrl Pts',(3.98480422348451,-1.,0.769485566245545));
#36313=CARTESIAN_POINT('Ctrl Pts',(3.98480422348451,1.,0.769485566245545));
#36314=CARTESIAN_POINT('Ctrl Pts',(3.9923468788101,-1.,0.767968531377915));
#36315=CARTESIAN_POINT('Ctrl Pts',(3.9923468788101,1.,0.767968531377915));
#36316=CARTESIAN_POINT('Ctrl Pts',(3.99989129179622,-1.,0.766412457136064));
#36317=CARTESIAN_POINT('Ctrl Pts',(3.99989129179622,1.,0.766412457136064));
#36318=CARTESIAN_POINT('Ctrl Pts',(4.00743706791509,-1.,0.764817648785198));
#36319=CARTESIAN_POINT('Ctrl Pts',(4.00743706791509,1.,0.764817648785198));
#36320=CARTESIAN_POINT('Ctrl Pts',(4.01498370680496,-1.,0.763184371182936));
#36321=CARTESIAN_POINT('Ctrl Pts',(4.01498370680496,1.,0.763184371182936));
#36322=CARTESIAN_POINT('Ctrl Pts',(4.02253072741268,-1.,0.761512875859805));
#36323=CARTESIAN_POINT('Ctrl Pts',(4.02253072741268,1.,0.761512875859805));
#36324=CARTESIAN_POINT('Ctrl Pts',(4.03007781954412,-1.,0.759803433243752));
#36325=CARTESIAN_POINT('Ctrl Pts',(4.03007781954412,1.,0.759803433243752));
#36326=CARTESIAN_POINT('Ctrl Pts',(4.03762485803119,-1.,0.758056338884945));
#36327=CARTESIAN_POINT('Ctrl Pts',(4.03762485803119,1.,0.758056338884945));
#36328=CARTESIAN_POINT('Ctrl Pts',(4.04517182653997,-1.,0.756271902369581));
#36329=CARTESIAN_POINT('Ctrl Pts',(4.04517182653997,1.,0.756271902369581));
#36330=CARTESIAN_POINT('Ctrl Pts',(4.05271876687915,-1.,0.754450441816078));
#36331=CARTESIAN_POINT('Ctrl Pts',(4.05271876687915,1.,0.754450441816078));
#36332=CARTESIAN_POINT('Ctrl Pts',(4.06026572221515,-1.,0.752592276483073));
#36333=CARTESIAN_POINT('Ctrl Pts',(4.06026572221515,1.,0.752592276483073));
#36334=CARTESIAN_POINT('Ctrl Pts',(4.06781267242378,-1.,0.750697720484037));
#36335=CARTESIAN_POINT('Ctrl Pts',(4.06781267242378,1.,0.750697720484037));
#36336=CARTESIAN_POINT('Ctrl Pts',(4.07535951056152,-1.,0.748767076680558));
#36337=CARTESIAN_POINT('Ctrl Pts',(4.07535951056152,1.,0.748767076680558));
#36338=CARTESIAN_POINT('Ctrl Pts',(4.08290608095642,-1.,0.746800631492316));
#36339=CARTESIAN_POINT('Ctrl Pts',(4.08290608095642,1.,0.746800631492316));
#36340=CARTESIAN_POINT('Ctrl Pts',(4.09045220253573,-1.,0.744798649706501));
#36341=CARTESIAN_POINT('Ctrl Pts',(4.09045220253573,1.,0.744798649706501));
#36342=CARTESIAN_POINT('Ctrl Pts',(4.09799769702611,-1.,0.742761369689842));
#36343=CARTESIAN_POINT('Ctrl Pts',(4.09799769702611,1.,0.742761369689842));
#36344=CARTESIAN_POINT('Ctrl Pts',(4.10554241757547,-1.,0.740688998553377));
#36345=CARTESIAN_POINT('Ctrl Pts',(4.10554241757547,1.,0.740688998553377));
#36346=CARTESIAN_POINT('Ctrl Pts',(4.11308626951927,-1.,0.738581708225844));
#36347=CARTESIAN_POINT('Ctrl Pts',(4.11308626951927,1.,0.738581708225844));
#36348=CARTESIAN_POINT('Ctrl Pts',(4.120629196238,-1.,0.736439634331345));
#36349=CARTESIAN_POINT('Ctrl Pts',(4.120629196238,1.,0.736439634331345));
#36350=CARTESIAN_POINT('Ctrl Pts',(4.12666277570844,-1.,0.734698226764093));
#36351=CARTESIAN_POINT('Ctrl Pts',(4.12666277570844,1.,0.734698226764093));
#36352=CARTESIAN_POINT('Ctrl Pts',(4.13118752795207,-1.,0.733376589323547));
#36353=CARTESIAN_POINT('Ctrl Pts',(4.13118752795207,1.,0.733376589323547));
#36354=CARTESIAN_POINT('Ctrl Pts',(4.1342038373684,-1.,0.73248857513516));
#36355=CARTESIAN_POINT('Ctrl Pts',(4.1342038373684,1.,0.73248857513516));
#36356=CARTESIAN_POINT('Ctrl Pts',(4.13571194405636,-1.,0.732042837400621));
#36357=CARTESIAN_POINT('Ctrl Pts',(4.13571194405636,1.,0.732042837400621));
#36358=CARTESIAN_POINT('',(3.66661143271685,1.,0.786422660831985));
#36359=CARTESIAN_POINT('Ctrl Pts',(3.66661143271685,-1.,0.786422660831986));
#36360=CARTESIAN_POINT('Ctrl Pts',(3.66661143271685,-0.666666666666667,
0.786422660831986));
#36361=CARTESIAN_POINT('Ctrl Pts',(3.66661143271685,-0.333333333333333,
0.786422660831986));
#36362=CARTESIAN_POINT('Ctrl Pts',(3.66661143271685,0.333333333333333,0.786422660831986));
#36363=CARTESIAN_POINT('Ctrl Pts',(3.66661143271685,0.666666666666667,0.786422660831986));
#36364=CARTESIAN_POINT('Ctrl Pts',(3.66661143271685,1.,0.786422660831986));
#36365=CARTESIAN_POINT('',(4.13571194405636,1.,0.732042837400621));
#36366=CARTESIAN_POINT('',(4.13571194405636,0.,0.732042837400621));
#36367=CARTESIAN_POINT('Ctrl Pts',(3.66661143271685,1.,0.786422660831985));
#36368=CARTESIAN_POINT('Ctrl Pts',(3.6666431041522,1.,0.786459983895432));
#36369=CARTESIAN_POINT('Ctrl Pts',(3.66680946938292,1.,0.786565919558984));
#36370=CARTESIAN_POINT('Ctrl Pts',(3.66743103898702,1.,0.786774337198063));
#36371=CARTESIAN_POINT('Ctrl Pts',(3.66907505398677,1.,0.787145041181546));
#36372=CARTESIAN_POINT('Ctrl Pts',(3.67252923663655,1.,0.787758799995743));
#36373=CARTESIAN_POINT('Ctrl Pts',(3.67777119516252,1.,0.788569566220286));
#36374=CARTESIAN_POINT('Ctrl Pts',(3.68428439783905,1.,0.789483546064387));
#36375=CARTESIAN_POINT('Ctrl Pts',(3.69172044327364,1.,0.790436284988788));
#36376=CARTESIAN_POINT('Ctrl Pts',(3.69968940808721,1.,0.79135657569598));
#36377=CARTESIAN_POINT('Ctrl Pts',(3.70781724021806,1.,0.792177688845818));
#36378=CARTESIAN_POINT('Ctrl Pts',(3.71580242396124,1.,0.792848377370287));
#36379=CARTESIAN_POINT('Ctrl Pts',(3.72348797293734,1.,0.793347023784205));
#36380=CARTESIAN_POINT('Ctrl Pts',(3.73086914695805,1.,0.793682750269684));
#36381=CARTESIAN_POINT('Ctrl Pts',(3.73803280541687,1.,0.793882700937017));
#36382=CARTESIAN_POINT('Ctrl Pts',(3.74511357728861,1.,0.793982700459952));
#36383=CARTESIAN_POINT('Ctrl Pts',(3.75224692493864,1.,0.794017347371378));
#36384=CARTESIAN_POINT('Ctrl Pts',(3.75951468666257,1.,0.794008429134908));
#36385=CARTESIAN_POINT('Ctrl Pts',(3.76692626931111,1.,0.793961083688992));
#36386=CARTESIAN_POINT('Ctrl Pts',(3.77444863801212,1.,0.793870523787408));
#36387=CARTESIAN_POINT('Ctrl Pts',(3.78202460377598,1.,0.793726235781301));
#36388=CARTESIAN_POINT('Ctrl Pts',(3.78959439439235,1.,0.793516871680994));
#36389=CARTESIAN_POINT('Ctrl Pts',(3.79711921389897,1.,0.793235612973274));
#36390=CARTESIAN_POINT('Ctrl Pts',(3.80459229925637,1.,0.792882695234778));
#36391=CARTESIAN_POINT('Ctrl Pts',(3.81202588694756,1.,0.792462483517635));
#36392=CARTESIAN_POINT('Ctrl Pts',(3.81944345442249,1.,0.791981740718635));
#36393=CARTESIAN_POINT('Ctrl Pts',(3.82687033899792,1.,0.791447528662369));
#36394=CARTESIAN_POINT('Ctrl Pts',(3.83432392054786,1.,0.790865012705301));
#36395=CARTESIAN_POINT('Ctrl Pts',(3.84180762342454,1.,0.790236124191243));
#36396=CARTESIAN_POINT('Ctrl Pts',(3.84931637808894,1.,0.789560798155583));
#36397=CARTESIAN_POINT('Ctrl Pts',(3.85683995872529,1.,0.788837734090672));
#36398=CARTESIAN_POINT('Ctrl Pts',(3.86436702561345,1.,0.788065315093778));
#36399=CARTESIAN_POINT('Ctrl Pts',(3.87188916600912,1.,0.787242527617999));
#36400=CARTESIAN_POINT('Ctrl Pts',(3.8794040281819,1.,0.786369675812609));
#36401=CARTESIAN_POINT('Ctrl Pts',(3.88691313167398,1.,0.785447890340731));
#36402=CARTESIAN_POINT('Ctrl Pts',(3.89442039235103,1.,0.784478799358337));
#36403=CARTESIAN_POINT('Ctrl Pts',(3.9019303904397,1.,0.783464141529082));
#36404=CARTESIAN_POINT('Ctrl Pts',(3.90944671004542,1.,0.782405395622765));
#36405=CARTESIAN_POINT('Ctrl Pts',(3.91697036054676,1.,0.781303428618367));
#36406=CARTESIAN_POINT('Ctrl Pts',(3.92450058323823,1.,0.780158678615543));
#36407=CARTESIAN_POINT('Ctrl Pts',(3.93203552473174,1.,0.778971308134821));
#36408=CARTESIAN_POINT('Ctrl Pts',(3.93957296768103,1.,0.777741370568559));
#36409=CARTESIAN_POINT('Ctrl Pts',(3.94711101619447,1.,0.776468966697922));
#36410=CARTESIAN_POINT('Ctrl Pts',(3.9546488545231,1.,0.775154418039352));
#36411=CARTESIAN_POINT('Ctrl Pts',(3.96218649639807,1.,0.773798212026566));
#36412=CARTESIAN_POINT('Ctrl Pts',(3.96972446532772,1.,0.772400931772137));
#36413=CARTESIAN_POINT('Ctrl Pts',(3.97726349165488,1.,0.770963190030471));
#36414=CARTESIAN_POINT('Ctrl Pts',(3.98480422348451,1.,0.769485566245545));
#36415=CARTESIAN_POINT('Ctrl Pts',(3.9923468788101,1.,0.767968531377915));
#36416=CARTESIAN_POINT('Ctrl Pts',(3.99989129179622,1.,0.766412457136064));
#36417=CARTESIAN_POINT('Ctrl Pts',(4.00743706791509,1.,0.764817648785198));
#36418=CARTESIAN_POINT('Ctrl Pts',(4.01498370680496,1.,0.763184371182936));
#36419=CARTESIAN_POINT('Ctrl Pts',(4.02253072741268,1.,0.761512875859805));
#36420=CARTESIAN_POINT('Ctrl Pts',(4.03007781954412,1.,0.759803433243752));
#36421=CARTESIAN_POINT('Ctrl Pts',(4.03762485803119,1.,0.758056338884945));
#36422=CARTESIAN_POINT('Ctrl Pts',(4.04517182653997,1.,0.756271902369581));
#36423=CARTESIAN_POINT('Ctrl Pts',(4.05271876687915,1.,0.754450441816078));
#36424=CARTESIAN_POINT('Ctrl Pts',(4.06026572221515,1.,0.752592276483073));
#36425=CARTESIAN_POINT('Ctrl Pts',(4.06781267242378,1.,0.750697720484037));
#36426=CARTESIAN_POINT('Ctrl Pts',(4.07535951056152,1.,0.748767076680558));
#36427=CARTESIAN_POINT('Ctrl Pts',(4.08290608095642,1.,0.746800631492316));
#36428=CARTESIAN_POINT('Ctrl Pts',(4.09045220253573,1.,0.744798649706501));
#36429=CARTESIAN_POINT('Ctrl Pts',(4.09799769702611,1.,0.742761369689842));
#36430=CARTESIAN_POINT('Ctrl Pts',(4.10554241757547,1.,0.740688998553377));
#36431=CARTESIAN_POINT('Ctrl Pts',(4.11308626951927,1.,0.738581708225844));
#36432=CARTESIAN_POINT('Ctrl Pts',(4.120629196238,1.,0.736439634331345));
#36433=CARTESIAN_POINT('Ctrl Pts',(4.12666277570844,1.,0.734698226764093));
#36434=CARTESIAN_POINT('Ctrl Pts',(4.13118752795207,1.,0.733376589323547));
#36435=CARTESIAN_POINT('Ctrl Pts',(4.1342038373684,1.,0.73248857513516));
#36436=CARTESIAN_POINT('Ctrl Pts',(4.13571194405636,1.,0.732042837400621));
#36437=CARTESIAN_POINT('Origin',(4.13571194405636,0.,0.732042837400621));
#36438=CARTESIAN_POINT('',(4.15950947128175,1.,0.581791163835816));
#36439=CARTESIAN_POINT('Origin',(0.,0.,0.));
#36440=CARTESIAN_POINT('',(3.62400312501245,1.,0.963899035117249));
#36441=CARTESIAN_POINT('Origin',(0.,1.,0.));
#36442=CARTESIAN_POINT('Ctrl Pts',(3.62400312501245,1.,0.963899035117249));
#36443=CARTESIAN_POINT('Ctrl Pts',(3.62400312501245,0.666666666666667,0.963899035117249));
#36444=CARTESIAN_POINT('Ctrl Pts',(3.62400312501245,0.333333333333333,0.963899035117249));
#36445=CARTESIAN_POINT('Ctrl Pts',(3.62400312501245,-0.333333333333333,
0.963899035117249));
#36446=CARTESIAN_POINT('Ctrl Pts',(3.62400312501245,-0.666666666666667,
0.96389903511725));
#36447=CARTESIAN_POINT('Ctrl Pts',(3.62400312501245,-1.,0.96389903511725));
#36448=CARTESIAN_POINT('Ctrl Pts',(4.01728681790024,-1.,1.22531898815164));
#36449=CARTESIAN_POINT('Ctrl Pts',(4.01728681790024,1.,1.22531898815164));
#36450=CARTESIAN_POINT('Ctrl Pts',(4.0161454457032,-1.,1.22423716681447));
#36451=CARTESIAN_POINT('Ctrl Pts',(4.0161454457032,1.,1.22423716681447));
#36452=CARTESIAN_POINT('Ctrl Pts',(4.01386104434674,-1.,1.22207656456199));
#36453=CARTESIAN_POINT('Ctrl Pts',(4.01386104434674,1.,1.22207656456199));
#36454=CARTESIAN_POINT('Ctrl Pts',(4.01042947142681,-1.,1.21884478244983));
#36455=CARTESIAN_POINT('Ctrl Pts',(4.01042947142681,1.,1.21884478244983));
#36456=CARTESIAN_POINT('Ctrl Pts',(4.00584409524937,-1.,1.21455398918813));
#36457=CARTESIAN_POINT('Ctrl Pts',(4.00584409524937,1.,1.21455398918813));
#36458=CARTESIAN_POINT('Ctrl Pts',(4.00009577952534,-1.,1.20922097030107));
#36459=CARTESIAN_POINT('Ctrl Pts',(4.00009577952534,1.,1.20922097030107));
#36460=CARTESIAN_POINT('Ctrl Pts',(3.99433084800649,-1.,1.2039185237544));
#36461=CARTESIAN_POINT('Ctrl Pts',(3.99433084800649,1.,1.2039185237544));
#36462=CARTESIAN_POINT('Ctrl Pts',(3.98854928957287,-1.,1.19864679609596));
#36463=CARTESIAN_POINT('Ctrl Pts',(3.98854928957287,1.,1.19864679609596));
#36464=CARTESIAN_POINT('Ctrl Pts',(3.98275111052015,-1.,1.19340598349307));
#36465=CARTESIAN_POINT('Ctrl Pts',(3.98275111052015,1.,1.19340598349307));
#36466=CARTESIAN_POINT('Ctrl Pts',(3.97693634766926,-1.,1.18819633715285));
#36467=CARTESIAN_POINT('Ctrl Pts',(3.97693634766926,1.,1.18819633715285));
#36468=CARTESIAN_POINT('Ctrl Pts',(3.9711050516465,-1.,1.18301815039596));
#36469=CARTESIAN_POINT('Ctrl Pts',(3.9711050516465,1.,1.18301815039596));
#36470=CARTESIAN_POINT('Ctrl Pts',(3.96525726357682,-1.,1.17787174135446));
#36471=CARTESIAN_POINT('Ctrl Pts',(3.96525726357682,1.,1.17787174135446));
#36472=CARTESIAN_POINT('Ctrl Pts',(3.95939299213164,-1.,1.17275743590327));
#36473=CARTESIAN_POINT('Ctrl Pts',(3.95939299213164,1.,1.17275743590327));
#36474=CARTESIAN_POINT('Ctrl Pts',(3.95351219510062,-1.,1.16767555244495));
#36475=CARTESIAN_POINT('Ctrl Pts',(3.95351219510062,1.,1.16767555244495));
#36476=CARTESIAN_POINT('Ctrl Pts',(3.9476147478092,-1.,1.16262637999261));
#36477=CARTESIAN_POINT('Ctrl Pts',(3.9476147478092,1.,1.16262637999261));
#36478=CARTESIAN_POINT('Ctrl Pts',(3.94170046685542,-1.,1.15761018341061));
#36479=CARTESIAN_POINT('Ctrl Pts',(3.94170046685542,1.,1.15761018341061));
#36480=CARTESIAN_POINT('Ctrl Pts',(3.9357691705651,-1.,1.15262722716391));
#36481=CARTESIAN_POINT('Ctrl Pts',(3.9357691705651,1.,1.15262722716391));
#36482=CARTESIAN_POINT('Ctrl Pts',(3.92982073294334,-1.,1.14767779451147));
#36483=CARTESIAN_POINT('Ctrl Pts',(3.92982073294334,1.,1.14767779451147));
#36484=CARTESIAN_POINT('Ctrl Pts',(3.92385513133937,-1.,1.14276220561575));
#36485=CARTESIAN_POINT('Ctrl Pts',(3.92385513133937,1.,1.14276220561575));
#36486=CARTESIAN_POINT('Ctrl Pts',(3.91787251936688,-1.,1.13788084225511));
#36487=CARTESIAN_POINT('Ctrl Pts',(3.91787251936688,1.,1.13788084225511));
#36488=CARTESIAN_POINT('Ctrl Pts',(3.91187321145495,-1.,1.13303414693849));
#36489=CARTESIAN_POINT('Ctrl Pts',(3.91187321145495,1.,1.13303414693849));
#36490=CARTESIAN_POINT('Ctrl Pts',(3.90585753318622,-1.,1.12822258281518));
#36491=CARTESIAN_POINT('Ctrl Pts',(3.90585753318622,1.,1.12822258281518));
#36492=CARTESIAN_POINT('Ctrl Pts',(3.89982569749978,-1.,1.12344660099029));
#36493=CARTESIAN_POINT('Ctrl Pts',(3.89982569749978,1.,1.12344660099029));
#36494=CARTESIAN_POINT('Ctrl Pts',(3.89377768340362,-1.,1.11870660794609));
#36495=CARTESIAN_POINT('Ctrl Pts',(3.89377768340362,1.,1.11870660794609));
#36496=CARTESIAN_POINT('Ctrl Pts',(3.88771308285229,-1.,1.11400292434447));
#36497=CARTESIAN_POINT('Ctrl Pts',(3.88771308285229,1.,1.11400292434447));
#36498=CARTESIAN_POINT('Ctrl Pts',(3.88163105531791,-1.,1.10933577224029));
#36499=CARTESIAN_POINT('Ctrl Pts',(3.88163105531791,1.,1.10933577224029));
#36500=CARTESIAN_POINT('Ctrl Pts',(3.87553067187566,-1.,1.10470536603303));
#36501=CARTESIAN_POINT('Ctrl Pts',(3.87553067187566,1.,1.10470536603303));
#36502=CARTESIAN_POINT('Ctrl Pts',(3.86941120134872,-1.,1.10011198761203));
#36503=CARTESIAN_POINT('Ctrl Pts',(3.86941120134872,1.,1.10011198761203));
#36504=CARTESIAN_POINT('Ctrl Pts',(3.86327241021242,-1.,1.09555606505012));
#36505=CARTESIAN_POINT('Ctrl Pts',(3.86327241021242,1.,1.09555606505012));
#36506=CARTESIAN_POINT('Ctrl Pts',(3.85711487933911,-1.,1.09103825516288));
#36507=CARTESIAN_POINT('Ctrl Pts',(3.85711487933911,1.,1.09103825516288));
#36508=CARTESIAN_POINT('Ctrl Pts',(3.8509402522269,-1.,1.08655950846377));
#36509=CARTESIAN_POINT('Ctrl Pts',(3.8509402522269,1.,1.08655950846377));
#36510=CARTESIAN_POINT('Ctrl Pts',(3.84475048030615,-1.,1.08212087917986));
#36511=CARTESIAN_POINT('Ctrl Pts',(3.84475048030615,1.,1.08212087917986));
#36512=CARTESIAN_POINT('Ctrl Pts',(3.83854714117486,-1.,1.07772335353856));
#36513=CARTESIAN_POINT('Ctrl Pts',(3.83854714117486,1.,1.07772335353856));
#36514=CARTESIAN_POINT('Ctrl Pts',(3.83233071195145,-1.,1.0733676663346));
#36515=CARTESIAN_POINT('Ctrl Pts',(3.83233071195145,1.,1.0733676663346));
#36516=CARTESIAN_POINT('Ctrl Pts',(3.82609989967278,-1.,1.0690541318036));
#36517=CARTESIAN_POINT('Ctrl Pts',(3.82609989967278,1.,1.0690541318036));
#36518=CARTESIAN_POINT('Ctrl Pts',(3.81985083953012,-1.,1.06478244038931));
#36519=CARTESIAN_POINT('Ctrl Pts',(3.81985083953012,1.,1.06478244038931));
#36520=CARTESIAN_POINT('Ctrl Pts',(3.81357866117485,-1.,1.06055206187298));
#36521=CARTESIAN_POINT('Ctrl Pts',(3.81357866117485,1.,1.06055206187298));
#36522=CARTESIAN_POINT('Ctrl Pts',(3.80727913637784,-1.,1.05636266918643));
#36523=CARTESIAN_POINT('Ctrl Pts',(3.80727913637784,1.,1.05636266918643));
#36524=CARTESIAN_POINT('Ctrl Pts',(3.80095039790678,-1.,1.05221457990015));
#36525=CARTESIAN_POINT('Ctrl Pts',(3.80095039790678,1.,1.05221457990015));
#36526=CARTESIAN_POINT('Ctrl Pts',(3.79459440308793,-1.,1.04810913267641));
#36527=CARTESIAN_POINT('Ctrl Pts',(3.79459440308793,1.,1.04810913267641));
#36528=CARTESIAN_POINT('Ctrl Pts',(3.78821910787195,-1.,1.04404924374426));
#36529=CARTESIAN_POINT('Ctrl Pts',(3.78821910787195,1.,1.04404924374426));
#36530=CARTESIAN_POINT('Ctrl Pts',(3.78183535008192,-1.,1.04003862055804));
#36531=CARTESIAN_POINT('Ctrl Pts',(3.78183535008192,1.,1.04003862055804));
#36532=CARTESIAN_POINT('Ctrl Pts',(3.77545283140445,-1.,1.03608074678013));
#36533=CARTESIAN_POINT('Ctrl Pts',(3.77545283140445,1.,1.03608074678013));
#36534=CARTESIAN_POINT('Ctrl Pts',(3.76907609832522,-1.,1.0321778660492));
#36535=CARTESIAN_POINT('Ctrl Pts',(3.76907609832522,1.,1.0321778660492));
#36536=CARTESIAN_POINT('Ctrl Pts',(3.76270122291232,-1.,1.02833014458181));
#36537=CARTESIAN_POINT('Ctrl Pts',(3.76270122291232,1.,1.02833014458181));
#36538=CARTESIAN_POINT('Ctrl Pts',(3.75631037456194,-1.,1.0245342944466));
#36539=CARTESIAN_POINT('Ctrl Pts',(3.75631037456194,1.,1.0245342944466));
#36540=CARTESIAN_POINT('Ctrl Pts',(3.74987777155834,-1.,1.02078510487428));
#36541=CARTESIAN_POINT('Ctrl Pts',(3.74987777155834,1.,1.02078510487428));
#36542=CARTESIAN_POINT('Ctrl Pts',(3.74337942504959,-1.,1.01707794311079));
#36543=CARTESIAN_POINT('Ctrl Pts',(3.74337942504959,1.,1.01707794311079));
#36544=CARTESIAN_POINT('Ctrl Pts',(3.73680245055734,-1.,1.01341114319903));
#36545=CARTESIAN_POINT('Ctrl Pts',(3.73680245055734,1.,1.01341114319903));
#36546=CARTESIAN_POINT('Ctrl Pts',(3.73015276704426,-1.,1.00978798539496));
#36547=CARTESIAN_POINT('Ctrl Pts',(3.73015276704426,1.,1.00978798539496));
#36548=CARTESIAN_POINT('Ctrl Pts',(3.72346803750595,-1.,1.0062200073571));
#36549=CARTESIAN_POINT('Ctrl Pts',(3.72346803750595,1.,1.0062200073571));
#36550=CARTESIAN_POINT('Ctrl Pts',(3.71680667125118,-1.,1.00272423396822));
#36551=CARTESIAN_POINT('Ctrl Pts',(3.71680667125118,1.,1.00272423396822));
#36552=CARTESIAN_POINT('Ctrl Pts',(3.71022439713938,-1.,0.999317260756531));
#36553=CARTESIAN_POINT('Ctrl Pts',(3.71022439713938,1.,0.999317260756531));
#36554=CARTESIAN_POINT('Ctrl Pts',(3.70375282282138,-1.,0.996009819772518));
#36555=CARTESIAN_POINT('Ctrl Pts',(3.70375282282138,1.,0.996009819772518));
#36556=CARTESIAN_POINT('Ctrl Pts',(3.69738123415662,-1.,0.992802218332011));
#36557=CARTESIAN_POINT('Ctrl Pts',(3.69738123415662,1.,0.992802218332011));
#36558=CARTESIAN_POINT('Ctrl Pts',(3.69102682138846,-1.,0.989676715398559));
#36559=CARTESIAN_POINT('Ctrl Pts',(3.69102682138846,1.,0.989676715398559));
#36560=CARTESIAN_POINT('Ctrl Pts',(3.68455317926068,-1.,0.986602639863838));
#36561=CARTESIAN_POINT('Ctrl Pts',(3.68455317926068,1.,0.986602639863838));
#36562=CARTESIAN_POINT('Ctrl Pts',(3.67782408841715,-1.,0.98355079147042));
#36563=CARTESIAN_POINT('Ctrl Pts',(3.67782408841715,1.,0.98355079147042));
#36564=CARTESIAN_POINT('Ctrl Pts',(3.67074983340361,-1.,0.980505922458267));
#36565=CARTESIAN_POINT('Ctrl Pts',(3.67074983340361,1.,0.980505922458267));
#36566=CARTESIAN_POINT('Ctrl Pts',(3.66333049637475,-1.,0.977478312751618));
#36567=CARTESIAN_POINT('Ctrl Pts',(3.66333049637475,1.,0.977478312751618));
#36568=CARTESIAN_POINT('Ctrl Pts',(3.65571576735126,-1.,0.974519971354849));
#36569=CARTESIAN_POINT('Ctrl Pts',(3.65571576735126,1.,0.974519971354849));
#36570=CARTESIAN_POINT('Ctrl Pts',(3.64819756447455,-1.,0.971722122061341));
#36571=CARTESIAN_POINT('Ctrl Pts',(3.64819756447455,1.,0.971722122061341));
#36572=CARTESIAN_POINT('Ctrl Pts',(3.64113946505766,-1.,0.969195124675866));
#36573=CARTESIAN_POINT('Ctrl Pts',(3.64113946505766,1.,0.969195124675866));
#36574=CARTESIAN_POINT('Ctrl Pts',(3.63492122081143,-1.,0.967052554541386));
#36575=CARTESIAN_POINT('Ctrl Pts',(3.63492122081143,1.,0.967052554541386));
#36576=CARTESIAN_POINT('Ctrl Pts',(3.62988252139846,-1.,0.965395153165294));
#36577=CARTESIAN_POINT('Ctrl Pts',(3.62988252139846,1.,0.965395153165294));
#36578=CARTESIAN_POINT('Ctrl Pts',(3.62625391254797,-1.,0.964291001273288));
#36579=CARTESIAN_POINT('Ctrl Pts',(3.62625391254797,1.,0.964291001273288));
#36580=CARTESIAN_POINT('Ctrl Pts',(3.6245656860652,-1.,0.96387577453062));
#36581=CARTESIAN_POINT('Ctrl Pts',(3.6245656860652,1.,0.96387577453062));
#36582=CARTESIAN_POINT('Ctrl Pts',(3.62399933639914,-1.,0.963832486395052));
#36583=CARTESIAN_POINT('Ctrl Pts',(3.62399933639914,1.,0.963832486395052));
#36584=CARTESIAN_POINT('Ctrl Pts',(3.62393257642052,-1.,0.963922720982194));
#36585=CARTESIAN_POINT('Ctrl Pts',(3.62393257642052,1.,0.963922720982194));
#36586=CARTESIAN_POINT('Ctrl Pts',(3.62397690409552,-1.,0.963997613369571));
#36587=CARTESIAN_POINT('Ctrl Pts',(3.62397690409552,1.,0.963997613369571));
#36588=CARTESIAN_POINT('',(4.01728681790024,1.,1.22531898815164));
#36589=CARTESIAN_POINT('Ctrl Pts',(4.01728681790024,1.,1.22531898815164));
#36590=CARTESIAN_POINT('Ctrl Pts',(4.0161454457032,1.,1.22423716681447));
#36591=CARTESIAN_POINT('Ctrl Pts',(4.01386104434674,1.,1.22207656456199));
#36592=CARTESIAN_POINT('Ctrl Pts',(4.01042947142681,1.,1.21884478244983));
#36593=CARTESIAN_POINT('Ctrl Pts',(4.00584409524937,1.,1.21455398918813));
#36594=CARTESIAN_POINT('Ctrl Pts',(4.00009577952534,1.,1.20922097030107));
#36595=CARTESIAN_POINT('Ctrl Pts',(3.99433084800649,1.,1.2039185237544));
#36596=CARTESIAN_POINT('Ctrl Pts',(3.98854928957287,1.,1.19864679609596));
#36597=CARTESIAN_POINT('Ctrl Pts',(3.98275111052015,1.,1.19340598349307));
#36598=CARTESIAN_POINT('Ctrl Pts',(3.97693634766926,1.,1.18819633715285));
#36599=CARTESIAN_POINT('Ctrl Pts',(3.9711050516465,1.,1.18301815039596));
#36600=CARTESIAN_POINT('Ctrl Pts',(3.96525726357682,1.,1.17787174135446));
#36601=CARTESIAN_POINT('Ctrl Pts',(3.95939299213164,1.,1.17275743590327));
#36602=CARTESIAN_POINT('Ctrl Pts',(3.95351219510062,1.,1.16767555244495));
#36603=CARTESIAN_POINT('Ctrl Pts',(3.9476147478092,1.,1.16262637999261));
#36604=CARTESIAN_POINT('Ctrl Pts',(3.94170046685542,1.,1.15761018341061));
#36605=CARTESIAN_POINT('Ctrl Pts',(3.9357691705651,1.,1.15262722716391));
#36606=CARTESIAN_POINT('Ctrl Pts',(3.92982073294334,1.,1.14767779451147));
#36607=CARTESIAN_POINT('Ctrl Pts',(3.92385513133937,1.,1.14276220561575));
#36608=CARTESIAN_POINT('Ctrl Pts',(3.91787251936688,1.,1.13788084225511));
#36609=CARTESIAN_POINT('Ctrl Pts',(3.91187321145495,1.,1.13303414693849));
#36610=CARTESIAN_POINT('Ctrl Pts',(3.90585753318622,1.,1.12822258281518));
#36611=CARTESIAN_POINT('Ctrl Pts',(3.89982569749978,1.,1.12344660099029));
#36612=CARTESIAN_POINT('Ctrl Pts',(3.89377768340362,1.,1.11870660794609));
#36613=CARTESIAN_POINT('Ctrl Pts',(3.88771308285229,1.,1.11400292434447));
#36614=CARTESIAN_POINT('Ctrl Pts',(3.88163105531791,1.,1.10933577224029));
#36615=CARTESIAN_POINT('Ctrl Pts',(3.87553067187566,1.,1.10470536603303));
#36616=CARTESIAN_POINT('Ctrl Pts',(3.86941120134872,1.,1.10011198761203));
#36617=CARTESIAN_POINT('Ctrl Pts',(3.86327241021242,1.,1.09555606505012));
#36618=CARTESIAN_POINT('Ctrl Pts',(3.85711487933911,1.,1.09103825516288));
#36619=CARTESIAN_POINT('Ctrl Pts',(3.8509402522269,1.,1.08655950846377));
#36620=CARTESIAN_POINT('Ctrl Pts',(3.84475048030615,1.,1.08212087917986));
#36621=CARTESIAN_POINT('Ctrl Pts',(3.83854714117486,1.,1.07772335353856));
#36622=CARTESIAN_POINT('Ctrl Pts',(3.83233071195145,1.,1.0733676663346));
#36623=CARTESIAN_POINT('Ctrl Pts',(3.82609989967278,1.,1.0690541318036));
#36624=CARTESIAN_POINT('Ctrl Pts',(3.81985083953012,1.,1.06478244038931));
#36625=CARTESIAN_POINT('Ctrl Pts',(3.81357866117485,1.,1.06055206187298));
#36626=CARTESIAN_POINT('Ctrl Pts',(3.80727913637784,1.,1.05636266918643));
#36627=CARTESIAN_POINT('Ctrl Pts',(3.80095039790678,1.,1.05221457990015));
#36628=CARTESIAN_POINT('Ctrl Pts',(3.79459440308793,1.,1.04810913267641));
#36629=CARTESIAN_POINT('Ctrl Pts',(3.78821910787195,1.,1.04404924374426));
#36630=CARTESIAN_POINT('Ctrl Pts',(3.78183535008192,1.,1.04003862055804));
#36631=CARTESIAN_POINT('Ctrl Pts',(3.77545283140445,1.,1.03608074678013));
#36632=CARTESIAN_POINT('Ctrl Pts',(3.76907609832522,1.,1.0321778660492));
#36633=CARTESIAN_POINT('Ctrl Pts',(3.76270122291232,1.,1.02833014458181));
#36634=CARTESIAN_POINT('Ctrl Pts',(3.75631037456194,1.,1.0245342944466));
#36635=CARTESIAN_POINT('Ctrl Pts',(3.74987777155834,1.,1.02078510487428));
#36636=CARTESIAN_POINT('Ctrl Pts',(3.74337942504959,1.,1.01707794311079));
#36637=CARTESIAN_POINT('Ctrl Pts',(3.73680245055734,1.,1.01341114319903));
#36638=CARTESIAN_POINT('Ctrl Pts',(3.73015276704426,1.,1.00978798539496));
#36639=CARTESIAN_POINT('Ctrl Pts',(3.72346803750595,1.,1.0062200073571));
#36640=CARTESIAN_POINT('Ctrl Pts',(3.71680667125118,1.,1.00272423396822));
#36641=CARTESIAN_POINT('Ctrl Pts',(3.71022439713938,1.,0.999317260756531));
#36642=CARTESIAN_POINT('Ctrl Pts',(3.70375282282138,1.,0.996009819772518));
#36643=CARTESIAN_POINT('Ctrl Pts',(3.69738123415662,1.,0.992802218332011));
#36644=CARTESIAN_POINT('Ctrl Pts',(3.69102682138846,1.,0.989676715398559));
#36645=CARTESIAN_POINT('Ctrl Pts',(3.68455317926068,1.,0.986602639863838));
#36646=CARTESIAN_POINT('Ctrl Pts',(3.67782408841715,1.,0.98355079147042));
#36647=CARTESIAN_POINT('Ctrl Pts',(3.67074983340361,1.,0.980505922458267));
#36648=CARTESIAN_POINT('Ctrl Pts',(3.66333049637475,1.,0.977478312751618));
#36649=CARTESIAN_POINT('Ctrl Pts',(3.65571576735126,1.,0.974519971354849));
#36650=CARTESIAN_POINT('Ctrl Pts',(3.64819756447455,1.,0.971722122061341));
#36651=CARTESIAN_POINT('Ctrl Pts',(3.64113946505766,1.,0.969195124675866));
#36652=CARTESIAN_POINT('Ctrl Pts',(3.63492122081143,1.,0.967052554541386));
#36653=CARTESIAN_POINT('Ctrl Pts',(3.62988252139846,1.,0.965395153165294));
#36654=CARTESIAN_POINT('Ctrl Pts',(3.62652618145335,1.,0.964373850166458));
#36655=CARTESIAN_POINT('Ctrl Pts',(3.62489305727662,1.,0.963957782642844));
#36656=CARTESIAN_POINT('Ctrl Pts',(3.62424461507588,1.,0.963861297423241));
#36657=CARTESIAN_POINT('Ctrl Pts',(3.6240482887845,1.,0.963880158555582));
#36658=CARTESIAN_POINT('Ctrl Pts',(3.62400312501245,1.,0.963899035117249));
#36659=CARTESIAN_POINT('',(4.01728681790024,0.,1.22531898815164));
#36660=CARTESIAN_POINT('Ctrl Pts',(3.49848248301936,-1.,1.35022972712301));
#36661=CARTESIAN_POINT('Ctrl Pts',(3.49848248301936,1.,1.35022972712301));
#36662=CARTESIAN_POINT('Ctrl Pts',(3.4984026005375,-1.,1.35026426118402));
#36663=CARTESIAN_POINT('Ctrl Pts',(3.4984026005375,1.,1.35026426118402));
#36664=CARTESIAN_POINT('Ctrl Pts',(3.49840357193736,-1.,1.35037650303019));
#36665=CARTESIAN_POINT('Ctrl Pts',(3.49840357193736,1.,1.35037650303019));
#36666=CARTESIAN_POINT('Ctrl Pts',(3.49888720257132,-1.,1.35067437417484));
#36667=CARTESIAN_POINT('Ctrl Pts',(3.49888720257132,1.,1.35067437417484));
#36668=CARTESIAN_POINT('Ctrl Pts',(3.5004970706414,-1.,1.3513307633124));
#36669=CARTESIAN_POINT('Ctrl Pts',(3.5004970706414,1.,1.3513307633124));
#36670=CARTESIAN_POINT('Ctrl Pts',(3.50408168106261,-1.,1.35257032843486));
#36671=CARTESIAN_POINT('Ctrl Pts',(3.50408168106261,1.,1.35257032843486));
#36672=CARTESIAN_POINT('Ctrl Pts',(3.50913227059999,-1.,1.35419113575956));
#36673=CARTESIAN_POINT('Ctrl Pts',(3.50913227059999,1.,1.35419113575956));
#36674=CARTESIAN_POINT('Ctrl Pts',(3.51542230699556,-1.,1.35611275237152));
#36675=CARTESIAN_POINT('Ctrl Pts',(3.51542230699556,1.,1.35611275237152));
#36676=CARTESIAN_POINT('Ctrl Pts',(3.52261776116748,-1.,1.35821701528836));
#36677=CARTESIAN_POINT('Ctrl Pts',(3.52261776116748,1.,1.35821701528836));
#36678=CARTESIAN_POINT('Ctrl Pts',(3.530344649616,-1.,1.36037259643734));
#36679=CARTESIAN_POINT('Ctrl Pts',(3.530344649616,1.,1.36037259643734));
#36680=CARTESIAN_POINT('Ctrl Pts',(3.53824396424961,-1.,1.36245507339307));
#36681=CARTESIAN_POINT('Ctrl Pts',(3.53824396424961,1.,1.36245507339307));
#36682=CARTESIAN_POINT('Ctrl Pts',(3.54602591832973,-1.,1.36436666257598));
#36683=CARTESIAN_POINT('Ctrl Pts',(3.54602591832973,1.,1.36436666257598));
#36684=CARTESIAN_POINT('Ctrl Pts',(3.55353883995949,-1.,1.3660614545677));
#36685=CARTESIAN_POINT('Ctrl Pts',(3.55353883995949,1.,1.3660614545677));
#36686=CARTESIAN_POINT('Ctrl Pts',(3.56077662028649,-1.,1.36754771771233));
#36687=CARTESIAN_POINT('Ctrl Pts',(3.56077662028649,1.,1.36754771771233));
#36688=CARTESIAN_POINT('Ctrl Pts',(3.5678208030466,-1.,1.36886584973389));
#36689=CARTESIAN_POINT('Ctrl Pts',(3.5678208030466,1.,1.36886584973389));
#36690=CARTESIAN_POINT('Ctrl Pts',(3.57479875549486,-1.,1.37007229485659));
#36691=CARTESIAN_POINT('Ctrl Pts',(3.57479875549486,1.,1.37007229485659));
#36692=CARTESIAN_POINT('Ctrl Pts',(3.58183885982715,-1.,1.37122241663062));
#36693=CARTESIAN_POINT('Ctrl Pts',(3.58183885982715,1.,1.37122241663062));
#36694=CARTESIAN_POINT('Ctrl Pts',(3.58901853846365,-1.,1.37235053660976));
#36695=CARTESIAN_POINT('Ctrl Pts',(3.58901853846365,1.,1.37235053660976));
#36696=CARTESIAN_POINT('Ctrl Pts',(3.59634627869048,-1.,1.37346320103157));
#36697=CARTESIAN_POINT('Ctrl Pts',(3.59634627869048,1.,1.37346320103157));
#36698=CARTESIAN_POINT('Ctrl Pts',(3.60379020123988,-1.,1.37455051379623));
#36699=CARTESIAN_POINT('Ctrl Pts',(3.60379020123988,1.,1.37455051379623));
#36700=CARTESIAN_POINT('Ctrl Pts',(3.61129546591064,-1.,1.37559314436634));
#36701=CARTESIAN_POINT('Ctrl Pts',(3.61129546591064,1.,1.37559314436634));
#36702=CARTESIAN_POINT('Ctrl Pts',(3.6188048116042,-1.,1.37657053403107));
#36703=CARTESIAN_POINT('Ctrl Pts',(3.6188048116042,1.,1.37657053403107));
#36704=CARTESIAN_POINT('Ctrl Pts',(3.62628098665145,-1.,1.37746987919881));
#36705=CARTESIAN_POINT('Ctrl Pts',(3.62628098665145,1.,1.37746987919881));
#36706=CARTESIAN_POINT('Ctrl Pts',(3.63371727442486,-1.,1.37829035457339));
#36707=CARTESIAN_POINT('Ctrl Pts',(3.63371727442486,1.,1.37829035457339));
#36708=CARTESIAN_POINT('Ctrl Pts',(3.64112507791141,-1.,1.37903818567359));
#36709=CARTESIAN_POINT('Ctrl Pts',(3.64112507791141,1.,1.37903818567359));
#36710=CARTESIAN_POINT('Ctrl Pts',(3.64852652756456,-1.,1.37972372481603));
#36711=CARTESIAN_POINT('Ctrl Pts',(3.64852652756456,1.,1.37972372481603));
#36712=CARTESIAN_POINT('Ctrl Pts',(3.6559455440439,-1.,1.38035791051213));
#36713=CARTESIAN_POINT('Ctrl Pts',(3.6559455440439,1.,1.38035791051213));
#36714=CARTESIAN_POINT('Ctrl Pts',(3.66339848520857,-1.,1.38094856333552));
#36715=CARTESIAN_POINT('Ctrl Pts',(3.66339848520857,1.,1.38094856333552));
#36716=CARTESIAN_POINT('Ctrl Pts',(3.67088843112262,-1.,1.38149812653868));
#36717=CARTESIAN_POINT('Ctrl Pts',(3.67088843112262,1.,1.38149812653868));
#36718=CARTESIAN_POINT('Ctrl Pts',(3.67841038482414,-1.,1.3820057429062));
#36719=CARTESIAN_POINT('Ctrl Pts',(3.67841038482414,1.,1.3820057429062));
#36720=CARTESIAN_POINT('Ctrl Pts',(3.68595444983837,-1.,1.38246852827182));
#36721=CARTESIAN_POINT('Ctrl Pts',(3.68595444983837,1.,1.38246852827182));
#36722=CARTESIAN_POINT('Ctrl Pts',(3.69350967899526,-1.,1.38288311171651));
#36723=CARTESIAN_POINT('Ctrl Pts',(3.69350967899526,1.,1.38288311171651));
#36724=CARTESIAN_POINT('Ctrl Pts',(3.701067921679,-1.,1.38324717612865));
#36725=CARTESIAN_POINT('Ctrl Pts',(3.701067921679,1.,1.38324717612865));
#36726=CARTESIAN_POINT('Ctrl Pts',(3.70862680753347,-1.,1.38356065402124));
#36727=CARTESIAN_POINT('Ctrl Pts',(3.70862680753347,1.,1.38356065402124));
#36728=CARTESIAN_POINT('Ctrl Pts',(3.7161876605181,-1.,1.38382489984586));
#36729=CARTESIAN_POINT('Ctrl Pts',(3.7161876605181,1.,1.38382489984586));
#36730=CARTESIAN_POINT('Ctrl Pts',(3.72375409358803,-1.,1.3840421342895));
#36731=CARTESIAN_POINT('Ctrl Pts',(3.72375409358803,1.,1.3840421342895));
#36732=CARTESIAN_POINT('Ctrl Pts',(3.73133035859282,-1.,1.38421479111531));
#36733=CARTESIAN_POINT('Ctrl Pts',(3.73133035859282,1.,1.38421479111531));
#36734=CARTESIAN_POINT('Ctrl Pts',(3.73891976418104,-1.,1.38434489156458));
#36735=CARTESIAN_POINT('Ctrl Pts',(3.73891976418104,1.,1.38434489156458));
#36736=CARTESIAN_POINT('Ctrl Pts',(3.74652317167876,-1.,1.38443344984394));
#36737=CARTESIAN_POINT('Ctrl Pts',(3.74652317167876,1.,1.38443344984394));
#36738=CARTESIAN_POINT('Ctrl Pts',(3.7541397631875,-1.,1.38448077997163));
#36739=CARTESIAN_POINT('Ctrl Pts',(3.7541397631875,1.,1.38448077997163));
#36740=CARTESIAN_POINT('Ctrl Pts',(3.76176768271367,-1.,1.3844867525335));
#36741=CARTESIAN_POINT('Ctrl Pts',(3.76176768271367,1.,1.3844867525335));
#36742=CARTESIAN_POINT('Ctrl Pts',(3.76940473185779,-1.,1.38445107339518));
#36743=CARTESIAN_POINT('Ctrl Pts',(3.76940473185779,1.,1.38445107339518));
#36744=CARTESIAN_POINT('Ctrl Pts',(3.77704902230418,-1.,1.38437354551428));
#36745=CARTESIAN_POINT('Ctrl Pts',(3.77704902230418,1.,1.38437354551428));
#36746=CARTESIAN_POINT('Ctrl Pts',(3.78469969805082,-1.,1.38425435883756));
#36747=CARTESIAN_POINT('Ctrl Pts',(3.78469969805082,1.,1.38425435883756));
#36748=CARTESIAN_POINT('Ctrl Pts',(3.79235669640841,-1.,1.38409399694566));
#36749=CARTESIAN_POINT('Ctrl Pts',(3.79235669640841,1.,1.38409399694566));
#36750=CARTESIAN_POINT('Ctrl Pts',(3.80002044322111,-1.,1.38389311766682));
#36751=CARTESIAN_POINT('Ctrl Pts',(3.80002044322111,1.,1.38389311766682));
#36752=CARTESIAN_POINT('Ctrl Pts',(3.80769156398411,-1.,1.3836524404622));
#36753=CARTESIAN_POINT('Ctrl Pts',(3.80769156398411,1.,1.3836524404622));
#36754=CARTESIAN_POINT('Ctrl Pts',(3.81537060817811,-1.,1.38337263902782));
#36755=CARTESIAN_POINT('Ctrl Pts',(3.81537060817811,1.,1.38337263902782));
#36756=CARTESIAN_POINT('Ctrl Pts',(3.82305771743829,-1.,1.38305421262763));
#36757=CARTESIAN_POINT('Ctrl Pts',(3.82305771743829,1.,1.38305421262763));
#36758=CARTESIAN_POINT('Ctrl Pts',(3.8307526698229,-1.,1.38269750245138));
#36759=CARTESIAN_POINT('Ctrl Pts',(3.8307526698229,1.,1.38269750245138));
#36760=CARTESIAN_POINT('Ctrl Pts',(3.83845502790746,-1.,1.38230274828822));
#36761=CARTESIAN_POINT('Ctrl Pts',(3.83845502790746,1.,1.38230274828822));
#36762=CARTESIAN_POINT('Ctrl Pts',(3.84616425605764,-1.,1.38187013346109));
#36763=CARTESIAN_POINT('Ctrl Pts',(3.84616425605764,1.,1.38187013346109));
#36764=CARTESIAN_POINT('Ctrl Pts',(3.85387983979481,-1.,1.3813998311505));
#36765=CARTESIAN_POINT('Ctrl Pts',(3.85387983979481,1.,1.3813998311505));
#36766=CARTESIAN_POINT('Ctrl Pts',(3.86160143043959,-1.,1.3808920599299));
#36767=CARTESIAN_POINT('Ctrl Pts',(3.86160143043959,1.,1.3808920599299));
#36768=CARTESIAN_POINT('Ctrl Pts',(3.86932885813068,-1.,1.38034709213014));
#36769=CARTESIAN_POINT('Ctrl Pts',(3.86932885813068,1.,1.38034709213014));
#36770=CARTESIAN_POINT('Ctrl Pts',(3.87706205830532,-1.,1.37976523097073));
#36771=CARTESIAN_POINT('Ctrl Pts',(3.87706205830532,1.,1.37976523097073));
#36772=CARTESIAN_POINT('Ctrl Pts',(3.88480102249277,-1.,1.37914679719383));
#36773=CARTESIAN_POINT('Ctrl Pts',(3.88480102249277,1.,1.37914679719383));
#36774=CARTESIAN_POINT('Ctrl Pts',(3.89254574338496,-1.,1.3784921128802));
#36775=CARTESIAN_POINT('Ctrl Pts',(3.89254574338496,1.,1.3784921128802));
#36776=CARTESIAN_POINT('Ctrl Pts',(3.90029615196727,-1.,1.37780148512792));
#36777=CARTESIAN_POINT('Ctrl Pts',(3.90029615196727,1.,1.37780148512792));
#36778=CARTESIAN_POINT('Ctrl Pts',(3.90805209523486,-1.,1.3770751963402));
#36779=CARTESIAN_POINT('Ctrl Pts',(3.90805209523486,1.,1.3770751963402));
#36780=CARTESIAN_POINT('Ctrl Pts',(3.91581337462644,-1.,1.37631350505797));
#36781=CARTESIAN_POINT('Ctrl Pts',(3.91581337462644,1.,1.37631350505797));
#36782=CARTESIAN_POINT('Ctrl Pts',(3.92357976987672,-1.,1.37551664448242));
#36783=CARTESIAN_POINT('Ctrl Pts',(3.92357976987672,1.,1.37551664448242));
#36784=CARTESIAN_POINT('Ctrl Pts',(3.93135106761844,-1.,1.37468482215751));
#36785=CARTESIAN_POINT('Ctrl Pts',(3.93135106761844,1.,1.37468482215751));
#36786=CARTESIAN_POINT('Ctrl Pts',(3.93912709040818,-1.,1.37381821967165));
#36787=CARTESIAN_POINT('Ctrl Pts',(3.93912709040818,1.,1.37381821967165));
#36788=CARTESIAN_POINT('Ctrl Pts',(3.94690771785133,-1.,1.37291699202807));
#36789=CARTESIAN_POINT('Ctrl Pts',(3.94690771785133,1.,1.37291699202807));
#36790=CARTESIAN_POINT('Ctrl Pts',(3.95469287280914,-1.,1.37198126432386));
#36791=CARTESIAN_POINT('Ctrl Pts',(3.95469287280914,1.,1.37198126432386));
#36792=CARTESIAN_POINT('Ctrl Pts',(3.96092458506535,-1.,1.3712051561502));
#36793=CARTESIAN_POINT('Ctrl Pts',(3.96092458506535,1.,1.3712051561502));
#36794=CARTESIAN_POINT('Ctrl Pts',(3.96560037974645,-1.,1.37060761745635));
#36795=CARTESIAN_POINT('Ctrl Pts',(3.96560037974645,1.,1.37060761745635));
#36796=CARTESIAN_POINT('Ctrl Pts',(3.9687184694131,-1.,1.37020239094614));
#36797=CARTESIAN_POINT('Ctrl Pts',(3.9687184694131,1.,1.37020239094614));
#36798=CARTESIAN_POINT('Ctrl Pts',(3.97027773754922,-1.,1.36999806084573));
#36799=CARTESIAN_POINT('Ctrl Pts',(3.97027773754922,1.,1.36999806084573));
#36800=CARTESIAN_POINT('',(3.4984457533445,1.,1.35032489087101));
#36801=CARTESIAN_POINT('Ctrl Pts',(3.4984457533445,-1.,1.35032489087101));
#36802=CARTESIAN_POINT('Ctrl Pts',(3.4984457533445,-0.666666666666667,1.35032489087101));
#36803=CARTESIAN_POINT('Ctrl Pts',(3.4984457533445,-0.333333333333333,1.35032489087101));
#36804=CARTESIAN_POINT('Ctrl Pts',(3.4984457533445,0.333333333333333,1.35032489087101));
#36805=CARTESIAN_POINT('Ctrl Pts',(3.4984457533445,0.666666666666667,1.35032489087101));
#36806=CARTESIAN_POINT('Ctrl Pts',(3.4984457533445,1.,1.35032489087101));
#36807=CARTESIAN_POINT('',(3.97027773754922,1.,1.36999806084573));
#36808=CARTESIAN_POINT('',(3.97027773754922,0.,1.36999806084573));
#36809=CARTESIAN_POINT('Ctrl Pts',(3.4984457533445,1.,1.35032489087101));
#36810=CARTESIAN_POINT('Ctrl Pts',(3.49847119623846,1.,1.35036670892966));
#36811=CARTESIAN_POINT('Ctrl Pts',(3.49861894124827,1.,1.35049736560527));
#36812=CARTESIAN_POINT('Ctrl Pts',(3.49920025459723,1.,1.35080045218587));
#36813=CARTESIAN_POINT('Ctrl Pts',(3.5007660381649,1.,1.35142377279517));
#36814=CARTESIAN_POINT('Ctrl Pts',(3.50408168106261,1.,1.35257032843486));
#36815=CARTESIAN_POINT('Ctrl Pts',(3.50913227059999,1.,1.35419113575956));
#36816=CARTESIAN_POINT('Ctrl Pts',(3.51542230699556,1.,1.35611275237152));
#36817=CARTESIAN_POINT('Ctrl Pts',(3.52261776116748,1.,1.35821701528836));
#36818=CARTESIAN_POINT('Ctrl Pts',(3.530344649616,1.,1.36037259643734));
#36819=CARTESIAN_POINT('Ctrl Pts',(3.53824396424961,1.,1.36245507339307));
#36820=CARTESIAN_POINT('Ctrl Pts',(3.54602591832973,1.,1.36436666257598));
#36821=CARTESIAN_POINT('Ctrl Pts',(3.55353883995949,1.,1.3660614545677));
#36822=CARTESIAN_POINT('Ctrl Pts',(3.56077662028649,1.,1.36754771771233));
#36823=CARTESIAN_POINT('Ctrl Pts',(3.5678208030466,1.,1.36886584973389));
#36824=CARTESIAN_POINT('Ctrl Pts',(3.57479875549486,1.,1.37007229485659));
#36825=CARTESIAN_POINT('Ctrl Pts',(3.58183885982715,1.,1.37122241663062));
#36826=CARTESIAN_POINT('Ctrl Pts',(3.58901853846365,1.,1.37235053660976));
#36827=CARTESIAN_POINT('Ctrl Pts',(3.59634627869048,1.,1.37346320103157));
#36828=CARTESIAN_POINT('Ctrl Pts',(3.60379020123988,1.,1.37455051379623));
#36829=CARTESIAN_POINT('Ctrl Pts',(3.61129546591064,1.,1.37559314436634));
#36830=CARTESIAN_POINT('Ctrl Pts',(3.6188048116042,1.,1.37657053403107));
#36831=CARTESIAN_POINT('Ctrl Pts',(3.62628098665145,1.,1.37746987919881));
#36832=CARTESIAN_POINT('Ctrl Pts',(3.63371727442486,1.,1.37829035457339));
#36833=CARTESIAN_POINT('Ctrl Pts',(3.64112507791141,1.,1.37903818567359));
#36834=CARTESIAN_POINT('Ctrl Pts',(3.64852652756456,1.,1.37972372481603));
#36835=CARTESIAN_POINT('Ctrl Pts',(3.6559455440439,1.,1.38035791051213));
#36836=CARTESIAN_POINT('Ctrl Pts',(3.66339848520857,1.,1.38094856333552));
#36837=CARTESIAN_POINT('Ctrl Pts',(3.67088843112262,1.,1.38149812653868));
#36838=CARTESIAN_POINT('Ctrl Pts',(3.67841038482414,1.,1.3820057429062));
#36839=CARTESIAN_POINT('Ctrl Pts',(3.68595444983837,1.,1.38246852827182));
#36840=CARTESIAN_POINT('Ctrl Pts',(3.69350967899526,1.,1.38288311171651));
#36841=CARTESIAN_POINT('Ctrl Pts',(3.701067921679,1.,1.38324717612865));
#36842=CARTESIAN_POINT('Ctrl Pts',(3.70862680753347,1.,1.38356065402124));
#36843=CARTESIAN_POINT('Ctrl Pts',(3.7161876605181,1.,1.38382489984586));
#36844=CARTESIAN_POINT('Ctrl Pts',(3.72375409358803,1.,1.3840421342895));
#36845=CARTESIAN_POINT('Ctrl Pts',(3.73133035859282,1.,1.38421479111531));
#36846=CARTESIAN_POINT('Ctrl Pts',(3.73891976418104,1.,1.38434489156458));
#36847=CARTESIAN_POINT('Ctrl Pts',(3.74652317167876,1.,1.38443344984394));
#36848=CARTESIAN_POINT('Ctrl Pts',(3.7541397631875,1.,1.38448077997163));
#36849=CARTESIAN_POINT('Ctrl Pts',(3.76176768271367,1.,1.3844867525335));
#36850=CARTESIAN_POINT('Ctrl Pts',(3.76940473185779,1.,1.38445107339518));
#36851=CARTESIAN_POINT('Ctrl Pts',(3.77704902230418,1.,1.38437354551428));
#36852=CARTESIAN_POINT('Ctrl Pts',(3.78469969805082,1.,1.38425435883756));
#36853=CARTESIAN_POINT('Ctrl Pts',(3.79235669640841,1.,1.38409399694566));
#36854=CARTESIAN_POINT('Ctrl Pts',(3.80002044322111,1.,1.38389311766682));
#36855=CARTESIAN_POINT('Ctrl Pts',(3.80769156398411,1.,1.3836524404622));
#36856=CARTESIAN_POINT('Ctrl Pts',(3.81537060817811,1.,1.38337263902782));
#36857=CARTESIAN_POINT('Ctrl Pts',(3.82305771743829,1.,1.38305421262763));
#36858=CARTESIAN_POINT('Ctrl Pts',(3.8307526698229,1.,1.38269750245138));
#36859=CARTESIAN_POINT('Ctrl Pts',(3.83845502790746,1.,1.38230274828822));
#36860=CARTESIAN_POINT('Ctrl Pts',(3.84616425605764,1.,1.38187013346109));
#36861=CARTESIAN_POINT('Ctrl Pts',(3.85387983979481,1.,1.3813998311505));
#36862=CARTESIAN_POINT('Ctrl Pts',(3.86160143043959,1.,1.3808920599299));
#36863=CARTESIAN_POINT('Ctrl Pts',(3.86932885813068,1.,1.38034709213014));
#36864=CARTESIAN_POINT('Ctrl Pts',(3.87706205830532,1.,1.37976523097073));
#36865=CARTESIAN_POINT('Ctrl Pts',(3.88480102249277,1.,1.37914679719383));
#36866=CARTESIAN_POINT('Ctrl Pts',(3.89254574338496,1.,1.3784921128802));
#36867=CARTESIAN_POINT('Ctrl Pts',(3.90029615196727,1.,1.37780148512792));
#36868=CARTESIAN_POINT('Ctrl Pts',(3.90805209523486,1.,1.3770751963402));
#36869=CARTESIAN_POINT('Ctrl Pts',(3.91581337462644,1.,1.37631350505797));
#36870=CARTESIAN_POINT('Ctrl Pts',(3.92357976987672,1.,1.37551664448242));
#36871=CARTESIAN_POINT('Ctrl Pts',(3.93135106761844,1.,1.37468482215751));
#36872=CARTESIAN_POINT('Ctrl Pts',(3.93912709040818,1.,1.37381821967165));
#36873=CARTESIAN_POINT('Ctrl Pts',(3.94690771785133,1.,1.37291699202807));
#36874=CARTESIAN_POINT('Ctrl Pts',(3.95469287280914,1.,1.37198126432386));
#36875=CARTESIAN_POINT('Ctrl Pts',(3.96092458506535,1.,1.3712051561502));
#36876=CARTESIAN_POINT('Ctrl Pts',(3.96560037974645,1.,1.37060761745635));
#36877=CARTESIAN_POINT('Ctrl Pts',(3.9687184694131,1.,1.37020239094614));
#36878=CARTESIAN_POINT('Ctrl Pts',(3.97027773754922,1.,1.36999806084573));
#36879=CARTESIAN_POINT('Origin',(3.97027773754922,0.,1.36999806084573));
#36880=CARTESIAN_POINT('',(4.01728681790024,1.,1.22531898815164));
#36881=CARTESIAN_POINT('Origin',(0.,0.,0.));
#36882=CARTESIAN_POINT('',(3.42859860294378,1.,1.51895082866166));
#36883=CARTESIAN_POINT('Origin',(0.,1.,0.));
#36884=CARTESIAN_POINT('Ctrl Pts',(3.42859860294378,1.,1.51895082866166));
#36885=CARTESIAN_POINT('Ctrl Pts',(3.42859860294378,0.666666666666667,1.51895082866166));
#36886=CARTESIAN_POINT('Ctrl Pts',(3.42859860294378,0.333333333333333,1.51895082866166));
#36887=CARTESIAN_POINT('Ctrl Pts',(3.42859860294378,-0.333333333333333,
1.51895082866166));
#36888=CARTESIAN_POINT('Ctrl Pts',(3.42859860294378,-0.666666666666667,
1.51895082866166));
#36889=CARTESIAN_POINT('Ctrl Pts',(3.42859860294378,-1.,1.51895082866166));
#36890=CARTESIAN_POINT('Ctrl Pts',(3.77614523045147,-1.,1.83867539237861));
#36891=CARTESIAN_POINT('Ctrl Pts',(3.77614523045147,1.,1.83867539237861));
#36892=CARTESIAN_POINT('Ctrl Pts',(3.77518714458232,-1.,1.83742834010821));
#36893=CARTESIAN_POINT('Ctrl Pts',(3.77518714458232,1.,1.83742834010821));
#36894=CARTESIAN_POINT('Ctrl Pts',(3.77326886065484,-1.,1.83493697935064));
#36895=CARTESIAN_POINT('Ctrl Pts',(3.77326886065484,1.,1.83493697935064));
#36896=CARTESIAN_POINT('Ctrl Pts',(3.77038509819777,-1.,1.83120816956515));
#36897=CARTESIAN_POINT('Ctrl Pts',(3.77038509819777,1.,1.83120816956515));
#36898=CARTESIAN_POINT('Ctrl Pts',(3.76652740355856,-1.,1.82625289221933));
#36899=CARTESIAN_POINT('Ctrl Pts',(3.76652740355856,1.,1.82625289221933));
#36900=CARTESIAN_POINT('Ctrl Pts',(3.76168412709652,-1.,1.82008629694924));
#36901=CARTESIAN_POINT('Ctrl Pts',(3.76168412709652,1.,1.82008629694924));
#36902=CARTESIAN_POINT('Ctrl Pts',(3.75681965683995,-1.,1.81394729834032));
#36903=CARTESIAN_POINT('Ctrl Pts',(3.75681965683995,1.,1.81394729834032));
#36904=CARTESIAN_POINT('Ctrl Pts',(3.75193395888069,-1.,1.80783603939662));
#36905=CARTESIAN_POINT('Ctrl Pts',(3.75193395888069,1.,1.80783603939662));
#36906=CARTESIAN_POINT('Ctrl Pts',(3.74702700874954,-1.,1.80175271485519));
#36907=CARTESIAN_POINT('Ctrl Pts',(3.74702700874954,1.,1.80175271485519));
#36908=CARTESIAN_POINT('Ctrl Pts',(3.74209880351667,-1.,1.79569757859041));
#36909=CARTESIAN_POINT('Ctrl Pts',(3.74209880351667,1.,1.79569757859041));
#36910=CARTESIAN_POINT('Ctrl Pts',(3.73714934729962,-1.,1.78967092823139));
#36911=CARTESIAN_POINT('Ctrl Pts',(3.73714934729962,1.,1.78967092823139));
#36912=CARTESIAN_POINT('Ctrl Pts',(3.73217863095022,-1.,1.78367308442682));
#36913=CARTESIAN_POINT('Ctrl Pts',(3.73217863095022,1.,1.78367308442682));
#36914=CARTESIAN_POINT('Ctrl Pts',(3.72718661205504,-1.,1.77770437039606));
#36915=CARTESIAN_POINT('Ctrl Pts',(3.72718661205504,1.,1.77770437039606));
#36916=CARTESIAN_POINT('Ctrl Pts',(3.72217319911429,-1.,1.77176509401846));
#36917=CARTESIAN_POINT('Ctrl Pts',(3.72217319911429,1.,1.77176509401846));
#36918=CARTESIAN_POINT('Ctrl Pts',(3.71713822377675,-1.,1.76585552124549));
#36919=CARTESIAN_POINT('Ctrl Pts',(3.71713822377675,1.,1.76585552124549));
#36920=CARTESIAN_POINT('Ctrl Pts',(3.71208146346454,-1.,1.75997588499021));
#36921=CARTESIAN_POINT('Ctrl Pts',(3.71208146346454,1.,1.75997588499021));
#36922=CARTESIAN_POINT('Ctrl Pts',(3.70700269736876,-1.,1.75412641804148));
#36923=CARTESIAN_POINT('Ctrl Pts',(3.70700269736876,1.,1.75412641804148));
#36924=CARTESIAN_POINT('Ctrl Pts',(3.70190175673422,-1.,1.74830738046092));
#36925=CARTESIAN_POINT('Ctrl Pts',(3.70190175673422,1.,1.74830738046092));
#36926=CARTESIAN_POINT('Ctrl Pts',(3.6967785691046,-1.,1.74251908492589));
#36927=CARTESIAN_POINT('Ctrl Pts',(3.6967785691046,1.,1.74251908492589));
#36928=CARTESIAN_POINT('Ctrl Pts',(3.69163322647906,-1.,1.73676193254493));
#36929=CARTESIAN_POINT('Ctrl Pts',(3.69163322647906,1.,1.73676193254493));
#36930=CARTESIAN_POINT('Ctrl Pts',(3.68646597019188,-1.,1.73103640956647));
#36931=CARTESIAN_POINT('Ctrl Pts',(3.68646597019188,1.,1.73103640956647));
#36932=CARTESIAN_POINT('Ctrl Pts',(3.68127704936472,-1.,1.72534302437003));
#36933=CARTESIAN_POINT('Ctrl Pts',(3.68127704936472,1.,1.72534302437003));
#36934=CARTESIAN_POINT('Ctrl Pts',(3.67606660374665,-1.,1.71968225581787));
#36935=CARTESIAN_POINT('Ctrl Pts',(3.67606660374665,1.,1.71968225581787));
#36936=CARTESIAN_POINT('Ctrl Pts',(3.67083454901629,-1.,1.71405450210392));
#36937=CARTESIAN_POINT('Ctrl Pts',(3.67083454901629,1.,1.71405450210392));
#36938=CARTESIAN_POINT('Ctrl Pts',(3.6655804319893,-1.,1.70846001610983));
#36939=CARTESIAN_POINT('Ctrl Pts',(3.6655804319893,1.,1.70846001610983));
#36940=CARTESIAN_POINT('Ctrl Pts',(3.6603033877491,-1.,1.70289888566904));
#36941=CARTESIAN_POINT('Ctrl Pts',(3.6603033877491,1.,1.70289888566904));
#36942=CARTESIAN_POINT('Ctrl Pts',(3.65500246526798,-1.,1.69737117722559));
#36943=CARTESIAN_POINT('Ctrl Pts',(3.65500246526798,1.,1.69737117722559));
#36944=CARTESIAN_POINT('Ctrl Pts',(3.64967689827393,-1.,1.691877054817));
#36945=CARTESIAN_POINT('Ctrl Pts',(3.64967689827393,1.,1.691877054817));
#36946=CARTESIAN_POINT('Ctrl Pts',(3.64432638915199,-1.,1.68641690471455));
#36947=CARTESIAN_POINT('Ctrl Pts',(3.64432638915199,1.,1.68641690471455));
#36948=CARTESIAN_POINT('Ctrl Pts',(3.63895140887443,-1.,1.68099146651577));
#36949=CARTESIAN_POINT('Ctrl Pts',(3.63895140887443,1.,1.68099146651577));
#36950=CARTESIAN_POINT('Ctrl Pts',(3.63355343201211,-1.,1.67560193613145));
#36951=CARTESIAN_POINT('Ctrl Pts',(3.63355343201211,1.,1.67560193613145));
#36952=CARTESIAN_POINT('Ctrl Pts',(3.62813422105257,-1.,1.67024966008037));
#36953=CARTESIAN_POINT('Ctrl Pts',(3.62813422105257,1.,1.67024966008037));
#36954=CARTESIAN_POINT('Ctrl Pts',(3.62269517989104,-1.,1.66493585923853));
#36955=CARTESIAN_POINT('Ctrl Pts',(3.62269517989104,1.,1.66493585923853));
#36956=CARTESIAN_POINT('Ctrl Pts',(3.61723666482457,-1.,1.65966133399186));
#36957=CARTESIAN_POINT('Ctrl Pts',(3.61723666482457,1.,1.65966133399186));
#36958=CARTESIAN_POINT('Ctrl Pts',(3.61175734965129,-1.,1.65442619244327));
#36959=CARTESIAN_POINT('Ctrl Pts',(3.61175734965129,1.,1.65442619244327));
#36960=CARTESIAN_POINT('Ctrl Pts',(3.60625346556992,-1.,1.64922952425833));
#36961=CARTESIAN_POINT('Ctrl Pts',(3.60625346556992,1.,1.64922952425833));
#36962=CARTESIAN_POINT('Ctrl Pts',(3.6007202851384,-1.,1.6440700438558));
#36963=CARTESIAN_POINT('Ctrl Pts',(3.6007202851384,1.,1.6440700438558));
#36964=CARTESIAN_POINT('Ctrl Pts',(3.59515368334887,-1.,1.63894676675349));
#36965=CARTESIAN_POINT('Ctrl Pts',(3.59515368334887,1.,1.63894676675349));
#36966=CARTESIAN_POINT('Ctrl Pts',(3.58955176627876,-1.,1.63385971451259));
#36967=CARTESIAN_POINT('Ctrl Pts',(3.58955176627876,1.,1.63385971451259));
#36968=CARTESIAN_POINT('Ctrl Pts',(3.5839162577435,-1.,1.62881051550748));
#36969=CARTESIAN_POINT('Ctrl Pts',(3.5839162577435,1.,1.62881051550748));
#36970=CARTESIAN_POINT('Ctrl Pts',(3.57825455954405,-1.,1.62380329464851));
#36971=CARTESIAN_POINT('Ctrl Pts',(3.57825455954405,1.,1.62380329464851));
#36972=CARTESIAN_POINT('Ctrl Pts',(3.57257679609826,-1.,1.61884340915412));
#36973=CARTESIAN_POINT('Ctrl Pts',(3.57257679609826,1.,1.61884340915412));
#36974=CARTESIAN_POINT('Ctrl Pts',(3.56689200468404,-1.,1.61393581747522));
#36975=CARTESIAN_POINT('Ctrl Pts',(3.56689200468404,1.,1.61393581747522));
#36976=CARTESIAN_POINT('Ctrl Pts',(3.56120432482986,-1.,1.60908344685459));
#36977=CARTESIAN_POINT('Ctrl Pts',(3.56120432482986,1.,1.60908344685459));
#36978=CARTESIAN_POINT('Ctrl Pts',(3.55550985096117,-1.,1.60428584699848));
#36979=CARTESIAN_POINT('Ctrl Pts',(3.55550985096117,1.,1.60428584699848));
#36980=CARTESIAN_POINT('Ctrl Pts',(3.54979148634426,-1.,1.59953698113444));
#36981=CARTESIAN_POINT('Ctrl Pts',(3.54979148634426,1.,1.59953698113444));
#36982=CARTESIAN_POINT('Ctrl Pts',(3.544024581823,-1.,1.5948276694975));
#36983=CARTESIAN_POINT('Ctrl Pts',(3.544024581823,1.,1.5948276694975));
#36984=CARTESIAN_POINT('Ctrl Pts',(3.53818616861045,-1.,1.59014958368725));
#36985=CARTESIAN_POINT('Ctrl Pts',(3.53818616861045,1.,1.59014958368725));
#36986=CARTESIAN_POINT('Ctrl Pts',(3.53226378147068,-1.,1.58549906268083));
#36987=CARTESIAN_POINT('Ctrl Pts',(3.53226378147068,1.,1.58549906268083));
#36988=CARTESIAN_POINT('Ctrl Pts',(3.52626275334899,-1.,1.58088027227856));
#36989=CARTESIAN_POINT('Ctrl Pts',(3.52626275334899,1.,1.58088027227856));
#36990=CARTESIAN_POINT('Ctrl Pts',(3.52021847865961,-1.,1.5763104998818));
#36991=CARTESIAN_POINT('Ctrl Pts',(3.52021847865961,1.,1.5763104998818));
#36992=CARTESIAN_POINT('Ctrl Pts',(3.51418598431733,-1.,1.57181569799774));
#36993=CARTESIAN_POINT('Ctrl Pts',(3.51418598431733,1.,1.57181569799774));
#36994=CARTESIAN_POINT('Ctrl Pts',(3.50821771695427,-1.,1.56742097575041));
#36995=CARTESIAN_POINT('Ctrl Pts',(3.50821771695427,1.,1.56742097575041));
#36996=CARTESIAN_POINT('Ctrl Pts',(3.50234321621607,-1.,1.56314187758689));
#36997=CARTESIAN_POINT('Ctrl Pts',(3.50234321621607,1.,1.56314187758689));
#36998=CARTESIAN_POINT('Ctrl Pts',(3.49655185179623,-1.,1.55897703097859));
#36999=CARTESIAN_POINT('Ctrl Pts',(3.49655185179623,1.,1.55897703097859));
#37000=CARTESIAN_POINT('Ctrl Pts',(3.49076460877317,-1.,1.5548959590107));
#37001=CARTESIAN_POINT('Ctrl Pts',(3.49076460877317,1.,1.5548959590107));
#37002=CARTESIAN_POINT('Ctrl Pts',(3.48485155928414,-1.,1.55084702970382));
#37003=CARTESIAN_POINT('Ctrl Pts',(3.48485155928414,1.,1.55084702970382));
#37004=CARTESIAN_POINT('Ctrl Pts',(3.47868272898599,-1.,1.54678009290207));
#37005=CARTESIAN_POINT('Ctrl Pts',(3.47868272898599,1.,1.54678009290207));
#37006=CARTESIAN_POINT('Ctrl Pts',(3.47217189224576,-1.,1.54266605398152));
#37007=CARTESIAN_POINT('Ctrl Pts',(3.47217189224576,1.,1.54266605398152));
#37008=CARTESIAN_POINT('Ctrl Pts',(3.46531752207222,-1.,1.53851507915533));
#37009=CARTESIAN_POINT('Ctrl Pts',(3.46531752207222,1.,1.53851507915533));
#37010=CARTESIAN_POINT('Ctrl Pts',(3.45825932955273,-1.,1.53440195378902));
#37011=CARTESIAN_POINT('Ctrl Pts',(3.45825932955273,1.,1.53440195378902));
#37012=CARTESIAN_POINT('Ctrl Pts',(3.45127136828667,-1.,1.530462444618));
#37013=CARTESIAN_POINT('Ctrl Pts',(3.45127136828667,1.,1.530462444618));
#37014=CARTESIAN_POINT('Ctrl Pts',(3.44469547527,-1.,1.52686242875717));
#37015=CARTESIAN_POINT('Ctrl Pts',(3.44469547527,1.,1.52686242875717));
#37016=CARTESIAN_POINT('Ctrl Pts',(3.43888895974182,-1.,1.52377348950429));
#37017=CARTESIAN_POINT('Ctrl Pts',(3.43888895974182,1.,1.52377348950429));
#37018=CARTESIAN_POINT('Ctrl Pts',(3.43417156977749,-1.,1.52134826724227));
#37019=CARTESIAN_POINT('Ctrl Pts',(3.43417156977749,1.,1.52134826724227));
#37020=CARTESIAN_POINT('Ctrl Pts',(3.43076036253384,-1.,1.51969006980792));
#37021=CARTESIAN_POINT('Ctrl Pts',(3.43076036253384,1.,1.51969006980792));
#37022=CARTESIAN_POINT('Ctrl Pts',(3.42915787669388,-1.,1.51901585838879));
#37023=CARTESIAN_POINT('Ctrl Pts',(3.42915787669388,1.,1.51901585838879));
#37024=CARTESIAN_POINT('Ctrl Pts',(3.42860527148835,-1.,1.51888450659497));
#37025=CARTESIAN_POINT('Ctrl Pts',(3.42860527148835,1.,1.51888450659497));
#37026=CARTESIAN_POINT('Ctrl Pts',(3.42852521763648,-1.,1.51896318668306));
#37027=CARTESIAN_POINT('Ctrl Pts',(3.42852521763648,1.,1.51896318668306));
#37028=CARTESIAN_POINT('Ctrl Pts',(3.42855728381368,-1.,1.519044091397));
#37029=CARTESIAN_POINT('Ctrl Pts',(3.42855728381368,1.,1.519044091397));
#37030=CARTESIAN_POINT('',(3.77614523045147,1.,1.83867539237861));
#37031=CARTESIAN_POINT('Ctrl Pts',(3.77614523045147,1.,1.83867539237861));
#37032=CARTESIAN_POINT('Ctrl Pts',(3.77518714458232,1.,1.83742834010821));
#37033=CARTESIAN_POINT('Ctrl Pts',(3.77326886065484,1.,1.83493697935064));
#37034=CARTESIAN_POINT('Ctrl Pts',(3.77038509819777,1.,1.83120816956515));
#37035=CARTESIAN_POINT('Ctrl Pts',(3.76652740355856,1.,1.82625289221933));
#37036=CARTESIAN_POINT('Ctrl Pts',(3.76168412709652,1.,1.82008629694924));
#37037=CARTESIAN_POINT('Ctrl Pts',(3.75681965683995,1.,1.81394729834032));
#37038=CARTESIAN_POINT('Ctrl Pts',(3.75193395888069,1.,1.80783603939662));
#37039=CARTESIAN_POINT('Ctrl Pts',(3.74702700874954,1.,1.80175271485519));
#37040=CARTESIAN_POINT('Ctrl Pts',(3.74209880351667,1.,1.79569757859041));
#37041=CARTESIAN_POINT('Ctrl Pts',(3.73714934729962,1.,1.78967092823139));
#37042=CARTESIAN_POINT('Ctrl Pts',(3.73217863095022,1.,1.78367308442682));
#37043=CARTESIAN_POINT('Ctrl Pts',(3.72718661205504,1.,1.77770437039606));
#37044=CARTESIAN_POINT('Ctrl Pts',(3.72217319911429,1.,1.77176509401846));
#37045=CARTESIAN_POINT('Ctrl Pts',(3.71713822377675,1.,1.76585552124549));
#37046=CARTESIAN_POINT('Ctrl Pts',(3.71208146346454,1.,1.75997588499021));
#37047=CARTESIAN_POINT('Ctrl Pts',(3.70700269736876,1.,1.75412641804148));
#37048=CARTESIAN_POINT('Ctrl Pts',(3.70190175673422,1.,1.74830738046092));
#37049=CARTESIAN_POINT('Ctrl Pts',(3.6967785691046,1.,1.74251908492589));
#37050=CARTESIAN_POINT('Ctrl Pts',(3.69163322647906,1.,1.73676193254493));
#37051=CARTESIAN_POINT('Ctrl Pts',(3.68646597019188,1.,1.73103640956647));
#37052=CARTESIAN_POINT('Ctrl Pts',(3.68127704936472,1.,1.72534302437003));
#37053=CARTESIAN_POINT('Ctrl Pts',(3.67606660374665,1.,1.71968225581787));
#37054=CARTESIAN_POINT('Ctrl Pts',(3.67083454901629,1.,1.71405450210392));
#37055=CARTESIAN_POINT('Ctrl Pts',(3.6655804319893,1.,1.70846001610983));
#37056=CARTESIAN_POINT('Ctrl Pts',(3.6603033877491,1.,1.70289888566904));
#37057=CARTESIAN_POINT('Ctrl Pts',(3.65500246526798,1.,1.69737117722559));
#37058=CARTESIAN_POINT('Ctrl Pts',(3.64967689827393,1.,1.691877054817));
#37059=CARTESIAN_POINT('Ctrl Pts',(3.64432638915199,1.,1.68641690471455));
#37060=CARTESIAN_POINT('Ctrl Pts',(3.63895140887443,1.,1.68099146651577));
#37061=CARTESIAN_POINT('Ctrl Pts',(3.63355343201211,1.,1.67560193613145));
#37062=CARTESIAN_POINT('Ctrl Pts',(3.62813422105257,1.,1.67024966008037));
#37063=CARTESIAN_POINT('Ctrl Pts',(3.62269517989104,1.,1.66493585923853));
#37064=CARTESIAN_POINT('Ctrl Pts',(3.61723666482457,1.,1.65966133399186));
#37065=CARTESIAN_POINT('Ctrl Pts',(3.61175734965129,1.,1.65442619244327));
#37066=CARTESIAN_POINT('Ctrl Pts',(3.60625346556992,1.,1.64922952425833));
#37067=CARTESIAN_POINT('Ctrl Pts',(3.6007202851384,1.,1.6440700438558));
#37068=CARTESIAN_POINT('Ctrl Pts',(3.59515368334887,1.,1.63894676675349));
#37069=CARTESIAN_POINT('Ctrl Pts',(3.58955176627876,1.,1.63385971451259));
#37070=CARTESIAN_POINT('Ctrl Pts',(3.5839162577435,1.,1.62881051550748));
#37071=CARTESIAN_POINT('Ctrl Pts',(3.57825455954405,1.,1.62380329464851));
#37072=CARTESIAN_POINT('Ctrl Pts',(3.57257679609826,1.,1.61884340915412));
#37073=CARTESIAN_POINT('Ctrl Pts',(3.56689200468404,1.,1.61393581747522));
#37074=CARTESIAN_POINT('Ctrl Pts',(3.56120432482986,1.,1.60908344685459));
#37075=CARTESIAN_POINT('Ctrl Pts',(3.55550985096117,1.,1.60428584699848));
#37076=CARTESIAN_POINT('Ctrl Pts',(3.54979148634426,1.,1.59953698113444));
#37077=CARTESIAN_POINT('Ctrl Pts',(3.544024581823,1.,1.5948276694975));
#37078=CARTESIAN_POINT('Ctrl Pts',(3.53818616861045,1.,1.59014958368725));
#37079=CARTESIAN_POINT('Ctrl Pts',(3.53226378147068,1.,1.58549906268083));
#37080=CARTESIAN_POINT('Ctrl Pts',(3.52626275334899,1.,1.58088027227856));
#37081=CARTESIAN_POINT('Ctrl Pts',(3.52021847865961,1.,1.5763104998818));
#37082=CARTESIAN_POINT('Ctrl Pts',(3.51418598431733,1.,1.57181569799774));
#37083=CARTESIAN_POINT('Ctrl Pts',(3.50821771695427,1.,1.56742097575041));
#37084=CARTESIAN_POINT('Ctrl Pts',(3.50234321621607,1.,1.56314187758689));
#37085=CARTESIAN_POINT('Ctrl Pts',(3.49655185179623,1.,1.55897703097859));
#37086=CARTESIAN_POINT('Ctrl Pts',(3.49076460877317,1.,1.5548959590107));
#37087=CARTESIAN_POINT('Ctrl Pts',(3.48485155928414,1.,1.55084702970382));
#37088=CARTESIAN_POINT('Ctrl Pts',(3.47868272898599,1.,1.54678009290207));
#37089=CARTESIAN_POINT('Ctrl Pts',(3.47217189224576,1.,1.54266605398152));
#37090=CARTESIAN_POINT('Ctrl Pts',(3.46531752207222,1.,1.53851507915533));
#37091=CARTESIAN_POINT('Ctrl Pts',(3.45825932955273,1.,1.53440195378902));
#37092=CARTESIAN_POINT('Ctrl Pts',(3.45127136828667,1.,1.530462444618));
#37093=CARTESIAN_POINT('Ctrl Pts',(3.44469547527,1.,1.52686242875717));
#37094=CARTESIAN_POINT('Ctrl Pts',(3.43888895974182,1.,1.52377348950429));
#37095=CARTESIAN_POINT('Ctrl Pts',(3.43417156977749,1.,1.52134826724227));
#37096=CARTESIAN_POINT('Ctrl Pts',(3.4310163189349,1.,1.5198144909343));
#37097=CARTESIAN_POINT('Ctrl Pts',(3.42946838852728,1.,1.51914806898539));
#37098=CARTESIAN_POINT('Ctrl Pts',(3.42884302333978,1.,1.51895133295017));
#37099=CARTESIAN_POINT('Ctrl Pts',(3.42864616361967,1.,1.51893924967231));
#37100=CARTESIAN_POINT('Ctrl Pts',(3.42859860294378,1.,1.51895082866166));
#37101=CARTESIAN_POINT('',(3.77614523045147,0.,1.83867539237861));
#37102=CARTESIAN_POINT('Ctrl Pts',(3.24418789321065,-1.,1.88088939428811));
#37103=CARTESIAN_POINT('Ctrl Pts',(3.24418789321065,1.,1.88088939428811));
#37104=CARTESIAN_POINT('Ctrl Pts',(3.24410359189733,-1.,1.8809110068042));
#37105=CARTESIAN_POINT('Ctrl Pts',(3.24410359189733,1.,1.8809110068042));
#37106=CARTESIAN_POINT('Ctrl Pts',(3.24408699284449,-1.,1.8810220187274));
#37107=CARTESIAN_POINT('Ctrl Pts',(3.24408699284449,1.,1.8810220187274));
#37108=CARTESIAN_POINT('Ctrl Pts',(3.24451807186964,-1.,1.88139187908347));
#37109=CARTESIAN_POINT('Ctrl Pts',(3.24451807186964,1.,1.88139187908347));
#37110=CARTESIAN_POINT('Ctrl Pts',(3.24600543790876,-1.,1.88229202583187));
#37111=CARTESIAN_POINT('Ctrl Pts',(3.24600543790876,1.,1.88229202583187));
#37112=CARTESIAN_POINT('Ctrl Pts',(3.24935200512055,-1.,1.88407708646435));
#37113=CARTESIAN_POINT('Ctrl Pts',(3.24935200512055,1.,1.88407708646435));
#37114=CARTESIAN_POINT('Ctrl Pts',(3.25408686339298,-1.,1.88646802523372));
#37115=CARTESIAN_POINT('Ctrl Pts',(3.25408686339298,1.,1.88646802523372));
#37116=CARTESIAN_POINT('Ctrl Pts',(3.2599988519361,-1.,1.88934996203508));
#37117=CARTESIAN_POINT('Ctrl Pts',(3.2599988519361,1.,1.88934996203508));
#37118=CARTESIAN_POINT('Ctrl Pts',(3.2667765388833,-1.,1.89255393500769));
#37119=CARTESIAN_POINT('Ctrl Pts',(3.2667765388833,1.,1.89255393500769));
#37120=CARTESIAN_POINT('Ctrl Pts',(3.27407108932908,-1.,1.89589172903662));
#37121=CARTESIAN_POINT('Ctrl Pts',(3.27407108932908,1.,1.89589172903662));
#37122=CARTESIAN_POINT('Ctrl Pts',(3.28154737912287,-1.,1.89918429230425));
#37123=CARTESIAN_POINT('Ctrl Pts',(3.28154737912287,1.,1.89918429230425));
#37124=CARTESIAN_POINT('Ctrl Pts',(3.28893448600364,-1.,1.9022897124757));
#37125=CARTESIAN_POINT('Ctrl Pts',(3.28893448600364,1.,1.9022897124757));
#37126=CARTESIAN_POINT('Ctrl Pts',(3.29608978722258,-1.,1.9051389186417));
#37127=CARTESIAN_POINT('Ctrl Pts',(3.29608978722258,1.,1.9051389186417));
#37128=CARTESIAN_POINT('Ctrl Pts',(3.30300595568341,-1.,1.90773912171424));
#37129=CARTESIAN_POINT('Ctrl Pts',(3.30300595568341,1.,1.90773912171424));
#37130=CARTESIAN_POINT('Ctrl Pts',(3.30975721158694,-1.,1.91014297830502));
#37131=CARTESIAN_POINT('Ctrl Pts',(3.30975721158694,1.,1.91014297830502));
#37132=CARTESIAN_POINT('Ctrl Pts',(3.31646052426395,-1.,1.91242616234459));
#37133=CARTESIAN_POINT('Ctrl Pts',(3.31646052426395,1.,1.91242616234459));
#37134=CARTESIAN_POINT('Ctrl Pts',(3.32323403454507,-1.,1.91466343916612));
#37135=CARTESIAN_POINT('Ctrl Pts',(3.32323403454507,1.,1.91466343916612));
#37136=CARTESIAN_POINT('Ctrl Pts',(3.33014884257812,-1.,1.91690081930297));
#37137=CARTESIAN_POINT('Ctrl Pts',(3.33014884257812,1.,1.91690081930297));
#37138=CARTESIAN_POINT('Ctrl Pts',(3.33721230709948,-1.,1.91914609610173));
#37139=CARTESIAN_POINT('Ctrl Pts',(3.33721230709948,1.,1.91914609610173));
#37140=CARTESIAN_POINT('Ctrl Pts',(3.34439448941915,-1.,1.92138450828378));
#37141=CARTESIAN_POINT('Ctrl Pts',(3.34439448941915,1.,1.92138450828378));
#37142=CARTESIAN_POINT('Ctrl Pts',(3.35164424847206,-1.,1.92358838440518));
#37143=CARTESIAN_POINT('Ctrl Pts',(3.35164424847206,1.,1.92358838440518));
#37144=CARTESIAN_POINT('Ctrl Pts',(3.35890824422976,-1.,1.92572846125763));
#37145=CARTESIAN_POINT('Ctrl Pts',(3.35890824422976,1.,1.92572846125763));
#37146=CARTESIAN_POINT('Ctrl Pts',(3.36615168657597,-1.,1.92778626543803));
#37147=CARTESIAN_POINT('Ctrl Pts',(3.36615168657597,1.,1.92778626543803));
#37148=CARTESIAN_POINT('Ctrl Pts',(3.37336807068078,-1.,1.92975993109897));
#37149=CARTESIAN_POINT('Ctrl Pts',(3.37336807068078,1.,1.92975993109897));
#37150=CARTESIAN_POINT('Ctrl Pts',(3.38056768525577,-1.,1.93165739093292));
#37151=CARTESIAN_POINT('Ctrl Pts',(3.38056768525577,1.,1.93165739093292));
#37152=CARTESIAN_POINT('Ctrl Pts',(3.38777076883267,-1.,1.93349233176794));
#37153=CARTESIAN_POINT('Ctrl Pts',(3.38777076883267,1.,1.93349233176794));
#37154=CARTESIAN_POINT('Ctrl Pts',(3.39499923640789,-1.,1.93527929945982));
#37155=CARTESIAN_POINT('Ctrl Pts',(3.39499923640789,1.,1.93527929945982));
#37156=CARTESIAN_POINT('Ctrl Pts',(3.40226802104093,-1.,1.93702857723089));
#37157=CARTESIAN_POINT('Ctrl Pts',(3.40226802104093,1.,1.93702857723089));
#37158=CARTESIAN_POINT('Ctrl Pts',(3.40957978266622,-1.,1.93874306008132));
#37159=CARTESIAN_POINT('Ctrl Pts',(3.40957978266622,1.,1.93874306008132));
#37160=CARTESIAN_POINT('Ctrl Pts',(3.41692971994082,-1.,1.94042111965237));
#37161=CARTESIAN_POINT('Ctrl Pts',(3.41692971994082,1.,1.94042111965237));
#37162=CARTESIAN_POINT('Ctrl Pts',(3.42430850941497,-1.,1.94205835913692));
#37163=CARTESIAN_POINT('Ctrl Pts',(3.42430850941497,1.,1.94205835913692));
#37164=CARTESIAN_POINT('Ctrl Pts',(3.43170586602436,-1.,1.94364973660285));
#37165=CARTESIAN_POINT('Ctrl Pts',(3.43170586602436,1.,1.94364973660285));
#37166=CARTESIAN_POINT('Ctrl Pts',(3.43911410197693,-1.,1.94519168842883));
#37167=CARTESIAN_POINT('Ctrl Pts',(3.43911410197693,1.,1.94519168842883));
#37168=CARTESIAN_POINT('Ctrl Pts',(3.44653088665685,-1.,1.94668377715332));
#37169=CARTESIAN_POINT('Ctrl Pts',(3.44653088665685,1.,1.94668377715332));
#37170=CARTESIAN_POINT('Ctrl Pts',(3.45395731584051,-1.,1.94812754766524));
#37171=CARTESIAN_POINT('Ctrl Pts',(3.45395731584051,1.,1.94812754766524));
#37172=CARTESIAN_POINT('Ctrl Pts',(3.46139661060959,-1.,1.94952575850196));
#37173=CARTESIAN_POINT('Ctrl Pts',(3.46139661060959,1.,1.94952575850196));
#37174=CARTESIAN_POINT('Ctrl Pts',(3.4688525897419,-1.,1.95088147859876));
#37175=CARTESIAN_POINT('Ctrl Pts',(3.4688525897419,1.,1.95088147859876));
#37176=CARTESIAN_POINT('Ctrl Pts',(3.47632820495926,-1.,1.95219722189878));
#37177=CARTESIAN_POINT('Ctrl Pts',(3.47632820495926,1.,1.95219722189878));
#37178=CARTESIAN_POINT('Ctrl Pts',(3.48382414832648,-1.,1.95347412486316));
#37179=CARTESIAN_POINT('Ctrl Pts',(3.48382414832648,1.,1.95347412486316));
#37180=CARTESIAN_POINT('Ctrl Pts',(3.49133956289154,-1.,1.95471236969653));
#37181=CARTESIAN_POINT('Ctrl Pts',(3.49133956289154,1.,1.95471236969653));
#37182=CARTESIAN_POINT('Ctrl Pts',(3.49887263575602,-1.,1.9559115382367));
#37183=CARTESIAN_POINT('Ctrl Pts',(3.49887263575602,1.,1.9559115382367));
#37184=CARTESIAN_POINT('Ctrl Pts',(3.50642124159913,-1.,1.95707099606514));
#37185=CARTESIAN_POINT('Ctrl Pts',(3.50642124159913,1.,1.95707099606514));
#37186=CARTESIAN_POINT('Ctrl Pts',(3.51398354617772,-1.,1.95819025316768));
#37187=CARTESIAN_POINT('Ctrl Pts',(3.51398354617772,1.,1.95819025316768));
#37188=CARTESIAN_POINT('Ctrl Pts',(3.52155867431438,-1.,1.95926936324436));
#37189=CARTESIAN_POINT('Ctrl Pts',(3.52155867431438,1.,1.95926936324436));
#37190=CARTESIAN_POINT('Ctrl Pts',(3.52914648844289,-1.,1.96030879411534));
#37191=CARTESIAN_POINT('Ctrl Pts',(3.52914648844289,1.,1.96030879411534));
#37192=CARTESIAN_POINT('Ctrl Pts',(3.53674730625759,-1.,1.96130926212661));
#37193=CARTESIAN_POINT('Ctrl Pts',(3.53674730625759,1.,1.96130926212661));
#37194=CARTESIAN_POINT('Ctrl Pts',(3.54436163300425,-1.,1.96227157573058));
#37195=CARTESIAN_POINT('Ctrl Pts',(3.54436163300425,1.,1.96227157573058));
#37196=CARTESIAN_POINT('Ctrl Pts',(3.55198990600929,-1.,1.96319648628667));
#37197=CARTESIAN_POINT('Ctrl Pts',(3.55198990600929,1.,1.96319648628667));
#37198=CARTESIAN_POINT('Ctrl Pts',(3.55963218706201,-1.,1.96408450906868));
#37199=CARTESIAN_POINT('Ctrl Pts',(3.55963218706201,1.,1.96408450906868));
#37200=CARTESIAN_POINT('Ctrl Pts',(3.56728820357933,-1.,1.96493594634643));
#37201=CARTESIAN_POINT('Ctrl Pts',(3.56728820357933,1.,1.96493594634643));
#37202=CARTESIAN_POINT('Ctrl Pts',(3.57495748601088,-1.,1.96575096652857));
#37203=CARTESIAN_POINT('Ctrl Pts',(3.57495748601088,1.,1.96575096652857));
#37204=CARTESIAN_POINT('Ctrl Pts',(3.58263947663884,-1.,1.9665296668894));
#37205=CARTESIAN_POINT('Ctrl Pts',(3.58263947663884,1.,1.9665296668894));
#37206=CARTESIAN_POINT('Ctrl Pts',(3.5903336402273,-1.,1.96727213799507));
#37207=CARTESIAN_POINT('Ctrl Pts',(3.5903336402273,1.,1.96727213799507));
#37208=CARTESIAN_POINT('Ctrl Pts',(3.59803959819725,-1.,1.96797854118257));
#37209=CARTESIAN_POINT('Ctrl Pts',(3.59803959819725,1.,1.96797854118257));
#37210=CARTESIAN_POINT('Ctrl Pts',(3.60575714017676,-1.,1.96864911885775));
#37211=CARTESIAN_POINT('Ctrl Pts',(3.60575714017676,1.,1.96864911885775));
#37212=CARTESIAN_POINT('Ctrl Pts',(3.61348615496393,-1.,1.96928416040712));
#37213=CARTESIAN_POINT('Ctrl Pts',(3.61348615496393,1.,1.96928416040712));
#37214=CARTESIAN_POINT('Ctrl Pts',(3.62122658401722,-1.,1.96988398129888));
#37215=CARTESIAN_POINT('Ctrl Pts',(3.62122658401722,1.,1.96988398129888));
#37216=CARTESIAN_POINT('Ctrl Pts',(3.62897836973397,-1.,1.97044889850518));
#37217=CARTESIAN_POINT('Ctrl Pts',(3.62897836973397,1.,1.97044889850518));
#37218=CARTESIAN_POINT('Ctrl Pts',(3.63674139590853,-1.,1.97097920454698));
#37219=CARTESIAN_POINT('Ctrl Pts',(3.63674139590853,1.,1.97097920454698));
#37220=CARTESIAN_POINT('Ctrl Pts',(3.64451546724221,-1.,1.97147515441539));
#37221=CARTESIAN_POINT('Ctrl Pts',(3.64451546724221,1.,1.97147515441539));
#37222=CARTESIAN_POINT('Ctrl Pts',(3.65230034717364,-1.,1.97193697240645));
#37223=CARTESIAN_POINT('Ctrl Pts',(3.65230034717364,1.,1.97193697240645));
#37224=CARTESIAN_POINT('Ctrl Pts',(3.66009578166865,-1.,1.97236485439317));
#37225=CARTESIAN_POINT('Ctrl Pts',(3.66009578166865,1.,1.97236485439317));
#37226=CARTESIAN_POINT('Ctrl Pts',(3.66790152751984,-1.,1.9727589719863));
#37227=CARTESIAN_POINT('Ctrl Pts',(3.66790152751984,1.,1.9727589719863));
#37228=CARTESIAN_POINT('Ctrl Pts',(3.67571738106175,-1.,1.97311947678035));
#37229=CARTESIAN_POINT('Ctrl Pts',(3.67571738106175,1.,1.97311947678035));
#37230=CARTESIAN_POINT('Ctrl Pts',(3.68354319913416,-1.,1.97344650303631));
#37231=CARTESIAN_POINT('Ctrl Pts',(3.68354319913416,1.,1.97344650303631));
#37232=CARTESIAN_POINT('Ctrl Pts',(3.69137888597855,-1.,1.97374016224397));
#37233=CARTESIAN_POINT('Ctrl Pts',(3.69137888597855,1.,1.97374016224397));
#37234=CARTESIAN_POINT('Ctrl Pts',(3.69765528558292,-1.,1.97394846382289));
#37235=CARTESIAN_POINT('Ctrl Pts',(3.69765528558292,1.,1.97394846382289));
#37236=CARTESIAN_POINT('Ctrl Pts',(3.70236698911837,-1.,1.97408973726149));
#37237=CARTESIAN_POINT('Ctrl Pts',(3.70236698911837,1.,1.97408973726149));
#37238=CARTESIAN_POINT('Ctrl Pts',(3.7055100813194,-1.,1.974177276451));
#37239=CARTESIAN_POINT('Ctrl Pts',(3.7055100813194,1.,1.974177276451));
#37240=CARTESIAN_POINT('Ctrl Pts',(3.70708211654725,-1.,1.97421938526992));
#37241=CARTESIAN_POINT('Ctrl Pts',(3.70708211654725,1.,1.97421938526992));
#37242=CARTESIAN_POINT('',(3.24413672884902,1.,1.88097764062542));
#37243=CARTESIAN_POINT('Ctrl Pts',(3.24413672884902,-1.,1.88097764062542));
#37244=CARTESIAN_POINT('Ctrl Pts',(3.24413672884902,-0.666666666666667,
1.88097764062542));
#37245=CARTESIAN_POINT('Ctrl Pts',(3.24413672884902,-0.333333333333333,
1.88097764062542));
#37246=CARTESIAN_POINT('Ctrl Pts',(3.24413672884902,0.333333333333333,1.88097764062542));
#37247=CARTESIAN_POINT('Ctrl Pts',(3.24413672884902,0.666666666666667,1.88097764062541));
#37248=CARTESIAN_POINT('Ctrl Pts',(3.24413672884902,1.,1.88097764062541));
#37249=CARTESIAN_POINT('',(3.70708211654725,1.,1.97421938526992));
#37250=CARTESIAN_POINT('',(3.70708211654725,0.,1.97421938526992));
#37251=CARTESIAN_POINT('Ctrl Pts',(3.24413672884902,1.,1.88097764062542));
#37252=CARTESIAN_POINT('Ctrl Pts',(3.24415531671311,1.,1.88102292397987));
#37253=CARTESIAN_POINT('Ctrl Pts',(3.24428080352952,1.,1.88117508446657));
#37254=CARTESIAN_POINT('Ctrl Pts',(3.24480754675942,1.,1.88156537699118));
#37255=CARTESIAN_POINT('Ctrl Pts',(3.24625654410705,1.,1.88242596600422));
#37256=CARTESIAN_POINT('Ctrl Pts',(3.24935200512055,1.,1.88407708646435));
#37257=CARTESIAN_POINT('Ctrl Pts',(3.25408686339298,1.,1.88646802523372));
#37258=CARTESIAN_POINT('Ctrl Pts',(3.2599988519361,1.,1.88934996203508));
#37259=CARTESIAN_POINT('Ctrl Pts',(3.2667765388833,1.,1.89255393500769));
#37260=CARTESIAN_POINT('Ctrl Pts',(3.27407108932908,1.,1.89589172903662));
#37261=CARTESIAN_POINT('Ctrl Pts',(3.28154737912287,1.,1.89918429230425));
#37262=CARTESIAN_POINT('Ctrl Pts',(3.28893448600364,1.,1.9022897124757));
#37263=CARTESIAN_POINT('Ctrl Pts',(3.29608978722258,1.,1.9051389186417));
#37264=CARTESIAN_POINT('Ctrl Pts',(3.30300595568341,1.,1.90773912171424));
#37265=CARTESIAN_POINT('Ctrl Pts',(3.30975721158694,1.,1.91014297830502));
#37266=CARTESIAN_POINT('Ctrl Pts',(3.31646052426395,1.,1.91242616234459));
#37267=CARTESIAN_POINT('Ctrl Pts',(3.32323403454507,1.,1.91466343916612));
#37268=CARTESIAN_POINT('Ctrl Pts',(3.33014884257812,1.,1.91690081930297));
#37269=CARTESIAN_POINT('Ctrl Pts',(3.33721230709948,1.,1.91914609610173));
#37270=CARTESIAN_POINT('Ctrl Pts',(3.34439448941915,1.,1.92138450828378));
#37271=CARTESIAN_POINT('Ctrl Pts',(3.35164424847206,1.,1.92358838440518));
#37272=CARTESIAN_POINT('Ctrl Pts',(3.35890824422976,1.,1.92572846125763));
#37273=CARTESIAN_POINT('Ctrl Pts',(3.36615168657597,1.,1.92778626543803));
#37274=CARTESIAN_POINT('Ctrl Pts',(3.37336807068078,1.,1.92975993109897));
#37275=CARTESIAN_POINT('Ctrl Pts',(3.38056768525577,1.,1.93165739093292));
#37276=CARTESIAN_POINT('Ctrl Pts',(3.38777076883267,1.,1.93349233176794));
#37277=CARTESIAN_POINT('Ctrl Pts',(3.39499923640789,1.,1.93527929945982));
#37278=CARTESIAN_POINT('Ctrl Pts',(3.40226802104093,1.,1.93702857723089));
#37279=CARTESIAN_POINT('Ctrl Pts',(3.40957978266622,1.,1.93874306008132));
#37280=CARTESIAN_POINT('Ctrl Pts',(3.41692971994082,1.,1.94042111965237));
#37281=CARTESIAN_POINT('Ctrl Pts',(3.42430850941497,1.,1.94205835913692));
#37282=CARTESIAN_POINT('Ctrl Pts',(3.43170586602436,1.,1.94364973660285));
#37283=CARTESIAN_POINT('Ctrl Pts',(3.43911410197693,1.,1.94519168842883));
#37284=CARTESIAN_POINT('Ctrl Pts',(3.44653088665685,1.,1.94668377715332));
#37285=CARTESIAN_POINT('Ctrl Pts',(3.45395731584051,1.,1.94812754766524));
#37286=CARTESIAN_POINT('Ctrl Pts',(3.46139661060959,1.,1.94952575850196));
#37287=CARTESIAN_POINT('Ctrl Pts',(3.4688525897419,1.,1.95088147859876));
#37288=CARTESIAN_POINT('Ctrl Pts',(3.47632820495926,1.,1.95219722189878));
#37289=CARTESIAN_POINT('Ctrl Pts',(3.48382414832648,1.,1.95347412486316));
#37290=CARTESIAN_POINT('Ctrl Pts',(3.49133956289154,1.,1.95471236969653));
#37291=CARTESIAN_POINT('Ctrl Pts',(3.49887263575602,1.,1.9559115382367));
#37292=CARTESIAN_POINT('Ctrl Pts',(3.50642124159913,1.,1.95707099606514));
#37293=CARTESIAN_POINT('Ctrl Pts',(3.51398354617772,1.,1.95819025316768));
#37294=CARTESIAN_POINT('Ctrl Pts',(3.52155867431438,1.,1.95926936324436));
#37295=CARTESIAN_POINT('Ctrl Pts',(3.52914648844289,1.,1.96030879411534));
#37296=CARTESIAN_POINT('Ctrl Pts',(3.53674730625759,1.,1.96130926212661));
#37297=CARTESIAN_POINT('Ctrl Pts',(3.54436163300425,1.,1.96227157573058));
#37298=CARTESIAN_POINT('Ctrl Pts',(3.55198990600929,1.,1.96319648628667));
#37299=CARTESIAN_POINT('Ctrl Pts',(3.55963218706201,1.,1.96408450906868));
#37300=CARTESIAN_POINT('Ctrl Pts',(3.56728820357933,1.,1.96493594634643));
#37301=CARTESIAN_POINT('Ctrl Pts',(3.57495748601088,1.,1.96575096652857));
#37302=CARTESIAN_POINT('Ctrl Pts',(3.58263947663884,1.,1.9665296668894));
#37303=CARTESIAN_POINT('Ctrl Pts',(3.5903336402273,1.,1.96727213799507));
#37304=CARTESIAN_POINT('Ctrl Pts',(3.59803959819725,1.,1.96797854118257));
#37305=CARTESIAN_POINT('Ctrl Pts',(3.60575714017676,1.,1.96864911885775));
#37306=CARTESIAN_POINT('Ctrl Pts',(3.61348615496393,1.,1.96928416040712));
#37307=CARTESIAN_POINT('Ctrl Pts',(3.62122658401722,1.,1.96988398129888));
#37308=CARTESIAN_POINT('Ctrl Pts',(3.62897836973397,1.,1.97044889850518));
#37309=CARTESIAN_POINT('Ctrl Pts',(3.63674139590853,1.,1.97097920454698));
#37310=CARTESIAN_POINT('Ctrl Pts',(3.64451546724221,1.,1.97147515441539));
#37311=CARTESIAN_POINT('Ctrl Pts',(3.65230034717364,1.,1.97193697240645));
#37312=CARTESIAN_POINT('Ctrl Pts',(3.66009578166865,1.,1.97236485439317));
#37313=CARTESIAN_POINT('Ctrl Pts',(3.66790152751984,1.,1.9727589719863));
#37314=CARTESIAN_POINT('Ctrl Pts',(3.67571738106175,1.,1.97311947678035));
#37315=CARTESIAN_POINT('Ctrl Pts',(3.68354319913416,1.,1.97344650303631));
#37316=CARTESIAN_POINT('Ctrl Pts',(3.69137888597855,1.,1.97374016224397));
#37317=CARTESIAN_POINT('Ctrl Pts',(3.69765528558292,1.,1.97394846382289));
#37318=CARTESIAN_POINT('Ctrl Pts',(3.70236698911837,1.,1.97408973726149));
#37319=CARTESIAN_POINT('Ctrl Pts',(3.7055100813194,1.,1.974177276451));
#37320=CARTESIAN_POINT('Ctrl Pts',(3.70708211654725,1.,1.97421938526992));
#37321=CARTESIAN_POINT('Origin',(3.70708211654725,0.,1.97421938526992));
#37322=CARTESIAN_POINT('',(3.77614523045147,1.,1.83867539237861));
#37323=CARTESIAN_POINT('Origin',(0.,0.,0.));
#37324=CARTESIAN_POINT('',(3.14877060440425,1.,2.03660101169564));
#37325=CARTESIAN_POINT('Origin',(0.,1.,0.));
#37326=CARTESIAN_POINT('Ctrl Pts',(3.14877060440425,1.,2.03660101169564));
#37327=CARTESIAN_POINT('Ctrl Pts',(3.14877060440425,0.666666666666667,2.03660101169564));
#37328=CARTESIAN_POINT('Ctrl Pts',(3.14877060440425,0.333333333333333,2.03660101169564));
#37329=CARTESIAN_POINT('Ctrl Pts',(3.14877060440425,-0.333333333333333,
2.03660101169564));
#37330=CARTESIAN_POINT('Ctrl Pts',(3.14877060440425,-0.666666666666667,
2.03660101169564));
#37331=CARTESIAN_POINT('Ctrl Pts',(3.14877060440425,-1.,2.03660101169564));
#37332=CARTESIAN_POINT('Ctrl Pts',(3.44202241512147,-1.,2.40675750623143));
#37333=CARTESIAN_POINT('Ctrl Pts',(3.44202241512147,1.,2.40675750623143));
#37334=CARTESIAN_POINT('Ctrl Pts',(3.44127120683402,-1.,2.40537592959345));
#37335=CARTESIAN_POINT('Ctrl Pts',(3.44127120683402,1.,2.40537592959345));
#37336=CARTESIAN_POINT('Ctrl Pts',(3.43976627485223,-1.,2.40261515590099));
#37337=CARTESIAN_POINT('Ctrl Pts',(3.43976627485223,1.,2.40261515590099));
#37338=CARTESIAN_POINT('Ctrl Pts',(3.43750133066036,-1.,2.39848113411429));
#37339=CARTESIAN_POINT('Ctrl Pts',(3.43750133066036,1.,2.39848113411429));
#37340=CARTESIAN_POINT('Ctrl Pts',(3.43446630680436,-1.,2.39298338805823));
#37341=CARTESIAN_POINT('Ctrl Pts',(3.43446630680436,1.,2.39298338805823));
#37342=CARTESIAN_POINT('Ctrl Pts',(3.43064732714472,-1.,2.38613505844641));
#37343=CARTESIAN_POINT('Ctrl Pts',(3.43064732714472,1.,2.38613505844641));
#37344=CARTESIAN_POINT('Ctrl Pts',(3.42680309755241,-1.,2.37931067029517));
#37345=CARTESIAN_POINT('Ctrl Pts',(3.42680309755241,1.,2.37931067029517));
#37346=CARTESIAN_POINT('Ctrl Pts',(3.42293356216595,-1.,2.37251035954351));
#37347=CARTESIAN_POINT('Ctrl Pts',(3.42293356216595,1.,2.37251035954351));
#37348=CARTESIAN_POINT('Ctrl Pts',(3.41903866635384,-1.,2.36573431470314));
#37349=CARTESIAN_POINT('Ctrl Pts',(3.41903866635384,1.,2.36573431470314));
#37350=CARTESIAN_POINT('Ctrl Pts',(3.4151183675076,-1.,2.35898278606449));
#37351=CARTESIAN_POINT('Ctrl Pts',(3.4151183675076,1.,2.35898278606449));
#37352=CARTESIAN_POINT('Ctrl Pts',(3.41117262313464,-1.,2.35225606823649));
#37353=CARTESIAN_POINT('Ctrl Pts',(3.41117262313464,1.,2.35225606823649));
#37354=CARTESIAN_POINT('Ctrl Pts',(3.40720137403888,-1.,2.34555447648901));
#37355=CARTESIAN_POINT('Ctrl Pts',(3.40720137403888,1.,2.34555447648901));
#37356=CARTESIAN_POINT('Ctrl Pts',(3.40320452776646,-1.,2.33887832342715));
#37357=CARTESIAN_POINT('Ctrl Pts',(3.40320452776646,1.,2.33887832342715));
#37358=CARTESIAN_POINT('Ctrl Pts',(3.39918194578115,-1.,2.33222789882601));
#37359=CARTESIAN_POINT('Ctrl Pts',(3.39918194578115,1.,2.33222789882601));
#37360=CARTESIAN_POINT('Ctrl Pts',(3.39513342020045,-1.,2.32560343902683));
#37361=CARTESIAN_POINT('Ctrl Pts',(3.39513342020045,1.,2.32560343902683));
#37362=CARTESIAN_POINT('Ctrl Pts',(3.39105869475112,-1.,2.31900513925627));
#37363=CARTESIAN_POINT('Ctrl Pts',(3.39105869475112,1.,2.31900513925627));
#37364=CARTESIAN_POINT('Ctrl Pts',(3.38695751492659,-1.,2.31243319489505));
#37365=CARTESIAN_POINT('Ctrl Pts',(3.38695751492659,1.,2.31243319489505));
#37366=CARTESIAN_POINT('Ctrl Pts',(3.38282967336676,-1.,2.30588783640389));
#37367=CARTESIAN_POINT('Ctrl Pts',(3.38282967336676,1.,2.30588783640389));
#37368=CARTESIAN_POINT('Ctrl Pts',(3.37867504959382,-1.,2.29936936127588));
#37369=CARTESIAN_POINT('Ctrl Pts',(3.37867504959382,1.,2.29936936127588));
#37370=CARTESIAN_POINT('Ctrl Pts',(3.37449367172707,-1.,2.2928781800731));
#37371=CARTESIAN_POINT('Ctrl Pts',(3.37449367172707,1.,2.2928781800731));
#37372=CARTESIAN_POINT('Ctrl Pts',(3.37028570206357,-1.,2.28641481081045));
#37373=CARTESIAN_POINT('Ctrl Pts',(3.37028570206357,1.,2.28641481081045));
#37374=CARTESIAN_POINT('Ctrl Pts',(3.36605130712978,-1.,2.27997979457968));
#37375=CARTESIAN_POINT('Ctrl Pts',(3.36605130712978,1.,2.27997979457968));
#37376=CARTESIAN_POINT('Ctrl Pts',(3.36179055004369,-1.,2.27357362620902));
#37377=CARTESIAN_POINT('Ctrl Pts',(3.36179055004369,1.,2.27357362620902));
#37378=CARTESIAN_POINT('Ctrl Pts',(3.35750328523077,-1.,2.26719668579921));
#37379=CARTESIAN_POINT('Ctrl Pts',(3.35750328523077,1.,2.26719668579921));
#37380=CARTESIAN_POINT('Ctrl Pts',(3.35318902552676,-1.,2.26084915222484));
#37381=CARTESIAN_POINT('Ctrl Pts',(3.35318902552676,1.,2.26084915222484));
#37382=CARTESIAN_POINT('Ctrl Pts',(3.34884690292342,-1.,2.25453097693524));
#37383=CARTESIAN_POINT('Ctrl Pts',(3.34884690292342,1.,2.25453097693524));
#37384=CARTESIAN_POINT('Ctrl Pts',(3.34447596770768,-1.,2.24824207678288));
#37385=CARTESIAN_POINT('Ctrl Pts',(3.34447596770768,1.,2.24824207678288));
#37386=CARTESIAN_POINT('Ctrl Pts',(3.34007543738044,-1.,2.24198249391437));
#37387=CARTESIAN_POINT('Ctrl Pts',(3.34007543738044,1.,2.24198249391437));
#37388=CARTESIAN_POINT('Ctrl Pts',(3.33564495756478,-1.,2.2357525632881));
#37389=CARTESIAN_POINT('Ctrl Pts',(3.33564495756478,1.,2.2357525632881));
#37390=CARTESIAN_POINT('Ctrl Pts',(3.33118487773593,-1.,2.22955308907221));
#37391=CARTESIAN_POINT('Ctrl Pts',(3.33118487773593,1.,2.22955308907221));
#37392=CARTESIAN_POINT('Ctrl Pts',(3.32669646722871,-1.,2.22338548312759));
#37393=CARTESIAN_POINT('Ctrl Pts',(3.32669646722871,1.,2.22338548312759));
#37394=CARTESIAN_POINT('Ctrl Pts',(3.32218125618955,-1.,2.21725135110889));
#37395=CARTESIAN_POINT('Ctrl Pts',(3.32218125618955,1.,2.21725135110889));
#37396=CARTESIAN_POINT('Ctrl Pts',(3.31764044024231,-1.,2.21115211847872));
#37397=CARTESIAN_POINT('Ctrl Pts',(3.31764044024231,1.,2.21115211847872));
#37398=CARTESIAN_POINT('Ctrl Pts',(3.3130742460895,-1.,2.20508863150608));
#37399=CARTESIAN_POINT('Ctrl Pts',(3.3130742460895,1.,2.20508863150608));
#37400=CARTESIAN_POINT('Ctrl Pts',(3.30848134694596,-1.,2.19906078949925));
#37401=CARTESIAN_POINT('Ctrl Pts',(3.30848134694596,1.,2.19906078949925));
#37402=CARTESIAN_POINT('Ctrl Pts',(3.30385816281831,-1.,2.19306710376112));
#37403=CARTESIAN_POINT('Ctrl Pts',(3.30385816281831,1.,2.19306710376112));
#37404=CARTESIAN_POINT('Ctrl Pts',(3.29920022557635,-1.,2.18710556500325));
#37405=CARTESIAN_POINT('Ctrl Pts',(3.29920022557635,1.,2.18710556500325));
#37406=CARTESIAN_POINT('Ctrl Pts',(3.29450361500484,-1.,2.18117455557062));
#37407=CARTESIAN_POINT('Ctrl Pts',(3.29450361500484,1.,2.18117455557062));
#37408=CARTESIAN_POINT('Ctrl Pts',(3.28976645712566,-1.,2.17527380048422));
#37409=CARTESIAN_POINT('Ctrl Pts',(3.28976645712566,1.,2.17527380048422));
#37410=CARTESIAN_POINT('Ctrl Pts',(3.2849901997973,-1.,2.16940517773459));
#37411=CARTESIAN_POINT('Ctrl Pts',(3.2849901997973,1.,2.16940517773459));
#37412=CARTESIAN_POINT('Ctrl Pts',(3.28018150841414,-1.,2.16357391934434));
#37413=CARTESIAN_POINT('Ctrl Pts',(3.28018150841414,1.,2.16357391934434));
#37414=CARTESIAN_POINT('Ctrl Pts',(3.27534954469206,-1.,2.15778690038359));
#37415=CARTESIAN_POINT('Ctrl Pts',(3.27534954469206,1.,2.15778690038359));
#37416=CARTESIAN_POINT('Ctrl Pts',(3.27050245897244,-1.,2.15205043199818));
#37417=CARTESIAN_POINT('Ctrl Pts',(3.27050245897244,1.,2.15205043199818));
#37418=CARTESIAN_POINT('Ctrl Pts',(3.26564388189764,-1.,2.14636805295663));
#37419=CARTESIAN_POINT('Ctrl Pts',(3.26564388189764,1.,2.14636805295663));
#37420=CARTESIAN_POINT('Ctrl Pts',(3.26077002641868,-1.,2.14073870754258));
#37421=CARTESIAN_POINT('Ctrl Pts',(3.26077002641868,1.,2.14073870754258));
#37422=CARTESIAN_POINT('Ctrl Pts',(3.25586495065027,-1.,2.13515375878786));
#37423=CARTESIAN_POINT('Ctrl Pts',(3.25586495065027,1.,2.13515375878786));
#37424=CARTESIAN_POINT('Ctrl Pts',(3.25090574493994,-1.,2.1296002839681));
#37425=CARTESIAN_POINT('Ctrl Pts',(3.25090574493994,1.,2.1296002839681));
#37426=CARTESIAN_POINT('Ctrl Pts',(3.24587102613347,-1.,2.12406646410943));
#37427=CARTESIAN_POINT('Ctrl Pts',(3.24587102613347,1.,2.12406646410943));
#37428=CARTESIAN_POINT('Ctrl Pts',(3.24074905517282,-1.,2.11854673326972));
#37429=CARTESIAN_POINT('Ctrl Pts',(3.24074905517282,1.,2.11854673326972));
#37430=CARTESIAN_POINT('Ctrl Pts',(3.23554444767115,-1.,2.11304604021784));
#37431=CARTESIAN_POINT('Ctrl Pts',(3.23554444767115,1.,2.11304604021784));
#37432=CARTESIAN_POINT('Ctrl Pts',(3.23028945793334,-1.,2.1075869964248));
#37433=CARTESIAN_POINT('Ctrl Pts',(3.23028945793334,1.,2.1075869964248));
#37434=CARTESIAN_POINT('Ctrl Pts',(3.22503437553496,-1.,2.10220384298534));
#37435=CARTESIAN_POINT('Ctrl Pts',(3.22503437553496,1.,2.10220384298534));
#37436=CARTESIAN_POINT('Ctrl Pts',(3.21982707347067,-1.,2.09692958434933));
#37437=CARTESIAN_POINT('Ctrl Pts',(3.21982707347067,1.,2.09692958434933));
#37438=CARTESIAN_POINT('Ctrl Pts',(3.2146942960168,-1.,2.0917841946046));
#37439=CARTESIAN_POINT('Ctrl Pts',(3.2146942960168,1.,2.0917841946046));
#37440=CARTESIAN_POINT('Ctrl Pts',(3.20962575845433,-1.,2.08676465517435));
#37441=CARTESIAN_POINT('Ctrl Pts',(3.20962575845433,1.,2.08676465517435));
#37442=CARTESIAN_POINT('Ctrl Pts',(3.20454818630635,-1.,2.08182850370816));
#37443=CARTESIAN_POINT('Ctrl Pts',(3.20454818630635,1.,2.08182850370816));
#37444=CARTESIAN_POINT('Ctrl Pts',(3.19934132835879,-1.,2.0769044187063));
#37445=CARTESIAN_POINT('Ctrl Pts',(3.19934132835879,1.,2.0769044187063));
#37446=CARTESIAN_POINT('Ctrl Pts',(3.19388465568113,-1.,2.07192253497765));
#37447=CARTESIAN_POINT('Ctrl Pts',(3.19388465568113,1.,2.07192253497765));
#37448=CARTESIAN_POINT('Ctrl Pts',(3.18809755562297,-1.,2.06684062744065));
#37449=CARTESIAN_POINT('Ctrl Pts',(3.18809755562297,1.,2.06684062744065));
#37450=CARTESIAN_POINT('Ctrl Pts',(3.18197692964677,-1.,2.06166849827143));
#37451=CARTESIAN_POINT('Ctrl Pts',(3.18197692964677,1.,2.06166849827143));
#37452=CARTESIAN_POINT('Ctrl Pts',(3.17564906975592,-1.,2.05650186773279));
#37453=CARTESIAN_POINT('Ctrl Pts',(3.17564906975592,1.,2.05650186773279));
#37454=CARTESIAN_POINT('Ctrl Pts',(3.16936341689859,-1.,2.05151770247452));
#37455=CARTESIAN_POINT('Ctrl Pts',(3.16936341689859,1.,2.05151770247452));
#37456=CARTESIAN_POINT('Ctrl Pts',(3.16343165059235,-1.,2.0469333124766));
#37457=CARTESIAN_POINT('Ctrl Pts',(3.16343165059235,1.,2.0469333124766));
#37458=CARTESIAN_POINT('Ctrl Pts',(3.15817983946525,-1.,2.04297406404132));
#37459=CARTESIAN_POINT('Ctrl Pts',(3.15817983946525,1.,2.04297406404132));
#37460=CARTESIAN_POINT('Ctrl Pts',(3.1538999167466,-1.,2.03984073791432));
#37461=CARTESIAN_POINT('Ctrl Pts',(3.1538999167466,1.,2.03984073791432));
#37462=CARTESIAN_POINT('Ctrl Pts',(3.15079010635326,-1.,2.03766932526171));
#37463=CARTESIAN_POINT('Ctrl Pts',(3.15079010635326,1.,2.03766932526171));
#37464=CARTESIAN_POINT('Ctrl Pts',(3.14931281967585,-1.,2.03675273048882));
#37465=CARTESIAN_POINT('Ctrl Pts',(3.14931281967585,1.,2.03675273048882));
#37466=CARTESIAN_POINT('Ctrl Pts',(3.14878756590499,-1.,2.03653654935384));
#37467=CARTESIAN_POINT('Ctrl Pts',(3.14878756590499,1.,2.03653654935384));
#37468=CARTESIAN_POINT('Ctrl Pts',(3.14869618937138,-1.,2.036601737578));
#37469=CARTESIAN_POINT('Ctrl Pts',(3.14869618937138,1.,2.036601737578));
#37470=CARTESIAN_POINT('Ctrl Pts',(3.1487152044751,-1.,2.03668666247593));
#37471=CARTESIAN_POINT('Ctrl Pts',(3.1487152044751,1.,2.03668666247593));
#37472=CARTESIAN_POINT('',(3.44202241512147,1.,2.40675750623143));
#37473=CARTESIAN_POINT('Ctrl Pts',(3.44202241512147,1.,2.40675750623143));
#37474=CARTESIAN_POINT('Ctrl Pts',(3.44127120683402,1.,2.40537592959345));
#37475=CARTESIAN_POINT('Ctrl Pts',(3.43976627485223,1.,2.40261515590099));
#37476=CARTESIAN_POINT('Ctrl Pts',(3.43750133066036,1.,2.39848113411429));
#37477=CARTESIAN_POINT('Ctrl Pts',(3.43446630680436,1.,2.39298338805823));
#37478=CARTESIAN_POINT('Ctrl Pts',(3.43064732714472,1.,2.38613505844641));
#37479=CARTESIAN_POINT('Ctrl Pts',(3.42680309755241,1.,2.37931067029517));
#37480=CARTESIAN_POINT('Ctrl Pts',(3.42293356216595,1.,2.37251035954351));
#37481=CARTESIAN_POINT('Ctrl Pts',(3.41903866635384,1.,2.36573431470314));
#37482=CARTESIAN_POINT('Ctrl Pts',(3.4151183675076,1.,2.35898278606449));
#37483=CARTESIAN_POINT('Ctrl Pts',(3.41117262313464,1.,2.35225606823649));
#37484=CARTESIAN_POINT('Ctrl Pts',(3.40720137403888,1.,2.34555447648901));
#37485=CARTESIAN_POINT('Ctrl Pts',(3.40320452776646,1.,2.33887832342715));
#37486=CARTESIAN_POINT('Ctrl Pts',(3.39918194578115,1.,2.33222789882601));
#37487=CARTESIAN_POINT('Ctrl Pts',(3.39513342020045,1.,2.32560343902683));
#37488=CARTESIAN_POINT('Ctrl Pts',(3.39105869475112,1.,2.31900513925627));
#37489=CARTESIAN_POINT('Ctrl Pts',(3.38695751492659,1.,2.31243319489505));
#37490=CARTESIAN_POINT('Ctrl Pts',(3.38282967336676,1.,2.30588783640389));
#37491=CARTESIAN_POINT('Ctrl Pts',(3.37867504959382,1.,2.29936936127588));
#37492=CARTESIAN_POINT('Ctrl Pts',(3.37449367172707,1.,2.2928781800731));
#37493=CARTESIAN_POINT('Ctrl Pts',(3.37028570206357,1.,2.28641481081045));
#37494=CARTESIAN_POINT('Ctrl Pts',(3.36605130712978,1.,2.27997979457968));
#37495=CARTESIAN_POINT('Ctrl Pts',(3.36179055004369,1.,2.27357362620902));
#37496=CARTESIAN_POINT('Ctrl Pts',(3.35750328523077,1.,2.26719668579921));
#37497=CARTESIAN_POINT('Ctrl Pts',(3.35318902552676,1.,2.26084915222484));
#37498=CARTESIAN_POINT('Ctrl Pts',(3.34884690292342,1.,2.25453097693524));
#37499=CARTESIAN_POINT('Ctrl Pts',(3.34447596770768,1.,2.24824207678288));
#37500=CARTESIAN_POINT('Ctrl Pts',(3.34007543738044,1.,2.24198249391437));
#37501=CARTESIAN_POINT('Ctrl Pts',(3.33564495756478,1.,2.2357525632881));
#37502=CARTESIAN_POINT('Ctrl Pts',(3.33118487773593,1.,2.22955308907221));
#37503=CARTESIAN_POINT('Ctrl Pts',(3.32669646722871,1.,2.22338548312759));
#37504=CARTESIAN_POINT('Ctrl Pts',(3.32218125618955,1.,2.21725135110889));
#37505=CARTESIAN_POINT('Ctrl Pts',(3.31764044024231,1.,2.21115211847872));
#37506=CARTESIAN_POINT('Ctrl Pts',(3.3130742460895,1.,2.20508863150608));
#37507=CARTESIAN_POINT('Ctrl Pts',(3.30848134694596,1.,2.19906078949925));
#37508=CARTESIAN_POINT('Ctrl Pts',(3.30385816281831,1.,2.19306710376112));
#37509=CARTESIAN_POINT('Ctrl Pts',(3.29920022557635,1.,2.18710556500325));
#37510=CARTESIAN_POINT('Ctrl Pts',(3.29450361500484,1.,2.18117455557062));
#37511=CARTESIAN_POINT('Ctrl Pts',(3.28976645712566,1.,2.17527380048422));
#37512=CARTESIAN_POINT('Ctrl Pts',(3.2849901997973,1.,2.16940517773459));
#37513=CARTESIAN_POINT('Ctrl Pts',(3.28018150841414,1.,2.16357391934434));
#37514=CARTESIAN_POINT('Ctrl Pts',(3.27534954469206,1.,2.15778690038359));
#37515=CARTESIAN_POINT('Ctrl Pts',(3.27050245897244,1.,2.15205043199818));
#37516=CARTESIAN_POINT('Ctrl Pts',(3.26564388189764,1.,2.14636805295663));
#37517=CARTESIAN_POINT('Ctrl Pts',(3.26077002641868,1.,2.14073870754258));
#37518=CARTESIAN_POINT('Ctrl Pts',(3.25586495065027,1.,2.13515375878786));
#37519=CARTESIAN_POINT('Ctrl Pts',(3.25090574493994,1.,2.1296002839681));
#37520=CARTESIAN_POINT('Ctrl Pts',(3.24587102613347,1.,2.12406646410943));
#37521=CARTESIAN_POINT('Ctrl Pts',(3.24074905517282,1.,2.11854673326972));
#37522=CARTESIAN_POINT('Ctrl Pts',(3.23554444767115,1.,2.11304604021784));
#37523=CARTESIAN_POINT('Ctrl Pts',(3.23028945793334,1.,2.1075869964248));
#37524=CARTESIAN_POINT('Ctrl Pts',(3.22503437553496,1.,2.10220384298534));
#37525=CARTESIAN_POINT('Ctrl Pts',(3.21982707347067,1.,2.09692958434933));
#37526=CARTESIAN_POINT('Ctrl Pts',(3.2146942960168,1.,2.0917841946046));
#37527=CARTESIAN_POINT('Ctrl Pts',(3.20962575845433,1.,2.08676465517435));
#37528=CARTESIAN_POINT('Ctrl Pts',(3.20454818630635,1.,2.08182850370816));
#37529=CARTESIAN_POINT('Ctrl Pts',(3.19934132835879,1.,2.0769044187063));
#37530=CARTESIAN_POINT('Ctrl Pts',(3.19388465568113,1.,2.07192253497765));
#37531=CARTESIAN_POINT('Ctrl Pts',(3.18809755562297,1.,2.06684062744065));
#37532=CARTESIAN_POINT('Ctrl Pts',(3.18197692964677,1.,2.06166849827143));
#37533=CARTESIAN_POINT('Ctrl Pts',(3.17564906975592,1.,2.05650186773279));
#37534=CARTESIAN_POINT('Ctrl Pts',(3.16936341689859,1.,2.05151770247452));
#37535=CARTESIAN_POINT('Ctrl Pts',(3.16343165059235,1.,2.0469333124766));
#37536=CARTESIAN_POINT('Ctrl Pts',(3.15817983946525,1.,2.04297406404132));
#37537=CARTESIAN_POINT('Ctrl Pts',(3.1538999167466,1.,2.03984073791432));
#37538=CARTESIAN_POINT('Ctrl Pts',(3.15102344775396,1.,2.03783225496023));
#37539=CARTESIAN_POINT('Ctrl Pts',(3.14959882629936,1.,2.03693188810614));
#37540=CARTESIAN_POINT('Ctrl Pts',(3.14901193669147,1.,2.03663974554941));
#37541=CARTESIAN_POINT('Ctrl Pts',(3.1488193908823,1.,2.03659701539175));
#37542=CARTESIAN_POINT('Ctrl Pts',(3.14877060440425,1.,2.03660101169564));
#37543=CARTESIAN_POINT('',(3.44202241512147,0.,2.40675750623143));
#37544=CARTESIAN_POINT('Ctrl Pts',(2.91001063062876,-1.,2.36523532225181));
#37545=CARTESIAN_POINT('Ctrl Pts',(2.91001063062876,1.,2.36523532225181));
#37546=CARTESIAN_POINT('Ctrl Pts',(2.90992398626211,-1.,2.36524348105112));
#37547=CARTESIAN_POINT('Ctrl Pts',(2.90992398626211,1.,2.36524348105112));
#37548=CARTESIAN_POINT('Ctrl Pts',(2.90989022548032,-1.,2.36535052956938));
#37549=CARTESIAN_POINT('Ctrl Pts',(2.90989022548032,1.,2.36535052956938));
#37550=CARTESIAN_POINT('Ctrl Pts',(2.91025813830041,-1.,2.36578327194741));
#37551=CARTESIAN_POINT('Ctrl Pts',(2.91025813830041,1.,2.36578327194741));
#37552=CARTESIAN_POINT('Ctrl Pts',(2.9115863784204,-1.,2.36690501170627));
#37553=CARTESIAN_POINT('Ctrl Pts',(2.9115863784204,1.,2.36690501170627));
#37554=CARTESIAN_POINT('Ctrl Pts',(2.9146124988314,-1.,2.36919161373173));
#37555=CARTESIAN_POINT('Ctrl Pts',(2.9146124988314,1.,2.36919161373173));
#37556=CARTESIAN_POINT('Ctrl Pts',(2.91891503791411,-1.,2.37229381109821));
#37557=CARTESIAN_POINT('Ctrl Pts',(2.91891503791411,1.,2.37229381109821));
#37558=CARTESIAN_POINT('Ctrl Pts',(2.92430340582608,-1.,2.3760651052403));
#37559=CARTESIAN_POINT('Ctrl Pts',(2.92430340582608,1.,2.3760651052403));
#37560=CARTESIAN_POINT('Ctrl Pts',(2.93049643640206,-1.,2.38028989582073));
#37561=CARTESIAN_POINT('Ctrl Pts',(2.93049643640206,1.,2.38028989582073));
#37562=CARTESIAN_POINT('Ctrl Pts',(2.93717903280391,-1.,2.38472771516311));
#37563=CARTESIAN_POINT('Ctrl Pts',(2.93717903280391,1.,2.38472771516311));
#37564=CARTESIAN_POINT('Ctrl Pts',(2.94404820669076,-1.,2.38914929090759));
#37565=CARTESIAN_POINT('Ctrl Pts',(2.94404820669076,1.,2.38914929090759));
#37566=CARTESIAN_POINT('Ctrl Pts',(2.95085857128439,-1.,2.39337207631667));
#37567=CARTESIAN_POINT('Ctrl Pts',(2.95085857128439,1.,2.39337207631667));
#37568=CARTESIAN_POINT('Ctrl Pts',(2.95748006482942,-1.,2.39730553974517));
#37569=CARTESIAN_POINT('Ctrl Pts',(2.95748006482942,1.,2.39730553974517));
#37570=CARTESIAN_POINT('Ctrl Pts',(2.96390432240312,-1.,2.4009556571164));
#37571=CARTESIAN_POINT('Ctrl Pts',(2.96390432240312,1.,2.4009556571164));
#37572=CARTESIAN_POINT('Ctrl Pts',(2.9701964131236,-1.,2.40438604734919));
#37573=CARTESIAN_POINT('Ctrl Pts',(2.9701964131236,1.,2.40438604734919));
#37574=CARTESIAN_POINT('Ctrl Pts',(2.97646002822422,-1.,2.40768975073713));
#37575=CARTESIAN_POINT('Ctrl Pts',(2.97646002822422,1.,2.40768975073713));
#37576=CARTESIAN_POINT('Ctrl Pts',(2.98280015815107,-1.,2.41095909342571));
#37577=CARTESIAN_POINT('Ctrl Pts',(2.98280015815107,1.,2.41095909342571));
#37578=CARTESIAN_POINT('Ctrl Pts',(2.98927983005796,-1.,2.41425064199586));
#37579=CARTESIAN_POINT('Ctrl Pts',(2.98927983005796,1.,2.41425064199586));
#37580=CARTESIAN_POINT('Ctrl Pts',(2.99590509293503,-1.,2.41757324500514));
#37581=CARTESIAN_POINT('Ctrl Pts',(2.99590509293503,1.,2.41757324500514));
#37582=CARTESIAN_POINT('Ctrl Pts',(3.00264868585996,-1.,2.42090763946779));
#37583=CARTESIAN_POINT('Ctrl Pts',(3.00264868585996,1.,2.42090763946779));
#37584=CARTESIAN_POINT('Ctrl Pts',(3.00946442616658,-1.,2.42421849439613));
#37585=CARTESIAN_POINT('Ctrl Pts',(3.00946442616658,1.,2.42421849439613));
#37586=CARTESIAN_POINT('Ctrl Pts',(3.01630420830504,-1.,2.42746856264168));
#37587=CARTESIAN_POINT('Ctrl Pts',(3.01630420830504,1.,2.42746856264168));
#37588=CARTESIAN_POINT('Ctrl Pts',(3.02313656036004,-1.,2.43063415586637));
#37589=CARTESIAN_POINT('Ctrl Pts',(3.02313656036004,1.,2.43063415586637));
#37590=CARTESIAN_POINT('Ctrl Pts',(3.02995534946978,-1.,2.43371241361488));
#37591=CARTESIAN_POINT('Ctrl Pts',(3.02995534946978,1.,2.43371241361488));
#37592=CARTESIAN_POINT('Ctrl Pts',(3.03676949672821,-1.,2.43671278042414));
#37593=CARTESIAN_POINT('Ctrl Pts',(3.03676949672821,1.,2.43671278042414));
#37594=CARTESIAN_POINT('Ctrl Pts',(3.04359685040555,-1.,2.43965194061857));
#37595=CARTESIAN_POINT('Ctrl Pts',(3.04359685040555,1.,2.43965194061857));
#37596=CARTESIAN_POINT('Ctrl Pts',(3.05045678021504,-1.,2.44254768923105));
#37597=CARTESIAN_POINT('Ctrl Pts',(3.05045678021504,1.,2.44254768923105));
#37598=CARTESIAN_POINT('Ctrl Pts',(3.05736242671506,-1.,2.44541251892556));
#37599=CARTESIAN_POINT('Ctrl Pts',(3.05736242671506,1.,2.44541251892556));
#37600=CARTESIAN_POINT('Ctrl Pts',(3.06431596421405,-1.,2.44824970516544));
#37601=CARTESIAN_POINT('Ctrl Pts',(3.06431596421405,1.,2.44824970516544));
#37602=CARTESIAN_POINT('Ctrl Pts',(3.07131290521297,-1.,2.45105688854422));
#37603=CARTESIAN_POINT('Ctrl Pts',(3.07131290521297,1.,2.45105688854422));
#37604=CARTESIAN_POINT('Ctrl Pts',(3.07834472886139,-1.,2.4538282678779));
#37605=CARTESIAN_POINT('Ctrl Pts',(3.07834472886139,1.,2.4538282678779));
#37606=CARTESIAN_POINT('Ctrl Pts',(3.08540206545315,-1.,2.45655725437039));
#37607=CARTESIAN_POINT('Ctrl Pts',(3.08540206545315,1.,2.45655725437039));
#37608=CARTESIAN_POINT('Ctrl Pts',(3.09247787931887,-1.,2.4592391256388));
#37609=CARTESIAN_POINT('Ctrl Pts',(3.09247787931887,1.,2.4592391256388));
#37610=CARTESIAN_POINT('Ctrl Pts',(3.09956993697052,-1.,2.46187308501884));
#37611=CARTESIAN_POINT('Ctrl Pts',(3.09956993697052,1.,2.46187308501884));
#37612=CARTESIAN_POINT('Ctrl Pts',(3.1066790790198,-1.,2.46446082979646));
#37613=CARTESIAN_POINT('Ctrl Pts',(3.1066790790198,1.,2.46446082979646));
#37614=CARTESIAN_POINT('Ctrl Pts',(3.11380805536122,-1.,2.46700558843506));
#37615=CARTESIAN_POINT('Ctrl Pts',(3.11380805536122,1.,2.46700558843506));
#37616=CARTESIAN_POINT('Ctrl Pts',(3.12096015766983,-1.,2.46951098947469));
#37617=CARTESIAN_POINT('Ctrl Pts',(3.12096015766983,1.,2.46951098947469));
#37618=CARTESIAN_POINT('Ctrl Pts',(3.12813790805952,-1.,2.47197997765871));
#37619=CARTESIAN_POINT('Ctrl Pts',(3.12813790805952,1.,2.47197997765871));
#37620=CARTESIAN_POINT('Ctrl Pts',(3.13534181229295,-1.,2.47441378371932));
#37621=CARTESIAN_POINT('Ctrl Pts',(3.13534181229295,1.,2.47441378371932));
#37622=CARTESIAN_POINT('Ctrl Pts',(3.1425709954655,-1.,2.47681245356109));
#37623=CARTESIAN_POINT('Ctrl Pts',(3.1425709954655,1.,2.47681245356109));
#37624=CARTESIAN_POINT('Ctrl Pts',(3.14982373241352,-1.,2.47917529057029));
#37625=CARTESIAN_POINT('Ctrl Pts',(3.14982373241352,1.,2.47917529057029));
#37626=CARTESIAN_POINT('Ctrl Pts',(3.15709802322739,-1.,2.48150133566571));
#37627=CARTESIAN_POINT('Ctrl Pts',(3.15709802322739,1.,2.48150133566571));
#37628=CARTESIAN_POINT('Ctrl Pts',(3.16439213290161,-1.,2.48378981792725));
#37629=CARTESIAN_POINT('Ctrl Pts',(3.16439213290161,1.,2.48378981792725));
#37630=CARTESIAN_POINT('Ctrl Pts',(3.17170518863313,-1.,2.48604065348587));
#37631=CARTESIAN_POINT('Ctrl Pts',(3.17170518863313,1.,2.48604065348587));
#37632=CARTESIAN_POINT('Ctrl Pts',(3.17903698136622,-1.,2.48825428288201));
#37633=CARTESIAN_POINT('Ctrl Pts',(3.17903698136622,1.,2.48825428288201));
#37634=CARTESIAN_POINT('Ctrl Pts',(3.18638771282266,-1.,2.49043146334059));
#37635=CARTESIAN_POINT('Ctrl Pts',(3.18638771282266,1.,2.49043146334059));
#37636=CARTESIAN_POINT('Ctrl Pts',(3.19375775555798,-1.,2.49257307239848));
#37637=CARTESIAN_POINT('Ctrl Pts',(3.19375775555798,1.,2.49257307239848));
#37638=CARTESIAN_POINT('Ctrl Pts',(3.20114742397588,-1.,2.49467992057755));
#37639=CARTESIAN_POINT('Ctrl Pts',(3.20114742397588,1.,2.49467992057755));
#37640=CARTESIAN_POINT('Ctrl Pts',(3.20855669849836,-1.,2.4967525264737));
#37641=CARTESIAN_POINT('Ctrl Pts',(3.20855669849836,1.,2.4967525264737));
#37642=CARTESIAN_POINT('Ctrl Pts',(3.21598526261286,-1.,2.4987911459939));
#37643=CARTESIAN_POINT('Ctrl Pts',(3.21598526261286,1.,2.4987911459939));
#37644=CARTESIAN_POINT('Ctrl Pts',(3.22343262620503,-1.,2.50079587201958));
#37645=CARTESIAN_POINT('Ctrl Pts',(3.22343262620503,1.,2.50079587201958));
#37646=CARTESIAN_POINT('Ctrl Pts',(3.23089822320646,-1.,2.50276671338111));
#37647=CARTESIAN_POINT('Ctrl Pts',(3.23089822320646,1.,2.50276671338111));
#37648=CARTESIAN_POINT('Ctrl Pts',(3.23838151080319,-1.,2.5047036758003));
#37649=CARTESIAN_POINT('Ctrl Pts',(3.23838151080319,1.,2.5047036758003));
#37650=CARTESIAN_POINT('Ctrl Pts',(3.24588208983849,-1.,2.506606859405));
#37651=CARTESIAN_POINT('Ctrl Pts',(3.24588208983849,1.,2.506606859405));
#37652=CARTESIAN_POINT('Ctrl Pts',(3.25339971460982,-1.,2.50847647070723));
#37653=CARTESIAN_POINT('Ctrl Pts',(3.25339971460982,1.,2.50847647070723));
#37654=CARTESIAN_POINT('Ctrl Pts',(3.26093423001434,-1.,2.51031277813486));
#37655=CARTESIAN_POINT('Ctrl Pts',(3.26093423001434,1.,2.51031277813486));
#37656=CARTESIAN_POINT('Ctrl Pts',(3.26848552888115,-1.,2.51211608411423));
#37657=CARTESIAN_POINT('Ctrl Pts',(3.26848552888115,1.,2.51211608411423));
#37658=CARTESIAN_POINT('Ctrl Pts',(3.27605350473142,-1.,2.513886692704));
#37659=CARTESIAN_POINT('Ctrl Pts',(3.27605350473142,1.,2.513886692704));
#37660=CARTESIAN_POINT('Ctrl Pts',(3.28363799702982,-1.,2.51562487464514));
#37661=CARTESIAN_POINT('Ctrl Pts',(3.28363799702982,1.,2.51562487464514));
#37662=CARTESIAN_POINT('Ctrl Pts',(3.2912387729927,-1.,2.51733085123797));
#37663=CARTESIAN_POINT('Ctrl Pts',(3.2912387729927,1.,2.51733085123797));
#37664=CARTESIAN_POINT('Ctrl Pts',(3.29885556388352,-1.,2.51900480701069));
#37665=CARTESIAN_POINT('Ctrl Pts',(3.29885556388352,1.,2.51900480701069));
#37666=CARTESIAN_POINT('Ctrl Pts',(3.30648808815442,-1.,2.52064689568511));
#37667=CARTESIAN_POINT('Ctrl Pts',(3.30648808815442,1.,2.52064689568511));
#37668=CARTESIAN_POINT('Ctrl Pts',(3.31413607874645,-1.,2.52225724871313));
#37669=CARTESIAN_POINT('Ctrl Pts',(3.31413607874645,1.,2.52225724871313));
#37670=CARTESIAN_POINT('Ctrl Pts',(3.32179931078699,-1.,2.5238359839626));
#37671=CARTESIAN_POINT('Ctrl Pts',(3.32179931078699,1.,2.5238359839626));
#37672=CARTESIAN_POINT('Ctrl Pts',(3.32947762187533,-1.,2.52538321164634));
#37673=CARTESIAN_POINT('Ctrl Pts',(3.32947762187533,1.,2.52538321164634));
#37674=CARTESIAN_POINT('Ctrl Pts',(3.33717089999103,-1.,2.52689902690158));
#37675=CARTESIAN_POINT('Ctrl Pts',(3.33717089999103,1.,2.52689902690158));
#37676=CARTESIAN_POINT('Ctrl Pts',(3.34333744115511,-1.,2.52808660915689));
#37677=CARTESIAN_POINT('Ctrl Pts',(3.34333744115511,1.,2.52808660915689));
#37678=CARTESIAN_POINT('Ctrl Pts',(3.34796903576663,-1.,2.52896321610703));
#37679=CARTESIAN_POINT('Ctrl Pts',(3.34796903576663,1.,2.52896321610703));
#37680=CARTESIAN_POINT('Ctrl Pts',(3.35105973714071,-1.,2.5295413654909));
#37681=CARTESIAN_POINT('Ctrl Pts',(3.35105973714071,1.,2.5295413654909));
#37682=CARTESIAN_POINT('Ctrl Pts',(3.35260583073571,-1.,2.52982887637028));
#37683=CARTESIAN_POINT('Ctrl Pts',(3.35260583073571,1.,2.52982887637028));
#37684=CARTESIAN_POINT('',(2.90994629141676,1.,2.36531447826073));
#37685=CARTESIAN_POINT('Ctrl Pts',(2.90994629141676,-1.,2.36531447826073));
#37686=CARTESIAN_POINT('Ctrl Pts',(2.90994629141676,-0.666666666666667,
2.36531447826073));
#37687=CARTESIAN_POINT('Ctrl Pts',(2.90994629141676,-0.333333333333333,
2.36531447826073));
#37688=CARTESIAN_POINT('Ctrl Pts',(2.90994629141676,0.333333333333333,2.36531447826073));
#37689=CARTESIAN_POINT('Ctrl Pts',(2.90994629141676,0.666666666666667,2.36531447826073));
#37690=CARTESIAN_POINT('Ctrl Pts',(2.90994629141676,1.,2.36531447826073));
#37691=CARTESIAN_POINT('',(3.35260583073571,1.,2.52982887637028));
#37692=CARTESIAN_POINT('',(3.35260583073571,0.,2.52982887637028));
#37693=CARTESIAN_POINT('Ctrl Pts',(2.90994629141676,1.,2.36531447826073));
#37694=CARTESIAN_POINT('Ctrl Pts',(2.90995756655606,1.,2.36536211188453));
#37695=CARTESIAN_POINT('Ctrl Pts',(2.91005770527719,1.,2.36553202948613));
#37696=CARTESIAN_POINT('Ctrl Pts',(2.91051690822156,1.,2.36599991765749));
#37697=CARTESIAN_POINT('Ctrl Pts',(2.91181344022548,1.,2.36707658451664));
#37698=CARTESIAN_POINT('Ctrl Pts',(2.9146124988314,1.,2.36919161373173));
#37699=CARTESIAN_POINT('Ctrl Pts',(2.91891503791411,1.,2.37229381109821));
#37700=CARTESIAN_POINT('Ctrl Pts',(2.92430340582608,1.,2.3760651052403));
#37701=CARTESIAN_POINT('Ctrl Pts',(2.93049643640206,1.,2.38028989582073));
#37702=CARTESIAN_POINT('Ctrl Pts',(2.93717903280391,1.,2.38472771516311));
#37703=CARTESIAN_POINT('Ctrl Pts',(2.94404820669076,1.,2.38914929090759));
#37704=CARTESIAN_POINT('Ctrl Pts',(2.95085857128439,1.,2.39337207631667));
#37705=CARTESIAN_POINT('Ctrl Pts',(2.95748006482942,1.,2.39730553974517));
#37706=CARTESIAN_POINT('Ctrl Pts',(2.96390432240312,1.,2.4009556571164));
#37707=CARTESIAN_POINT('Ctrl Pts',(2.9701964131236,1.,2.40438604734919));
#37708=CARTESIAN_POINT('Ctrl Pts',(2.97646002822422,1.,2.40768975073713));
#37709=CARTESIAN_POINT('Ctrl Pts',(2.98280015815107,1.,2.41095909342571));
#37710=CARTESIAN_POINT('Ctrl Pts',(2.98927983005796,1.,2.41425064199586));
#37711=CARTESIAN_POINT('Ctrl Pts',(2.99590509293503,1.,2.41757324500514));
#37712=CARTESIAN_POINT('Ctrl Pts',(3.00264868585996,1.,2.42090763946779));
#37713=CARTESIAN_POINT('Ctrl Pts',(3.00946442616658,1.,2.42421849439613));
#37714=CARTESIAN_POINT('Ctrl Pts',(3.01630420830504,1.,2.42746856264168));
#37715=CARTESIAN_POINT('Ctrl Pts',(3.02313656036004,1.,2.43063415586637));
#37716=CARTESIAN_POINT('Ctrl Pts',(3.02995534946978,1.,2.43371241361488));
#37717=CARTESIAN_POINT('Ctrl Pts',(3.03676949672821,1.,2.43671278042414));
#37718=CARTESIAN_POINT('Ctrl Pts',(3.04359685040555,1.,2.43965194061857));
#37719=CARTESIAN_POINT('Ctrl Pts',(3.05045678021504,1.,2.44254768923105));
#37720=CARTESIAN_POINT('Ctrl Pts',(3.05736242671506,1.,2.44541251892556));
#37721=CARTESIAN_POINT('Ctrl Pts',(3.06431596421405,1.,2.44824970516544));
#37722=CARTESIAN_POINT('Ctrl Pts',(3.07131290521297,1.,2.45105688854422));
#37723=CARTESIAN_POINT('Ctrl Pts',(3.07834472886139,1.,2.4538282678779));
#37724=CARTESIAN_POINT('Ctrl Pts',(3.08540206545315,1.,2.45655725437039));
#37725=CARTESIAN_POINT('Ctrl Pts',(3.09247787931887,1.,2.4592391256388));
#37726=CARTESIAN_POINT('Ctrl Pts',(3.09956993697052,1.,2.46187308501884));
#37727=CARTESIAN_POINT('Ctrl Pts',(3.1066790790198,1.,2.46446082979646));
#37728=CARTESIAN_POINT('Ctrl Pts',(3.11380805536122,1.,2.46700558843506));
#37729=CARTESIAN_POINT('Ctrl Pts',(3.12096015766983,1.,2.46951098947469));
#37730=CARTESIAN_POINT('Ctrl Pts',(3.12813790805952,1.,2.47197997765871));
#37731=CARTESIAN_POINT('Ctrl Pts',(3.13534181229295,1.,2.47441378371932));
#37732=CARTESIAN_POINT('Ctrl Pts',(3.1425709954655,1.,2.47681245356109));
#37733=CARTESIAN_POINT('Ctrl Pts',(3.14982373241352,1.,2.47917529057029));
#37734=CARTESIAN_POINT('Ctrl Pts',(3.15709802322739,1.,2.48150133566571));
#37735=CARTESIAN_POINT('Ctrl Pts',(3.16439213290161,1.,2.48378981792725));
#37736=CARTESIAN_POINT('Ctrl Pts',(3.17170518863313,1.,2.48604065348587));
#37737=CARTESIAN_POINT('Ctrl Pts',(3.17903698136622,1.,2.48825428288201));
#37738=CARTESIAN_POINT('Ctrl Pts',(3.18638771282266,1.,2.49043146334059));
#37739=CARTESIAN_POINT('Ctrl Pts',(3.19375775555798,1.,2.49257307239848));
#37740=CARTESIAN_POINT('Ctrl Pts',(3.20114742397588,1.,2.49467992057755));
#37741=CARTESIAN_POINT('Ctrl Pts',(3.20855669849836,1.,2.4967525264737));
#37742=CARTESIAN_POINT('Ctrl Pts',(3.21598526261286,1.,2.4987911459939));
#37743=CARTESIAN_POINT('Ctrl Pts',(3.22343262620503,1.,2.50079587201958));
#37744=CARTESIAN_POINT('Ctrl Pts',(3.23089822320646,1.,2.50276671338111));
#37745=CARTESIAN_POINT('Ctrl Pts',(3.23838151080319,1.,2.5047036758003));
#37746=CARTESIAN_POINT('Ctrl Pts',(3.24588208983849,1.,2.506606859405));
#37747=CARTESIAN_POINT('Ctrl Pts',(3.25339971460982,1.,2.50847647070723));
#37748=CARTESIAN_POINT('Ctrl Pts',(3.26093423001434,1.,2.51031277813486));
#37749=CARTESIAN_POINT('Ctrl Pts',(3.26848552888115,1.,2.51211608411423));
#37750=CARTESIAN_POINT('Ctrl Pts',(3.27605350473142,1.,2.513886692704));
#37751=CARTESIAN_POINT('Ctrl Pts',(3.28363799702982,1.,2.51562487464514));
#37752=CARTESIAN_POINT('Ctrl Pts',(3.2912387729927,1.,2.51733085123797));
#37753=CARTESIAN_POINT('Ctrl Pts',(3.29885556388352,1.,2.51900480701069));
#37754=CARTESIAN_POINT('Ctrl Pts',(3.30648808815442,1.,2.52064689568511));
#37755=CARTESIAN_POINT('Ctrl Pts',(3.31413607874645,1.,2.52225724871313));
#37756=CARTESIAN_POINT('Ctrl Pts',(3.32179931078699,1.,2.5238359839626));
#37757=CARTESIAN_POINT('Ctrl Pts',(3.32947762187533,1.,2.52538321164634));
#37758=CARTESIAN_POINT('Ctrl Pts',(3.33717089999103,1.,2.52689902690158));
#37759=CARTESIAN_POINT('Ctrl Pts',(3.34333744115511,1.,2.52808660915689));
#37760=CARTESIAN_POINT('Ctrl Pts',(3.34796903576663,1.,2.52896321610703));
#37761=CARTESIAN_POINT('Ctrl Pts',(3.35105973714071,1.,2.5295413654909));
#37762=CARTESIAN_POINT('Ctrl Pts',(3.35260583073571,1.,2.52982887637028));
#37763=CARTESIAN_POINT('Origin',(3.35260583073571,0.,2.52982887637028));
#37764=CARTESIAN_POINT('',(3.44202241512147,1.,2.40675750623143));
#37765=CARTESIAN_POINT('Origin',(0.,0.,0.));
#37766=CARTESIAN_POINT('',(2.79140942341378,1.,2.50410331873042));
#37767=CARTESIAN_POINT('Origin',(0.,1.,0.));
#37768=CARTESIAN_POINT('Ctrl Pts',(2.79140942341378,1.,2.50410331873043));
#37769=CARTESIAN_POINT('Ctrl Pts',(2.79140942341378,0.666666666666667,2.50410331873043));
#37770=CARTESIAN_POINT('Ctrl Pts',(2.79140942341378,0.333333333333333,2.50410331873042));
#37771=CARTESIAN_POINT('Ctrl Pts',(2.79140942341378,-0.333333333333333,
2.50410331873042));
#37772=CARTESIAN_POINT('Ctrl Pts',(2.79140942341378,-0.666666666666667,
2.50410331873042));
#37773=CARTESIAN_POINT('Ctrl Pts',(2.79140942341378,-1.,2.50410331873042));
#37774=CARTESIAN_POINT('Ctrl Pts',(3.02314558451372,-1.,2.91557726271063));
#37775=CARTESIAN_POINT('Ctrl Pts',(3.02314558451372,1.,2.91557726271063));
#37776=CARTESIAN_POINT('Ctrl Pts',(3.02261975104912,-1.,2.91409518070707));
#37777=CARTESIAN_POINT('Ctrl Pts',(3.02261975104912,1.,2.91409518070707));
#37778=CARTESIAN_POINT('Ctrl Pts',(3.02156522743299,-1.,2.91113297349052));
#37779=CARTESIAN_POINT('Ctrl Pts',(3.02156522743299,1.,2.91113297349052));
#37780=CARTESIAN_POINT('Ctrl Pts',(3.01997487194926,-1.,2.90669553303902));
#37781=CARTESIAN_POINT('Ctrl Pts',(3.01997487194926,1.,2.90669553303902));
#37782=CARTESIAN_POINT('Ctrl Pts',(3.01783725123646,-1.,2.90079069102661));
#37783=CARTESIAN_POINT('Ctrl Pts',(3.01783725123646,1.,2.90079069102661));
#37784=CARTESIAN_POINT('Ctrl Pts',(3.01513660433291,-1.,2.8934292556764));
#37785=CARTESIAN_POINT('Ctrl Pts',(3.01513660433291,1.,2.8934292556764));
#37786=CARTESIAN_POINT('Ctrl Pts',(3.01240727309568,-1.,2.88608751706796));
#37787=CARTESIAN_POINT('Ctrl Pts',(3.01240727309568,1.,2.88608751706796));
#37788=CARTESIAN_POINT('Ctrl Pts',(3.0096491810855,-1.,2.87876560072799));
#37789=CARTESIAN_POINT('Ctrl Pts',(3.0096491810855,1.,2.87876560072799));
#37790=CARTESIAN_POINT('Ctrl Pts',(3.00686224485374,-1.,2.87146368430104));
#37791=CARTESIAN_POINT('Ctrl Pts',(3.00686224485374,1.,2.87146368430104));
#37792=CARTESIAN_POINT('Ctrl Pts',(3.00404638316245,-1.,2.86418200833065));
#37793=CARTESIAN_POINT('Ctrl Pts',(3.00404638316245,1.,2.86418200833065));
#37794=CARTESIAN_POINT('Ctrl Pts',(3.0012015079552,-1.,2.85692085715129));
#37795=CARTESIAN_POINT('Ctrl Pts',(3.0012015079552,1.,2.85692085715129));
#37796=CARTESIAN_POINT('Ctrl Pts',(2.99832751144566,-1.,2.84968053289104));
#37797=CARTESIAN_POINT('Ctrl Pts',(2.99832751144566,1.,2.84968053289104));
#37798=CARTESIAN_POINT('Ctrl Pts',(2.995424253416,-1.,2.84246132984334));
#37799=CARTESIAN_POINT('Ctrl Pts',(2.995424253416,1.,2.84246132984334));
#37800=CARTESIAN_POINT('Ctrl Pts',(2.99249155170479,-1.,2.83526351254383));
#37801=CARTESIAN_POINT('Ctrl Pts',(2.99249155170479,1.,2.83526351254383));
#37802=CARTESIAN_POINT('Ctrl Pts',(2.98952916401699,-1.,2.82808728190402));
#37803=CARTESIAN_POINT('Ctrl Pts',(2.98952916401699,1.,2.82808728190402));
#37804=CARTESIAN_POINT('Ctrl Pts',(2.98653680669434,-1.,2.82093279065704));
#37805=CARTESIAN_POINT('Ctrl Pts',(2.98653680669434,1.,2.82093279065704));
#37806=CARTESIAN_POINT('Ctrl Pts',(2.9835141977994,-1.,2.81380019196454));
#37807=CARTESIAN_POINT('Ctrl Pts',(2.9835141977994,1.,2.81380019196454));
#37808=CARTESIAN_POINT('Ctrl Pts',(2.98046109647299,-1.,2.80668968101162));
#37809=CARTESIAN_POINT('Ctrl Pts',(2.98046109647299,1.,2.80668968101162));
#37810=CARTESIAN_POINT('Ctrl Pts',(2.97737733718242,-1.,2.79960153278186));
#37811=CARTESIAN_POINT('Ctrl Pts',(2.97737733718242,1.,2.79960153278186));
#37812=CARTESIAN_POINT('Ctrl Pts',(2.97426288347475,-1.,2.79253615718147));
#37813=CARTESIAN_POINT('Ctrl Pts',(2.97426288347475,1.,2.79253615718147));
#37814=CARTESIAN_POINT('Ctrl Pts',(2.97111781461349,-1.,2.78549409123657));
#37815=CARTESIAN_POINT('Ctrl Pts',(2.97111781461349,1.,2.78549409123657));
#37816=CARTESIAN_POINT('Ctrl Pts',(2.9679422104295,-1.,2.77847589542767));
#37817=CARTESIAN_POINT('Ctrl Pts',(2.9679422104295,1.,2.77847589542767));
#37818=CARTESIAN_POINT('Ctrl Pts',(2.96473605585548,-1.,2.77148206836464));
#37819=CARTESIAN_POINT('Ctrl Pts',(2.96473605585548,1.,2.77148206836464));
#37820=CARTESIAN_POINT('Ctrl Pts',(2.96149914764832,-1.,2.76451296269571));
#37821=CARTESIAN_POINT('Ctrl Pts',(2.96149914764832,1.,2.76451296269571));
#37822=CARTESIAN_POINT('Ctrl Pts',(2.9582309766594,-1.,2.75756867888393));
#37823=CARTESIAN_POINT('Ctrl Pts',(2.9582309766594,1.,2.75756867888393));
#37824=CARTESIAN_POINT('Ctrl Pts',(2.95493069316211,-1.,2.75064903318996));
#37825=CARTESIAN_POINT('Ctrl Pts',(2.95493069316211,1.,2.75064903318996));
#37826=CARTESIAN_POINT('Ctrl Pts',(2.95159737214304,-1.,2.7437537949221));
#37827=CARTESIAN_POINT('Ctrl Pts',(2.95159737214304,1.,2.7437537949221));
#37828=CARTESIAN_POINT('Ctrl Pts',(2.94823023414381,-1.,2.73688288329825));
#37829=CARTESIAN_POINT('Ctrl Pts',(2.94823023414381,1.,2.73688288329825));
#37830=CARTESIAN_POINT('Ctrl Pts',(2.94482887675139,-1.,2.73003657371613));
#37831=CARTESIAN_POINT('Ctrl Pts',(2.94482887675139,1.,2.73003657371613));
#37832=CARTESIAN_POINT('Ctrl Pts',(2.94139351933882,-1.,2.72321571511322));
#37833=CARTESIAN_POINT('Ctrl Pts',(2.94139351933882,1.,2.72321571511322));
#37834=CARTESIAN_POINT('Ctrl Pts',(2.93792519474955,-1.,2.71642190053575));
#37835=CARTESIAN_POINT('Ctrl Pts',(2.93792519474955,1.,2.71642190053575));
#37836=CARTESIAN_POINT('Ctrl Pts',(2.93442516311167,-1.,2.70965695523776));
#37837=CARTESIAN_POINT('Ctrl Pts',(2.93442516311167,1.,2.70965695523776));
#37838=CARTESIAN_POINT('Ctrl Pts',(2.93089438233746,-1.,2.70292247416881));
#37839=CARTESIAN_POINT('Ctrl Pts',(2.93089438233746,1.,2.70292247416881));
#37840=CARTESIAN_POINT('Ctrl Pts',(2.92733294395268,-1.,2.69621932864302));
#37841=CARTESIAN_POINT('Ctrl Pts',(2.92733294395268,1.,2.69621932864302));
#37842=CARTESIAN_POINT('Ctrl Pts',(2.92373955325876,-1.,2.68954721165342));
#37843=CARTESIAN_POINT('Ctrl Pts',(2.92373955325876,1.,2.68954721165342));
#37844=CARTESIAN_POINT('Ctrl Pts',(2.92011090722152,-1.,2.68290409279689));
#37845=CARTESIAN_POINT('Ctrl Pts',(2.92011090722152,1.,2.68290409279689));
#37846=CARTESIAN_POINT('Ctrl Pts',(2.91644290704281,-1.,2.67628728855309));
#37847=CARTESIAN_POINT('Ctrl Pts',(2.91644290704281,1.,2.67628728855309));
#37848=CARTESIAN_POINT('Ctrl Pts',(2.91273193382876,-1.,2.66969458792627));
#37849=CARTESIAN_POINT('Ctrl Pts',(2.91273193382876,1.,2.66969458792627));
#37850=CARTESIAN_POINT('Ctrl Pts',(2.90897617968921,-1.,2.66312542616809));
#37851=CARTESIAN_POINT('Ctrl Pts',(2.90897617968921,1.,2.66312542616809));
#37852=CARTESIAN_POINT('Ctrl Pts',(2.90517678087467,-1.,2.65658188464287));
#37853=CARTESIAN_POINT('Ctrl Pts',(2.90517678087467,1.,2.65658188464287));
#37854=CARTESIAN_POINT('Ctrl Pts',(2.90133950224879,-1.,2.65007017365576));
#37855=CARTESIAN_POINT('Ctrl Pts',(2.90133950224879,1.,2.65007017365576));
#37856=CARTESIAN_POINT('Ctrl Pts',(2.89747231723361,-1.,2.64359851684146));
#37857=CARTESIAN_POINT('Ctrl Pts',(2.89747231723361,1.,2.64359851684146));
#37858=CARTESIAN_POINT('Ctrl Pts',(2.89358228854557,-1.,2.63717442263944));
#37859=CARTESIAN_POINT('Ctrl Pts',(2.89358228854557,1.,2.63717442263944));
#37860=CARTESIAN_POINT('Ctrl Pts',(2.88967244854243,-1.,2.63080195420771));
#37861=CARTESIAN_POINT('Ctrl Pts',(2.88967244854243,1.,2.63080195420771));
#37862=CARTESIAN_POINT('Ctrl Pts',(2.88573922195049,-1.,2.62447947640253));
#37863=CARTESIAN_POINT('Ctrl Pts',(2.88573922195049,1.,2.62447947640253));
#37864=CARTESIAN_POINT('Ctrl Pts',(2.88176821427502,-1.,2.61819596473087));
#37865=CARTESIAN_POINT('Ctrl Pts',(2.88176821427502,1.,2.61819596473087));
#37866=CARTESIAN_POINT('Ctrl Pts',(2.87773881947885,-1.,2.61193507170928));
#37867=CARTESIAN_POINT('Ctrl Pts',(2.87773881947885,1.,2.61193507170928));
#37868=CARTESIAN_POINT('Ctrl Pts',(2.87363176656475,-1.,2.6056817788128));
#37869=CARTESIAN_POINT('Ctrl Pts',(2.87363176656475,1.,2.6056817788128));
#37870=CARTESIAN_POINT('Ctrl Pts',(2.86943633170712,-1.,2.59942875223202));
#37871=CARTESIAN_POINT('Ctrl Pts',(2.86943633170712,1.,2.59942875223202));
#37872=CARTESIAN_POINT('Ctrl Pts',(2.86515629953528,-1.,2.59318160184921));
#37873=CARTESIAN_POINT('Ctrl Pts',(2.86515629953528,1.,2.59318160184921));
#37874=CARTESIAN_POINT('Ctrl Pts',(2.86081999003668,-1.,2.5869677064356));
#37875=CARTESIAN_POINT('Ctrl Pts',(2.86081999003668,1.,2.5869677064356));
#37876=CARTESIAN_POINT('Ctrl Pts',(2.85647171715147,-1.,2.58082875254407));
#37877=CARTESIAN_POINT('Ctrl Pts',(2.85647171715147,1.,2.58082875254407));
#37878=CARTESIAN_POINT('Ctrl Pts',(2.85215360144482,-1.,2.57480482727128));
#37879=CARTESIAN_POINT('Ctrl Pts',(2.85215360144482,1.,2.57480482727128));
#37880=CARTESIAN_POINT('Ctrl Pts',(2.84788893329091,-1.,2.56891984251743));
#37881=CARTESIAN_POINT('Ctrl Pts',(2.84788893329091,1.,2.56891984251743));
#37882=CARTESIAN_POINT('Ctrl Pts',(2.84366802680211,-1.,2.56316920798489));
#37883=CARTESIAN_POINT('Ctrl Pts',(2.84366802680211,1.,2.56316920798489));
#37884=CARTESIAN_POINT('Ctrl Pts',(2.83942515220699,-1.,2.55749952145165));
#37885=CARTESIAN_POINT('Ctrl Pts',(2.83942515220699,1.,2.55749952145165));
#37886=CARTESIAN_POINT('Ctrl Pts',(2.83505269592412,-1.,2.55182152806964));
#37887=CARTESIAN_POINT('Ctrl Pts',(2.83505269592412,1.,2.55182152806964));
#37888=CARTESIAN_POINT('Ctrl Pts',(2.83044254225794,-1.,2.54604736792542));
#37889=CARTESIAN_POINT('Ctrl Pts',(2.83044254225794,1.,2.54604736792542));
#37890=CARTESIAN_POINT('Ctrl Pts',(2.82552167649157,-1.,2.54012272520141));
#37891=CARTESIAN_POINT('Ctrl Pts',(2.82552167649157,1.,2.54012272520141));
#37892=CARTESIAN_POINT('Ctrl Pts',(2.82028550483744,-1.,2.53405679667463));
#37893=CARTESIAN_POINT('Ctrl Pts',(2.82028550483744,1.,2.53405679667463));
#37894=CARTESIAN_POINT('Ctrl Pts',(2.8148437904867,-1.,2.52796388055457));
#37895=CARTESIAN_POINT('Ctrl Pts',(2.8148437904867,1.,2.52796388055457));
#37896=CARTESIAN_POINT('Ctrl Pts',(2.80941521967234,-1.,2.52205778589922));
#37897=CARTESIAN_POINT('Ctrl Pts',(2.80941521967234,1.,2.52205778589922));
#37898=CARTESIAN_POINT('Ctrl Pts',(2.80427363984939,-1.,2.51660190466067));
#37899=CARTESIAN_POINT('Ctrl Pts',(2.80427363984939,1.,2.51660190466067));
#37900=CARTESIAN_POINT('Ctrl Pts',(2.79970585014308,-1.,2.51186983687947));
#37901=CARTESIAN_POINT('Ctrl Pts',(2.79970585014308,1.,2.51186983687947));
#37902=CARTESIAN_POINT('Ctrl Pts',(2.7959687805717,-1.,2.50810555977564));
#37903=CARTESIAN_POINT('Ctrl Pts',(2.7959687805717,1.,2.50810555977564));
#37904=CARTESIAN_POINT('Ctrl Pts',(2.79323694088143,-1.,2.50547439929077));
#37905=CARTESIAN_POINT('Ctrl Pts',(2.79323694088143,1.,2.50547439929077));
#37906=CARTESIAN_POINT('Ctrl Pts',(2.79192122906739,-1.,2.50433799076945));
#37907=CARTESIAN_POINT('Ctrl Pts',(2.79192122906739,1.,2.50433799076945));
#37908=CARTESIAN_POINT('Ctrl Pts',(2.79143626022225,-1.,2.50404230339032));
#37909=CARTESIAN_POINT('Ctrl Pts',(2.79143626022225,1.,2.50404230339032));
#37910=CARTESIAN_POINT('Ctrl Pts',(2.79133581100044,-1.,2.50409239460011));
#37911=CARTESIAN_POINT('Ctrl Pts',(2.79133581100044,1.,2.50409239460011));
#37912=CARTESIAN_POINT('Ctrl Pts',(2.79134130681569,-1.,2.50417924854921));
#37913=CARTESIAN_POINT('Ctrl Pts',(2.79134130681569,1.,2.50417924854921));
#37914=CARTESIAN_POINT('',(3.02314558451372,1.,2.91557726271063));
#37915=CARTESIAN_POINT('Ctrl Pts',(3.02314558451372,1.,2.91557726271063));
#37916=CARTESIAN_POINT('Ctrl Pts',(3.02261975104912,1.,2.91409518070707));
#37917=CARTESIAN_POINT('Ctrl Pts',(3.02156522743299,1.,2.91113297349052));
#37918=CARTESIAN_POINT('Ctrl Pts',(3.01997487194926,1.,2.90669553303902));
#37919=CARTESIAN_POINT('Ctrl Pts',(3.01783725123646,1.,2.90079069102661));
#37920=CARTESIAN_POINT('Ctrl Pts',(3.01513660433291,1.,2.8934292556764));
#37921=CARTESIAN_POINT('Ctrl Pts',(3.01240727309568,1.,2.88608751706796));
#37922=CARTESIAN_POINT('Ctrl Pts',(3.0096491810855,1.,2.87876560072799));
#37923=CARTESIAN_POINT('Ctrl Pts',(3.00686224485374,1.,2.87146368430104));
#37924=CARTESIAN_POINT('Ctrl Pts',(3.00404638316245,1.,2.86418200833065));
#37925=CARTESIAN_POINT('Ctrl Pts',(3.0012015079552,1.,2.85692085715129));
#37926=CARTESIAN_POINT('Ctrl Pts',(2.99832751144566,1.,2.84968053289104));
#37927=CARTESIAN_POINT('Ctrl Pts',(2.995424253416,1.,2.84246132984334));
#37928=CARTESIAN_POINT('Ctrl Pts',(2.99249155170479,1.,2.83526351254383));
#37929=CARTESIAN_POINT('Ctrl Pts',(2.98952916401699,1.,2.82808728190402));
#37930=CARTESIAN_POINT('Ctrl Pts',(2.98653680669434,1.,2.82093279065704));
#37931=CARTESIAN_POINT('Ctrl Pts',(2.9835141977994,1.,2.81380019196454));
#37932=CARTESIAN_POINT('Ctrl Pts',(2.98046109647299,1.,2.80668968101162));
#37933=CARTESIAN_POINT('Ctrl Pts',(2.97737733718242,1.,2.79960153278186));
#37934=CARTESIAN_POINT('Ctrl Pts',(2.97426288347475,1.,2.79253615718147));
#37935=CARTESIAN_POINT('Ctrl Pts',(2.97111781461349,1.,2.78549409123657));
#37936=CARTESIAN_POINT('Ctrl Pts',(2.9679422104295,1.,2.77847589542767));
#37937=CARTESIAN_POINT('Ctrl Pts',(2.96473605585548,1.,2.77148206836464));
#37938=CARTESIAN_POINT('Ctrl Pts',(2.96149914764832,1.,2.76451296269571));
#37939=CARTESIAN_POINT('Ctrl Pts',(2.9582309766594,1.,2.75756867888393));
#37940=CARTESIAN_POINT('Ctrl Pts',(2.95493069316211,1.,2.75064903318996));
#37941=CARTESIAN_POINT('Ctrl Pts',(2.95159737214304,1.,2.7437537949221));
#37942=CARTESIAN_POINT('Ctrl Pts',(2.94823023414381,1.,2.73688288329825));
#37943=CARTESIAN_POINT('Ctrl Pts',(2.94482887675139,1.,2.73003657371613));
#37944=CARTESIAN_POINT('Ctrl Pts',(2.94139351933882,1.,2.72321571511322));
#37945=CARTESIAN_POINT('Ctrl Pts',(2.93792519474955,1.,2.71642190053575));
#37946=CARTESIAN_POINT('Ctrl Pts',(2.93442516311167,1.,2.70965695523776));
#37947=CARTESIAN_POINT('Ctrl Pts',(2.93089438233746,1.,2.70292247416881));
#37948=CARTESIAN_POINT('Ctrl Pts',(2.92733294395268,1.,2.69621932864302));
#37949=CARTESIAN_POINT('Ctrl Pts',(2.92373955325876,1.,2.68954721165342));
#37950=CARTESIAN_POINT('Ctrl Pts',(2.92011090722152,1.,2.68290409279689));
#37951=CARTESIAN_POINT('Ctrl Pts',(2.91644290704281,1.,2.67628728855309));
#37952=CARTESIAN_POINT('Ctrl Pts',(2.91273193382876,1.,2.66969458792627));
#37953=CARTESIAN_POINT('Ctrl Pts',(2.90897617968921,1.,2.66312542616809));
#37954=CARTESIAN_POINT('Ctrl Pts',(2.90517678087467,1.,2.65658188464287));
#37955=CARTESIAN_POINT('Ctrl Pts',(2.90133950224879,1.,2.65007017365576));
#37956=CARTESIAN_POINT('Ctrl Pts',(2.89747231723361,1.,2.64359851684146));
#37957=CARTESIAN_POINT('Ctrl Pts',(2.89358228854557,1.,2.63717442263944));
#37958=CARTESIAN_POINT('Ctrl Pts',(2.88967244854243,1.,2.63080195420771));
#37959=CARTESIAN_POINT('Ctrl Pts',(2.88573922195049,1.,2.62447947640253));
#37960=CARTESIAN_POINT('Ctrl Pts',(2.88176821427502,1.,2.61819596473087));
#37961=CARTESIAN_POINT('Ctrl Pts',(2.87773881947885,1.,2.61193507170928));
#37962=CARTESIAN_POINT('Ctrl Pts',(2.87363176656475,1.,2.6056817788128));
#37963=CARTESIAN_POINT('Ctrl Pts',(2.86943633170712,1.,2.59942875223202));
#37964=CARTESIAN_POINT('Ctrl Pts',(2.86515629953528,1.,2.59318160184921));
#37965=CARTESIAN_POINT('Ctrl Pts',(2.86081999003668,1.,2.5869677064356));
#37966=CARTESIAN_POINT('Ctrl Pts',(2.85647171715147,1.,2.58082875254407));
#37967=CARTESIAN_POINT('Ctrl Pts',(2.85215360144482,1.,2.57480482727128));
#37968=CARTESIAN_POINT('Ctrl Pts',(2.84788893329091,1.,2.56891984251743));
#37969=CARTESIAN_POINT('Ctrl Pts',(2.84366802680211,1.,2.56316920798489));
#37970=CARTESIAN_POINT('Ctrl Pts',(2.83942515220699,1.,2.55749952145165));
#37971=CARTESIAN_POINT('Ctrl Pts',(2.83505269592412,1.,2.55182152806964));
#37972=CARTESIAN_POINT('Ctrl Pts',(2.83044254225794,1.,2.54604736792542));
#37973=CARTESIAN_POINT('Ctrl Pts',(2.82552167649157,1.,2.54012272520141));
#37974=CARTESIAN_POINT('Ctrl Pts',(2.82028550483744,1.,2.53405679667463));
#37975=CARTESIAN_POINT('Ctrl Pts',(2.8148437904867,1.,2.52796388055457));
#37976=CARTESIAN_POINT('Ctrl Pts',(2.80941521967234,1.,2.52205778589922));
#37977=CARTESIAN_POINT('Ctrl Pts',(2.80427363984939,1.,2.51660190466067));
#37978=CARTESIAN_POINT('Ctrl Pts',(2.79970585014308,1.,2.51186983687947));
#37979=CARTESIAN_POINT('Ctrl Pts',(2.7959687805717,1.,2.50810555977564));
#37980=CARTESIAN_POINT('Ctrl Pts',(2.79344192164204,1.,2.50567182569153));
#37981=CARTESIAN_POINT('Ctrl Pts',(2.79217568804874,1.,2.50455968395235));
#37982=CARTESIAN_POINT('Ctrl Pts',(2.79164172519039,1.,2.50417932839344));
#37983=CARTESIAN_POINT('Ctrl Pts',(2.79145823440899,1.,2.50410700351426));
#37984=CARTESIAN_POINT('Ctrl Pts',(2.79140942341378,1.,2.50410331873042));
#37985=CARTESIAN_POINT('',(3.02314558451372,0.,2.91557726271063));
#37986=CARTESIAN_POINT('Ctrl Pts',(2.5041792485492,-1.,2.79134130681569));
#37987=CARTESIAN_POINT('Ctrl Pts',(2.5041792485492,1.,2.79134130681569));
#37988=CARTESIAN_POINT('Ctrl Pts',(2.50409239460108,-1.,2.7913358110015));
#37989=CARTESIAN_POINT('Ctrl Pts',(2.50409239460108,1.,2.7913358110015));
#37990=CARTESIAN_POINT('Ctrl Pts',(2.50404230339286,-1.,2.79143626022503));
#37991=CARTESIAN_POINT('Ctrl Pts',(2.50404230339286,1.,2.79143626022503));
#37992=CARTESIAN_POINT('Ctrl Pts',(2.5043379907732,-1.,2.79192122907148));
#37993=CARTESIAN_POINT('Ctrl Pts',(2.5043379907732,1.,2.79192122907148));
#37994=CARTESIAN_POINT('Ctrl Pts',(2.50547439929414,-1.,2.7932369408851));
#37995=CARTESIAN_POINT('Ctrl Pts',(2.50547439929414,1.,2.7932369408851));
#37996=CARTESIAN_POINT('Ctrl Pts',(2.5081055597767,-1.,2.79596878057287));
#37997=CARTESIAN_POINT('Ctrl Pts',(2.5081055597767,1.,2.79596878057287));
#37998=CARTESIAN_POINT('Ctrl Pts',(2.51186983687818,-1.,2.79970585014168));
#37999=CARTESIAN_POINT('Ctrl Pts',(2.51186983687818,1.,2.79970585014168));
#38000=CARTESIAN_POINT('Ctrl Pts',(2.51660190465805,-1.,2.80427363984653));
#38001=CARTESIAN_POINT('Ctrl Pts',(2.51660190465805,1.,2.80427363984653));
#38002=CARTESIAN_POINT('Ctrl Pts',(2.52205778589653,-1.,2.80941521966941));
#38003=CARTESIAN_POINT('Ctrl Pts',(2.52205778589653,1.,2.80941521966941));
#38004=CARTESIAN_POINT('Ctrl Pts',(2.52796388055278,-1.,2.81484379048475));
#38005=CARTESIAN_POINT('Ctrl Pts',(2.52796388055278,1.,2.81484379048475));
#38006=CARTESIAN_POINT('Ctrl Pts',(2.53405679667412,-1.,2.82028550483689));
#38007=CARTESIAN_POINT('Ctrl Pts',(2.53405679667412,1.,2.82028550483689));
#38008=CARTESIAN_POINT('Ctrl Pts',(2.54012272520199,-1.,2.8255216764922));
#38009=CARTESIAN_POINT('Ctrl Pts',(2.54012272520199,1.,2.8255216764922));
#38010=CARTESIAN_POINT('Ctrl Pts',(2.54604736792655,-1.,2.83044254225917));
#38011=CARTESIAN_POINT('Ctrl Pts',(2.54604736792655,1.,2.83044254225917));
#38012=CARTESIAN_POINT('Ctrl Pts',(2.55182152807077,-1.,2.83505269592536));
#38013=CARTESIAN_POINT('Ctrl Pts',(2.55182152807077,1.,2.83505269592536));
#38014=CARTESIAN_POINT('Ctrl Pts',(2.55749952145241,-1.,2.83942515220782));
#38015=CARTESIAN_POINT('Ctrl Pts',(2.55749952145241,1.,2.83942515220782));
#38016=CARTESIAN_POINT('Ctrl Pts',(2.56316920798513,-1.,2.84366802680237));
#38017=CARTESIAN_POINT('Ctrl Pts',(2.56316920798513,1.,2.84366802680237));
#38018=CARTESIAN_POINT('Ctrl Pts',(2.56891984251721,-1.,2.84788893329067));
#38019=CARTESIAN_POINT('Ctrl Pts',(2.56891984251721,1.,2.84788893329067));
#38020=CARTESIAN_POINT('Ctrl Pts',(2.57480482727081,-1.,2.85215360144431));
#38021=CARTESIAN_POINT('Ctrl Pts',(2.57480482727081,1.,2.85215360144431));
#38022=CARTESIAN_POINT('Ctrl Pts',(2.58082875254357,-1.,2.85647171715092));
#38023=CARTESIAN_POINT('Ctrl Pts',(2.58082875254357,1.,2.85647171715092));
#38024=CARTESIAN_POINT('Ctrl Pts',(2.58696770643524,-1.,2.86081999003629));
#38025=CARTESIAN_POINT('Ctrl Pts',(2.58696770643524,1.,2.86081999003629));
#38026=CARTESIAN_POINT('Ctrl Pts',(2.59318160184908,-1.,2.86515629953513));
#38027=CARTESIAN_POINT('Ctrl Pts',(2.59318160184908,1.,2.86515629953513));
#38028=CARTESIAN_POINT('Ctrl Pts',(2.5994287522321,-1.,2.86943633170722));
#38029=CARTESIAN_POINT('Ctrl Pts',(2.5994287522321,1.,2.86943633170722));
#38030=CARTESIAN_POINT('Ctrl Pts',(2.60568177881303,-1.,2.87363176656501));
#38031=CARTESIAN_POINT('Ctrl Pts',(2.60568177881303,1.,2.87363176656501));
#38032=CARTESIAN_POINT('Ctrl Pts',(2.61193507170955,-1.,2.87773881947916));
#38033=CARTESIAN_POINT('Ctrl Pts',(2.61193507170955,1.,2.87773881947916));
#38034=CARTESIAN_POINT('Ctrl Pts',(2.61819596473108,-1.,2.88176821427525));
#38035=CARTESIAN_POINT('Ctrl Pts',(2.61819596473108,1.,2.88176821427525));
#38036=CARTESIAN_POINT('Ctrl Pts',(2.62447947640262,-1.,2.88573922195059));
#38037=CARTESIAN_POINT('Ctrl Pts',(2.62447947640262,1.,2.88573922195059));
#38038=CARTESIAN_POINT('Ctrl Pts',(2.63080195420767,-1.,2.88967244854239));
#38039=CARTESIAN_POINT('Ctrl Pts',(2.63080195420767,1.,2.88967244854239));
#38040=CARTESIAN_POINT('Ctrl Pts',(2.63717442263932,-1.,2.89358228854544));
#38041=CARTESIAN_POINT('Ctrl Pts',(2.63717442263932,1.,2.89358228854544));
#38042=CARTESIAN_POINT('Ctrl Pts',(2.64359851684131,-1.,2.89747231723345));
#38043=CARTESIAN_POINT('Ctrl Pts',(2.64359851684131,1.,2.89747231723345));
#38044=CARTESIAN_POINT('Ctrl Pts',(2.65007017365564,-1.,2.90133950224867));
#38045=CARTESIAN_POINT('Ctrl Pts',(2.65007017365564,1.,2.90133950224867));
#38046=CARTESIAN_POINT('Ctrl Pts',(2.65658188464282,-1.,2.90517678087461));
#38047=CARTESIAN_POINT('Ctrl Pts',(2.65658188464282,1.,2.90517678087461));
#38048=CARTESIAN_POINT('Ctrl Pts',(2.6631254261681,-1.,2.90897617968923));
#38049=CARTESIAN_POINT('Ctrl Pts',(2.6631254261681,1.,2.90897617968923));
#38050=CARTESIAN_POINT('Ctrl Pts',(2.66969458792631,-1.,2.91273193382882));
#38051=CARTESIAN_POINT('Ctrl Pts',(2.66969458792631,1.,2.91273193382882));
#38052=CARTESIAN_POINT('Ctrl Pts',(2.67628728855312,-1.,2.91644290704285));
#38053=CARTESIAN_POINT('Ctrl Pts',(2.67628728855312,1.,2.91644290704285));
#38054=CARTESIAN_POINT('Ctrl Pts',(2.68290409279688,-1.,2.92011090722152));
#38055=CARTESIAN_POINT('Ctrl Pts',(2.68290409279688,1.,2.92011090722152));
#38056=CARTESIAN_POINT('Ctrl Pts',(2.68954721165339,-1.,2.92373955325875));
#38057=CARTESIAN_POINT('Ctrl Pts',(2.68954721165339,1.,2.92373955325875));
#38058=CARTESIAN_POINT('Ctrl Pts',(2.69621932864301,-1.,2.92733294395267));
#38059=CARTESIAN_POINT('Ctrl Pts',(2.69621932864301,1.,2.92733294395267));
#38060=CARTESIAN_POINT('Ctrl Pts',(2.70292247416885,-1.,2.9308943823375));
#38061=CARTESIAN_POINT('Ctrl Pts',(2.70292247416885,1.,2.9308943823375));
#38062=CARTESIAN_POINT('Ctrl Pts',(2.70965695523787,-1.,2.93442516311179));
#38063=CARTESIAN_POINT('Ctrl Pts',(2.70965695523787,1.,2.93442516311179));
#38064=CARTESIAN_POINT('Ctrl Pts',(2.71642190053592,-1.,2.93792519474972));
#38065=CARTESIAN_POINT('Ctrl Pts',(2.71642190053592,1.,2.93792519474972));
#38066=CARTESIAN_POINT('Ctrl Pts',(2.72321571511337,-1.,2.94139351933897));
#38067=CARTESIAN_POINT('Ctrl Pts',(2.72321571511337,1.,2.94139351933897));
#38068=CARTESIAN_POINT('Ctrl Pts',(2.73003657371616,-1.,2.94482887675143));
#38069=CARTESIAN_POINT('Ctrl Pts',(2.73003657371616,1.,2.94482887675143));
#38070=CARTESIAN_POINT('Ctrl Pts',(2.73688288329808,-1.,2.94823023414364));
#38071=CARTESIAN_POINT('Ctrl Pts',(2.73688288329808,1.,2.94823023414364));
#38072=CARTESIAN_POINT('Ctrl Pts',(2.74375379492172,-1.,2.95159737214266));
#38073=CARTESIAN_POINT('Ctrl Pts',(2.74375379492172,1.,2.95159737214266));
#38074=CARTESIAN_POINT('Ctrl Pts',(2.75064903318947,-1.,2.95493069316161));
#38075=CARTESIAN_POINT('Ctrl Pts',(2.75064903318947,1.,2.95493069316161));
#38076=CARTESIAN_POINT('Ctrl Pts',(2.7575686788835,-1.,2.95823097665896));
#38077=CARTESIAN_POINT('Ctrl Pts',(2.7575686788835,1.,2.95823097665896));
#38078=CARTESIAN_POINT('Ctrl Pts',(2.76451296269557,-1.,2.96149914764818));
#38079=CARTESIAN_POINT('Ctrl Pts',(2.76451296269557,1.,2.96149914764818));
#38080=CARTESIAN_POINT('Ctrl Pts',(2.77148206836498,-1.,2.96473605585583));
#38081=CARTESIAN_POINT('Ctrl Pts',(2.77148206836498,1.,2.96473605585583));
#38082=CARTESIAN_POINT('Ctrl Pts',(2.7784758954285,-1.,2.96794221043036));
#38083=CARTESIAN_POINT('Ctrl Pts',(2.7784758954285,1.,2.96794221043036));
#38084=CARTESIAN_POINT('Ctrl Pts',(2.78549409123769,-1.,2.97111781461465));
#38085=CARTESIAN_POINT('Ctrl Pts',(2.78549409123769,1.,2.97111781461465));
#38086=CARTESIAN_POINT('Ctrl Pts',(2.79253615718248,-1.,2.9742628834758));
#38087=CARTESIAN_POINT('Ctrl Pts',(2.79253615718248,1.,2.9742628834758));
#38088=CARTESIAN_POINT('Ctrl Pts',(2.7996015327823,-1.,2.97737733718287));
#38089=CARTESIAN_POINT('Ctrl Pts',(2.7996015327823,1.,2.97737733718287));
#38090=CARTESIAN_POINT('Ctrl Pts',(2.80668968101106,-1.,2.98046109647241));
#38091=CARTESIAN_POINT('Ctrl Pts',(2.80668968101106,1.,2.98046109647241));
#38092=CARTESIAN_POINT('Ctrl Pts',(2.81380019196286,-1.,2.98351419779767));
#38093=CARTESIAN_POINT('Ctrl Pts',(2.81380019196286,1.,2.98351419779767));
#38094=CARTESIAN_POINT('Ctrl Pts',(2.82093279065457,-1.,2.9865368066918));
#38095=CARTESIAN_POINT('Ctrl Pts',(2.82093279065457,1.,2.9865368066918));
#38096=CARTESIAN_POINT('Ctrl Pts',(2.82808728190157,-1.,2.98952916401446));
#38097=CARTESIAN_POINT('Ctrl Pts',(2.82808728190157,1.,2.98952916401446));
#38098=CARTESIAN_POINT('Ctrl Pts',(2.83526351254248,-1.,2.9924915517034));
#38099=CARTESIAN_POINT('Ctrl Pts',(2.83526351254248,1.,2.9924915517034));
#38100=CARTESIAN_POINT('Ctrl Pts',(2.84246132984415,-1.,2.99542425341685));
#38101=CARTESIAN_POINT('Ctrl Pts',(2.84246132984415,1.,2.99542425341685));
#38102=CARTESIAN_POINT('Ctrl Pts',(2.84968053289451,-1.,2.99832751144925));
#38103=CARTESIAN_POINT('Ctrl Pts',(2.84968053289451,1.,2.99832751144925));
#38104=CARTESIAN_POINT('Ctrl Pts',(2.85692085715685,-1.,3.00120150796095));
#38105=CARTESIAN_POINT('Ctrl Pts',(2.85692085715685,1.,3.00120150796095));
#38106=CARTESIAN_POINT('Ctrl Pts',(2.86418200833667,-1.,3.00404638316867));
#38107=CARTESIAN_POINT('Ctrl Pts',(2.86418200833667,1.,3.00404638316867));
#38108=CARTESIAN_POINT('Ctrl Pts',(2.87146368430501,-1.,3.00686224485784));
#38109=CARTESIAN_POINT('Ctrl Pts',(2.87146368430501,1.,3.00686224485784));
#38110=CARTESIAN_POINT('Ctrl Pts',(2.87876560072727,-1.,3.00964918108476));
#38111=CARTESIAN_POINT('Ctrl Pts',(2.87876560072727,1.,3.00964918108476));
#38112=CARTESIAN_POINT('Ctrl Pts',(2.8860875170608,-1.,3.01240727308829));
#38113=CARTESIAN_POINT('Ctrl Pts',(2.8860875170608,1.,3.01240727308829));
#38114=CARTESIAN_POINT('Ctrl Pts',(2.89342925566321,-1.,3.01513660431928));
#38115=CARTESIAN_POINT('Ctrl Pts',(2.89342925566321,1.,3.01513660431928));
#38116=CARTESIAN_POINT('Ctrl Pts',(2.9007906910105,-1.,3.01783725121981));
#38117=CARTESIAN_POINT('Ctrl Pts',(2.9007906910105,1.,3.01783725121981));
#38118=CARTESIAN_POINT('Ctrl Pts',(2.90669553302526,-1.,3.01997487193503));
#38119=CARTESIAN_POINT('Ctrl Pts',(2.90669553302526,1.,3.01997487193503));
#38120=CARTESIAN_POINT('Ctrl Pts',(2.91113297348212,-1.,3.02156522742431));
#38121=CARTESIAN_POINT('Ctrl Pts',(2.91113297348212,1.,3.02156522742431));
#38122=CARTESIAN_POINT('Ctrl Pts',(2.91409518070399,-1.,3.02261975104593));
#38123=CARTESIAN_POINT('Ctrl Pts',(2.91409518070399,1.,3.02261975104593));
#38124=CARTESIAN_POINT('Ctrl Pts',(2.91557726271063,-1.,3.02314558451372));
#38125=CARTESIAN_POINT('Ctrl Pts',(2.91557726271063,1.,3.02314558451372));
#38126=CARTESIAN_POINT('',(2.50410331873176,1.,2.79140942341258));
#38127=CARTESIAN_POINT('Ctrl Pts',(2.50410331873176,-1.,2.79140942341258));
#38128=CARTESIAN_POINT('Ctrl Pts',(2.50410331873176,-0.666666666666667,
2.79140942341258));
#38129=CARTESIAN_POINT('Ctrl Pts',(2.50410331873176,-0.333333333333333,
2.79140942341258));
#38130=CARTESIAN_POINT('Ctrl Pts',(2.50410331873176,0.333333333333333,2.79140942341258));
#38131=CARTESIAN_POINT('Ctrl Pts',(2.50410331873176,0.666666666666667,2.79140942341258));
#38132=CARTESIAN_POINT('Ctrl Pts',(2.50410331873176,1.,2.79140942341258));
#38133=CARTESIAN_POINT('',(2.91557726271063,1.,3.02314558451372));
#38134=CARTESIAN_POINT('',(2.91557726271063,0.,3.02314558451372));
#38135=CARTESIAN_POINT('Ctrl Pts',(2.50410331873176,1.,2.79140942341258));
#38136=CARTESIAN_POINT('Ctrl Pts',(2.50410700351493,1.,2.79145823440781));
#38137=CARTESIAN_POINT('Ctrl Pts',(2.50417932839313,1.,2.79164172518905));
#38138=CARTESIAN_POINT('Ctrl Pts',(2.50455968395146,1.,2.79217568804755));
#38139=CARTESIAN_POINT('Ctrl Pts',(2.50567182569081,1.,2.79344192164147));
#38140=CARTESIAN_POINT('Ctrl Pts',(2.5081055597767,1.,2.79596878057287));
#38141=CARTESIAN_POINT('Ctrl Pts',(2.51186983687818,1.,2.79970585014168));
#38142=CARTESIAN_POINT('Ctrl Pts',(2.51660190465805,1.,2.80427363984653));
#38143=CARTESIAN_POINT('Ctrl Pts',(2.52205778589653,1.,2.80941521966941));
#38144=CARTESIAN_POINT('Ctrl Pts',(2.52796388055278,1.,2.81484379048475));
#38145=CARTESIAN_POINT('Ctrl Pts',(2.53405679667412,1.,2.82028550483689));
#38146=CARTESIAN_POINT('Ctrl Pts',(2.54012272520199,1.,2.8255216764922));
#38147=CARTESIAN_POINT('Ctrl Pts',(2.54604736792655,1.,2.83044254225917));
#38148=CARTESIAN_POINT('Ctrl Pts',(2.55182152807077,1.,2.83505269592536));
#38149=CARTESIAN_POINT('Ctrl Pts',(2.55749952145241,1.,2.83942515220782));
#38150=CARTESIAN_POINT('Ctrl Pts',(2.56316920798513,1.,2.84366802680237));
#38151=CARTESIAN_POINT('Ctrl Pts',(2.56891984251721,1.,2.84788893329067));
#38152=CARTESIAN_POINT('Ctrl Pts',(2.57480482727081,1.,2.85215360144431));
#38153=CARTESIAN_POINT('Ctrl Pts',(2.58082875254357,1.,2.85647171715092));
#38154=CARTESIAN_POINT('Ctrl Pts',(2.58696770643524,1.,2.86081999003629));
#38155=CARTESIAN_POINT('Ctrl Pts',(2.59318160184908,1.,2.86515629953513));
#38156=CARTESIAN_POINT('Ctrl Pts',(2.5994287522321,1.,2.86943633170722));
#38157=CARTESIAN_POINT('Ctrl Pts',(2.60568177881303,1.,2.87363176656501));
#38158=CARTESIAN_POINT('Ctrl Pts',(2.61193507170955,1.,2.87773881947916));
#38159=CARTESIAN_POINT('Ctrl Pts',(2.61819596473108,1.,2.88176821427525));
#38160=CARTESIAN_POINT('Ctrl Pts',(2.62447947640262,1.,2.88573922195059));
#38161=CARTESIAN_POINT('Ctrl Pts',(2.63080195420767,1.,2.88967244854239));
#38162=CARTESIAN_POINT('Ctrl Pts',(2.63717442263932,1.,2.89358228854544));
#38163=CARTESIAN_POINT('Ctrl Pts',(2.64359851684131,1.,2.89747231723345));
#38164=CARTESIAN_POINT('Ctrl Pts',(2.65007017365564,1.,2.90133950224867));
#38165=CARTESIAN_POINT('Ctrl Pts',(2.65658188464282,1.,2.90517678087461));
#38166=CARTESIAN_POINT('Ctrl Pts',(2.6631254261681,1.,2.90897617968923));
#38167=CARTESIAN_POINT('Ctrl Pts',(2.66969458792631,1.,2.91273193382882));
#38168=CARTESIAN_POINT('Ctrl Pts',(2.67628728855312,1.,2.91644290704285));
#38169=CARTESIAN_POINT('Ctrl Pts',(2.68290409279688,1.,2.92011090722152));
#38170=CARTESIAN_POINT('Ctrl Pts',(2.68954721165339,1.,2.92373955325875));
#38171=CARTESIAN_POINT('Ctrl Pts',(2.69621932864301,1.,2.92733294395267));
#38172=CARTESIAN_POINT('Ctrl Pts',(2.70292247416885,1.,2.9308943823375));
#38173=CARTESIAN_POINT('Ctrl Pts',(2.70965695523787,1.,2.93442516311179));
#38174=CARTESIAN_POINT('Ctrl Pts',(2.71642190053592,1.,2.93792519474972));
#38175=CARTESIAN_POINT('Ctrl Pts',(2.72321571511337,1.,2.94139351933897));
#38176=CARTESIAN_POINT('Ctrl Pts',(2.73003657371616,1.,2.94482887675143));
#38177=CARTESIAN_POINT('Ctrl Pts',(2.73688288329808,1.,2.94823023414364));
#38178=CARTESIAN_POINT('Ctrl Pts',(2.74375379492172,1.,2.95159737214266));
#38179=CARTESIAN_POINT('Ctrl Pts',(2.75064903318947,1.,2.95493069316161));
#38180=CARTESIAN_POINT('Ctrl Pts',(2.7575686788835,1.,2.95823097665896));
#38181=CARTESIAN_POINT('Ctrl Pts',(2.76451296269557,1.,2.96149914764818));
#38182=CARTESIAN_POINT('Ctrl Pts',(2.77148206836498,1.,2.96473605585583));
#38183=CARTESIAN_POINT('Ctrl Pts',(2.7784758954285,1.,2.96794221043036));
#38184=CARTESIAN_POINT('Ctrl Pts',(2.78549409123769,1.,2.97111781461465));
#38185=CARTESIAN_POINT('Ctrl Pts',(2.79253615718248,1.,2.9742628834758));
#38186=CARTESIAN_POINT('Ctrl Pts',(2.7996015327823,1.,2.97737733718287));
#38187=CARTESIAN_POINT('Ctrl Pts',(2.80668968101106,1.,2.98046109647241));
#38188=CARTESIAN_POINT('Ctrl Pts',(2.81380019196286,1.,2.98351419779767));
#38189=CARTESIAN_POINT('Ctrl Pts',(2.82093279065457,1.,2.9865368066918));
#38190=CARTESIAN_POINT('Ctrl Pts',(2.82808728190157,1.,2.98952916401446));
#38191=CARTESIAN_POINT('Ctrl Pts',(2.83526351254248,1.,2.9924915517034));
#38192=CARTESIAN_POINT('Ctrl Pts',(2.84246132984415,1.,2.99542425341685));
#38193=CARTESIAN_POINT('Ctrl Pts',(2.84968053289451,1.,2.99832751144925));
#38194=CARTESIAN_POINT('Ctrl Pts',(2.85692085715685,1.,3.00120150796095));
#38195=CARTESIAN_POINT('Ctrl Pts',(2.86418200833667,1.,3.00404638316867));
#38196=CARTESIAN_POINT('Ctrl Pts',(2.87146368430501,1.,3.00686224485784));
#38197=CARTESIAN_POINT('Ctrl Pts',(2.87876560072727,1.,3.00964918108476));
#38198=CARTESIAN_POINT('Ctrl Pts',(2.8860875170608,1.,3.01240727308829));
#38199=CARTESIAN_POINT('Ctrl Pts',(2.89342925566321,1.,3.01513660431928));
#38200=CARTESIAN_POINT('Ctrl Pts',(2.9007906910105,1.,3.01783725121981));
#38201=CARTESIAN_POINT('Ctrl Pts',(2.90669553302526,1.,3.01997487193503));
#38202=CARTESIAN_POINT('Ctrl Pts',(2.91113297348212,1.,3.02156522742431));
#38203=CARTESIAN_POINT('Ctrl Pts',(2.91409518070399,1.,3.02261975104593));
#38204=CARTESIAN_POINT('Ctrl Pts',(2.91557726271063,1.,3.02314558451372));
#38205=CARTESIAN_POINT('Origin',(2.91557726271063,0.,3.02314558451372));
#38206=CARTESIAN_POINT('',(3.02314558451372,1.,2.91557726271063));
#38207=CARTESIAN_POINT('Origin',(0.,0.,0.));
#38208=CARTESIAN_POINT('',(2.36531447826213,1.,2.90994629141562));
#38209=CARTESIAN_POINT('Origin',(0.,1.,0.));
#38210=CARTESIAN_POINT('Ctrl Pts',(2.36531447826213,1.,2.90994629141563));
#38211=CARTESIAN_POINT('Ctrl Pts',(2.36531447826213,0.666666666666667,2.90994629141563));
#38212=CARTESIAN_POINT('Ctrl Pts',(2.36531447826213,0.333333333333333,2.90994629141563));
#38213=CARTESIAN_POINT('Ctrl Pts',(2.36531447826213,-0.333333333333333,
2.90994629141563));
#38214=CARTESIAN_POINT('Ctrl Pts',(2.36531447826213,-0.666666666666667,
2.90994629141563));
#38215=CARTESIAN_POINT('Ctrl Pts',(2.36531447826213,-1.,2.90994629141563));
#38216=CARTESIAN_POINT('Ctrl Pts',(2.52982887637028,-1.,3.35260583073571));
#38217=CARTESIAN_POINT('Ctrl Pts',(2.52982887637028,1.,3.35260583073571));
#38218=CARTESIAN_POINT('Ctrl Pts',(2.52954136549357,-1.,3.35105973714426));
#38219=CARTESIAN_POINT('Ctrl Pts',(2.52954136549357,1.,3.35105973714426));
#38220=CARTESIAN_POINT('Ctrl Pts',(2.5289632161143,-1.,3.34796903577628));
#38221=CARTESIAN_POINT('Ctrl Pts',(2.5289632161143,1.,3.34796903577628));
#38222=CARTESIAN_POINT('Ctrl Pts',(2.52808660916879,-1.,3.34333744117093));
#38223=CARTESIAN_POINT('Ctrl Pts',(2.52808660916879,1.,3.34333744117093));
#38224=CARTESIAN_POINT('Ctrl Pts',(2.52689902691551,-1.,3.33717090000955));
#38225=CARTESIAN_POINT('Ctrl Pts',(2.52689902691551,1.,3.33717090000955));
#38226=CARTESIAN_POINT('Ctrl Pts',(2.52538321165774,-1.,3.32947762189049));
#38227=CARTESIAN_POINT('Ctrl Pts',(2.52538321165774,1.,3.32947762189049));
#38228=CARTESIAN_POINT('Ctrl Pts',(2.52383598396878,-1.,3.32179931079521));
#38229=CARTESIAN_POINT('Ctrl Pts',(2.52383598396878,1.,3.32179931079521));
#38230=CARTESIAN_POINT('Ctrl Pts',(2.52225724871375,-1.,3.31413607874727));
#38231=CARTESIAN_POINT('Ctrl Pts',(2.52225724871375,1.,3.31413607874727));
#38232=CARTESIAN_POINT('Ctrl Pts',(2.52064689568167,-1.,3.30648808814986));
#38233=CARTESIAN_POINT('Ctrl Pts',(2.52064689568167,1.,3.30648808814986));
#38234=CARTESIAN_POINT('Ctrl Pts',(2.51900480700548,-1.,3.29885556387661));
#38235=CARTESIAN_POINT('Ctrl Pts',(2.51900480700548,1.,3.29885556387661));
#38236=CARTESIAN_POINT('Ctrl Pts',(2.51733085123316,-1.,3.2912387729863));
#38237=CARTESIAN_POINT('Ctrl Pts',(2.51733085123316,1.,3.2912387729863));
#38238=CARTESIAN_POINT('Ctrl Pts',(2.51562487464214,-1.,3.28363799702583));
#38239=CARTESIAN_POINT('Ctrl Pts',(2.51562487464214,1.,3.28363799702583));
#38240=CARTESIAN_POINT('Ctrl Pts',(2.51388669270329,-1.,3.27605350473048));
#38241=CARTESIAN_POINT('Ctrl Pts',(2.51388669270329,1.,3.27605350473048));
#38242=CARTESIAN_POINT('Ctrl Pts',(2.51211608411539,-1.,3.26848552888271));
#38243=CARTESIAN_POINT('Ctrl Pts',(2.51211608411539,1.,3.26848552888271));
#38244=CARTESIAN_POINT('Ctrl Pts',(2.51031277813697,-1.,3.26093423001716));
#38245=CARTESIAN_POINT('Ctrl Pts',(2.51031277813697,1.,3.26093423001716));
#38246=CARTESIAN_POINT('Ctrl Pts',(2.50847647070936,-1.,3.25339971461265));
#38247=CARTESIAN_POINT('Ctrl Pts',(2.50847647070936,1.,3.25339971461265));
#38248=CARTESIAN_POINT('Ctrl Pts',(2.50660685940645,-1.,3.24588208984042));
#38249=CARTESIAN_POINT('Ctrl Pts',(2.50660685940645,1.,3.24588208984042));
#38250=CARTESIAN_POINT('Ctrl Pts',(2.50470367580078,-1.,3.23838151080383));
#38251=CARTESIAN_POINT('Ctrl Pts',(2.50470367580078,1.,3.23838151080383));
#38252=CARTESIAN_POINT('Ctrl Pts',(2.50276671338074,-1.,3.23089822320596));
#38253=CARTESIAN_POINT('Ctrl Pts',(2.50276671338074,1.,3.23089822320596));
#38254=CARTESIAN_POINT('Ctrl Pts',(2.5007958720187,-1.,3.22343262620387));
#38255=CARTESIAN_POINT('Ctrl Pts',(2.5007958720187,1.,3.22343262620387));
#38256=CARTESIAN_POINT('Ctrl Pts',(2.49879114599293,-1.,3.21598526261157));
#38257=CARTESIAN_POINT('Ctrl Pts',(2.49879114599293,1.,3.21598526261157));
#38258=CARTESIAN_POINT('Ctrl Pts',(2.49675252647298,-1.,3.2085566984974));
#38259=CARTESIAN_POINT('Ctrl Pts',(2.49675252647298,1.,3.2085566984974));
#38260=CARTESIAN_POINT('Ctrl Pts',(2.49467992057726,-1.,3.20114742397549));
#38261=CARTESIAN_POINT('Ctrl Pts',(2.49467992057726,1.,3.20114742397549));
#38262=CARTESIAN_POINT('Ctrl Pts',(2.4925730723986,-1.,3.19375775555814));
#38263=CARTESIAN_POINT('Ctrl Pts',(2.4925730723986,1.,3.19375775555814));
#38264=CARTESIAN_POINT('Ctrl Pts',(2.49043146334095,-1.,3.18638771282315));
#38265=CARTESIAN_POINT('Ctrl Pts',(2.49043146334095,1.,3.18638771282315));
#38266=CARTESIAN_POINT('Ctrl Pts',(2.48825428288242,-1.,3.17903698136679));
#38267=CARTESIAN_POINT('Ctrl Pts',(2.48825428288242,1.,3.17903698136679));
#38268=CARTESIAN_POINT('Ctrl Pts',(2.48604065348619,-1.,3.17170518863357));
#38269=CARTESIAN_POINT('Ctrl Pts',(2.48604065348619,1.,3.17170518863357));
#38270=CARTESIAN_POINT('Ctrl Pts',(2.48378981792739,-1.,3.16439213290181));
#38271=CARTESIAN_POINT('Ctrl Pts',(2.48378981792739,1.,3.16439213290181));
#38272=CARTESIAN_POINT('Ctrl Pts',(2.48150133566568,-1.,3.15709802322735));
#38273=CARTESIAN_POINT('Ctrl Pts',(2.48150133566568,1.,3.15709802322735));
#38274=CARTESIAN_POINT('Ctrl Pts',(2.47917529057016,-1.,3.14982373241335));
#38275=CARTESIAN_POINT('Ctrl Pts',(2.47917529057016,1.,3.14982373241335));
#38276=CARTESIAN_POINT('Ctrl Pts',(2.47681245356095,-1.,3.14257099546531));
#38277=CARTESIAN_POINT('Ctrl Pts',(2.47681245356095,1.,3.14257099546531));
#38278=CARTESIAN_POINT('Ctrl Pts',(2.47441378371923,-1.,3.13534181229282));
#38279=CARTESIAN_POINT('Ctrl Pts',(2.47441378371923,1.,3.13534181229282));
#38280=CARTESIAN_POINT('Ctrl Pts',(2.47197997765868,-1.,3.12813790805948));
#38281=CARTESIAN_POINT('Ctrl Pts',(2.47197997765868,1.,3.12813790805948));
#38282=CARTESIAN_POINT('Ctrl Pts',(2.4695109894747,-1.,3.12096015766984));
#38283=CARTESIAN_POINT('Ctrl Pts',(2.4695109894747,1.,3.12096015766984));
#38284=CARTESIAN_POINT('Ctrl Pts',(2.46700558843507,-1.,3.11380805536124));
#38285=CARTESIAN_POINT('Ctrl Pts',(2.46700558843507,1.,3.11380805536124));
#38286=CARTESIAN_POINT('Ctrl Pts',(2.46446082979645,-1.,3.10667907901981));
#38287=CARTESIAN_POINT('Ctrl Pts',(2.46446082979645,1.,3.10667907901981));
#38288=CARTESIAN_POINT('Ctrl Pts',(2.4618730850188,-1.,3.09956993697048));
#38289=CARTESIAN_POINT('Ctrl Pts',(2.4618730850188,1.,3.09956993697048));
#38290=CARTESIAN_POINT('Ctrl Pts',(2.45923912563875,-1.,3.09247787931881));
#38291=CARTESIAN_POINT('Ctrl Pts',(2.45923912563875,1.,3.09247787931881));
#38292=CARTESIAN_POINT('Ctrl Pts',(2.45655725437037,-1.,3.08540206545313));
#38293=CARTESIAN_POINT('Ctrl Pts',(2.45655725437037,1.,3.08540206545313));
#38294=CARTESIAN_POINT('Ctrl Pts',(2.45382826787795,-1.,3.07834472886145));
#38295=CARTESIAN_POINT('Ctrl Pts',(2.45382826787795,1.,3.07834472886145));
#38296=CARTESIAN_POINT('Ctrl Pts',(2.45105688854432,-1.,3.0713129052131));
#38297=CARTESIAN_POINT('Ctrl Pts',(2.45105688854432,1.,3.0713129052131));
#38298=CARTESIAN_POINT('Ctrl Pts',(2.44824970516557,-1.,3.06431596421422));
#38299=CARTESIAN_POINT('Ctrl Pts',(2.44824970516557,1.,3.06431596421422));
#38300=CARTESIAN_POINT('Ctrl Pts',(2.44541251892568,-1.,3.05736242671521));
#38301=CARTESIAN_POINT('Ctrl Pts',(2.44541251892568,1.,3.05736242671521));
#38302=CARTESIAN_POINT('Ctrl Pts',(2.44254768923109,-1.,3.05045678021509));
#38303=CARTESIAN_POINT('Ctrl Pts',(2.44254768923109,1.,3.05045678021509));
#38304=CARTESIAN_POINT('Ctrl Pts',(2.43965194061849,-1.,3.04359685040545));
#38305=CARTESIAN_POINT('Ctrl Pts',(2.43965194061849,1.,3.04359685040545));
#38306=CARTESIAN_POINT('Ctrl Pts',(2.43671278042394,-1.,3.03676949672797));
#38307=CARTESIAN_POINT('Ctrl Pts',(2.43671278042394,1.,3.03676949672797));
#38308=CARTESIAN_POINT('Ctrl Pts',(2.43371241361462,-1.,3.02995534946946));
#38309=CARTESIAN_POINT('Ctrl Pts',(2.43371241361462,1.,3.02995534946946));
#38310=CARTESIAN_POINT('Ctrl Pts',(2.43063415586615,-1.,3.02313656035977));
#38311=CARTESIAN_POINT('Ctrl Pts',(2.43063415586615,1.,3.02313656035977));
#38312=CARTESIAN_POINT('Ctrl Pts',(2.4274685626416,-1.,3.01630420830494));
#38313=CARTESIAN_POINT('Ctrl Pts',(2.4274685626416,1.,3.01630420830494));
#38314=CARTESIAN_POINT('Ctrl Pts',(2.42421849439625,-1.,3.00946442616674));
#38315=CARTESIAN_POINT('Ctrl Pts',(2.42421849439625,1.,3.00946442616674));
#38316=CARTESIAN_POINT('Ctrl Pts',(2.42090763946812,-1.,3.00264868586038));
#38317=CARTESIAN_POINT('Ctrl Pts',(2.42090763946812,1.,3.00264868586038));
#38318=CARTESIAN_POINT('Ctrl Pts',(2.4175732450056,-1.,2.99590509293561));
#38319=CARTESIAN_POINT('Ctrl Pts',(2.4175732450056,1.,2.99590509293561));
#38320=CARTESIAN_POINT('Ctrl Pts',(2.4142506419963,-1.,2.98927983005851));
#38321=CARTESIAN_POINT('Ctrl Pts',(2.4142506419963,1.,2.98927983005851));
#38322=CARTESIAN_POINT('Ctrl Pts',(2.41095909342591,-1.,2.98280015815132));
#38323=CARTESIAN_POINT('Ctrl Pts',(2.41095909342591,1.,2.98280015815132));
#38324=CARTESIAN_POINT('Ctrl Pts',(2.40768975073691,-1.,2.97646002822395));
#38325=CARTESIAN_POINT('Ctrl Pts',(2.40768975073691,1.,2.97646002822395));
#38326=CARTESIAN_POINT('Ctrl Pts',(2.40438604734848,-1.,2.97019641312272));
#38327=CARTESIAN_POINT('Ctrl Pts',(2.40438604734848,1.,2.97019641312272));
#38328=CARTESIAN_POINT('Ctrl Pts',(2.40095565711535,-1.,2.96390432240181));
#38329=CARTESIAN_POINT('Ctrl Pts',(2.40095565711535,1.,2.96390432240181));
#38330=CARTESIAN_POINT('Ctrl Pts',(2.39730553974412,-1.,2.95748006482811));
#38331=CARTESIAN_POINT('Ctrl Pts',(2.39730553974412,1.,2.95748006482811));
#38332=CARTESIAN_POINT('Ctrl Pts',(2.39337207631613,-1.,2.95085857128372));
#38333=CARTESIAN_POINT('Ctrl Pts',(2.39337207631613,1.,2.95085857128372));
#38334=CARTESIAN_POINT('Ctrl Pts',(2.38914929090806,-1.,2.94404820669135));
#38335=CARTESIAN_POINT('Ctrl Pts',(2.38914929090806,1.,2.94404820669135));
#38336=CARTESIAN_POINT('Ctrl Pts',(2.38472771516476,-1.,2.93717903280599));
#38337=CARTESIAN_POINT('Ctrl Pts',(2.38472771516476,1.,2.93717903280599));
#38338=CARTESIAN_POINT('Ctrl Pts',(2.3802898958232,-1.,2.93049643640517));
#38339=CARTESIAN_POINT('Ctrl Pts',(2.3802898958232,1.,2.93049643640517));
#38340=CARTESIAN_POINT('Ctrl Pts',(2.37606510524271,-1.,2.92430340582912));
#38341=CARTESIAN_POINT('Ctrl Pts',(2.37606510524271,1.,2.92430340582912));
#38342=CARTESIAN_POINT('Ctrl Pts',(2.37229381109939,-1.,2.9189150379156));
#38343=CARTESIAN_POINT('Ctrl Pts',(2.37229381109939,1.,2.9189150379156));
#38344=CARTESIAN_POINT('Ctrl Pts',(2.36919161373074,-1.,2.91461249883016));
#38345=CARTESIAN_POINT('Ctrl Pts',(2.36919161373074,1.,2.91461249883016));
#38346=CARTESIAN_POINT('Ctrl Pts',(2.36690501170317,-1.,2.9115863784165));
#38347=CARTESIAN_POINT('Ctrl Pts',(2.36690501170317,1.,2.9115863784165));
#38348=CARTESIAN_POINT('Ctrl Pts',(2.36578327194396,-1.,2.91025813829606));
#38349=CARTESIAN_POINT('Ctrl Pts',(2.36578327194396,1.,2.91025813829606));
#38350=CARTESIAN_POINT('Ctrl Pts',(2.36535052956704,-1.,2.90989022547738));
#38351=CARTESIAN_POINT('Ctrl Pts',(2.36535052956704,1.,2.90989022547738));
#38352=CARTESIAN_POINT('Ctrl Pts',(2.36524348105023,-1.,2.90992398626098));
#38353=CARTESIAN_POINT('Ctrl Pts',(2.36524348105023,1.,2.90992398626098));
#38354=CARTESIAN_POINT('Ctrl Pts',(2.36523532225181,-1.,2.91001063062876));
#38355=CARTESIAN_POINT('Ctrl Pts',(2.36523532225181,1.,2.91001063062876));
#38356=CARTESIAN_POINT('',(2.52982887637028,1.,3.35260583073571));
#38357=CARTESIAN_POINT('Ctrl Pts',(2.52982887637028,1.,3.35260583073571));
#38358=CARTESIAN_POINT('Ctrl Pts',(2.52954136549357,1.,3.35105973714426));
#38359=CARTESIAN_POINT('Ctrl Pts',(2.5289632161143,1.,3.34796903577628));
#38360=CARTESIAN_POINT('Ctrl Pts',(2.52808660916879,1.,3.34333744117093));
#38361=CARTESIAN_POINT('Ctrl Pts',(2.52689902691551,1.,3.33717090000955));
#38362=CARTESIAN_POINT('Ctrl Pts',(2.52538321165774,1.,3.32947762189049));
#38363=CARTESIAN_POINT('Ctrl Pts',(2.52383598396878,1.,3.32179931079521));
#38364=CARTESIAN_POINT('Ctrl Pts',(2.52225724871375,1.,3.31413607874727));
#38365=CARTESIAN_POINT('Ctrl Pts',(2.52064689568167,1.,3.30648808814986));
#38366=CARTESIAN_POINT('Ctrl Pts',(2.51900480700548,1.,3.29885556387661));
#38367=CARTESIAN_POINT('Ctrl Pts',(2.51733085123316,1.,3.2912387729863));
#38368=CARTESIAN_POINT('Ctrl Pts',(2.51562487464214,1.,3.28363799702583));
#38369=CARTESIAN_POINT('Ctrl Pts',(2.51388669270329,1.,3.27605350473048));
#38370=CARTESIAN_POINT('Ctrl Pts',(2.51211608411539,1.,3.26848552888271));
#38371=CARTESIAN_POINT('Ctrl Pts',(2.51031277813697,1.,3.26093423001716));
#38372=CARTESIAN_POINT('Ctrl Pts',(2.50847647070936,1.,3.25339971461265));
#38373=CARTESIAN_POINT('Ctrl Pts',(2.50660685940645,1.,3.24588208984042));
#38374=CARTESIAN_POINT('Ctrl Pts',(2.50470367580078,1.,3.23838151080383));
#38375=CARTESIAN_POINT('Ctrl Pts',(2.50276671338074,1.,3.23089822320596));
#38376=CARTESIAN_POINT('Ctrl Pts',(2.5007958720187,1.,3.22343262620387));
#38377=CARTESIAN_POINT('Ctrl Pts',(2.49879114599293,1.,3.21598526261157));
#38378=CARTESIAN_POINT('Ctrl Pts',(2.49675252647298,1.,3.2085566984974));
#38379=CARTESIAN_POINT('Ctrl Pts',(2.49467992057726,1.,3.20114742397549));
#38380=CARTESIAN_POINT('Ctrl Pts',(2.4925730723986,1.,3.19375775555814));
#38381=CARTESIAN_POINT('Ctrl Pts',(2.49043146334095,1.,3.18638771282315));
#38382=CARTESIAN_POINT('Ctrl Pts',(2.48825428288242,1.,3.17903698136679));
#38383=CARTESIAN_POINT('Ctrl Pts',(2.48604065348619,1.,3.17170518863357));
#38384=CARTESIAN_POINT('Ctrl Pts',(2.48378981792739,1.,3.16439213290181));
#38385=CARTESIAN_POINT('Ctrl Pts',(2.48150133566568,1.,3.15709802322735));
#38386=CARTESIAN_POINT('Ctrl Pts',(2.47917529057016,1.,3.14982373241335));
#38387=CARTESIAN_POINT('Ctrl Pts',(2.47681245356095,1.,3.14257099546531));
#38388=CARTESIAN_POINT('Ctrl Pts',(2.47441378371923,1.,3.13534181229282));
#38389=CARTESIAN_POINT('Ctrl Pts',(2.47197997765868,1.,3.12813790805948));
#38390=CARTESIAN_POINT('Ctrl Pts',(2.4695109894747,1.,3.12096015766984));
#38391=CARTESIAN_POINT('Ctrl Pts',(2.46700558843507,1.,3.11380805536124));
#38392=CARTESIAN_POINT('Ctrl Pts',(2.46446082979645,1.,3.10667907901981));
#38393=CARTESIAN_POINT('Ctrl Pts',(2.4618730850188,1.,3.09956993697048));
#38394=CARTESIAN_POINT('Ctrl Pts',(2.45923912563875,1.,3.09247787931881));
#38395=CARTESIAN_POINT('Ctrl Pts',(2.45655725437037,1.,3.08540206545313));
#38396=CARTESIAN_POINT('Ctrl Pts',(2.45382826787795,1.,3.07834472886145));
#38397=CARTESIAN_POINT('Ctrl Pts',(2.45105688854432,1.,3.0713129052131));
#38398=CARTESIAN_POINT('Ctrl Pts',(2.44824970516557,1.,3.06431596421422));
#38399=CARTESIAN_POINT('Ctrl Pts',(2.44541251892568,1.,3.05736242671521));
#38400=CARTESIAN_POINT('Ctrl Pts',(2.44254768923109,1.,3.05045678021509));
#38401=CARTESIAN_POINT('Ctrl Pts',(2.43965194061849,1.,3.04359685040545));
#38402=CARTESIAN_POINT('Ctrl Pts',(2.43671278042394,1.,3.03676949672797));
#38403=CARTESIAN_POINT('Ctrl Pts',(2.43371241361462,1.,3.02995534946946));
#38404=CARTESIAN_POINT('Ctrl Pts',(2.43063415586615,1.,3.02313656035977));
#38405=CARTESIAN_POINT('Ctrl Pts',(2.4274685626416,1.,3.01630420830494));
#38406=CARTESIAN_POINT('Ctrl Pts',(2.42421849439625,1.,3.00946442616674));
#38407=CARTESIAN_POINT('Ctrl Pts',(2.42090763946812,1.,3.00264868586038));
#38408=CARTESIAN_POINT('Ctrl Pts',(2.4175732450056,1.,2.99590509293561));
#38409=CARTESIAN_POINT('Ctrl Pts',(2.4142506419963,1.,2.98927983005851));
#38410=CARTESIAN_POINT('Ctrl Pts',(2.41095909342591,1.,2.98280015815132));
#38411=CARTESIAN_POINT('Ctrl Pts',(2.40768975073691,1.,2.97646002822395));
#38412=CARTESIAN_POINT('Ctrl Pts',(2.40438604734848,1.,2.97019641312272));
#38413=CARTESIAN_POINT('Ctrl Pts',(2.40095565711535,1.,2.96390432240181));
#38414=CARTESIAN_POINT('Ctrl Pts',(2.39730553974412,1.,2.95748006482811));
#38415=CARTESIAN_POINT('Ctrl Pts',(2.39337207631613,1.,2.95085857128372));
#38416=CARTESIAN_POINT('Ctrl Pts',(2.38914929090806,1.,2.94404820669135));
#38417=CARTESIAN_POINT('Ctrl Pts',(2.38472771516476,1.,2.93717903280599));
#38418=CARTESIAN_POINT('Ctrl Pts',(2.3802898958232,1.,2.93049643640517));
#38419=CARTESIAN_POINT('Ctrl Pts',(2.37606510524271,1.,2.92430340582912));
#38420=CARTESIAN_POINT('Ctrl Pts',(2.37229381109939,1.,2.9189150379156));
#38421=CARTESIAN_POINT('Ctrl Pts',(2.36919161373074,1.,2.91461249883016));
#38422=CARTESIAN_POINT('Ctrl Pts',(2.36707658451709,1.,2.91181344022628));
#38423=CARTESIAN_POINT('Ctrl Pts',(2.36599991765853,1.,2.91051690822262));
#38424=CARTESIAN_POINT('Ctrl Pts',(2.36553202948741,1.,2.91005770527771));
#38425=CARTESIAN_POINT('Ctrl Pts',(2.3653621118858,1.,2.90995756655559));
#38426=CARTESIAN_POINT('Ctrl Pts',(2.36531447826213,1.,2.90994629141563));
#38427=CARTESIAN_POINT('',(2.52982887637028,0.,3.35260583073571));
#38428=CARTESIAN_POINT('Ctrl Pts',(2.03668666247593,-1.,3.1487152044751));
#38429=CARTESIAN_POINT('Ctrl Pts',(2.03668666247593,1.,3.1487152044751));
#38430=CARTESIAN_POINT('Ctrl Pts',(2.03660173757879,-1.,3.14869618937258));
#38431=CARTESIAN_POINT('Ctrl Pts',(2.03660173757879,1.,3.14869618937258));
#38432=CARTESIAN_POINT('Ctrl Pts',(2.03653654935591,-1.,3.14878756590812));
#38433=CARTESIAN_POINT('Ctrl Pts',(2.03653654935591,1.,3.14878756590812));
#38434=CARTESIAN_POINT('Ctrl Pts',(2.03675273049189,-1.,3.14931281968048));
#38435=CARTESIAN_POINT('Ctrl Pts',(2.03675273049189,1.,3.14931281968048));
#38436=CARTESIAN_POINT('Ctrl Pts',(2.03766932526445,-1.,3.15079010635742));
#38437=CARTESIAN_POINT('Ctrl Pts',(2.03766932526445,1.,3.15079010635742));
#38438=CARTESIAN_POINT('Ctrl Pts',(2.03984073791519,-1.,3.15389991674792));
#38439=CARTESIAN_POINT('Ctrl Pts',(2.03984073791519,1.,3.15389991674792));
#38440=CARTESIAN_POINT('Ctrl Pts',(2.04297406404027,-1.,3.15817983946367));
#38441=CARTESIAN_POINT('Ctrl Pts',(2.04297406404027,1.,3.15817983946367));
#38442=CARTESIAN_POINT('Ctrl Pts',(2.04693331247446,-1.,3.16343165058912));
#38443=CARTESIAN_POINT('Ctrl Pts',(2.04693331247446,1.,3.16343165058912));
#38444=CARTESIAN_POINT('Ctrl Pts',(2.05151770247233,-1.,3.16936341689527));
#38445=CARTESIAN_POINT('Ctrl Pts',(2.05151770247233,1.,3.16936341689527));
#38446=CARTESIAN_POINT('Ctrl Pts',(2.05650186773132,-1.,3.17564906975371));
#38447=CARTESIAN_POINT('Ctrl Pts',(2.05650186773132,1.,3.17564906975371));
#38448=CARTESIAN_POINT('Ctrl Pts',(2.06166849827101,-1.,3.18197692964614));
#38449=CARTESIAN_POINT('Ctrl Pts',(2.06166849827101,1.,3.18197692964614));
#38450=CARTESIAN_POINT('Ctrl Pts',(2.06684062744112,-1.,3.18809755562368));
#38451=CARTESIAN_POINT('Ctrl Pts',(2.06684062744112,1.,3.18809755562368));
#38452=CARTESIAN_POINT('Ctrl Pts',(2.07192253497857,-1.,3.19388465568252));
#38453=CARTESIAN_POINT('Ctrl Pts',(2.07192253497857,1.,3.19388465568252));
#38454=CARTESIAN_POINT('Ctrl Pts',(2.07690441870722,-1.,3.19934132836019));
#38455=CARTESIAN_POINT('Ctrl Pts',(2.07690441870722,1.,3.19934132836019));
#38456=CARTESIAN_POINT('Ctrl Pts',(2.08182850370878,-1.,3.2045481863073));
#38457=CARTESIAN_POINT('Ctrl Pts',(2.08182850370878,1.,3.2045481863073));
#38458=CARTESIAN_POINT('Ctrl Pts',(2.08676465517455,-1.,3.20962575845463));
#38459=CARTESIAN_POINT('Ctrl Pts',(2.08676465517455,1.,3.20962575845463));
#38460=CARTESIAN_POINT('Ctrl Pts',(2.09178419460443,-1.,3.21469429601654));
#38461=CARTESIAN_POINT('Ctrl Pts',(2.09178419460443,1.,3.21469429601654));
#38462=CARTESIAN_POINT('Ctrl Pts',(2.09692958434895,-1.,3.21982707347009));
#38463=CARTESIAN_POINT('Ctrl Pts',(2.09692958434895,1.,3.21982707347009));
#38464=CARTESIAN_POINT('Ctrl Pts',(2.10220384298492,-1.,3.22503437553434));
#38465=CARTESIAN_POINT('Ctrl Pts',(2.10220384298492,1.,3.22503437553434));
#38466=CARTESIAN_POINT('Ctrl Pts',(2.10758699642451,-1.,3.23028945793289));
#38467=CARTESIAN_POINT('Ctrl Pts',(2.10758699642451,1.,3.23028945793289));
#38468=CARTESIAN_POINT('Ctrl Pts',(2.11304604021773,-1.,3.23554444767099));
#38469=CARTESIAN_POINT('Ctrl Pts',(2.11304604021773,1.,3.23554444767099));
#38470=CARTESIAN_POINT('Ctrl Pts',(2.11854673326979,-1.,3.24074905517293));
#38471=CARTESIAN_POINT('Ctrl Pts',(2.11854673326979,1.,3.24074905517293));
#38472=CARTESIAN_POINT('Ctrl Pts',(2.12406646410962,-1.,3.24587102613376));
#38473=CARTESIAN_POINT('Ctrl Pts',(2.12406646410962,1.,3.24587102613376));
#38474=CARTESIAN_POINT('Ctrl Pts',(2.12960028396832,-1.,3.25090574494028));
#38475=CARTESIAN_POINT('Ctrl Pts',(2.12960028396832,1.,3.25090574494028));
#38476=CARTESIAN_POINT('Ctrl Pts',(2.13515375878803,-1.,3.25586495065054));
#38477=CARTESIAN_POINT('Ctrl Pts',(2.13515375878803,1.,3.25586495065054));
#38478=CARTESIAN_POINT('Ctrl Pts',(2.14073870754264,-1.,3.26077002641879));
#38479=CARTESIAN_POINT('Ctrl Pts',(2.14073870754264,1.,3.26077002641879));
#38480=CARTESIAN_POINT('Ctrl Pts',(2.1463680529566,-1.,3.26564388189759));
#38481=CARTESIAN_POINT('Ctrl Pts',(2.1463680529566,1.,3.26564388189759));
#38482=CARTESIAN_POINT('Ctrl Pts',(2.15205043199808,-1.,3.27050245897228));
#38483=CARTESIAN_POINT('Ctrl Pts',(2.15205043199808,1.,3.27050245897228));
#38484=CARTESIAN_POINT('Ctrl Pts',(2.15778690038347,-1.,3.27534954469187));
#38485=CARTESIAN_POINT('Ctrl Pts',(2.15778690038347,1.,3.27534954469187));
#38486=CARTESIAN_POINT('Ctrl Pts',(2.16357391934425,-1.,3.280181508414));
#38487=CARTESIAN_POINT('Ctrl Pts',(2.16357391934425,1.,3.280181508414));
#38488=CARTESIAN_POINT('Ctrl Pts',(2.16940517773455,-1.,3.28499019979724));
#38489=CARTESIAN_POINT('Ctrl Pts',(2.16940517773455,1.,3.28499019979724));
#38490=CARTESIAN_POINT('Ctrl Pts',(2.17527380048423,-1.,3.28976645712568));
#38491=CARTESIAN_POINT('Ctrl Pts',(2.17527380048423,1.,3.28976645712568));
#38492=CARTESIAN_POINT('Ctrl Pts',(2.18117455557065,-1.,3.2945036150049));
#38493=CARTESIAN_POINT('Ctrl Pts',(2.18117455557065,1.,3.2945036150049));
#38494=CARTESIAN_POINT('Ctrl Pts',(2.18710556500327,-1.,3.29920022557639));
#38495=CARTESIAN_POINT('Ctrl Pts',(2.18710556500327,1.,3.29920022557639));
#38496=CARTESIAN_POINT('Ctrl Pts',(2.19306710376111,-1.,3.30385816281831));
#38497=CARTESIAN_POINT('Ctrl Pts',(2.19306710376111,1.,3.30385816281831));
#38498=CARTESIAN_POINT('Ctrl Pts',(2.19906078949922,-1.,3.30848134694595));
#38499=CARTESIAN_POINT('Ctrl Pts',(2.19906078949922,1.,3.30848134694595));
#38500=CARTESIAN_POINT('Ctrl Pts',(2.20508863150607,-1.,3.31307424608949));
#38501=CARTESIAN_POINT('Ctrl Pts',(2.20508863150607,1.,3.31307424608949));
#38502=CARTESIAN_POINT('Ctrl Pts',(2.21115211847875,-1.,3.31764044024235));
#38503=CARTESIAN_POINT('Ctrl Pts',(2.21115211847875,1.,3.31764044024235));
#38504=CARTESIAN_POINT('Ctrl Pts',(2.21725135110898,-1.,3.32218125618968));
#38505=CARTESIAN_POINT('Ctrl Pts',(2.21725135110898,1.,3.32218125618968));
#38506=CARTESIAN_POINT('Ctrl Pts',(2.22338548312772,-1.,3.3266964672289));
#38507=CARTESIAN_POINT('Ctrl Pts',(2.22338548312772,1.,3.3266964672289));
#38508=CARTESIAN_POINT('Ctrl Pts',(2.22955308907233,-1.,3.33118487773611));
#38509=CARTESIAN_POINT('Ctrl Pts',(2.22955308907233,1.,3.33118487773611));
#38510=CARTESIAN_POINT('Ctrl Pts',(2.23575256328812,-1.,3.33564495756482));
#38511=CARTESIAN_POINT('Ctrl Pts',(2.23575256328812,1.,3.33564495756482));
#38512=CARTESIAN_POINT('Ctrl Pts',(2.24198249391422,-1.,3.34007543738025));
#38513=CARTESIAN_POINT('Ctrl Pts',(2.24198249391422,1.,3.34007543738025));
#38514=CARTESIAN_POINT('Ctrl Pts',(2.24824207678256,-1.,3.34447596770723));
#38515=CARTESIAN_POINT('Ctrl Pts',(2.24824207678256,1.,3.34447596770723));
#38516=CARTESIAN_POINT('Ctrl Pts',(2.25453097693483,-1.,3.34884690292285));
#38517=CARTESIAN_POINT('Ctrl Pts',(2.25453097693483,1.,3.34884690292285));
#38518=CARTESIAN_POINT('Ctrl Pts',(2.26084915222449,-1.,3.35318902552626));
#38519=CARTESIAN_POINT('Ctrl Pts',(2.26084915222449,1.,3.35318902552626));
#38520=CARTESIAN_POINT('Ctrl Pts',(2.26719668579909,-1.,3.35750328523061));
#38521=CARTESIAN_POINT('Ctrl Pts',(2.26719668579909,1.,3.35750328523061));
#38522=CARTESIAN_POINT('Ctrl Pts',(2.2735736262093,-1.,3.36179055004409));
#38523=CARTESIAN_POINT('Ctrl Pts',(2.2735736262093,1.,3.36179055004409));
#38524=CARTESIAN_POINT('Ctrl Pts',(2.27997979458037,-1.,3.36605130713076));
#38525=CARTESIAN_POINT('Ctrl Pts',(2.27997979458037,1.,3.36605130713076));
#38526=CARTESIAN_POINT('Ctrl Pts',(2.28641481081137,-1.,3.37028570206488));
#38527=CARTESIAN_POINT('Ctrl Pts',(2.28641481081137,1.,3.37028570206488));
#38528=CARTESIAN_POINT('Ctrl Pts',(2.29287818007393,-1.,3.37449367172826));
#38529=CARTESIAN_POINT('Ctrl Pts',(2.29287818007393,1.,3.37449367172826));
#38530=CARTESIAN_POINT('Ctrl Pts',(2.29936936127624,-1.,3.37867504959433));
#38531=CARTESIAN_POINT('Ctrl Pts',(2.29936936127624,1.,3.37867504959433));
#38532=CARTESIAN_POINT('Ctrl Pts',(2.30588783640343,-1.,3.3828296733661));
#38533=CARTESIAN_POINT('Ctrl Pts',(2.30588783640343,1.,3.3828296733661));
#38534=CARTESIAN_POINT('Ctrl Pts',(2.31243319489367,-1.,3.38695751492462));
#38535=CARTESIAN_POINT('Ctrl Pts',(2.31243319489367,1.,3.38695751492462));
#38536=CARTESIAN_POINT('Ctrl Pts',(2.31900513925424,-1.,3.39105869474822));
#38537=CARTESIAN_POINT('Ctrl Pts',(2.31900513925424,1.,3.39105869474822));
#38538=CARTESIAN_POINT('Ctrl Pts',(2.3256034390248,-1.,3.39513342019756));
#38539=CARTESIAN_POINT('Ctrl Pts',(2.3256034390248,1.,3.39513342019756));
#38540=CARTESIAN_POINT('Ctrl Pts',(2.33222789882489,-1.,3.39918194577956));
#38541=CARTESIAN_POINT('Ctrl Pts',(2.33222789882489,1.,3.39918194577956));
#38542=CARTESIAN_POINT('Ctrl Pts',(2.33887832342782,-1.,3.40320452776743));
#38543=CARTESIAN_POINT('Ctrl Pts',(2.33887832342782,1.,3.40320452776743));
#38544=CARTESIAN_POINT('Ctrl Pts',(2.34555447649188,-1.,3.40720137404297));
#38545=CARTESIAN_POINT('Ctrl Pts',(2.34555447649188,1.,3.40720137404297));
#38546=CARTESIAN_POINT('Ctrl Pts',(2.35225606824109,-1.,3.41117262314119));
#38547=CARTESIAN_POINT('Ctrl Pts',(2.35225606824109,1.,3.41117262314119));
#38548=CARTESIAN_POINT('Ctrl Pts',(2.35898278606946,-1.,3.41511836751469));
#38549=CARTESIAN_POINT('Ctrl Pts',(2.35898278606946,1.,3.41511836751469));
#38550=CARTESIAN_POINT('Ctrl Pts',(2.36573431470642,-1.,3.41903866635852));
#38551=CARTESIAN_POINT('Ctrl Pts',(2.36573431470642,1.,3.41903866635852));
#38552=CARTESIAN_POINT('Ctrl Pts',(2.37251035954292,-1.,3.42293356216511));
#38553=CARTESIAN_POINT('Ctrl Pts',(2.37251035954292,1.,3.42293356216511));
#38554=CARTESIAN_POINT('Ctrl Pts',(2.37931067028926,-1.,3.42680309754399));
#38555=CARTESIAN_POINT('Ctrl Pts',(2.37931067028926,1.,3.42680309754399));
#38556=CARTESIAN_POINT('Ctrl Pts',(2.38613505843552,-1.,3.4306473271292));
#38557=CARTESIAN_POINT('Ctrl Pts',(2.38613505843552,1.,3.4306473271292));
#38558=CARTESIAN_POINT('Ctrl Pts',(2.39298338804493,-1.,3.4344663067854));
#38559=CARTESIAN_POINT('Ctrl Pts',(2.39298338804493,1.,3.4344663067854));
#38560=CARTESIAN_POINT('Ctrl Pts',(2.39848113410292,-1.,3.43750133064416));
#38561=CARTESIAN_POINT('Ctrl Pts',(2.39848113410292,1.,3.43750133064416));
#38562=CARTESIAN_POINT('Ctrl Pts',(2.40261515589405,-1.,3.43976627484234));
#38563=CARTESIAN_POINT('Ctrl Pts',(2.40261515589405,1.,3.43976627484234));
#38564=CARTESIAN_POINT('Ctrl Pts',(2.4053759295909,-1.,3.44127120683039));
#38565=CARTESIAN_POINT('Ctrl Pts',(2.4053759295909,1.,3.44127120683039));
#38566=CARTESIAN_POINT('Ctrl Pts',(2.40675750623143,-1.,3.44202241512147));
#38567=CARTESIAN_POINT('Ctrl Pts',(2.40675750623143,1.,3.44202241512147));
#38568=CARTESIAN_POINT('',(2.03660101169714,1.,3.14877060440328));
#38569=CARTESIAN_POINT('Ctrl Pts',(2.03660101169714,-1.,3.14877060440327));
#38570=CARTESIAN_POINT('Ctrl Pts',(2.03660101169714,-0.666666666666667,
3.14877060440327));
#38571=CARTESIAN_POINT('Ctrl Pts',(2.03660101169714,-0.333333333333333,
3.14877060440327));
#38572=CARTESIAN_POINT('Ctrl Pts',(2.03660101169714,0.333333333333333,3.14877060440327));
#38573=CARTESIAN_POINT('Ctrl Pts',(2.03660101169714,0.666666666666667,3.14877060440327));
#38574=CARTESIAN_POINT('Ctrl Pts',(2.03660101169714,1.,3.14877060440327));
#38575=CARTESIAN_POINT('',(2.40675750623143,1.,3.44202241512147));
#38576=CARTESIAN_POINT('',(2.40675750623143,0.,3.44202241512147));
#38577=CARTESIAN_POINT('Ctrl Pts',(2.03660101169714,1.,3.14877060440328));
#38578=CARTESIAN_POINT('Ctrl Pts',(2.03659701539259,1.,3.14881939088124));
#38579=CARTESIAN_POINT('Ctrl Pts',(2.03663974554932,1.,3.1490119366901));
#38580=CARTESIAN_POINT('Ctrl Pts',(2.03693188810545,1.,3.14959882629805));
#38581=CARTESIAN_POINT('Ctrl Pts',(2.03783225495961,1.,3.15102344775328));
#38582=CARTESIAN_POINT('Ctrl Pts',(2.03984073791519,1.,3.15389991674792));
#38583=CARTESIAN_POINT('Ctrl Pts',(2.04297406404027,1.,3.15817983946367));
#38584=CARTESIAN_POINT('Ctrl Pts',(2.04693331247446,1.,3.16343165058912));
#38585=CARTESIAN_POINT('Ctrl Pts',(2.05151770247233,1.,3.16936341689527));
#38586=CARTESIAN_POINT('Ctrl Pts',(2.05650186773132,1.,3.17564906975371));
#38587=CARTESIAN_POINT('Ctrl Pts',(2.06166849827101,1.,3.18197692964614));
#38588=CARTESIAN_POINT('Ctrl Pts',(2.06684062744112,1.,3.18809755562368));
#38589=CARTESIAN_POINT('Ctrl Pts',(2.07192253497857,1.,3.19388465568252));
#38590=CARTESIAN_POINT('Ctrl Pts',(2.07690441870722,1.,3.19934132836019));
#38591=CARTESIAN_POINT('Ctrl Pts',(2.08182850370878,1.,3.2045481863073));
#38592=CARTESIAN_POINT('Ctrl Pts',(2.08676465517455,1.,3.20962575845463));
#38593=CARTESIAN_POINT('Ctrl Pts',(2.09178419460443,1.,3.21469429601654));
#38594=CARTESIAN_POINT('Ctrl Pts',(2.09692958434895,1.,3.21982707347009));
#38595=CARTESIAN_POINT('Ctrl Pts',(2.10220384298492,1.,3.22503437553434));
#38596=CARTESIAN_POINT('Ctrl Pts',(2.10758699642451,1.,3.23028945793289));
#38597=CARTESIAN_POINT('Ctrl Pts',(2.11304604021773,1.,3.23554444767099));
#38598=CARTESIAN_POINT('Ctrl Pts',(2.11854673326979,1.,3.24074905517293));
#38599=CARTESIAN_POINT('Ctrl Pts',(2.12406646410962,1.,3.24587102613376));
#38600=CARTESIAN_POINT('Ctrl Pts',(2.12960028396832,1.,3.25090574494028));
#38601=CARTESIAN_POINT('Ctrl Pts',(2.13515375878803,1.,3.25586495065054));
#38602=CARTESIAN_POINT('Ctrl Pts',(2.14073870754264,1.,3.26077002641879));
#38603=CARTESIAN_POINT('Ctrl Pts',(2.1463680529566,1.,3.26564388189759));
#38604=CARTESIAN_POINT('Ctrl Pts',(2.15205043199808,1.,3.27050245897228));
#38605=CARTESIAN_POINT('Ctrl Pts',(2.15778690038347,1.,3.27534954469187));
#38606=CARTESIAN_POINT('Ctrl Pts',(2.16357391934425,1.,3.280181508414));
#38607=CARTESIAN_POINT('Ctrl Pts',(2.16940517773455,1.,3.28499019979724));
#38608=CARTESIAN_POINT('Ctrl Pts',(2.17527380048423,1.,3.28976645712568));
#38609=CARTESIAN_POINT('Ctrl Pts',(2.18117455557065,1.,3.2945036150049));
#38610=CARTESIAN_POINT('Ctrl Pts',(2.18710556500327,1.,3.29920022557639));
#38611=CARTESIAN_POINT('Ctrl Pts',(2.19306710376111,1.,3.30385816281831));
#38612=CARTESIAN_POINT('Ctrl Pts',(2.19906078949922,1.,3.30848134694595));
#38613=CARTESIAN_POINT('Ctrl Pts',(2.20508863150607,1.,3.31307424608949));
#38614=CARTESIAN_POINT('Ctrl Pts',(2.21115211847875,1.,3.31764044024235));
#38615=CARTESIAN_POINT('Ctrl Pts',(2.21725135110898,1.,3.32218125618968));
#38616=CARTESIAN_POINT('Ctrl Pts',(2.22338548312772,1.,3.3266964672289));
#38617=CARTESIAN_POINT('Ctrl Pts',(2.22955308907233,1.,3.33118487773611));
#38618=CARTESIAN_POINT('Ctrl Pts',(2.23575256328812,1.,3.33564495756482));
#38619=CARTESIAN_POINT('Ctrl Pts',(2.24198249391422,1.,3.34007543738025));
#38620=CARTESIAN_POINT('Ctrl Pts',(2.24824207678256,1.,3.34447596770723));
#38621=CARTESIAN_POINT('Ctrl Pts',(2.25453097693483,1.,3.34884690292285));
#38622=CARTESIAN_POINT('Ctrl Pts',(2.26084915222449,1.,3.35318902552626));
#38623=CARTESIAN_POINT('Ctrl Pts',(2.26719668579909,1.,3.35750328523061));
#38624=CARTESIAN_POINT('Ctrl Pts',(2.2735736262093,1.,3.36179055004409));
#38625=CARTESIAN_POINT('Ctrl Pts',(2.27997979458037,1.,3.36605130713076));
#38626=CARTESIAN_POINT('Ctrl Pts',(2.28641481081137,1.,3.37028570206488));
#38627=CARTESIAN_POINT('Ctrl Pts',(2.29287818007393,1.,3.37449367172826));
#38628=CARTESIAN_POINT('Ctrl Pts',(2.29936936127624,1.,3.37867504959433));
#38629=CARTESIAN_POINT('Ctrl Pts',(2.30588783640343,1.,3.3828296733661));
#38630=CARTESIAN_POINT('Ctrl Pts',(2.31243319489367,1.,3.38695751492462));
#38631=CARTESIAN_POINT('Ctrl Pts',(2.31900513925424,1.,3.39105869474822));
#38632=CARTESIAN_POINT('Ctrl Pts',(2.3256034390248,1.,3.39513342019756));
#38633=CARTESIAN_POINT('Ctrl Pts',(2.33222789882489,1.,3.39918194577956));
#38634=CARTESIAN_POINT('Ctrl Pts',(2.33887832342782,1.,3.40320452776743));
#38635=CARTESIAN_POINT('Ctrl Pts',(2.34555447649188,1.,3.40720137404297));
#38636=CARTESIAN_POINT('Ctrl Pts',(2.35225606824109,1.,3.41117262314119));
#38637=CARTESIAN_POINT('Ctrl Pts',(2.35898278606946,1.,3.41511836751469));
#38638=CARTESIAN_POINT('Ctrl Pts',(2.36573431470642,1.,3.41903866635852));
#38639=CARTESIAN_POINT('Ctrl Pts',(2.37251035954292,1.,3.42293356216511));
#38640=CARTESIAN_POINT('Ctrl Pts',(2.37931067028926,1.,3.42680309754399));
#38641=CARTESIAN_POINT('Ctrl Pts',(2.38613505843552,1.,3.4306473271292));
#38642=CARTESIAN_POINT('Ctrl Pts',(2.39298338804493,1.,3.4344663067854));
#38643=CARTESIAN_POINT('Ctrl Pts',(2.39848113410292,1.,3.43750133064416));
#38644=CARTESIAN_POINT('Ctrl Pts',(2.40261515589405,1.,3.43976627484234));
#38645=CARTESIAN_POINT('Ctrl Pts',(2.4053759295909,1.,3.44127120683039));
#38646=CARTESIAN_POINT('Ctrl Pts',(2.40675750623143,1.,3.44202241512147));
#38647=CARTESIAN_POINT('Origin',(2.40675750623143,0.,3.44202241512147));
#38648=CARTESIAN_POINT('',(2.52982887637028,1.,3.35260583073571));
#38649=CARTESIAN_POINT('Origin',(0.,0.,0.));
#38650=CARTESIAN_POINT('',(1.88097764062697,1.,3.24413672884812));
#38651=CARTESIAN_POINT('Origin',(0.,1.,0.));
#38652=CARTESIAN_POINT('Ctrl Pts',(1.88097764062697,1.,3.24413672884812));
#38653=CARTESIAN_POINT('Ctrl Pts',(1.88097764062697,0.666666666666667,3.24413672884812));
#38654=CARTESIAN_POINT('Ctrl Pts',(1.88097764062697,0.333333333333333,3.24413672884812));
#38655=CARTESIAN_POINT('Ctrl Pts',(1.88097764062697,-0.333333333333333,
3.24413672884812));
#38656=CARTESIAN_POINT('Ctrl Pts',(1.88097764062697,-0.666666666666667,
3.24413672884812));
#38657=CARTESIAN_POINT('Ctrl Pts',(1.88097764062697,-1.,3.24413672884812));
#38658=CARTESIAN_POINT('Ctrl Pts',(1.97421938526992,-1.,3.70708211654725));
#38659=CARTESIAN_POINT('Ctrl Pts',(1.97421938526992,1.,3.70708211654725));
#38660=CARTESIAN_POINT('Ctrl Pts',(1.97417727645308,-1.,3.70551008132332));
#38661=CARTESIAN_POINT('Ctrl Pts',(1.97417727645308,1.,3.70551008132332));
#38662=CARTESIAN_POINT('Ctrl Pts',(1.97408973726715,-1.,3.70236698912904));
#38663=CARTESIAN_POINT('Ctrl Pts',(1.97408973726715,1.,3.70236698912904));
#38664=CARTESIAN_POINT('Ctrl Pts',(1.97394846383216,-1.,3.6976552856004));
#38665=CARTESIAN_POINT('Ctrl Pts',(1.97394846383216,1.,3.6976552856004));
#38666=CARTESIAN_POINT('Ctrl Pts',(1.97374016225483,-1.,3.69137888599902));
#38667=CARTESIAN_POINT('Ctrl Pts',(1.97374016225483,1.,3.69137888599902));
#38668=CARTESIAN_POINT('Ctrl Pts',(1.97344650304519,-1.,3.68354319915092));
#38669=CARTESIAN_POINT('Ctrl Pts',(1.97344650304519,1.,3.68354319915092));
#38670=CARTESIAN_POINT('Ctrl Pts',(1.97311947678516,-1.,3.67571738107084));
#38671=CARTESIAN_POINT('Ctrl Pts',(1.97311947678516,1.,3.67571738107084));
#38672=CARTESIAN_POINT('Ctrl Pts',(1.97275897198678,-1.,3.66790152752075));
#38673=CARTESIAN_POINT('Ctrl Pts',(1.97275897198678,1.,3.66790152752075));
#38674=CARTESIAN_POINT('Ctrl Pts',(1.9723648543905,-1.,3.6600957816636));
#38675=CARTESIAN_POINT('Ctrl Pts',(1.9723648543905,1.,3.6600957816636));
#38676=CARTESIAN_POINT('Ctrl Pts',(1.97193697240239,-1.,3.652300347166));
#38677=CARTESIAN_POINT('Ctrl Pts',(1.97193697240239,1.,3.652300347166));
#38678=CARTESIAN_POINT('Ctrl Pts',(1.97147515441164,-1.,3.64451546723514));
#38679=CARTESIAN_POINT('Ctrl Pts',(1.97147515441164,1.,3.64451546723514));
#38680=CARTESIAN_POINT('Ctrl Pts',(1.97097920454464,-1.,3.63674139590412));
#38681=CARTESIAN_POINT('Ctrl Pts',(1.97097920454464,1.,3.63674139590412));
#38682=CARTESIAN_POINT('Ctrl Pts',(1.97044889850463,-1.,3.62897836973293));
#38683=CARTESIAN_POINT('Ctrl Pts',(1.97044889850463,1.,3.62897836973293));
#38684=CARTESIAN_POINT('Ctrl Pts',(1.96988398129978,-1.,3.62122658401893));
#38685=CARTESIAN_POINT('Ctrl Pts',(1.96988398129978,1.,3.62122658401893));
#38686=CARTESIAN_POINT('Ctrl Pts',(1.96928416040877,-1.,3.61348615496704));
#38687=CARTESIAN_POINT('Ctrl Pts',(1.96928416040877,1.,3.61348615496704));
#38688=CARTESIAN_POINT('Ctrl Pts',(1.9686491188594,-1.,3.60575714017989));
#38689=CARTESIAN_POINT('Ctrl Pts',(1.9686491188594,1.,3.60575714017989));
#38690=CARTESIAN_POINT('Ctrl Pts',(1.96797854118369,-1.,3.59803959819938));
#38691=CARTESIAN_POINT('Ctrl Pts',(1.96797854118369,1.,3.59803959819938));
#38692=CARTESIAN_POINT('Ctrl Pts',(1.96727213799544,-1.,3.59033364022801));
#38693=CARTESIAN_POINT('Ctrl Pts',(1.96727213799544,1.,3.59033364022801));
#38694=CARTESIAN_POINT('Ctrl Pts',(1.96652966688911,-1.,3.58263947663829));
#38695=CARTESIAN_POINT('Ctrl Pts',(1.96652966688911,1.,3.58263947663829));
#38696=CARTESIAN_POINT('Ctrl Pts',(1.96575096652789,-1.,3.57495748600959));
#38697=CARTESIAN_POINT('Ctrl Pts',(1.96575096652789,1.,3.57495748600959));
#38698=CARTESIAN_POINT('Ctrl Pts',(1.96493594634567,-1.,3.56728820357791));
#38699=CARTESIAN_POINT('Ctrl Pts',(1.96493594634567,1.,3.56728820357791));
#38700=CARTESIAN_POINT('Ctrl Pts',(1.96408450906812,-1.,3.55963218706096));
#38701=CARTESIAN_POINT('Ctrl Pts',(1.96408450906812,1.,3.55963218706096));
#38702=CARTESIAN_POINT('Ctrl Pts',(1.96319648628644,-1.,3.55198990600886));
#38703=CARTESIAN_POINT('Ctrl Pts',(1.96319648628644,1.,3.55198990600886));
#38704=CARTESIAN_POINT('Ctrl Pts',(1.96227157573067,-1.,3.54436163300443));
#38705=CARTESIAN_POINT('Ctrl Pts',(1.96227157573067,1.,3.54436163300443));
#38706=CARTESIAN_POINT('Ctrl Pts',(1.96130926212689,-1.,3.53674730625813));
#38707=CARTESIAN_POINT('Ctrl Pts',(1.96130926212689,1.,3.53674730625813));
#38708=CARTESIAN_POINT('Ctrl Pts',(1.96030879411566,-1.,3.52914648844351));
#38709=CARTESIAN_POINT('Ctrl Pts',(1.96030879411566,1.,3.52914648844351));
#38710=CARTESIAN_POINT('Ctrl Pts',(1.95926936324461,-1.,3.52155867431486));
#38711=CARTESIAN_POINT('Ctrl Pts',(1.95926936324461,1.,3.52155867431486));
#38712=CARTESIAN_POINT('Ctrl Pts',(1.95819025316779,-1.,3.51398354617794));
#38713=CARTESIAN_POINT('Ctrl Pts',(1.95819025316779,1.,3.51398354617794));
#38714=CARTESIAN_POINT('Ctrl Pts',(1.95707099606511,-1.,3.50642124159909));
#38715=CARTESIAN_POINT('Ctrl Pts',(1.95707099606511,1.,3.50642124159909));
#38716=CARTESIAN_POINT('Ctrl Pts',(1.95591153823661,-1.,3.49887263575583));
#38717=CARTESIAN_POINT('Ctrl Pts',(1.95591153823661,1.,3.49887263575583));
#38718=CARTESIAN_POINT('Ctrl Pts',(1.95471236969643,-1.,3.49133956289133));
#38719=CARTESIAN_POINT('Ctrl Pts',(1.95471236969643,1.,3.49133956289133));
#38720=CARTESIAN_POINT('Ctrl Pts',(1.95347412486308,-1.,3.48382414832634));
#38721=CARTESIAN_POINT('Ctrl Pts',(1.95347412486308,1.,3.48382414832634));
#38722=CARTESIAN_POINT('Ctrl Pts',(1.95219722189876,-1.,3.47632820495921));
#38723=CARTESIAN_POINT('Ctrl Pts',(1.95219722189876,1.,3.47632820495921));
#38724=CARTESIAN_POINT('Ctrl Pts',(1.95088147859876,-1.,3.46885258974191));
#38725=CARTESIAN_POINT('Ctrl Pts',(1.95088147859876,1.,3.46885258974191));
#38726=CARTESIAN_POINT('Ctrl Pts',(1.94952575850197,-1.,3.46139661060962));
#38727=CARTESIAN_POINT('Ctrl Pts',(1.94952575850197,1.,3.46139661060962));
#38728=CARTESIAN_POINT('Ctrl Pts',(1.94812754766524,-1.,3.45395731584051));
#38729=CARTESIAN_POINT('Ctrl Pts',(1.94812754766524,1.,3.45395731584051));
#38730=CARTESIAN_POINT('Ctrl Pts',(1.94668377715329,-1.,3.44653088665681));
#38731=CARTESIAN_POINT('Ctrl Pts',(1.94668377715329,1.,3.44653088665681));
#38732=CARTESIAN_POINT('Ctrl Pts',(1.94519168842879,-1.,3.43911410197687));
#38733=CARTESIAN_POINT('Ctrl Pts',(1.94519168842879,1.,3.43911410197687));
#38734=CARTESIAN_POINT('Ctrl Pts',(1.94364973660284,-1.,3.43170586602434));
#38735=CARTESIAN_POINT('Ctrl Pts',(1.94364973660284,1.,3.43170586602434));
#38736=CARTESIAN_POINT('Ctrl Pts',(1.94205835913696,-1.,3.42430850941503));
#38737=CARTESIAN_POINT('Ctrl Pts',(1.94205835913696,1.,3.42430850941503));
#38738=CARTESIAN_POINT('Ctrl Pts',(1.94042111965246,-1.,3.41692971994096));
#38739=CARTESIAN_POINT('Ctrl Pts',(1.94042111965246,1.,3.41692971994096));
#38740=CARTESIAN_POINT('Ctrl Pts',(1.93874306008143,-1.,3.40957978266642));
#38741=CARTESIAN_POINT('Ctrl Pts',(1.93874306008143,1.,3.40957978266642));
#38742=CARTESIAN_POINT('Ctrl Pts',(1.93702857723098,-1.,3.40226802104109));
#38743=CARTESIAN_POINT('Ctrl Pts',(1.93702857723098,1.,3.40226802104109));
#38744=CARTESIAN_POINT('Ctrl Pts',(1.93527929945985,-1.,3.39499923640795));
#38745=CARTESIAN_POINT('Ctrl Pts',(1.93527929945985,1.,3.39499923640795));
#38746=CARTESIAN_POINT('Ctrl Pts',(1.93349233176788,-1.,3.38777076883256));
#38747=CARTESIAN_POINT('Ctrl Pts',(1.93349233176788,1.,3.38777076883256));
#38748=CARTESIAN_POINT('Ctrl Pts',(1.93165739093276,-1.,3.3805676852555));
#38749=CARTESIAN_POINT('Ctrl Pts',(1.93165739093276,1.,3.3805676852555));
#38750=CARTESIAN_POINT('Ctrl Pts',(1.92975993109877,-1.,3.37336807068043));
#38751=CARTESIAN_POINT('Ctrl Pts',(1.92975993109877,1.,3.37336807068043));
#38752=CARTESIAN_POINT('Ctrl Pts',(1.92778626543786,-1.,3.36615168657567));
#38753=CARTESIAN_POINT('Ctrl Pts',(1.92778626543786,1.,3.36615168657567));
#38754=CARTESIAN_POINT('Ctrl Pts',(1.92572846125756,-1.,3.35890824422965));
#38755=CARTESIAN_POINT('Ctrl Pts',(1.92572846125756,1.,3.35890824422965));
#38756=CARTESIAN_POINT('Ctrl Pts',(1.92358838440528,-1.,3.35164424847223));
#38757=CARTESIAN_POINT('Ctrl Pts',(1.92358838440528,1.,3.35164424847223));
#38758=CARTESIAN_POINT('Ctrl Pts',(1.92138450828404,-1.,3.34439448941961));
#38759=CARTESIAN_POINT('Ctrl Pts',(1.92138450828404,1.,3.34439448941961));
#38760=CARTESIAN_POINT('Ctrl Pts',(1.9191460961021,-1.,3.33721230710012));
#38761=CARTESIAN_POINT('Ctrl Pts',(1.9191460961021,1.,3.33721230710012));
#38762=CARTESIAN_POINT('Ctrl Pts',(1.91690081930331,-1.,3.33014884257873));
#38763=CARTESIAN_POINT('Ctrl Pts',(1.91690081930331,1.,3.33014884257873));
#38764=CARTESIAN_POINT('Ctrl Pts',(1.91466343916627,-1.,3.32323403454535));
#38765=CARTESIAN_POINT('Ctrl Pts',(1.91466343916627,1.,3.32323403454535));
#38766=CARTESIAN_POINT('Ctrl Pts',(1.91242616234442,-1.,3.31646052426364));
#38767=CARTESIAN_POINT('Ctrl Pts',(1.91242616234442,1.,3.31646052426364));
#38768=CARTESIAN_POINT('Ctrl Pts',(1.91014297830446,-1.,3.30975721158596));
#38769=CARTESIAN_POINT('Ctrl Pts',(1.91014297830446,1.,3.30975721158596));
#38770=CARTESIAN_POINT('Ctrl Pts',(1.90773912171341,-1.,3.30300595568195));
#38771=CARTESIAN_POINT('Ctrl Pts',(1.90773912171341,1.,3.30300595568195));
#38772=CARTESIAN_POINT('Ctrl Pts',(1.90513891864087,-1.,3.29608978722113));
#38773=CARTESIAN_POINT('Ctrl Pts',(1.90513891864087,1.,3.29608978722113));
#38774=CARTESIAN_POINT('Ctrl Pts',(1.90228971247527,-1.,3.2889344860029));
#38775=CARTESIAN_POINT('Ctrl Pts',(1.90228971247527,1.,3.2889344860029));
#38776=CARTESIAN_POINT('Ctrl Pts',(1.89918429230462,-1.,3.28154737912352));
#38777=CARTESIAN_POINT('Ctrl Pts',(1.89918429230462,1.,3.28154737912352));
#38778=CARTESIAN_POINT('Ctrl Pts',(1.89589172903793,-1.,3.27407108933139));
#38779=CARTESIAN_POINT('Ctrl Pts',(1.89589172903793,1.,3.27407108933139));
#38780=CARTESIAN_POINT('Ctrl Pts',(1.89255393500965,-1.,3.26677653888676));
#38781=CARTESIAN_POINT('Ctrl Pts',(1.89255393500965,1.,3.26677653888676));
#38782=CARTESIAN_POINT('Ctrl Pts',(1.88934996203698,-1.,3.25999885193947));
#38783=CARTESIAN_POINT('Ctrl Pts',(1.88934996203698,1.,3.25999885193947));
#38784=CARTESIAN_POINT('Ctrl Pts',(1.88646802523466,-1.,3.25408686339463));
#38785=CARTESIAN_POINT('Ctrl Pts',(1.88646802523466,1.,3.25408686339463));
#38786=CARTESIAN_POINT('Ctrl Pts',(1.88407708646357,-1.,3.24935200511918));
#38787=CARTESIAN_POINT('Ctrl Pts',(1.88407708646357,1.,3.24935200511918));
#38788=CARTESIAN_POINT('Ctrl Pts',(1.88229202582941,-1.,3.24600543790443));
#38789=CARTESIAN_POINT('Ctrl Pts',(1.88229202582941,1.,3.24600543790443));
#38790=CARTESIAN_POINT('Ctrl Pts',(1.88139187908074,-1.,3.24451807186481));
#38791=CARTESIAN_POINT('Ctrl Pts',(1.88139187908074,1.,3.24451807186481));
#38792=CARTESIAN_POINT('Ctrl Pts',(1.88102201872555,-1.,3.24408699284121));
#38793=CARTESIAN_POINT('Ctrl Pts',(1.88102201872555,1.,3.24408699284121));
#38794=CARTESIAN_POINT('Ctrl Pts',(1.88091100680349,-1.,3.24410359189609));
#38795=CARTESIAN_POINT('Ctrl Pts',(1.88091100680349,1.,3.24410359189609));
#38796=CARTESIAN_POINT('Ctrl Pts',(1.8808893942881,-1.,3.24418789321065));
#38797=CARTESIAN_POINT('Ctrl Pts',(1.8808893942881,1.,3.24418789321065));
#38798=CARTESIAN_POINT('',(1.97421938526992,1.,3.70708211654725));
#38799=CARTESIAN_POINT('Ctrl Pts',(1.97421938526992,1.,3.70708211654725));
#38800=CARTESIAN_POINT('Ctrl Pts',(1.97417727645308,1.,3.70551008132332));
#38801=CARTESIAN_POINT('Ctrl Pts',(1.97408973726715,1.,3.70236698912904));
#38802=CARTESIAN_POINT('Ctrl Pts',(1.97394846383216,1.,3.6976552856004));
#38803=CARTESIAN_POINT('Ctrl Pts',(1.97374016225483,1.,3.69137888599902));
#38804=CARTESIAN_POINT('Ctrl Pts',(1.97344650304519,1.,3.68354319915092));
#38805=CARTESIAN_POINT('Ctrl Pts',(1.97311947678516,1.,3.67571738107084));
#38806=CARTESIAN_POINT('Ctrl Pts',(1.97275897198678,1.,3.66790152752075));
#38807=CARTESIAN_POINT('Ctrl Pts',(1.9723648543905,1.,3.6600957816636));
#38808=CARTESIAN_POINT('Ctrl Pts',(1.97193697240239,1.,3.652300347166));
#38809=CARTESIAN_POINT('Ctrl Pts',(1.97147515441164,1.,3.64451546723514));
#38810=CARTESIAN_POINT('Ctrl Pts',(1.97097920454464,1.,3.63674139590412));
#38811=CARTESIAN_POINT('Ctrl Pts',(1.97044889850463,1.,3.62897836973293));
#38812=CARTESIAN_POINT('Ctrl Pts',(1.96988398129978,1.,3.62122658401893));
#38813=CARTESIAN_POINT('Ctrl Pts',(1.96928416040877,1.,3.61348615496704));
#38814=CARTESIAN_POINT('Ctrl Pts',(1.9686491188594,1.,3.60575714017989));
#38815=CARTESIAN_POINT('Ctrl Pts',(1.96797854118369,1.,3.59803959819938));
#38816=CARTESIAN_POINT('Ctrl Pts',(1.96727213799544,1.,3.59033364022801));
#38817=CARTESIAN_POINT('Ctrl Pts',(1.96652966688911,1.,3.58263947663829));
#38818=CARTESIAN_POINT('Ctrl Pts',(1.96575096652789,1.,3.57495748600959));
#38819=CARTESIAN_POINT('Ctrl Pts',(1.96493594634567,1.,3.56728820357791));
#38820=CARTESIAN_POINT('Ctrl Pts',(1.96408450906812,1.,3.55963218706096));
#38821=CARTESIAN_POINT('Ctrl Pts',(1.96319648628644,1.,3.55198990600886));
#38822=CARTESIAN_POINT('Ctrl Pts',(1.96227157573067,1.,3.54436163300443));
#38823=CARTESIAN_POINT('Ctrl Pts',(1.96130926212689,1.,3.53674730625813));
#38824=CARTESIAN_POINT('Ctrl Pts',(1.96030879411566,1.,3.52914648844351));
#38825=CARTESIAN_POINT('Ctrl Pts',(1.95926936324461,1.,3.52155867431486));
#38826=CARTESIAN_POINT('Ctrl Pts',(1.95819025316779,1.,3.51398354617794));
#38827=CARTESIAN_POINT('Ctrl Pts',(1.95707099606511,1.,3.50642124159909));
#38828=CARTESIAN_POINT('Ctrl Pts',(1.95591153823661,1.,3.49887263575583));
#38829=CARTESIAN_POINT('Ctrl Pts',(1.95471236969643,1.,3.49133956289133));
#38830=CARTESIAN_POINT('Ctrl Pts',(1.95347412486308,1.,3.48382414832634));
#38831=CARTESIAN_POINT('Ctrl Pts',(1.95219722189876,1.,3.47632820495921));
#38832=CARTESIAN_POINT('Ctrl Pts',(1.95088147859876,1.,3.46885258974191));
#38833=CARTESIAN_POINT('Ctrl Pts',(1.94952575850197,1.,3.46139661060962));
#38834=CARTESIAN_POINT('Ctrl Pts',(1.94812754766524,1.,3.45395731584051));
#38835=CARTESIAN_POINT('Ctrl Pts',(1.94668377715329,1.,3.44653088665681));
#38836=CARTESIAN_POINT('Ctrl Pts',(1.94519168842879,1.,3.43911410197687));
#38837=CARTESIAN_POINT('Ctrl Pts',(1.94364973660284,1.,3.43170586602434));
#38838=CARTESIAN_POINT('Ctrl Pts',(1.94205835913696,1.,3.42430850941503));
#38839=CARTESIAN_POINT('Ctrl Pts',(1.94042111965246,1.,3.41692971994096));
#38840=CARTESIAN_POINT('Ctrl Pts',(1.93874306008143,1.,3.40957978266642));
#38841=CARTESIAN_POINT('Ctrl Pts',(1.93702857723098,1.,3.40226802104109));
#38842=CARTESIAN_POINT('Ctrl Pts',(1.93527929945985,1.,3.39499923640795));
#38843=CARTESIAN_POINT('Ctrl Pts',(1.93349233176788,1.,3.38777076883256));
#38844=CARTESIAN_POINT('Ctrl Pts',(1.93165739093276,1.,3.3805676852555));
#38845=CARTESIAN_POINT('Ctrl Pts',(1.92975993109877,1.,3.37336807068043));
#38846=CARTESIAN_POINT('Ctrl Pts',(1.92778626543786,1.,3.36615168657567));
#38847=CARTESIAN_POINT('Ctrl Pts',(1.92572846125756,1.,3.35890824422965));
#38848=CARTESIAN_POINT('Ctrl Pts',(1.92358838440528,1.,3.35164424847223));
#38849=CARTESIAN_POINT('Ctrl Pts',(1.92138450828404,1.,3.34439448941961));
#38850=CARTESIAN_POINT('Ctrl Pts',(1.9191460961021,1.,3.33721230710012));
#38851=CARTESIAN_POINT('Ctrl Pts',(1.91690081930331,1.,3.33014884257873));
#38852=CARTESIAN_POINT('Ctrl Pts',(1.91466343916627,1.,3.32323403454535));
#38853=CARTESIAN_POINT('Ctrl Pts',(1.91242616234442,1.,3.31646052426364));
#38854=CARTESIAN_POINT('Ctrl Pts',(1.91014297830446,1.,3.30975721158596));
#38855=CARTESIAN_POINT('Ctrl Pts',(1.90773912171341,1.,3.30300595568195));
#38856=CARTESIAN_POINT('Ctrl Pts',(1.90513891864087,1.,3.29608978722113));
#38857=CARTESIAN_POINT('Ctrl Pts',(1.90228971247527,1.,3.2889344860029));
#38858=CARTESIAN_POINT('Ctrl Pts',(1.89918429230462,1.,3.28154737912352));
#38859=CARTESIAN_POINT('Ctrl Pts',(1.89589172903793,1.,3.27407108933139));
#38860=CARTESIAN_POINT('Ctrl Pts',(1.89255393500965,1.,3.26677653888676));
#38861=CARTESIAN_POINT('Ctrl Pts',(1.88934996203698,1.,3.25999885193947));
#38862=CARTESIAN_POINT('Ctrl Pts',(1.88646802523466,1.,3.25408686339463));
#38863=CARTESIAN_POINT('Ctrl Pts',(1.88407708646357,1.,3.24935200511918));
#38864=CARTESIAN_POINT('Ctrl Pts',(1.88242596600454,1.,3.2462565441079));
#38865=CARTESIAN_POINT('Ctrl Pts',(1.88156537699203,1.,3.24480754676064));
#38866=CARTESIAN_POINT('Ctrl Pts',(1.88117508446775,1.,3.24428080353022));
#38867=CARTESIAN_POINT('Ctrl Pts',(1.8810229239812,1.,3.24415531671284));
#38868=CARTESIAN_POINT('Ctrl Pts',(1.88097764062697,1.,3.24413672884812));
#38869=CARTESIAN_POINT('',(1.97421938526992,0.,3.70708211654725));
#38870=CARTESIAN_POINT('Ctrl Pts',(1.519044091397,-1.,3.42855728381368));
#38871=CARTESIAN_POINT('Ctrl Pts',(1.519044091397,1.,3.42855728381368));
#38872=CARTESIAN_POINT('Ctrl Pts',(1.51896318668366,-1.,3.42852521763778));
#38873=CARTESIAN_POINT('Ctrl Pts',(1.51896318668366,1.,3.42852521763778));
#38874=CARTESIAN_POINT('Ctrl Pts',(1.51888450659652,-1.,3.42860527149177));
#38875=CARTESIAN_POINT('Ctrl Pts',(1.51888450659652,1.,3.42860527149177));
#38876=CARTESIAN_POINT('Ctrl Pts',(1.51901585839109,-1.,3.42915787669893));
#38877=CARTESIAN_POINT('Ctrl Pts',(1.51901585839109,1.,3.42915787669893));
#38878=CARTESIAN_POINT('Ctrl Pts',(1.51969006980999,-1.,3.43076036253837));
#38879=CARTESIAN_POINT('Ctrl Pts',(1.51969006980999,1.,3.43076036253837));
#38880=CARTESIAN_POINT('Ctrl Pts',(1.52134826724292,-1.,3.43417156977893));
#38881=CARTESIAN_POINT('Ctrl Pts',(1.52134826724292,1.,3.43417156977893));
#38882=CARTESIAN_POINT('Ctrl Pts',(1.5237734895035,-1.,3.4388889597401));
#38883=CARTESIAN_POINT('Ctrl Pts',(1.5237734895035,1.,3.4388889597401));
#38884=CARTESIAN_POINT('Ctrl Pts',(1.52686242875556,-1.,3.44469547526647));
#38885=CARTESIAN_POINT('Ctrl Pts',(1.52686242875556,1.,3.44469547526647));
#38886=CARTESIAN_POINT('Ctrl Pts',(1.53046244461635,-1.,3.45127136828305));
#38887=CARTESIAN_POINT('Ctrl Pts',(1.53046244461635,1.,3.45127136828305));
#38888=CARTESIAN_POINT('Ctrl Pts',(1.53440195378792,-1.,3.45825932955032));
#38889=CARTESIAN_POINT('Ctrl Pts',(1.53440195378792,1.,3.45825932955032));
#38890=CARTESIAN_POINT('Ctrl Pts',(1.53851507915502,-1.,3.46531752207153));
#38891=CARTESIAN_POINT('Ctrl Pts',(1.53851507915502,1.,3.46531752207153));
#38892=CARTESIAN_POINT('Ctrl Pts',(1.54266605398187,-1.,3.47217189224653));
#38893=CARTESIAN_POINT('Ctrl Pts',(1.54266605398187,1.,3.47217189224653));
#38894=CARTESIAN_POINT('Ctrl Pts',(1.54678009290276,-1.,3.47868272898751));
#38895=CARTESIAN_POINT('Ctrl Pts',(1.54678009290276,1.,3.47868272898751));
#38896=CARTESIAN_POINT('Ctrl Pts',(1.55084702970452,-1.,3.48485155928567));
#38897=CARTESIAN_POINT('Ctrl Pts',(1.55084702970452,1.,3.48485155928567));
#38898=CARTESIAN_POINT('Ctrl Pts',(1.55489595901116,-1.,3.4907646087742));
#38899=CARTESIAN_POINT('Ctrl Pts',(1.55489595901116,1.,3.4907646087742));
#38900=CARTESIAN_POINT('Ctrl Pts',(1.55897703097874,-1.,3.49655185179655));
#38901=CARTESIAN_POINT('Ctrl Pts',(1.55897703097874,1.,3.49655185179655));
#38902=CARTESIAN_POINT('Ctrl Pts',(1.56314187758675,-1.,3.50234321621578));
#38903=CARTESIAN_POINT('Ctrl Pts',(1.56314187758675,1.,3.50234321621578));
#38904=CARTESIAN_POINT('Ctrl Pts',(1.56742097575012,-1.,3.50821771695363));
#38905=CARTESIAN_POINT('Ctrl Pts',(1.56742097575012,1.,3.50821771695363));
#38906=CARTESIAN_POINT('Ctrl Pts',(1.57181569799743,-1.,3.51418598431665));
#38907=CARTESIAN_POINT('Ctrl Pts',(1.57181569799743,1.,3.51418598431665));
#38908=CARTESIAN_POINT('Ctrl Pts',(1.57631049988158,-1.,3.52021847865912));
#38909=CARTESIAN_POINT('Ctrl Pts',(1.57631049988158,1.,3.52021847865912));
#38910=CARTESIAN_POINT('Ctrl Pts',(1.58088027227848,-1.,3.52626275334881));
#38911=CARTESIAN_POINT('Ctrl Pts',(1.58088027227848,1.,3.52626275334881));
#38912=CARTESIAN_POINT('Ctrl Pts',(1.58549906268088,-1.,3.5322637814708));
#38913=CARTESIAN_POINT('Ctrl Pts',(1.58549906268088,1.,3.5322637814708));
#38914=CARTESIAN_POINT('Ctrl Pts',(1.59014958368739,-1.,3.53818616861077));
#38915=CARTESIAN_POINT('Ctrl Pts',(1.59014958368739,1.,3.53818616861077));
#38916=CARTESIAN_POINT('Ctrl Pts',(1.59482766949766,-1.,3.54402458182337));
#38917=CARTESIAN_POINT('Ctrl Pts',(1.59482766949766,1.,3.54402458182337));
#38918=CARTESIAN_POINT('Ctrl Pts',(1.59953698113457,-1.,3.54979148634454));
#38919=CARTESIAN_POINT('Ctrl Pts',(1.59953698113457,1.,3.54979148634454));
#38920=CARTESIAN_POINT('Ctrl Pts',(1.60428584699853,-1.,3.55550985096129));
#38921=CARTESIAN_POINT('Ctrl Pts',(1.60428584699853,1.,3.55550985096129));
#38922=CARTESIAN_POINT('Ctrl Pts',(1.60908344685457,-1.,3.5612043248298));
#38923=CARTESIAN_POINT('Ctrl Pts',(1.60908344685457,1.,3.5612043248298));
#38924=CARTESIAN_POINT('Ctrl Pts',(1.61393581747514,-1.,3.56689200468387));
#38925=CARTESIAN_POINT('Ctrl Pts',(1.61393581747514,1.,3.56689200468387));
#38926=CARTESIAN_POINT('Ctrl Pts',(1.61884340915404,-1.,3.57257679609806));
#38927=CARTESIAN_POINT('Ctrl Pts',(1.61884340915404,1.,3.57257679609806));
#38928=CARTESIAN_POINT('Ctrl Pts',(1.62380329464844,-1.,3.5782545595439));
#38929=CARTESIAN_POINT('Ctrl Pts',(1.62380329464844,1.,3.5782545595439));
#38930=CARTESIAN_POINT('Ctrl Pts',(1.62881051550745,-1.,3.58391625774343));
#38931=CARTESIAN_POINT('Ctrl Pts',(1.62881051550745,1.,3.58391625774343));
#38932=CARTESIAN_POINT('Ctrl Pts',(1.6338597145126,-1.,3.58955176627879));
#38933=CARTESIAN_POINT('Ctrl Pts',(1.6338597145126,1.,3.58955176627879));
#38934=CARTESIAN_POINT('Ctrl Pts',(1.63894676675352,-1.,3.59515368334893));
#38935=CARTESIAN_POINT('Ctrl Pts',(1.63894676675352,1.,3.59515368334893));
#38936=CARTESIAN_POINT('Ctrl Pts',(1.64407004385582,-1.,3.60072028513845));
#38937=CARTESIAN_POINT('Ctrl Pts',(1.64407004385582,1.,3.60072028513845));
#38938=CARTESIAN_POINT('Ctrl Pts',(1.64922952425832,-1.,3.60625346556992));
#38939=CARTESIAN_POINT('Ctrl Pts',(1.64922952425832,1.,3.60625346556992));
#38940=CARTESIAN_POINT('Ctrl Pts',(1.65442619244325,-1.,3.61175734965127));
#38941=CARTESIAN_POINT('Ctrl Pts',(1.65442619244325,1.,3.61175734965127));
#38942=CARTESIAN_POINT('Ctrl Pts',(1.65966133399186,-1.,3.61723666482456));
#38943=CARTESIAN_POINT('Ctrl Pts',(1.65966133399186,1.,3.61723666482456));
#38944=CARTESIAN_POINT('Ctrl Pts',(1.66493585923855,-1.,3.62269517989109));
#38945=CARTESIAN_POINT('Ctrl Pts',(1.66493585923855,1.,3.62269517989109));
#38946=CARTESIAN_POINT('Ctrl Pts',(1.67024966008044,-1.,3.62813422105271));
#38947=CARTESIAN_POINT('Ctrl Pts',(1.67024966008044,1.,3.62813422105271));
#38948=CARTESIAN_POINT('Ctrl Pts',(1.67560193613156,-1.,3.63355343201232));
#38949=CARTESIAN_POINT('Ctrl Pts',(1.67560193613156,1.,3.63355343201232));
#38950=CARTESIAN_POINT('Ctrl Pts',(1.68099146651586,-1.,3.63895140887462));
#38951=CARTESIAN_POINT('Ctrl Pts',(1.68099146651586,1.,3.63895140887462));
#38952=CARTESIAN_POINT('Ctrl Pts',(1.68641690471457,-1.,3.64432638915203));
#38953=CARTESIAN_POINT('Ctrl Pts',(1.68641690471457,1.,3.64432638915203));
#38954=CARTESIAN_POINT('Ctrl Pts',(1.69187705481689,-1.,3.64967689827371));
#38955=CARTESIAN_POINT('Ctrl Pts',(1.69187705481689,1.,3.64967689827371));
#38956=CARTESIAN_POINT('Ctrl Pts',(1.69737117722534,-1.,3.65500246526749));
#38957=CARTESIAN_POINT('Ctrl Pts',(1.69737117722534,1.,3.65500246526749));
#38958=CARTESIAN_POINT('Ctrl Pts',(1.70289888566873,-1.,3.66030338774847));
#38959=CARTESIAN_POINT('Ctrl Pts',(1.70289888566873,1.,3.66030338774847));
#38960=CARTESIAN_POINT('Ctrl Pts',(1.70846001610956,-1.,3.66558043198876));
#38961=CARTESIAN_POINT('Ctrl Pts',(1.70846001610956,1.,3.66558043198876));
#38962=CARTESIAN_POINT('Ctrl Pts',(1.71405450210383,-1.,3.67083454901611));
#38963=CARTESIAN_POINT('Ctrl Pts',(1.71405450210383,1.,3.67083454901611));
#38964=CARTESIAN_POINT('Ctrl Pts',(1.71968225581808,-1.,3.67606660374709));
#38965=CARTESIAN_POINT('Ctrl Pts',(1.71968225581808,1.,3.67606660374709));
#38966=CARTESIAN_POINT('Ctrl Pts',(1.72534302437056,-1.,3.68127704936579));
#38967=CARTESIAN_POINT('Ctrl Pts',(1.72534302437056,1.,3.68127704936579));
#38968=CARTESIAN_POINT('Ctrl Pts',(1.73103640956717,-1.,3.68646597019332));
#38969=CARTESIAN_POINT('Ctrl Pts',(1.73103640956717,1.,3.68646597019332));
#38970=CARTESIAN_POINT('Ctrl Pts',(1.73676193254557,-1.,3.69163322648036));
#38971=CARTESIAN_POINT('Ctrl Pts',(1.73676193254557,1.,3.69163322648036));
#38972=CARTESIAN_POINT('Ctrl Pts',(1.74251908492617,-1.,3.69677856910517));
#38973=CARTESIAN_POINT('Ctrl Pts',(1.74251908492617,1.,3.69677856910517));
#38974=CARTESIAN_POINT('Ctrl Pts',(1.74830738046057,-1.,3.7019017567335));
#38975=CARTESIAN_POINT('Ctrl Pts',(1.74830738046057,1.,3.7019017567335));
#38976=CARTESIAN_POINT('Ctrl Pts',(1.75412641804042,-1.,3.70700269736659));
#38977=CARTESIAN_POINT('Ctrl Pts',(1.75412641804042,1.,3.70700269736659));
#38978=CARTESIAN_POINT('Ctrl Pts',(1.75997588498865,-1.,3.71208146346136));
#38979=CARTESIAN_POINT('Ctrl Pts',(1.75997588498865,1.,3.71208146346136));
#38980=CARTESIAN_POINT('Ctrl Pts',(1.76585552124394,-1.,3.71713822377359));
#38981=CARTESIAN_POINT('Ctrl Pts',(1.76585552124394,1.,3.71713822377359));
#38982=CARTESIAN_POINT('Ctrl Pts',(1.77176509401761,-1.,3.72217319911254));
#38983=CARTESIAN_POINT('Ctrl Pts',(1.77176509401761,1.,3.72217319911254));
#38984=CARTESIAN_POINT('Ctrl Pts',(1.77770437039658,-1.,3.72718661205609));
#38985=CARTESIAN_POINT('Ctrl Pts',(1.77770437039658,1.,3.72718661205609));
#38986=CARTESIAN_POINT('Ctrl Pts',(1.78367308442901,-1.,3.7321786309547));
#38987=CARTESIAN_POINT('Ctrl Pts',(1.78367308442901,1.,3.7321786309547));
#38988=CARTESIAN_POINT('Ctrl Pts',(1.78967092823491,-1.,3.73714934730681));
#38989=CARTESIAN_POINT('Ctrl Pts',(1.78967092823491,1.,3.73714934730681));
#38990=CARTESIAN_POINT('Ctrl Pts',(1.79569757859422,-1.,3.74209880352445));
#38991=CARTESIAN_POINT('Ctrl Pts',(1.79569757859422,1.,3.74209880352445));
#38992=CARTESIAN_POINT('Ctrl Pts',(1.8017527148577,-1.,3.74702700875467));
#38993=CARTESIAN_POINT('Ctrl Pts',(1.8017527148577,1.,3.74702700875467));
#38994=CARTESIAN_POINT('Ctrl Pts',(1.80783603939617,-1.,3.75193395887977));
#38995=CARTESIAN_POINT('Ctrl Pts',(1.80783603939617,1.,3.75193395887977));
#38996=CARTESIAN_POINT('Ctrl Pts',(1.8139472983358,-1.,3.75681965683071));
#38997=CARTESIAN_POINT('Ctrl Pts',(1.8139472983358,1.,3.75681965683071));
#38998=CARTESIAN_POINT('Ctrl Pts',(1.82008629694091,-1.,3.76168412707948));
#38999=CARTESIAN_POINT('Ctrl Pts',(1.82008629694091,1.,3.76168412707948));
#39000=CARTESIAN_POINT('Ctrl Pts',(1.82625289220915,-1.,3.76652740353775));
#39001=CARTESIAN_POINT('Ctrl Pts',(1.82625289220915,1.,3.76652740353775));
#39002=CARTESIAN_POINT('Ctrl Pts',(1.83120816955645,-1.,3.77038509817999));
#39003=CARTESIAN_POINT('Ctrl Pts',(1.83120816955645,1.,3.77038509817999));
#39004=CARTESIAN_POINT('Ctrl Pts',(1.83493697934534,-1.,3.77326886064398));
#39005=CARTESIAN_POINT('Ctrl Pts',(1.83493697934534,1.,3.77326886064398));
#39006=CARTESIAN_POINT('Ctrl Pts',(1.83742834010626,-1.,3.77518714457833));
#39007=CARTESIAN_POINT('Ctrl Pts',(1.83742834010626,1.,3.77518714457833));
#39008=CARTESIAN_POINT('Ctrl Pts',(1.8386753923786,-1.,3.77614523045147));
#39009=CARTESIAN_POINT('Ctrl Pts',(1.8386753923786,1.,3.77614523045147));
#39010=CARTESIAN_POINT('',(1.5189508286633,1.,3.42859860294306));
#39011=CARTESIAN_POINT('Ctrl Pts',(1.5189508286633,-1.,3.42859860294306));
#39012=CARTESIAN_POINT('Ctrl Pts',(1.5189508286633,-0.666666666666667,3.42859860294306));
#39013=CARTESIAN_POINT('Ctrl Pts',(1.5189508286633,-0.333333333333333,3.42859860294306));
#39014=CARTESIAN_POINT('Ctrl Pts',(1.5189508286633,0.333333333333333,3.42859860294306));
#39015=CARTESIAN_POINT('Ctrl Pts',(1.5189508286633,0.666666666666667,3.42859860294306));
#39016=CARTESIAN_POINT('Ctrl Pts',(1.5189508286633,1.,3.42859860294306));
#39017=CARTESIAN_POINT('',(1.8386753923786,1.,3.77614523045147));
#39018=CARTESIAN_POINT('',(1.8386753923786,0.,3.77614523045147));
#39019=CARTESIAN_POINT('Ctrl Pts',(1.5189508286633,1.,3.42859860294306));
#39020=CARTESIAN_POINT('Ctrl Pts',(1.51893924967331,1.,3.42864616361875));
#39021=CARTESIAN_POINT('Ctrl Pts',(1.5189513329503,1.,3.42884302333841));
#39022=CARTESIAN_POINT('Ctrl Pts',(1.51914806898491,1.,3.42946838852587));
#39023=CARTESIAN_POINT('Ctrl Pts',(1.5198144909338,1.,3.43101631893414));
#39024=CARTESIAN_POINT('Ctrl Pts',(1.52134826724292,1.,3.43417156977893));
#39025=CARTESIAN_POINT('Ctrl Pts',(1.5237734895035,1.,3.4388889597401));
#39026=CARTESIAN_POINT('Ctrl Pts',(1.52686242875556,1.,3.44469547526647));
#39027=CARTESIAN_POINT('Ctrl Pts',(1.53046244461635,1.,3.45127136828305));
#39028=CARTESIAN_POINT('Ctrl Pts',(1.53440195378792,1.,3.45825932955032));
#39029=CARTESIAN_POINT('Ctrl Pts',(1.53851507915502,1.,3.46531752207153));
#39030=CARTESIAN_POINT('Ctrl Pts',(1.54266605398187,1.,3.47217189224653));
#39031=CARTESIAN_POINT('Ctrl Pts',(1.54678009290276,1.,3.47868272898751));
#39032=CARTESIAN_POINT('Ctrl Pts',(1.55084702970452,1.,3.48485155928567));
#39033=CARTESIAN_POINT('Ctrl Pts',(1.55489595901116,1.,3.4907646087742));
#39034=CARTESIAN_POINT('Ctrl Pts',(1.55897703097874,1.,3.49655185179655));
#39035=CARTESIAN_POINT('Ctrl Pts',(1.56314187758675,1.,3.50234321621578));
#39036=CARTESIAN_POINT('Ctrl Pts',(1.56742097575012,1.,3.50821771695363));
#39037=CARTESIAN_POINT('Ctrl Pts',(1.57181569799743,1.,3.51418598431665));
#39038=CARTESIAN_POINT('Ctrl Pts',(1.57631049988158,1.,3.52021847865912));
#39039=CARTESIAN_POINT('Ctrl Pts',(1.58088027227848,1.,3.52626275334881));
#39040=CARTESIAN_POINT('Ctrl Pts',(1.58549906268088,1.,3.5322637814708));
#39041=CARTESIAN_POINT('Ctrl Pts',(1.59014958368739,1.,3.53818616861077));
#39042=CARTESIAN_POINT('Ctrl Pts',(1.59482766949766,1.,3.54402458182337));
#39043=CARTESIAN_POINT('Ctrl Pts',(1.59953698113457,1.,3.54979148634454));
#39044=CARTESIAN_POINT('Ctrl Pts',(1.60428584699853,1.,3.55550985096129));
#39045=CARTESIAN_POINT('Ctrl Pts',(1.60908344685457,1.,3.5612043248298));
#39046=CARTESIAN_POINT('Ctrl Pts',(1.61393581747514,1.,3.56689200468387));
#39047=CARTESIAN_POINT('Ctrl Pts',(1.61884340915404,1.,3.57257679609806));
#39048=CARTESIAN_POINT('Ctrl Pts',(1.62380329464844,1.,3.5782545595439));
#39049=CARTESIAN_POINT('Ctrl Pts',(1.62881051550745,1.,3.58391625774343));
#39050=CARTESIAN_POINT('Ctrl Pts',(1.6338597145126,1.,3.58955176627879));
#39051=CARTESIAN_POINT('Ctrl Pts',(1.63894676675352,1.,3.59515368334893));
#39052=CARTESIAN_POINT('Ctrl Pts',(1.64407004385582,1.,3.60072028513845));
#39053=CARTESIAN_POINT('Ctrl Pts',(1.64922952425832,1.,3.60625346556992));
#39054=CARTESIAN_POINT('Ctrl Pts',(1.65442619244325,1.,3.61175734965127));
#39055=CARTESIAN_POINT('Ctrl Pts',(1.65966133399186,1.,3.61723666482456));
#39056=CARTESIAN_POINT('Ctrl Pts',(1.66493585923855,1.,3.62269517989109));
#39057=CARTESIAN_POINT('Ctrl Pts',(1.67024966008044,1.,3.62813422105271));
#39058=CARTESIAN_POINT('Ctrl Pts',(1.67560193613156,1.,3.63355343201232));
#39059=CARTESIAN_POINT('Ctrl Pts',(1.68099146651586,1.,3.63895140887462));
#39060=CARTESIAN_POINT('Ctrl Pts',(1.68641690471457,1.,3.64432638915203));
#39061=CARTESIAN_POINT('Ctrl Pts',(1.69187705481689,1.,3.64967689827371));
#39062=CARTESIAN_POINT('Ctrl Pts',(1.69737117722534,1.,3.65500246526749));
#39063=CARTESIAN_POINT('Ctrl Pts',(1.70289888566873,1.,3.66030338774847));
#39064=CARTESIAN_POINT('Ctrl Pts',(1.70846001610956,1.,3.66558043198876));
#39065=CARTESIAN_POINT('Ctrl Pts',(1.71405450210383,1.,3.67083454901611));
#39066=CARTESIAN_POINT('Ctrl Pts',(1.71968225581808,1.,3.67606660374709));
#39067=CARTESIAN_POINT('Ctrl Pts',(1.72534302437056,1.,3.68127704936579));
#39068=CARTESIAN_POINT('Ctrl Pts',(1.73103640956717,1.,3.68646597019332));
#39069=CARTESIAN_POINT('Ctrl Pts',(1.73676193254557,1.,3.69163322648036));
#39070=CARTESIAN_POINT('Ctrl Pts',(1.74251908492617,1.,3.69677856910517));
#39071=CARTESIAN_POINT('Ctrl Pts',(1.74830738046057,1.,3.7019017567335));
#39072=CARTESIAN_POINT('Ctrl Pts',(1.75412641804042,1.,3.70700269736659));
#39073=CARTESIAN_POINT('Ctrl Pts',(1.75997588498865,1.,3.71208146346136));
#39074=CARTESIAN_POINT('Ctrl Pts',(1.76585552124394,1.,3.71713822377359));
#39075=CARTESIAN_POINT('Ctrl Pts',(1.77176509401761,1.,3.72217319911254));
#39076=CARTESIAN_POINT('Ctrl Pts',(1.77770437039658,1.,3.72718661205609));
#39077=CARTESIAN_POINT('Ctrl Pts',(1.78367308442901,1.,3.7321786309547));
#39078=CARTESIAN_POINT('Ctrl Pts',(1.78967092823491,1.,3.73714934730681));
#39079=CARTESIAN_POINT('Ctrl Pts',(1.79569757859422,1.,3.74209880352445));
#39080=CARTESIAN_POINT('Ctrl Pts',(1.8017527148577,1.,3.74702700875467));
#39081=CARTESIAN_POINT('Ctrl Pts',(1.80783603939617,1.,3.75193395887977));
#39082=CARTESIAN_POINT('Ctrl Pts',(1.8139472983358,1.,3.75681965683071));
#39083=CARTESIAN_POINT('Ctrl Pts',(1.82008629694091,1.,3.76168412707948));
#39084=CARTESIAN_POINT('Ctrl Pts',(1.82625289220915,1.,3.76652740353775));
#39085=CARTESIAN_POINT('Ctrl Pts',(1.83120816955645,1.,3.77038509817999));
#39086=CARTESIAN_POINT('Ctrl Pts',(1.83493697934534,1.,3.77326886064398));
#39087=CARTESIAN_POINT('Ctrl Pts',(1.83742834010626,1.,3.77518714457833));
#39088=CARTESIAN_POINT('Ctrl Pts',(1.8386753923786,1.,3.77614523045147));
#39089=CARTESIAN_POINT('Origin',(1.8386753923786,0.,3.77614523045147));
#39090=CARTESIAN_POINT('',(1.97421938526992,1.,3.70708211654725));
#39091=CARTESIAN_POINT('Origin',(0.,0.,0.));
#39092=CARTESIAN_POINT('',(1.35032489087269,1.,3.49844575334386));
#39093=CARTESIAN_POINT('Origin',(0.,1.,0.));
#39094=CARTESIAN_POINT('Ctrl Pts',(1.35032489087269,1.,3.49844575334386));
#39095=CARTESIAN_POINT('Ctrl Pts',(1.35032489087269,0.666666666666667,3.49844575334386));
#39096=CARTESIAN_POINT('Ctrl Pts',(1.35032489087269,0.333333333333333,3.49844575334386));
#39097=CARTESIAN_POINT('Ctrl Pts',(1.35032489087269,-0.333333333333333,
3.49844575334386));
#39098=CARTESIAN_POINT('Ctrl Pts',(1.35032489087269,-0.666666666666667,
3.49844575334386));
#39099=CARTESIAN_POINT('Ctrl Pts',(1.35032489087269,-1.,3.49844575334386));
#39100=CARTESIAN_POINT('Ctrl Pts',(1.36999806084572,-1.,3.97027773754922));
#39101=CARTESIAN_POINT('Ctrl Pts',(1.36999806084572,1.,3.97027773754922));
#39102=CARTESIAN_POINT('Ctrl Pts',(1.37020239094758,-1.,3.9687184694173));
#39103=CARTESIAN_POINT('Ctrl Pts',(1.37020239094758,1.,3.9687184694173));
#39104=CARTESIAN_POINT('Ctrl Pts',(1.37060761746027,-1.,3.96560037975788));
#39105=CARTESIAN_POINT('Ctrl Pts',(1.37060761746027,1.,3.96560037975788));
#39106=CARTESIAN_POINT('Ctrl Pts',(1.37120515615663,-1.,3.96092458508407));
#39107=CARTESIAN_POINT('Ctrl Pts',(1.37120515615663,1.,3.96092458508407));
#39108=CARTESIAN_POINT('Ctrl Pts',(1.37198126433139,-1.,3.95469287283105));
#39109=CARTESIAN_POINT('Ctrl Pts',(1.37198126433139,1.,3.95469287283105));
#39110=CARTESIAN_POINT('Ctrl Pts',(1.37291699203423,-1.,3.94690771786926));
#39111=CARTESIAN_POINT('Ctrl Pts',(1.37291699203423,1.,3.94690771786926));
#39112=CARTESIAN_POINT('Ctrl Pts',(1.37381821967499,-1.,3.93912709041791));
#39113=CARTESIAN_POINT('Ctrl Pts',(1.37381821967499,1.,3.93912709041791));
#39114=CARTESIAN_POINT('Ctrl Pts',(1.37468482215784,-1.,3.93135106761941));
#39115=CARTESIAN_POINT('Ctrl Pts',(1.37468482215784,1.,3.93135106761941));
#39116=CARTESIAN_POINT('Ctrl Pts',(1.37551664448057,-1.,3.92357976987132));
#39117=CARTESIAN_POINT('Ctrl Pts',(1.37551664448057,1.,3.92357976987132));
#39118=CARTESIAN_POINT('Ctrl Pts',(1.37631350505516,-1.,3.91581337461825));
#39119=CARTESIAN_POINT('Ctrl Pts',(1.37631350505516,1.,3.91581337461825));
#39120=CARTESIAN_POINT('Ctrl Pts',(1.3770751963376,-1.,3.90805209522729));
#39121=CARTESIAN_POINT('Ctrl Pts',(1.3770751963376,1.,3.90805209522729));
#39122=CARTESIAN_POINT('Ctrl Pts',(1.3778014851263,-1.,3.90029615196255));
#39123=CARTESIAN_POINT('Ctrl Pts',(1.3778014851263,1.,3.90029615196255));
#39124=CARTESIAN_POINT('Ctrl Pts',(1.37849211287981,-1.,3.89254574338385));
#39125=CARTESIAN_POINT('Ctrl Pts',(1.37849211287981,1.,3.89254574338385));
#39126=CARTESIAN_POINT('Ctrl Pts',(1.37914679719446,-1.,3.88480102249461));
#39127=CARTESIAN_POINT('Ctrl Pts',(1.37914679719446,1.,3.88480102249461));
#39128=CARTESIAN_POINT('Ctrl Pts',(1.37976523097187,-1.,3.87706205830865));
#39129=CARTESIAN_POINT('Ctrl Pts',(1.37976523097187,1.,3.87706205830865));
#39130=CARTESIAN_POINT('Ctrl Pts',(1.38034709213129,-1.,3.86932885813403));
#39131=CARTESIAN_POINT('Ctrl Pts',(1.38034709213129,1.,3.86932885813403));
#39132=CARTESIAN_POINT('Ctrl Pts',(1.38089205993067,-1.,3.86160143044187));
#39133=CARTESIAN_POINT('Ctrl Pts',(1.38089205993067,1.,3.86160143044187));
#39134=CARTESIAN_POINT('Ctrl Pts',(1.38139983115075,-1.,3.85387983979557));
#39135=CARTESIAN_POINT('Ctrl Pts',(1.38139983115075,1.,3.85387983979557));
#39136=CARTESIAN_POINT('Ctrl Pts',(1.38187013346089,-1.,3.84616425605705));
#39137=CARTESIAN_POINT('Ctrl Pts',(1.38187013346089,1.,3.84616425605705));
#39138=CARTESIAN_POINT('Ctrl Pts',(1.38230274828774,-1.,3.83845502790609));
#39139=CARTESIAN_POINT('Ctrl Pts',(1.38230274828774,1.,3.83845502790609));
#39140=CARTESIAN_POINT('Ctrl Pts',(1.38269750245086,-1.,3.83075266982138));
#39141=CARTESIAN_POINT('Ctrl Pts',(1.38269750245086,1.,3.83075266982138));
#39142=CARTESIAN_POINT('Ctrl Pts',(1.38305421262724,-1.,3.82305771743715));
#39143=CARTESIAN_POINT('Ctrl Pts',(1.38305421262724,1.,3.82305771743715));
#39144=CARTESIAN_POINT('Ctrl Pts',(1.38337263902766,-1.,3.81537060817765));
#39145=CARTESIAN_POINT('Ctrl Pts',(1.38337263902766,1.,3.81537060817765));
#39146=CARTESIAN_POINT('Ctrl Pts',(1.38365244046226,-1.,3.80769156398429));
#39147=CARTESIAN_POINT('Ctrl Pts',(1.38365244046226,1.,3.80769156398429));
#39148=CARTESIAN_POINT('Ctrl Pts',(1.38389311766701,-1.,3.80002044322169));
#39149=CARTESIAN_POINT('Ctrl Pts',(1.38389311766701,1.,3.80002044322169));
#39150=CARTESIAN_POINT('Ctrl Pts',(1.38409399694588,-1.,3.79235669640907));
#39151=CARTESIAN_POINT('Ctrl Pts',(1.38409399694588,1.,3.79235669640907));
#39152=CARTESIAN_POINT('Ctrl Pts',(1.38425435883773,-1.,3.78469969805134));
#39153=CARTESIAN_POINT('Ctrl Pts',(1.38425435883773,1.,3.78469969805134));
#39154=CARTESIAN_POINT('Ctrl Pts',(1.38437354551435,-1.,3.77704902230441));
#39155=CARTESIAN_POINT('Ctrl Pts',(1.38437354551435,1.,3.77704902230441));
#39156=CARTESIAN_POINT('Ctrl Pts',(1.38445107339517,-1.,3.76940473185775));
#39157=CARTESIAN_POINT('Ctrl Pts',(1.38445107339517,1.,3.76940473185775));
#39158=CARTESIAN_POINT('Ctrl Pts',(1.38448675253343,-1.,3.76176768271347));
#39159=CARTESIAN_POINT('Ctrl Pts',(1.38448675253343,1.,3.76176768271347));
#39160=CARTESIAN_POINT('Ctrl Pts',(1.38448077997155,-1.,3.75413976318727));
#39161=CARTESIAN_POINT('Ctrl Pts',(1.38448077997155,1.,3.75413976318727));
#39162=CARTESIAN_POINT('Ctrl Pts',(1.38443344984389,-1.,3.7465231716786));
#39163=CARTESIAN_POINT('Ctrl Pts',(1.38443344984389,1.,3.7465231716786));
#39164=CARTESIAN_POINT('Ctrl Pts',(1.38434489156456,-1.,3.73891976418099));
#39165=CARTESIAN_POINT('Ctrl Pts',(1.38434489156456,1.,3.73891976418099));
#39166=CARTESIAN_POINT('Ctrl Pts',(1.38421479111531,-1.,3.73133035859283));
#39167=CARTESIAN_POINT('Ctrl Pts',(1.38421479111531,1.,3.73133035859283));
#39168=CARTESIAN_POINT('Ctrl Pts',(1.3840421342895,-1.,3.72375409358805));
#39169=CARTESIAN_POINT('Ctrl Pts',(1.3840421342895,1.,3.72375409358805));
#39170=CARTESIAN_POINT('Ctrl Pts',(1.38382489984585,-1.,3.7161876605181));
#39171=CARTESIAN_POINT('Ctrl Pts',(1.38382489984585,1.,3.7161876605181));
#39172=CARTESIAN_POINT('Ctrl Pts',(1.38356065402122,-1.,3.70862680753343));
#39173=CARTESIAN_POINT('Ctrl Pts',(1.38356065402122,1.,3.70862680753343));
#39174=CARTESIAN_POINT('Ctrl Pts',(1.38324717612862,-1.,3.70106792167894));
#39175=CARTESIAN_POINT('Ctrl Pts',(1.38324717612862,1.,3.70106792167894));
#39176=CARTESIAN_POINT('Ctrl Pts',(1.38288311171649,-1.,3.69350967899523));
#39177=CARTESIAN_POINT('Ctrl Pts',(1.38288311171649,1.,3.69350967899523));
#39178=CARTESIAN_POINT('Ctrl Pts',(1.38246852827185,-1.,3.68595444983844));
#39179=CARTESIAN_POINT('Ctrl Pts',(1.38246852827185,1.,3.68595444983844));
#39180=CARTESIAN_POINT('Ctrl Pts',(1.38200574290626,-1.,3.6784103848243));
#39181=CARTESIAN_POINT('Ctrl Pts',(1.38200574290626,1.,3.6784103848243));
#39182=CARTESIAN_POINT('Ctrl Pts',(1.38149812653876,-1.,3.67088843112282));
#39183=CARTESIAN_POINT('Ctrl Pts',(1.38149812653876,1.,3.67088843112282));
#39184=CARTESIAN_POINT('Ctrl Pts',(1.38094856333558,-1.,3.66339848520874));
#39185=CARTESIAN_POINT('Ctrl Pts',(1.38094856333558,1.,3.66339848520874));
#39186=CARTESIAN_POINT('Ctrl Pts',(1.38035791051215,-1.,3.65594554404396));
#39187=CARTESIAN_POINT('Ctrl Pts',(1.38035791051215,1.,3.65594554404396));
#39188=CARTESIAN_POINT('Ctrl Pts',(1.37972372481598,-1.,3.64852652756444));
#39189=CARTESIAN_POINT('Ctrl Pts',(1.37972372481598,1.,3.64852652756444));
#39190=CARTESIAN_POINT('Ctrl Pts',(1.37903818567347,-1.,3.64112507791112));
#39191=CARTESIAN_POINT('Ctrl Pts',(1.37903818567347,1.,3.64112507791112));
#39192=CARTESIAN_POINT('Ctrl Pts',(1.37829035457324,-1.,3.63371727442448));
#39193=CARTESIAN_POINT('Ctrl Pts',(1.37829035457324,1.,3.63371727442448));
#39194=CARTESIAN_POINT('Ctrl Pts',(1.37746987919868,-1.,3.62628098665112));
#39195=CARTESIAN_POINT('Ctrl Pts',(1.37746987919868,1.,3.62628098665112));
#39196=CARTESIAN_POINT('Ctrl Pts',(1.37657053403102,-1.,3.61880481160408));
#39197=CARTESIAN_POINT('Ctrl Pts',(1.37657053403102,1.,3.61880481160408));
#39198=CARTESIAN_POINT('Ctrl Pts',(1.37559314436641,-1.,3.61129546591082));
#39199=CARTESIAN_POINT('Ctrl Pts',(1.37559314436641,1.,3.61129546591082));
#39200=CARTESIAN_POINT('Ctrl Pts',(1.37455051379642,-1.,3.60379020124038));
#39201=CARTESIAN_POINT('Ctrl Pts',(1.37455051379642,1.,3.60379020124038));
#39202=CARTESIAN_POINT('Ctrl Pts',(1.37346320103184,-1.,3.59634627869117));
#39203=CARTESIAN_POINT('Ctrl Pts',(1.37346320103184,1.,3.59634627869117));
#39204=CARTESIAN_POINT('Ctrl Pts',(1.37235053661,-1.,3.5890185384643));
#39205=CARTESIAN_POINT('Ctrl Pts',(1.37235053661,1.,3.5890185384643));
#39206=CARTESIAN_POINT('Ctrl Pts',(1.37122241663073,-1.,3.58183885982745));
#39207=CARTESIAN_POINT('Ctrl Pts',(1.37122241663073,1.,3.58183885982745));
#39208=CARTESIAN_POINT('Ctrl Pts',(1.37007229485646,-1.,3.57479875549453));
#39209=CARTESIAN_POINT('Ctrl Pts',(1.37007229485646,1.,3.57479875549453));
#39210=CARTESIAN_POINT('Ctrl Pts',(1.36886584973349,-1.,3.56782080304554));
#39211=CARTESIAN_POINT('Ctrl Pts',(1.36886584973349,1.,3.56782080304554));
#39212=CARTESIAN_POINT('Ctrl Pts',(1.36754771771174,-1.,3.56077662028492));
#39213=CARTESIAN_POINT('Ctrl Pts',(1.36754771771174,1.,3.56077662028492));
#39214=CARTESIAN_POINT('Ctrl Pts',(1.36606145456711,-1.,3.55353883995793));
#39215=CARTESIAN_POINT('Ctrl Pts',(1.36606145456711,1.,3.55353883995793));
#39216=CARTESIAN_POINT('Ctrl Pts',(1.36436666257567,-1.,3.54602591832893));
#39217=CARTESIAN_POINT('Ctrl Pts',(1.36436666257567,1.,3.54602591832893));
#39218=CARTESIAN_POINT('Ctrl Pts',(1.36245507339334,-1.,3.53824396425032));
#39219=CARTESIAN_POINT('Ctrl Pts',(1.36245507339334,1.,3.53824396425032));
#39220=CARTESIAN_POINT('Ctrl Pts',(1.36037259643827,-1.,3.53034464961849));
#39221=CARTESIAN_POINT('Ctrl Pts',(1.36037259643827,1.,3.53034464961849));
#39222=CARTESIAN_POINT('Ctrl Pts',(1.35821701528975,-1.,3.52261776117121));
#39223=CARTESIAN_POINT('Ctrl Pts',(1.35821701528975,1.,3.52261776117121));
#39224=CARTESIAN_POINT('Ctrl Pts',(1.35611275237288,-1.,3.51542230699919));
#39225=CARTESIAN_POINT('Ctrl Pts',(1.35611275237288,1.,3.51542230699919));
#39226=CARTESIAN_POINT('Ctrl Pts',(1.35419113576022,-1.,3.50913227060177));
#39227=CARTESIAN_POINT('Ctrl Pts',(1.35419113576022,1.,3.50913227060177));
#39228=CARTESIAN_POINT('Ctrl Pts',(1.3525703284343,-1.,3.50408168106113));
#39229=CARTESIAN_POINT('Ctrl Pts',(1.3525703284343,1.,3.50408168106113));
#39230=CARTESIAN_POINT('Ctrl Pts',(1.35133076331065,-1.,3.50049707063673));
#39231=CARTESIAN_POINT('Ctrl Pts',(1.35133076331065,1.,3.50049707063673));
#39232=CARTESIAN_POINT('Ctrl Pts',(1.35067437417289,-1.,3.49888720256612));
#39233=CARTESIAN_POINT('Ctrl Pts',(1.35067437417289,1.,3.49888720256612));
#39234=CARTESIAN_POINT('Ctrl Pts',(1.35037650302887,-1.,3.49840357193384));
#39235=CARTESIAN_POINT('Ctrl Pts',(1.35037650302887,1.,3.49840357193384));
#39236=CARTESIAN_POINT('Ctrl Pts',(1.35026426118351,-1.,3.49840260053616));
#39237=CARTESIAN_POINT('Ctrl Pts',(1.35026426118351,1.,3.49840260053616));
#39238=CARTESIAN_POINT('Ctrl Pts',(1.35022972712301,-1.,3.49848248301936));
#39239=CARTESIAN_POINT('Ctrl Pts',(1.35022972712301,1.,3.49848248301936));
#39240=CARTESIAN_POINT('',(1.36999806084572,1.,3.97027773754922));
#39241=CARTESIAN_POINT('Ctrl Pts',(1.36999806084572,1.,3.97027773754922));
#39242=CARTESIAN_POINT('Ctrl Pts',(1.37020239094758,1.,3.9687184694173));
#39243=CARTESIAN_POINT('Ctrl Pts',(1.37060761746027,1.,3.96560037975788));
#39244=CARTESIAN_POINT('Ctrl Pts',(1.37120515615663,1.,3.96092458508407));
#39245=CARTESIAN_POINT('Ctrl Pts',(1.37198126433139,1.,3.95469287283105));
#39246=CARTESIAN_POINT('Ctrl Pts',(1.37291699203423,1.,3.94690771786926));
#39247=CARTESIAN_POINT('Ctrl Pts',(1.37381821967499,1.,3.93912709041791));
#39248=CARTESIAN_POINT('Ctrl Pts',(1.37468482215784,1.,3.93135106761941));
#39249=CARTESIAN_POINT('Ctrl Pts',(1.37551664448057,1.,3.92357976987132));
#39250=CARTESIAN_POINT('Ctrl Pts',(1.37631350505516,1.,3.91581337461825));
#39251=CARTESIAN_POINT('Ctrl Pts',(1.3770751963376,1.,3.90805209522729));
#39252=CARTESIAN_POINT('Ctrl Pts',(1.3778014851263,1.,3.90029615196255));
#39253=CARTESIAN_POINT('Ctrl Pts',(1.37849211287981,1.,3.89254574338385));
#39254=CARTESIAN_POINT('Ctrl Pts',(1.37914679719446,1.,3.88480102249461));
#39255=CARTESIAN_POINT('Ctrl Pts',(1.37976523097187,1.,3.87706205830865));
#39256=CARTESIAN_POINT('Ctrl Pts',(1.38034709213129,1.,3.86932885813403));
#39257=CARTESIAN_POINT('Ctrl Pts',(1.38089205993067,1.,3.86160143044187));
#39258=CARTESIAN_POINT('Ctrl Pts',(1.38139983115075,1.,3.85387983979557));
#39259=CARTESIAN_POINT('Ctrl Pts',(1.38187013346089,1.,3.84616425605705));
#39260=CARTESIAN_POINT('Ctrl Pts',(1.38230274828774,1.,3.83845502790609));
#39261=CARTESIAN_POINT('Ctrl Pts',(1.38269750245086,1.,3.83075266982138));
#39262=CARTESIAN_POINT('Ctrl Pts',(1.38305421262724,1.,3.82305771743715));
#39263=CARTESIAN_POINT('Ctrl Pts',(1.38337263902766,1.,3.81537060817765));
#39264=CARTESIAN_POINT('Ctrl Pts',(1.38365244046226,1.,3.80769156398429));
#39265=CARTESIAN_POINT('Ctrl Pts',(1.38389311766701,1.,3.80002044322169));
#39266=CARTESIAN_POINT('Ctrl Pts',(1.38409399694588,1.,3.79235669640907));
#39267=CARTESIAN_POINT('Ctrl Pts',(1.38425435883773,1.,3.78469969805134));
#39268=CARTESIAN_POINT('Ctrl Pts',(1.38437354551435,1.,3.77704902230441));
#39269=CARTESIAN_POINT('Ctrl Pts',(1.38445107339517,1.,3.76940473185775));
#39270=CARTESIAN_POINT('Ctrl Pts',(1.38448675253343,1.,3.76176768271347));
#39271=CARTESIAN_POINT('Ctrl Pts',(1.38448077997155,1.,3.75413976318727));
#39272=CARTESIAN_POINT('Ctrl Pts',(1.38443344984389,1.,3.7465231716786));
#39273=CARTESIAN_POINT('Ctrl Pts',(1.38434489156456,1.,3.73891976418099));
#39274=CARTESIAN_POINT('Ctrl Pts',(1.38421479111531,1.,3.73133035859283));
#39275=CARTESIAN_POINT('Ctrl Pts',(1.3840421342895,1.,3.72375409358805));
#39276=CARTESIAN_POINT('Ctrl Pts',(1.38382489984585,1.,3.7161876605181));
#39277=CARTESIAN_POINT('Ctrl Pts',(1.38356065402122,1.,3.70862680753343));
#39278=CARTESIAN_POINT('Ctrl Pts',(1.38324717612862,1.,3.70106792167894));
#39279=CARTESIAN_POINT('Ctrl Pts',(1.38288311171649,1.,3.69350967899523));
#39280=CARTESIAN_POINT('Ctrl Pts',(1.38246852827185,1.,3.68595444983844));
#39281=CARTESIAN_POINT('Ctrl Pts',(1.38200574290626,1.,3.6784103848243));
#39282=CARTESIAN_POINT('Ctrl Pts',(1.38149812653876,1.,3.67088843112282));
#39283=CARTESIAN_POINT('Ctrl Pts',(1.38094856333558,1.,3.66339848520874));
#39284=CARTESIAN_POINT('Ctrl Pts',(1.38035791051215,1.,3.65594554404396));
#39285=CARTESIAN_POINT('Ctrl Pts',(1.37972372481598,1.,3.64852652756444));
#39286=CARTESIAN_POINT('Ctrl Pts',(1.37903818567347,1.,3.64112507791112));
#39287=CARTESIAN_POINT('Ctrl Pts',(1.37829035457324,1.,3.63371727442448));
#39288=CARTESIAN_POINT('Ctrl Pts',(1.37746987919868,1.,3.62628098665112));
#39289=CARTESIAN_POINT('Ctrl Pts',(1.37657053403102,1.,3.61880481160408));
#39290=CARTESIAN_POINT('Ctrl Pts',(1.37559314436641,1.,3.61129546591082));
#39291=CARTESIAN_POINT('Ctrl Pts',(1.37455051379642,1.,3.60379020124038));
#39292=CARTESIAN_POINT('Ctrl Pts',(1.37346320103184,1.,3.59634627869117));
#39293=CARTESIAN_POINT('Ctrl Pts',(1.37235053661,1.,3.5890185384643));
#39294=CARTESIAN_POINT('Ctrl Pts',(1.37122241663073,1.,3.58183885982745));
#39295=CARTESIAN_POINT('Ctrl Pts',(1.37007229485646,1.,3.57479875549453));
#39296=CARTESIAN_POINT('Ctrl Pts',(1.36886584973349,1.,3.56782080304554));
#39297=CARTESIAN_POINT('Ctrl Pts',(1.36754771771174,1.,3.56077662028492));
#39298=CARTESIAN_POINT('Ctrl Pts',(1.36606145456711,1.,3.55353883995793));
#39299=CARTESIAN_POINT('Ctrl Pts',(1.36436666257567,1.,3.54602591832893));
#39300=CARTESIAN_POINT('Ctrl Pts',(1.36245507339334,1.,3.53824396425032));
#39301=CARTESIAN_POINT('Ctrl Pts',(1.36037259643827,1.,3.53034464961849));
#39302=CARTESIAN_POINT('Ctrl Pts',(1.35821701528975,1.,3.52261776117121));
#39303=CARTESIAN_POINT('Ctrl Pts',(1.35611275237288,1.,3.51542230699919));
#39304=CARTESIAN_POINT('Ctrl Pts',(1.35419113576022,1.,3.50913227060177));
#39305=CARTESIAN_POINT('Ctrl Pts',(1.3525703284343,1.,3.50408168106113));
#39306=CARTESIAN_POINT('Ctrl Pts',(1.35142377279535,1.,3.5007660381658));
#39307=CARTESIAN_POINT('Ctrl Pts',(1.35080045218652,1.,3.49920025459856));
#39308=CARTESIAN_POINT('Ctrl Pts',(1.35049736560633,1.,3.49861894124915));
#39309=CARTESIAN_POINT('Ctrl Pts',(1.35036670893102,1.,3.49847119623841));
#39310=CARTESIAN_POINT('Ctrl Pts',(1.35032489087269,1.,3.49844575334386));
#39311=CARTESIAN_POINT('',(1.36999806084572,0.,3.97027773754922));
#39312=CARTESIAN_POINT('Ctrl Pts',(0.96399761336957,-1.,3.62397690409552));
#39313=CARTESIAN_POINT('Ctrl Pts',(0.96399761336957,1.,3.62397690409552));
#39314=CARTESIAN_POINT('Ctrl Pts',(0.963922720982576,-1.,3.62393257642191));
#39315=CARTESIAN_POINT('Ctrl Pts',(0.963922720982576,1.,3.62393257642191));
#39316=CARTESIAN_POINT('Ctrl Pts',(0.963832486396055,-1.,3.62399933640277));
#39317=CARTESIAN_POINT('Ctrl Pts',(0.963832486396055,1.,3.62399933640277));
#39318=CARTESIAN_POINT('Ctrl Pts',(0.963875774532102,-1.,3.62456568607055));
#39319=CARTESIAN_POINT('Ctrl Pts',(0.963875774532102,1.,3.62456568607055));
#39320=CARTESIAN_POINT('Ctrl Pts',(0.964291001274618,-1.,3.62625391255277));
#39321=CARTESIAN_POINT('Ctrl Pts',(0.964291001274618,1.,3.62625391255277));
#39322=CARTESIAN_POINT('Ctrl Pts',(0.965395153165715,-1.,3.62988252139998));
#39323=CARTESIAN_POINT('Ctrl Pts',(0.965395153165715,1.,3.62988252139998));
#39324=CARTESIAN_POINT('Ctrl Pts',(0.967052554540877,-1.,3.6349212208096));
#39325=CARTESIAN_POINT('Ctrl Pts',(0.967052554540877,1.,3.6349212208096));
#39326=CARTESIAN_POINT('Ctrl Pts',(0.969195124674828,-1.,3.64113946505393));
#39327=CARTESIAN_POINT('Ctrl Pts',(0.969195124674828,1.,3.64113946505393));
#39328=CARTESIAN_POINT('Ctrl Pts',(0.971722122060277,-1.,3.64819756447072));
#39329=CARTESIAN_POINT('Ctrl Pts',(0.971722122060277,1.,3.64819756447072));
#39330=CARTESIAN_POINT('Ctrl Pts',(0.974519971354138,-1.,3.6557157673487));
#39331=CARTESIAN_POINT('Ctrl Pts',(0.974519971354138,1.,3.6557157673487));
#39332=CARTESIAN_POINT('Ctrl Pts',(0.977478312751416,-1.,3.66333049637403));
#39333=CARTESIAN_POINT('Ctrl Pts',(0.977478312751416,1.,3.66333049637403));
#39334=CARTESIAN_POINT('Ctrl Pts',(0.980505922458494,-1.,3.67074983340444));
#39335=CARTESIAN_POINT('Ctrl Pts',(0.980505922458494,1.,3.67074983340444));
#39336=CARTESIAN_POINT('Ctrl Pts',(0.983550791470864,-1.,3.67782408841876));
#39337=CARTESIAN_POINT('Ctrl Pts',(0.983550791470864,1.,3.67782408841876));
#39338=CARTESIAN_POINT('Ctrl Pts',(0.986602639864285,-1.,3.6845531792623));
#39339=CARTESIAN_POINT('Ctrl Pts',(0.986602639864285,1.,3.6845531792623));
#39340=CARTESIAN_POINT('Ctrl Pts',(0.989676715398858,-1.,3.69102682138955));
#39341=CARTESIAN_POINT('Ctrl Pts',(0.989676715398858,1.,3.69102682138955));
#39342=CARTESIAN_POINT('Ctrl Pts',(0.992802218332103,-1.,3.69738123415696));
#39343=CARTESIAN_POINT('Ctrl Pts',(0.992802218332103,1.,3.69738123415696));
#39344=CARTESIAN_POINT('Ctrl Pts',(0.996009819772431,-1.,3.70375282282107));
#39345=CARTESIAN_POINT('Ctrl Pts',(0.996009819772431,1.,3.70375282282107));
#39346=CARTESIAN_POINT('Ctrl Pts',(0.999317260756344,-1.,3.7102243971387));
#39347=CARTESIAN_POINT('Ctrl Pts',(0.999317260756344,1.,3.7102243971387));
#39348=CARTESIAN_POINT('Ctrl Pts',(1.00272423396802,-1.,3.71680667125047));
#39349=CARTESIAN_POINT('Ctrl Pts',(1.00272423396802,1.,3.71680667125047));
#39350=CARTESIAN_POINT('Ctrl Pts',(1.00622000735696,-1.,3.72346803750544));
#39351=CARTESIAN_POINT('Ctrl Pts',(1.00622000735696,1.,3.72346803750544));
#39352=CARTESIAN_POINT('Ctrl Pts',(1.00978798539491,-1.,3.73015276704407));
#39353=CARTESIAN_POINT('Ctrl Pts',(1.00978798539491,1.,3.73015276704407));
#39354=CARTESIAN_POINT('Ctrl Pts',(1.01341114319906,-1.,3.73680245055747));
#39355=CARTESIAN_POINT('Ctrl Pts',(1.01341114319906,1.,3.73680245055747));
#39356=CARTESIAN_POINT('Ctrl Pts',(1.01707794311088,-1.,3.74337942504993));
#39357=CARTESIAN_POINT('Ctrl Pts',(1.01707794311088,1.,3.74337942504993));
#39358=CARTESIAN_POINT('Ctrl Pts',(1.02078510487439,-1.,3.74987777155873));
#39359=CARTESIAN_POINT('Ctrl Pts',(1.02078510487439,1.,3.74987777155873));
#39360=CARTESIAN_POINT('Ctrl Pts',(1.02453429444668,-1.,3.75631037456224));
#39361=CARTESIAN_POINT('Ctrl Pts',(1.02453429444668,1.,3.75631037456224));
#39362=CARTESIAN_POINT('Ctrl Pts',(1.02833014458184,-1.,3.76270122291245));
#39363=CARTESIAN_POINT('Ctrl Pts',(1.02833014458184,1.,3.76270122291245));
#39364=CARTESIAN_POINT('Ctrl Pts',(1.03217786604919,-1.,3.76907609832516));
#39365=CARTESIAN_POINT('Ctrl Pts',(1.03217786604919,1.,3.76907609832516));
#39366=CARTESIAN_POINT('Ctrl Pts',(1.03608074678008,-1.,3.77545283140427));
#39367=CARTESIAN_POINT('Ctrl Pts',(1.03608074678008,1.,3.77545283140427));
#39368=CARTESIAN_POINT('Ctrl Pts',(1.04003862055798,-1.,3.7818353500817));
#39369=CARTESIAN_POINT('Ctrl Pts',(1.04003862055798,1.,3.7818353500817));
#39370=CARTESIAN_POINT('Ctrl Pts',(1.04404924374422,-1.,3.78821910787179));
#39371=CARTESIAN_POINT('Ctrl Pts',(1.04404924374422,1.,3.78821910787179));
#39372=CARTESIAN_POINT('Ctrl Pts',(1.04810913267639,-1.,3.79459440308786));
#39373=CARTESIAN_POINT('Ctrl Pts',(1.04810913267639,1.,3.79459440308786));
#39374=CARTESIAN_POINT('Ctrl Pts',(1.05221457990016,-1.,3.80095039790681));
#39375=CARTESIAN_POINT('Ctrl Pts',(1.05221457990016,1.,3.80095039790681));
#39376=CARTESIAN_POINT('Ctrl Pts',(1.05636266918644,-1.,3.80727913637791));
#39377=CARTESIAN_POINT('Ctrl Pts',(1.05636266918644,1.,3.80727913637791));
#39378=CARTESIAN_POINT('Ctrl Pts',(1.06055206187299,-1.,3.8135786611749));
#39379=CARTESIAN_POINT('Ctrl Pts',(1.06055206187299,1.,3.8135786611749));
#39380=CARTESIAN_POINT('Ctrl Pts',(1.0647824403893,-1.,3.81985083953012));
#39381=CARTESIAN_POINT('Ctrl Pts',(1.0647824403893,1.,3.81985083953012));
#39382=CARTESIAN_POINT('Ctrl Pts',(1.06905413180359,-1.,3.82609989967276));
#39383=CARTESIAN_POINT('Ctrl Pts',(1.06905413180359,1.,3.82609989967276));
#39384=CARTESIAN_POINT('Ctrl Pts',(1.07336766633459,-1.,3.83233071195144));
#39385=CARTESIAN_POINT('Ctrl Pts',(1.07336766633459,1.,3.83233071195144));
#39386=CARTESIAN_POINT('Ctrl Pts',(1.07772335353858,-1.,3.83854714117491));
#39387=CARTESIAN_POINT('Ctrl Pts',(1.07772335353858,1.,3.83854714117491));
#39388=CARTESIAN_POINT('Ctrl Pts',(1.08212087917991,-1.,3.8447504803063));
#39389=CARTESIAN_POINT('Ctrl Pts',(1.08212087917991,1.,3.8447504803063));
#39390=CARTESIAN_POINT('Ctrl Pts',(1.08655950846384,-1.,3.85094025222713));
#39391=CARTESIAN_POINT('Ctrl Pts',(1.08655950846384,1.,3.85094025222713));
#39392=CARTESIAN_POINT('Ctrl Pts',(1.09103825516294,-1.,3.85711487933931));
#39393=CARTESIAN_POINT('Ctrl Pts',(1.09103825516294,1.,3.85711487933931));
#39394=CARTESIAN_POINT('Ctrl Pts',(1.09555606505013,-1.,3.86327241021247));
#39395=CARTESIAN_POINT('Ctrl Pts',(1.09555606505013,1.,3.86327241021247));
#39396=CARTESIAN_POINT('Ctrl Pts',(1.10011198761195,-1.,3.86941120134849));
#39397=CARTESIAN_POINT('Ctrl Pts',(1.10011198761195,1.,3.86941120134849));
#39398=CARTESIAN_POINT('Ctrl Pts',(1.10470536603287,-1.,3.87553067187514));
#39399=CARTESIAN_POINT('Ctrl Pts',(1.10470536603287,1.,3.87553067187514));
#39400=CARTESIAN_POINT('Ctrl Pts',(1.10933577224008,-1.,3.88163105531724));
#39401=CARTESIAN_POINT('Ctrl Pts',(1.10933577224008,1.,3.88163105531724));
#39402=CARTESIAN_POINT('Ctrl Pts',(1.11400292434429,-1.,3.88771308285171));
#39403=CARTESIAN_POINT('Ctrl Pts',(1.11400292434429,1.,3.88771308285171));
#39404=CARTESIAN_POINT('Ctrl Pts',(1.11870660794603,-1.,3.89377768340344));
#39405=CARTESIAN_POINT('Ctrl Pts',(1.11870660794603,1.,3.89377768340344));
#39406=CARTESIAN_POINT('Ctrl Pts',(1.12344660099043,-1.,3.89982569750025));
#39407=CARTESIAN_POINT('Ctrl Pts',(1.12344660099043,1.,3.89982569750025));
#39408=CARTESIAN_POINT('Ctrl Pts',(1.12822258281553,-1.,3.90585753318737));
#39409=CARTESIAN_POINT('Ctrl Pts',(1.12822258281553,1.,3.90585753318737));
#39410=CARTESIAN_POINT('Ctrl Pts',(1.13303414693896,-1.,3.91187321145649));
#39411=CARTESIAN_POINT('Ctrl Pts',(1.13303414693896,1.,3.91187321145649));
#39412=CARTESIAN_POINT('Ctrl Pts',(1.13788084225554,-1.,3.91787251936827));
#39413=CARTESIAN_POINT('Ctrl Pts',(1.13788084225554,1.,3.91787251936827));
#39414=CARTESIAN_POINT('Ctrl Pts',(1.14276220561593,-1.,3.92385513133997));
#39415=CARTESIAN_POINT('Ctrl Pts',(1.14276220561593,1.,3.92385513133997));
#39416=CARTESIAN_POINT('Ctrl Pts',(1.14767779451123,-1.,3.92982073294257));
#39417=CARTESIAN_POINT('Ctrl Pts',(1.14767779451123,1.,3.92982073294257));
#39418=CARTESIAN_POINT('Ctrl Pts',(1.1526272271632,-1.,3.9357691705628));
#39419=CARTESIAN_POINT('Ctrl Pts',(1.1526272271632,1.,3.9357691705628));
#39420=CARTESIAN_POINT('Ctrl Pts',(1.15761018340956,-1.,3.94170046685203));
#39421=CARTESIAN_POINT('Ctrl Pts',(1.15761018340956,1.,3.94170046685203));
#39422=CARTESIAN_POINT('Ctrl Pts',(1.16262637999157,-1.,3.94761474780583));
#39423=CARTESIAN_POINT('Ctrl Pts',(1.16262637999157,1.,3.94761474780583));
#39424=CARTESIAN_POINT('Ctrl Pts',(1.16767555244438,-1.,3.95351219509876));
#39425=CARTESIAN_POINT('Ctrl Pts',(1.16767555244438,1.,3.95351219509876));
#39426=CARTESIAN_POINT('Ctrl Pts',(1.17275743590361,-1.,3.95939299213276));
#39427=CARTESIAN_POINT('Ctrl Pts',(1.17275743590361,1.,3.95939299213276));
#39428=CARTESIAN_POINT('Ctrl Pts',(1.17787174135592,-1.,3.96525726358159));
#39429=CARTESIAN_POINT('Ctrl Pts',(1.17787174135592,1.,3.96525726358159));
#39430=CARTESIAN_POINT('Ctrl Pts',(1.18301815039831,-1.,3.97110505165415));
#39431=CARTESIAN_POINT('Ctrl Pts',(1.18301815039831,1.,3.97110505165415));
#39432=CARTESIAN_POINT('Ctrl Pts',(1.18819633715539,-1.,3.97693634767754));
#39433=CARTESIAN_POINT('Ctrl Pts',(1.18819633715539,1.,3.97693634767754));
#39434=CARTESIAN_POINT('Ctrl Pts',(1.19340598349475,-1.,3.98275111052561));
#39435=CARTESIAN_POINT('Ctrl Pts',(1.19340598349475,1.,3.98275111052561));
#39436=CARTESIAN_POINT('Ctrl Pts',(1.19864679609566,-1.,3.98854928957189));
#39437=CARTESIAN_POINT('Ctrl Pts',(1.19864679609566,1.,3.98854928957189));
#39438=CARTESIAN_POINT('Ctrl Pts',(1.20391852375138,-1.,3.99433084799666));
#39439=CARTESIAN_POINT('Ctrl Pts',(1.20391852375138,1.,3.99433084799666));
#39440=CARTESIAN_POINT('Ctrl Pts',(1.20922097029551,-1.,4.00009577950721));
#39441=CARTESIAN_POINT('Ctrl Pts',(1.20922097029551,1.,4.00009577950721));
#39442=CARTESIAN_POINT('Ctrl Pts',(1.21455398918133,-1.,4.00584409522722));
#39443=CARTESIAN_POINT('Ctrl Pts',(1.21455398918133,1.,4.00584409522722));
#39444=CARTESIAN_POINT('Ctrl Pts',(1.21884478244403,-1.,4.01042947140789));
#39445=CARTESIAN_POINT('Ctrl Pts',(1.21884478244403,1.,4.01042947140789));
#39446=CARTESIAN_POINT('Ctrl Pts',(1.22207656455845,-1.,4.01386104433519));
#39447=CARTESIAN_POINT('Ctrl Pts',(1.22207656455845,1.,4.01386104433519));
#39448=CARTESIAN_POINT('Ctrl Pts',(1.22423716681317,-1.,4.01614544569895));
#39449=CARTESIAN_POINT('Ctrl Pts',(1.22423716681317,1.,4.01614544569895));
#39450=CARTESIAN_POINT('Ctrl Pts',(1.22531898815164,-1.,4.01728681790024));
#39451=CARTESIAN_POINT('Ctrl Pts',(1.22531898815164,1.,4.01728681790024));
#39452=CARTESIAN_POINT('',(0.963899035118985,1.,3.62400312501199));
#39453=CARTESIAN_POINT('Ctrl Pts',(0.963899035118985,-1.,3.62400312501199));
#39454=CARTESIAN_POINT('Ctrl Pts',(0.963899035118985,-0.666666666666667,
3.62400312501199));
#39455=CARTESIAN_POINT('Ctrl Pts',(0.963899035118985,-0.333333333333333,
3.62400312501199));
#39456=CARTESIAN_POINT('Ctrl Pts',(0.963899035118985,0.333333333333333,
3.62400312501199));
#39457=CARTESIAN_POINT('Ctrl Pts',(0.963899035118985,0.666666666666667,
3.62400312501199));
#39458=CARTESIAN_POINT('Ctrl Pts',(0.963899035118985,1.,3.62400312501199));
#39459=CARTESIAN_POINT('',(1.22531898815164,1.,4.01728681790024));
#39460=CARTESIAN_POINT('',(1.22531898815164,0.,4.01728681790024));
#39461=CARTESIAN_POINT('Ctrl Pts',(0.963899035118985,1.,3.62400312501199));
#39462=CARTESIAN_POINT('Ctrl Pts',(0.963880158556712,1.,3.62404828878375));
#39463=CARTESIAN_POINT('Ctrl Pts',(0.963861297423578,1.,3.62424461507455));
#39464=CARTESIAN_POINT('Ctrl Pts',(0.963957782642589,1.,3.62489305727516));
#39465=CARTESIAN_POINT('Ctrl Pts',(0.964373850166081,1.,3.62652618145252));
#39466=CARTESIAN_POINT('Ctrl Pts',(0.965395153165715,1.,3.62988252139998));
#39467=CARTESIAN_POINT('Ctrl Pts',(0.967052554540877,1.,3.6349212208096));
#39468=CARTESIAN_POINT('Ctrl Pts',(0.969195124674828,1.,3.64113946505393));
#39469=CARTESIAN_POINT('Ctrl Pts',(0.971722122060277,1.,3.64819756447072));
#39470=CARTESIAN_POINT('Ctrl Pts',(0.974519971354138,1.,3.6557157673487));
#39471=CARTESIAN_POINT('Ctrl Pts',(0.977478312751416,1.,3.66333049637403));
#39472=CARTESIAN_POINT('Ctrl Pts',(0.980505922458494,1.,3.67074983340444));
#39473=CARTESIAN_POINT('Ctrl Pts',(0.983550791470864,1.,3.67782408841876));
#39474=CARTESIAN_POINT('Ctrl Pts',(0.986602639864285,1.,3.6845531792623));
#39475=CARTESIAN_POINT('Ctrl Pts',(0.989676715398858,1.,3.69102682138955));
#39476=CARTESIAN_POINT('Ctrl Pts',(0.992802218332103,1.,3.69738123415696));
#39477=CARTESIAN_POINT('Ctrl Pts',(0.996009819772431,1.,3.70375282282107));
#39478=CARTESIAN_POINT('Ctrl Pts',(0.999317260756344,1.,3.7102243971387));
#39479=CARTESIAN_POINT('Ctrl Pts',(1.00272423396802,1.,3.71680667125047));
#39480=CARTESIAN_POINT('Ctrl Pts',(1.00622000735696,1.,3.72346803750544));
#39481=CARTESIAN_POINT('Ctrl Pts',(1.00978798539491,1.,3.73015276704407));
#39482=CARTESIAN_POINT('Ctrl Pts',(1.01341114319906,1.,3.73680245055747));
#39483=CARTESIAN_POINT('Ctrl Pts',(1.01707794311088,1.,3.74337942504993));
#39484=CARTESIAN_POINT('Ctrl Pts',(1.02078510487439,1.,3.74987777155873));
#39485=CARTESIAN_POINT('Ctrl Pts',(1.02453429444668,1.,3.75631037456224));
#39486=CARTESIAN_POINT('Ctrl Pts',(1.02833014458184,1.,3.76270122291245));
#39487=CARTESIAN_POINT('Ctrl Pts',(1.03217786604919,1.,3.76907609832516));
#39488=CARTESIAN_POINT('Ctrl Pts',(1.03608074678008,1.,3.77545283140427));
#39489=CARTESIAN_POINT('Ctrl Pts',(1.04003862055798,1.,3.7818353500817));
#39490=CARTESIAN_POINT('Ctrl Pts',(1.04404924374422,1.,3.78821910787179));
#39491=CARTESIAN_POINT('Ctrl Pts',(1.04810913267639,1.,3.79459440308786));
#39492=CARTESIAN_POINT('Ctrl Pts',(1.05221457990016,1.,3.80095039790681));
#39493=CARTESIAN_POINT('Ctrl Pts',(1.05636266918644,1.,3.80727913637791));
#39494=CARTESIAN_POINT('Ctrl Pts',(1.06055206187299,1.,3.8135786611749));
#39495=CARTESIAN_POINT('Ctrl Pts',(1.0647824403893,1.,3.81985083953012));
#39496=CARTESIAN_POINT('Ctrl Pts',(1.06905413180359,1.,3.82609989967276));
#39497=CARTESIAN_POINT('Ctrl Pts',(1.07336766633459,1.,3.83233071195144));
#39498=CARTESIAN_POINT('Ctrl Pts',(1.07772335353858,1.,3.83854714117491));
#39499=CARTESIAN_POINT('Ctrl Pts',(1.08212087917991,1.,3.8447504803063));
#39500=CARTESIAN_POINT('Ctrl Pts',(1.08655950846384,1.,3.85094025222713));
#39501=CARTESIAN_POINT('Ctrl Pts',(1.09103825516294,1.,3.85711487933931));
#39502=CARTESIAN_POINT('Ctrl Pts',(1.09555606505013,1.,3.86327241021247));
#39503=CARTESIAN_POINT('Ctrl Pts',(1.10011198761195,1.,3.86941120134849));
#39504=CARTESIAN_POINT('Ctrl Pts',(1.10470536603287,1.,3.87553067187514));
#39505=CARTESIAN_POINT('Ctrl Pts',(1.10933577224008,1.,3.88163105531724));
#39506=CARTESIAN_POINT('Ctrl Pts',(1.11400292434429,1.,3.88771308285171));
#39507=CARTESIAN_POINT('Ctrl Pts',(1.11870660794603,1.,3.89377768340344));
#39508=CARTESIAN_POINT('Ctrl Pts',(1.12344660099043,1.,3.89982569750025));
#39509=CARTESIAN_POINT('Ctrl Pts',(1.12822258281553,1.,3.90585753318737));
#39510=CARTESIAN_POINT('Ctrl Pts',(1.13303414693896,1.,3.91187321145649));
#39511=CARTESIAN_POINT('Ctrl Pts',(1.13788084225554,1.,3.91787251936827));
#39512=CARTESIAN_POINT('Ctrl Pts',(1.14276220561593,1.,3.92385513133997));
#39513=CARTESIAN_POINT('Ctrl Pts',(1.14767779451123,1.,3.92982073294257));
#39514=CARTESIAN_POINT('Ctrl Pts',(1.1526272271632,1.,3.9357691705628));
#39515=CARTESIAN_POINT('Ctrl Pts',(1.15761018340956,1.,3.94170046685203));
#39516=CARTESIAN_POINT('Ctrl Pts',(1.16262637999157,1.,3.94761474780583));
#39517=CARTESIAN_POINT('Ctrl Pts',(1.16767555244438,1.,3.95351219509876));
#39518=CARTESIAN_POINT('Ctrl Pts',(1.17275743590361,1.,3.95939299213276));
#39519=CARTESIAN_POINT('Ctrl Pts',(1.17787174135592,1.,3.96525726358159));
#39520=CARTESIAN_POINT('Ctrl Pts',(1.18301815039831,1.,3.97110505165415));
#39521=CARTESIAN_POINT('Ctrl Pts',(1.18819633715539,1.,3.97693634767754));
#39522=CARTESIAN_POINT('Ctrl Pts',(1.19340598349475,1.,3.98275111052561));
#39523=CARTESIAN_POINT('Ctrl Pts',(1.19864679609566,1.,3.98854928957189));
#39524=CARTESIAN_POINT('Ctrl Pts',(1.20391852375138,1.,3.99433084799666));
#39525=CARTESIAN_POINT('Ctrl Pts',(1.20922097029551,1.,4.00009577950721));
#39526=CARTESIAN_POINT('Ctrl Pts',(1.21455398918133,1.,4.00584409522722));
#39527=CARTESIAN_POINT('Ctrl Pts',(1.21884478244403,1.,4.01042947140789));
#39528=CARTESIAN_POINT('Ctrl Pts',(1.22207656455845,1.,4.01386104433519));
#39529=CARTESIAN_POINT('Ctrl Pts',(1.22423716681317,1.,4.01614544569895));
#39530=CARTESIAN_POINT('Ctrl Pts',(1.22531898815164,1.,4.01728681790024));
#39531=CARTESIAN_POINT('Origin',(1.22531898815164,0.,4.01728681790024));
#39532=CARTESIAN_POINT('',(1.36999806084572,1.,3.97027773754922));
#39533=CARTESIAN_POINT('Origin',(0.,0.,0.));
#39534=CARTESIAN_POINT('',(0.786422660833742,1.,3.66661143271648));
#39535=CARTESIAN_POINT('Origin',(0.,1.,0.));
#39536=CARTESIAN_POINT('Ctrl Pts',(0.786422660833742,1.,3.66661143271648));
#39537=CARTESIAN_POINT('Ctrl Pts',(0.786422660833742,0.666666666666667,
3.66661143271648));
#39538=CARTESIAN_POINT('Ctrl Pts',(0.786422660833742,0.333333333333333,
3.66661143271648));
#39539=CARTESIAN_POINT('Ctrl Pts',(0.786422660833742,-0.333333333333333,
3.66661143271648));
#39540=CARTESIAN_POINT('Ctrl Pts',(0.786422660833742,-0.666666666666667,
3.66661143271648));
#39541=CARTESIAN_POINT('Ctrl Pts',(0.786422660833742,-1.,3.66661143271648));
#39542=CARTESIAN_POINT('Ctrl Pts',(0.732042837400619,-1.,4.13571194405636));
#39543=CARTESIAN_POINT('Ctrl Pts',(0.732042837400619,1.,4.13571194405636));
#39544=CARTESIAN_POINT('Ctrl Pts',(0.732488575135925,-1.,4.13420383737278));
#39545=CARTESIAN_POINT('Ctrl Pts',(0.732488575135925,1.,4.13420383737278));
#39546=CARTESIAN_POINT('Ctrl Pts',(0.733376589325634,-1.,4.13118752796397));
#39547=CARTESIAN_POINT('Ctrl Pts',(0.733376589325634,1.,4.13118752796397));
#39548=CARTESIAN_POINT('Ctrl Pts',(0.734698226767512,-1.,4.12666277572794));
#39549=CARTESIAN_POINT('Ctrl Pts',(0.734698226767512,1.,4.12666277572794));
#39550=CARTESIAN_POINT('Ctrl Pts',(0.736439634335347,-1.,4.12062919626082));
#39551=CARTESIAN_POINT('Ctrl Pts',(0.736439634335347,1.,4.12062919626082));
#39552=CARTESIAN_POINT('Ctrl Pts',(0.738581708229118,-1.,4.11308626953795));
#39553=CARTESIAN_POINT('Ctrl Pts',(0.738581708229118,1.,4.11308626953795));
#39554=CARTESIAN_POINT('Ctrl Pts',(0.740688998555151,-1.,4.1055424175856));
#39555=CARTESIAN_POINT('Ctrl Pts',(0.740688998555151,1.,4.1055424175856));
#39556=CARTESIAN_POINT('Ctrl Pts',(0.742761369690017,-1.,4.09799769702712));
#39557=CARTESIAN_POINT('Ctrl Pts',(0.742761369690017,1.,4.09799769702712));
#39558=CARTESIAN_POINT('Ctrl Pts',(0.744798649705513,-1.,4.09045220253011));
#39559=CARTESIAN_POINT('Ctrl Pts',(0.744798649705513,1.,4.09045220253011));
#39560=CARTESIAN_POINT('Ctrl Pts',(0.746800631490821,-1.,4.08290608094789));
#39561=CARTESIAN_POINT('Ctrl Pts',(0.746800631490821,1.,4.08290608094789));
#39562=CARTESIAN_POINT('Ctrl Pts',(0.748767076679176,-1.,4.07535951055363));
#39563=CARTESIAN_POINT('Ctrl Pts',(0.748767076679176,1.,4.07535951055363));
#39564=CARTESIAN_POINT('Ctrl Pts',(0.750697720483175,-1.,4.06781267241886));
#39565=CARTESIAN_POINT('Ctrl Pts',(0.750697720483175,1.,4.06781267241886));
#39566=CARTESIAN_POINT('Ctrl Pts',(0.752592276482868,-1.,4.06026572221399));
#39567=CARTESIAN_POINT('Ctrl Pts',(0.752592276482868,1.,4.06026572221399));
#39568=CARTESIAN_POINT('Ctrl Pts',(0.754450441816411,-1.,4.05271876688106));
#39569=CARTESIAN_POINT('Ctrl Pts',(0.754450441816411,1.,4.05271876688106));
#39570=CARTESIAN_POINT('Ctrl Pts',(0.756271902370186,-1.,4.04517182654344));
#39571=CARTESIAN_POINT('Ctrl Pts',(0.756271902370186,1.,4.04517182654344));
#39572=CARTESIAN_POINT('Ctrl Pts',(0.758056338885553,-1.,4.03762485803468));
#39573=CARTESIAN_POINT('Ctrl Pts',(0.758056338885553,1.,4.03762485803468));
#39574=CARTESIAN_POINT('Ctrl Pts',(0.759803433244165,-1.,4.0300778195465));
#39575=CARTESIAN_POINT('Ctrl Pts',(0.759803433244165,1.,4.0300778195465));
#39576=CARTESIAN_POINT('Ctrl Pts',(0.761512875859941,-1.,4.02253072741347));
#39577=CARTESIAN_POINT('Ctrl Pts',(0.761512875859941,1.,4.02253072741347));
#39578=CARTESIAN_POINT('Ctrl Pts',(0.763184371182826,-1.,4.01498370680434));
#39579=CARTESIAN_POINT('Ctrl Pts',(0.763184371182826,1.,4.01498370680434));
#39580=CARTESIAN_POINT('Ctrl Pts',(0.764817648784946,-1.,4.00743706791366));
#39581=CARTESIAN_POINT('Ctrl Pts',(0.764817648784946,1.,4.00743706791366));
#39582=CARTESIAN_POINT('Ctrl Pts',(0.766412457135785,-1.,3.99989129179464));
#39583=CARTESIAN_POINT('Ctrl Pts',(0.766412457135785,1.,3.99989129179464));
#39584=CARTESIAN_POINT('Ctrl Pts',(0.767968531377707,-1.,3.99234687880892));
#39585=CARTESIAN_POINT('Ctrl Pts',(0.767968531377707,1.,3.99234687880892));
#39586=CARTESIAN_POINT('Ctrl Pts',(0.769485566245459,-1.,3.98480422348403));
#39587=CARTESIAN_POINT('Ctrl Pts',(0.769485566245459,1.,3.98480422348403));
#39588=CARTESIAN_POINT('Ctrl Pts',(0.770963190030503,-1.,3.97726349165507));
#39589=CARTESIAN_POINT('Ctrl Pts',(0.770963190030503,1.,3.97726349165507));
#39590=CARTESIAN_POINT('Ctrl Pts',(0.772400931772238,-1.,3.96972446532832));
#39591=CARTESIAN_POINT('Ctrl Pts',(0.772400931772238,1.,3.96972446532832));
#39592=CARTESIAN_POINT('Ctrl Pts',(0.773798212026682,-1.,3.96218649639876));
#39593=CARTESIAN_POINT('Ctrl Pts',(0.773798212026682,1.,3.96218649639876));
#39594=CARTESIAN_POINT('Ctrl Pts',(0.775154418039441,-1.,3.95464885452364));
#39595=CARTESIAN_POINT('Ctrl Pts',(0.775154418039441,1.,3.95464885452364));
#39596=CARTESIAN_POINT('Ctrl Pts',(0.776468966697959,-1.,3.94711101619471));
#39597=CARTESIAN_POINT('Ctrl Pts',(0.776468966697959,1.,3.94711101619471));
#39598=CARTESIAN_POINT('Ctrl Pts',(0.777741370568549,-1.,3.93957296768098));
#39599=CARTESIAN_POINT('Ctrl Pts',(0.777741370568549,1.,3.93957296768098));
#39600=CARTESIAN_POINT('Ctrl Pts',(0.778971308134786,-1.,3.93203552473153));
#39601=CARTESIAN_POINT('Ctrl Pts',(0.778971308134786,1.,3.93203552473153));
#39602=CARTESIAN_POINT('Ctrl Pts',(0.780158678615506,-1.,3.92450058323799));
#39603=CARTESIAN_POINT('Ctrl Pts',(0.780158678615506,1.,3.92450058323799));
#39604=CARTESIAN_POINT('Ctrl Pts',(0.781303428618343,-1.,3.9169703605466));
#39605=CARTESIAN_POINT('Ctrl Pts',(0.781303428618343,1.,3.9169703605466));
#39606=CARTESIAN_POINT('Ctrl Pts',(0.782405395622758,-1.,3.90944671004536));
#39607=CARTESIAN_POINT('Ctrl Pts',(0.782405395622758,1.,3.90944671004536));
#39608=CARTESIAN_POINT('Ctrl Pts',(0.783464141529082,-1.,3.90193039043971));
#39609=CARTESIAN_POINT('Ctrl Pts',(0.783464141529082,1.,3.90193039043971));
#39610=CARTESIAN_POINT('Ctrl Pts',(0.784478799358335,-1.,3.89442039235105));
#39611=CARTESIAN_POINT('Ctrl Pts',(0.784478799358335,1.,3.89442039235105));
#39612=CARTESIAN_POINT('Ctrl Pts',(0.785447890340723,-1.,3.88691313167399));
#39613=CARTESIAN_POINT('Ctrl Pts',(0.785447890340723,1.,3.88691313167399));
#39614=CARTESIAN_POINT('Ctrl Pts',(0.786369675812591,-1.,3.87940402818186));
#39615=CARTESIAN_POINT('Ctrl Pts',(0.786369675812591,1.,3.87940402818186));
#39616=CARTESIAN_POINT('Ctrl Pts',(0.78724252761798,-1.,3.87188916600905));
#39617=CARTESIAN_POINT('Ctrl Pts',(0.78724252761798,1.,3.87188916600905));
#39618=CARTESIAN_POINT('Ctrl Pts',(0.78806531509377,-1.,3.86436702561342));
#39619=CARTESIAN_POINT('Ctrl Pts',(0.78806531509377,1.,3.86436702561342));
#39620=CARTESIAN_POINT('Ctrl Pts',(0.788837734090688,-1.,3.85683995872536));
#39621=CARTESIAN_POINT('Ctrl Pts',(0.788837734090688,1.,3.85683995872536));
#39622=CARTESIAN_POINT('Ctrl Pts',(0.789560798155618,-1.,3.8493163780891));
#39623=CARTESIAN_POINT('Ctrl Pts',(0.789560798155618,1.,3.8493163780891));
#39624=CARTESIAN_POINT('Ctrl Pts',(0.790236124191289,-1.,3.84180762342476));
#39625=CARTESIAN_POINT('Ctrl Pts',(0.790236124191289,1.,3.84180762342476));
#39626=CARTESIAN_POINT('Ctrl Pts',(0.790865012705339,-1.,3.83432392054804));
#39627=CARTESIAN_POINT('Ctrl Pts',(0.790865012705339,1.,3.83432392054804));
#39628=CARTESIAN_POINT('Ctrl Pts',(0.791447528662381,-1.,3.82687033899799));
#39629=CARTESIAN_POINT('Ctrl Pts',(0.791447528662381,1.,3.82687033899799));
#39630=CARTESIAN_POINT('Ctrl Pts',(0.791981740718606,-1.,3.81944345442237));
#39631=CARTESIAN_POINT('Ctrl Pts',(0.791981740718606,1.,3.81944345442237));
#39632=CARTESIAN_POINT('Ctrl Pts',(0.792462483517568,-1.,3.81202588694726));
#39633=CARTESIAN_POINT('Ctrl Pts',(0.792462483517568,1.,3.81202588694726));
#39634=CARTESIAN_POINT('Ctrl Pts',(0.792882695234692,-1.,3.80459229925598));
#39635=CARTESIAN_POINT('Ctrl Pts',(0.792882695234692,1.,3.80459229925598));
#39636=CARTESIAN_POINT('Ctrl Pts',(0.7932356129732,-1.,3.79711921389862));
#39637=CARTESIAN_POINT('Ctrl Pts',(0.7932356129732,1.,3.79711921389862));
#39638=CARTESIAN_POINT('Ctrl Pts',(0.793516871680965,-1.,3.78959439439222));
#39639=CARTESIAN_POINT('Ctrl Pts',(0.793516871680965,1.,3.78959439439222));
#39640=CARTESIAN_POINT('Ctrl Pts',(0.793726235781339,-1.,3.78202460377617));
#39641=CARTESIAN_POINT('Ctrl Pts',(0.793726235781339,1.,3.78202460377617));
#39642=CARTESIAN_POINT('Ctrl Pts',(0.793870523787515,-1.,3.77444863801264));
#39643=CARTESIAN_POINT('Ctrl Pts',(0.793870523787515,1.,3.77444863801264));
#39644=CARTESIAN_POINT('Ctrl Pts',(0.793961083689141,-1.,3.76692626931184));
#39645=CARTESIAN_POINT('Ctrl Pts',(0.793961083689141,1.,3.76692626931184));
#39646=CARTESIAN_POINT('Ctrl Pts',(0.794008429135046,-1.,3.75951468666325));
#39647=CARTESIAN_POINT('Ctrl Pts',(0.794008429135046,1.,3.75951468666325));
#39648=CARTESIAN_POINT('Ctrl Pts',(0.79401734737144,-1.,3.75224692493895));
#39649=CARTESIAN_POINT('Ctrl Pts',(0.79401734737144,1.,3.75224692493895));
#39650=CARTESIAN_POINT('Ctrl Pts',(0.79398270045988,-1.,3.74511357728827));
#39651=CARTESIAN_POINT('Ctrl Pts',(0.79398270045988,1.,3.74511357728827));
#39652=CARTESIAN_POINT('Ctrl Pts',(0.79388270093679,-1.,3.73803280541576));
#39653=CARTESIAN_POINT('Ctrl Pts',(0.79388270093679,1.,3.73803280541576));
#39654=CARTESIAN_POINT('Ctrl Pts',(0.793682750269347,-1.,3.7308691469564));
#39655=CARTESIAN_POINT('Ctrl Pts',(0.793682750269347,1.,3.7308691469564));
#39656=CARTESIAN_POINT('Ctrl Pts',(0.79334702378387,-1.,3.7234879729357));
#39657=CARTESIAN_POINT('Ctrl Pts',(0.79334702378387,1.,3.7234879729357));
#39658=CARTESIAN_POINT('Ctrl Pts',(0.792848377370115,-1.,3.7158024239604));
#39659=CARTESIAN_POINT('Ctrl Pts',(0.792848377370115,1.,3.7158024239604));
#39660=CARTESIAN_POINT('Ctrl Pts',(0.792177688845967,-1.,3.70781724021879));
#39661=CARTESIAN_POINT('Ctrl Pts',(0.792177688845967,1.,3.70781724021879));
#39662=CARTESIAN_POINT('Ctrl Pts',(0.791356575696508,-1.,3.69968940808982));
#39663=CARTESIAN_POINT('Ctrl Pts',(0.791356575696508,1.,3.69968940808982));
#39664=CARTESIAN_POINT('Ctrl Pts',(0.790436284989579,-1.,3.69172044327754));
#39665=CARTESIAN_POINT('Ctrl Pts',(0.790436284989579,1.,3.69172044327754));
#39666=CARTESIAN_POINT('Ctrl Pts',(0.789483546065158,-1.,3.68428439784285));
#39667=CARTESIAN_POINT('Ctrl Pts',(0.789483546065158,1.,3.68428439784285));
#39668=CARTESIAN_POINT('Ctrl Pts',(0.788569566220662,-1.,3.67777119516438));
#39669=CARTESIAN_POINT('Ctrl Pts',(0.788569566220662,1.,3.67777119516438));
#39670=CARTESIAN_POINT('Ctrl Pts',(0.787758799995426,-1.,3.672529236635));
#39671=CARTESIAN_POINT('Ctrl Pts',(0.787758799995426,1.,3.672529236635));
#39672=CARTESIAN_POINT('Ctrl Pts',(0.787095252589507,-1.,3.66879484800625));
#39673=CARTESIAN_POINT('Ctrl Pts',(0.787095252589507,1.,3.66879484800625));
#39674=CARTESIAN_POINT('Ctrl Pts',(0.786698783541657,-1.,3.66710211819938));
#39675=CARTESIAN_POINT('Ctrl Pts',(0.786698783541657,1.,3.66710211819938));
#39676=CARTESIAN_POINT('Ctrl Pts',(0.786480236184947,-1.,3.66657784454965));
#39677=CARTESIAN_POINT('Ctrl Pts',(0.786480236184947,1.,3.66657784454965));
#39678=CARTESIAN_POINT('Ctrl Pts',(0.786369528183039,-1.,3.66655932661846));
#39679=CARTESIAN_POINT('Ctrl Pts',(0.786369528183039,1.,3.66655932661846));
#39680=CARTESIAN_POINT('Ctrl Pts',(0.786322922920599,-1.,3.66663282329846));
#39681=CARTESIAN_POINT('Ctrl Pts',(0.786322922920599,1.,3.66663282329846));
#39682=CARTESIAN_POINT('',(0.732042837400619,1.,4.13571194405636));
#39683=CARTESIAN_POINT('Ctrl Pts',(0.732042837400619,1.,4.13571194405636));
#39684=CARTESIAN_POINT('Ctrl Pts',(0.732488575135925,1.,4.13420383737278));
#39685=CARTESIAN_POINT('Ctrl Pts',(0.733376589325634,1.,4.13118752796397));
#39686=CARTESIAN_POINT('Ctrl Pts',(0.734698226767512,1.,4.12666277572794));
#39687=CARTESIAN_POINT('Ctrl Pts',(0.736439634335347,1.,4.12062919626082));
#39688=CARTESIAN_POINT('Ctrl Pts',(0.738581708229118,1.,4.11308626953795));
#39689=CARTESIAN_POINT('Ctrl Pts',(0.740688998555151,1.,4.1055424175856));
#39690=CARTESIAN_POINT('Ctrl Pts',(0.742761369690017,1.,4.09799769702712));
#39691=CARTESIAN_POINT('Ctrl Pts',(0.744798649705513,1.,4.09045220253011));
#39692=CARTESIAN_POINT('Ctrl Pts',(0.746800631490821,1.,4.08290608094789));
#39693=CARTESIAN_POINT('Ctrl Pts',(0.748767076679176,1.,4.07535951055363));
#39694=CARTESIAN_POINT('Ctrl Pts',(0.750697720483175,1.,4.06781267241886));
#39695=CARTESIAN_POINT('Ctrl Pts',(0.752592276482868,1.,4.06026572221399));
#39696=CARTESIAN_POINT('Ctrl Pts',(0.754450441816411,1.,4.05271876688106));
#39697=CARTESIAN_POINT('Ctrl Pts',(0.756271902370186,1.,4.04517182654344));
#39698=CARTESIAN_POINT('Ctrl Pts',(0.758056338885553,1.,4.03762485803468));
#39699=CARTESIAN_POINT('Ctrl Pts',(0.759803433244165,1.,4.0300778195465));
#39700=CARTESIAN_POINT('Ctrl Pts',(0.761512875859941,1.,4.02253072741347));
#39701=CARTESIAN_POINT('Ctrl Pts',(0.763184371182826,1.,4.01498370680434));
#39702=CARTESIAN_POINT('Ctrl Pts',(0.764817648784946,1.,4.00743706791366));
#39703=CARTESIAN_POINT('Ctrl Pts',(0.766412457135785,1.,3.99989129179464));
#39704=CARTESIAN_POINT('Ctrl Pts',(0.767968531377707,1.,3.99234687880892));
#39705=CARTESIAN_POINT('Ctrl Pts',(0.769485566245459,1.,3.98480422348403));
#39706=CARTESIAN_POINT('Ctrl Pts',(0.770963190030503,1.,3.97726349165507));
#39707=CARTESIAN_POINT('Ctrl Pts',(0.772400931772238,1.,3.96972446532832));
#39708=CARTESIAN_POINT('Ctrl Pts',(0.773798212026682,1.,3.96218649639876));
#39709=CARTESIAN_POINT('Ctrl Pts',(0.775154418039441,1.,3.95464885452364));
#39710=CARTESIAN_POINT('Ctrl Pts',(0.776468966697959,1.,3.94711101619471));
#39711=CARTESIAN_POINT('Ctrl Pts',(0.777741370568549,1.,3.93957296768098));
#39712=CARTESIAN_POINT('Ctrl Pts',(0.778971308134786,1.,3.93203552473153));
#39713=CARTESIAN_POINT('Ctrl Pts',(0.780158678615506,1.,3.92450058323799));
#39714=CARTESIAN_POINT('Ctrl Pts',(0.781303428618343,1.,3.9169703605466));
#39715=CARTESIAN_POINT('Ctrl Pts',(0.782405395622758,1.,3.90944671004536));
#39716=CARTESIAN_POINT('Ctrl Pts',(0.783464141529082,1.,3.90193039043971));
#39717=CARTESIAN_POINT('Ctrl Pts',(0.784478799358335,1.,3.89442039235105));
#39718=CARTESIAN_POINT('Ctrl Pts',(0.785447890340723,1.,3.88691313167399));
#39719=CARTESIAN_POINT('Ctrl Pts',(0.786369675812591,1.,3.87940402818186));
#39720=CARTESIAN_POINT('Ctrl Pts',(0.78724252761798,1.,3.87188916600905));
#39721=CARTESIAN_POINT('Ctrl Pts',(0.78806531509377,1.,3.86436702561342));
#39722=CARTESIAN_POINT('Ctrl Pts',(0.788837734090688,1.,3.85683995872536));
#39723=CARTESIAN_POINT('Ctrl Pts',(0.789560798155618,1.,3.8493163780891));
#39724=CARTESIAN_POINT('Ctrl Pts',(0.790236124191289,1.,3.84180762342476));
#39725=CARTESIAN_POINT('Ctrl Pts',(0.790865012705339,1.,3.83432392054804));
#39726=CARTESIAN_POINT('Ctrl Pts',(0.791447528662381,1.,3.82687033899799));
#39727=CARTESIAN_POINT('Ctrl Pts',(0.791981740718606,1.,3.81944345442237));
#39728=CARTESIAN_POINT('Ctrl Pts',(0.792462483517568,1.,3.81202588694726));
#39729=CARTESIAN_POINT('Ctrl Pts',(0.792882695234692,1.,3.80459229925598));
#39730=CARTESIAN_POINT('Ctrl Pts',(0.7932356129732,1.,3.79711921389862));
#39731=CARTESIAN_POINT('Ctrl Pts',(0.793516871680965,1.,3.78959439439222));
#39732=CARTESIAN_POINT('Ctrl Pts',(0.793726235781339,1.,3.78202460377617));
#39733=CARTESIAN_POINT('Ctrl Pts',(0.793870523787515,1.,3.77444863801264));
#39734=CARTESIAN_POINT('Ctrl Pts',(0.793961083689141,1.,3.76692626931184));
#39735=CARTESIAN_POINT('Ctrl Pts',(0.794008429135046,1.,3.75951468666325));
#39736=CARTESIAN_POINT('Ctrl Pts',(0.79401734737144,1.,3.75224692493895));
#39737=CARTESIAN_POINT('Ctrl Pts',(0.79398270045988,1.,3.74511357728827));
#39738=CARTESIAN_POINT('Ctrl Pts',(0.79388270093679,1.,3.73803280541576));
#39739=CARTESIAN_POINT('Ctrl Pts',(0.793682750269347,1.,3.7308691469564));
#39740=CARTESIAN_POINT('Ctrl Pts',(0.79334702378387,1.,3.7234879729357));
#39741=CARTESIAN_POINT('Ctrl Pts',(0.792848377370115,1.,3.7158024239604));
#39742=CARTESIAN_POINT('Ctrl Pts',(0.792177688845967,1.,3.70781724021879));
#39743=CARTESIAN_POINT('Ctrl Pts',(0.791356575696508,1.,3.69968940808982));
#39744=CARTESIAN_POINT('Ctrl Pts',(0.790436284989579,1.,3.69172044327754));
#39745=CARTESIAN_POINT('Ctrl Pts',(0.789483546065158,1.,3.68428439784285));
#39746=CARTESIAN_POINT('Ctrl Pts',(0.788569566220662,1.,3.67777119516438));
#39747=CARTESIAN_POINT('Ctrl Pts',(0.787758799995426,1.,3.672529236635));
#39748=CARTESIAN_POINT('Ctrl Pts',(0.787145041181588,1.,3.66907505398769));
#39749=CARTESIAN_POINT('Ctrl Pts',(0.786774337198499,1.,3.66743103898844));
#39750=CARTESIAN_POINT('Ctrl Pts',(0.786565919559889,1.,3.66680946938396));
#39751=CARTESIAN_POINT('Ctrl Pts',(0.786459983896781,1.,3.66664310415236));
#39752=CARTESIAN_POINT('Ctrl Pts',(0.786422660833743,1.,3.66661143271648));
#39753=CARTESIAN_POINT('',(0.732042837400619,0.,4.13571194405636));
#39754=CARTESIAN_POINT('Ctrl Pts',(0.385214314776328,-1.,3.73016218570874));
#39755=CARTESIAN_POINT('Ctrl Pts',(0.385214314776328,1.,3.73016218570874));
#39756=CARTESIAN_POINT('Ctrl Pts',(0.385147278814803,-1.,3.73010668803185));
#39757=CARTESIAN_POINT('Ctrl Pts',(0.385147278814803,1.,3.73010668803185));
#39758=CARTESIAN_POINT('Ctrl Pts',(0.385047711603887,-1.,3.73015851028729));
#39759=CARTESIAN_POINT('Ctrl Pts',(0.385047711603887,1.,3.73015851028729));
#39760=CARTESIAN_POINT('Ctrl Pts',(0.385001870183841,-1.,3.73072465900727));
#39761=CARTESIAN_POINT('Ctrl Pts',(0.385001870183841,1.,3.73072465900727));
#39762=CARTESIAN_POINT('Ctrl Pts',(0.385147887989514,-1.,3.73245705639337));
#39763=CARTESIAN_POINT('Ctrl Pts',(0.385147887989514,1.,3.73245705639337));
#39764=CARTESIAN_POINT('Ctrl Pts',(0.385670806454744,-1.,3.73621371845475));
#39765=CARTESIAN_POINT('Ctrl Pts',(0.385670806454744,1.,3.73621371845475));
#39766=CARTESIAN_POINT('Ctrl Pts',(0.386519576222035,-1.,3.74144965781088));
#39767=CARTESIAN_POINT('Ctrl Pts',(0.386519576222035,1.,3.74144965781088));
#39768=CARTESIAN_POINT('Ctrl Pts',(0.387663020050396,-1.,3.74792651696269));
#39769=CARTESIAN_POINT('Ctrl Pts',(0.387663020050396,1.,3.74792651696269));
#39770=CARTESIAN_POINT('Ctrl Pts',(0.38905477589825,-1.,3.75529302894757));
#39771=CARTESIAN_POINT('Ctrl Pts',(0.38905477589825,1.,3.75529302894757));
#39772=CARTESIAN_POINT('Ctrl Pts',(0.390642072979258,-1.,3.76315635032993));
#39773=CARTESIAN_POINT('Ctrl Pts',(0.390642072979258,1.,3.76315635032993));
#39774=CARTESIAN_POINT('Ctrl Pts',(0.392372786223346,-1.,3.77114011595892));
#39775=CARTESIAN_POINT('Ctrl Pts',(0.392372786223346,1.,3.77114011595892));
#39776=CARTESIAN_POINT('Ctrl Pts',(0.394202481011595,-1.,3.77894173114368));
#39777=CARTESIAN_POINT('Ctrl Pts',(0.394202481011595,1.,3.77894173114368));
#39778=CARTESIAN_POINT('Ctrl Pts',(0.396103205335028,-1.,3.78640521279479));
#39779=CARTESIAN_POINT('Ctrl Pts',(0.396103205335028,1.,3.78640521279479));
#39780=CARTESIAN_POINT('Ctrl Pts',(0.398064818684158,-1.,3.79352887163457));
#39781=CARTESIAN_POINT('Ctrl Pts',(0.398064818684158,1.,3.79352887163457));
#39782=CARTESIAN_POINT('Ctrl Pts',(0.400088346504726,-1.,3.80040370384659));
#39783=CARTESIAN_POINT('Ctrl Pts',(0.400088346504726,1.,3.80040370384659));
#39784=CARTESIAN_POINT('Ctrl Pts',(0.402181320148474,-1.,3.80716881962763));
#39785=CARTESIAN_POINT('Ctrl Pts',(0.402181320148474,1.,3.80716881962763));
#39786=CARTESIAN_POINT('Ctrl Pts',(0.404352694628236,-1.,3.81396374287762));
#39787=CARTESIAN_POINT('Ctrl Pts',(0.404352694628236,1.,3.81396374287762));
#39788=CARTESIAN_POINT('Ctrl Pts',(0.406607038258906,-1.,3.82087303913741));
#39789=CARTESIAN_POINT('Ctrl Pts',(0.406607038258906,1.,3.82087303913741));
#39790=CARTESIAN_POINT('Ctrl Pts',(0.408942371447376,-1.,3.82790724256397));
#39791=CARTESIAN_POINT('Ctrl Pts',(0.408942371447376,1.,3.82790724256397));
#39792=CARTESIAN_POINT('Ctrl Pts',(0.411353038798459,-1.,3.83503345578645));
#39793=CARTESIAN_POINT('Ctrl Pts',(0.411353038798459,1.,3.83503345578645));
#39794=CARTESIAN_POINT('Ctrl Pts',(0.413831367016726,-1.,3.84219403994742));
#39795=CARTESIAN_POINT('Ctrl Pts',(0.413831367016726,1.,3.84219403994742));
#39796=CARTESIAN_POINT('Ctrl Pts',(0.41636967805292,-1.,3.8493286415751));
#39797=CARTESIAN_POINT('Ctrl Pts',(0.41636967805292,1.,3.8493286415751));
#39798=CARTESIAN_POINT('Ctrl Pts',(0.418962468086809,-1.,3.85639825648031));
#39799=CARTESIAN_POINT('Ctrl Pts',(0.418962468086809,1.,3.85639825648031));
#39800=CARTESIAN_POINT('Ctrl Pts',(0.421607423177575,-1.,3.86339652542749));
#39801=CARTESIAN_POINT('Ctrl Pts',(0.421607423177575,1.,3.86339652542749));
#39802=CARTESIAN_POINT('Ctrl Pts',(0.424304173195142,-1.,3.87033643487882));
#39803=CARTESIAN_POINT('Ctrl Pts',(0.424304173195142,1.,3.87033643487882));
#39804=CARTESIAN_POINT('Ctrl Pts',(0.427053541173469,-1.,3.87724240306609));
#39805=CARTESIAN_POINT('Ctrl Pts',(0.427053541173469,1.,3.87724240306609));
#39806=CARTESIAN_POINT('Ctrl Pts',(0.429856640579733,-1.,3.88414070943334));
#39807=CARTESIAN_POINT('Ctrl Pts',(0.429856640579733,1.,3.88414070943334));
#39808=CARTESIAN_POINT('Ctrl Pts',(0.432713929544439,-1.,3.89104947940592));
#39809=CARTESIAN_POINT('Ctrl Pts',(0.432713929544439,1.,3.89104947940592));
#39810=CARTESIAN_POINT('Ctrl Pts',(0.435624629433505,-1.,3.8979725665544));
#39811=CARTESIAN_POINT('Ctrl Pts',(0.435624629433505,1.,3.8979725665544));
#39812=CARTESIAN_POINT('Ctrl Pts',(0.438587235458233,-1.,3.90490512938546));
#39813=CARTESIAN_POINT('Ctrl Pts',(0.438587235458233,1.,3.90490512938546));
#39814=CARTESIAN_POINT('Ctrl Pts',(0.441599824524047,-1.,3.91183704069146));
#39815=CARTESIAN_POINT('Ctrl Pts',(0.441599824524047,1.,3.91183704069146));
#39816=CARTESIAN_POINT('Ctrl Pts',(0.444660430230592,-1.,3.91875701610721));
#39817=CARTESIAN_POINT('Ctrl Pts',(0.444660430230592,1.,3.91875701610721));
#39818=CARTESIAN_POINT('Ctrl Pts',(0.447767416837296,-1.,3.92565674143424));
#39819=CARTESIAN_POINT('Ctrl Pts',(0.447767416837296,1.,3.92565674143424));
#39820=CARTESIAN_POINT('Ctrl Pts',(0.450919768356346,-1.,3.93253407403128));
#39821=CARTESIAN_POINT('Ctrl Pts',(0.450919768356346,1.,3.93253407403128));
#39822=CARTESIAN_POINT('Ctrl Pts',(0.454116879027575,-1.,3.93939080846298));
#39823=CARTESIAN_POINT('Ctrl Pts',(0.454116879027575,1.,3.93939080846298));
#39824=CARTESIAN_POINT('Ctrl Pts',(0.457358410451673,-1.,3.94623117206675));
#39825=CARTESIAN_POINT('Ctrl Pts',(0.457358410451673,1.,3.94623117206675));
#39826=CARTESIAN_POINT('Ctrl Pts',(0.460644124429119,-1.,3.95306005817363));
#39827=CARTESIAN_POINT('Ctrl Pts',(0.460644124429119,1.,3.95306005817363));
#39828=CARTESIAN_POINT('Ctrl Pts',(0.463973722115744,-1.,3.95988133243543));
#39829=CARTESIAN_POINT('Ctrl Pts',(0.463973722115744,1.,3.95988133243543));
#39830=CARTESIAN_POINT('Ctrl Pts',(0.467346690880671,-1.,3.96669622273946));
#39831=CARTESIAN_POINT('Ctrl Pts',(0.467346690880671,1.,3.96669622273946));
#39832=CARTESIAN_POINT('Ctrl Pts',(0.470762379613477,-1.,3.97350414289415));
#39833=CARTESIAN_POINT('Ctrl Pts',(0.470762379613477,1.,3.97350414289415));
#39834=CARTESIAN_POINT('Ctrl Pts',(0.474220061019542,-1.,3.9803033804443));
#39835=CARTESIAN_POINT('Ctrl Pts',(0.474220061019542,1.,3.9803033804443));
#39836=CARTESIAN_POINT('Ctrl Pts',(0.477718999122033,-1.,3.98709184306743));
#39837=CARTESIAN_POINT('Ctrl Pts',(0.477718999122033,1.,3.98709184306743));
#39838=CARTESIAN_POINT('Ctrl Pts',(0.481258512209637,-1.,3.99386775880655));
#39839=CARTESIAN_POINT('Ctrl Pts',(0.481258512209637,1.,3.99386775880655));
#39840=CARTESIAN_POINT('Ctrl Pts',(0.484838042421754,-1.,4.00063045119234));
#39841=CARTESIAN_POINT('Ctrl Pts',(0.484838042421754,1.,4.00063045119234));
#39842=CARTESIAN_POINT('Ctrl Pts',(0.48845713042453,-1.,4.0073800839092));
#39843=CARTESIAN_POINT('Ctrl Pts',(0.48845713042453,1.,4.0073800839092));
#39844=CARTESIAN_POINT('Ctrl Pts',(0.49211538341793,-1.,4.01411733503486));
#39845=CARTESIAN_POINT('Ctrl Pts',(0.49211538341793,1.,4.01411733503486));
#39846=CARTESIAN_POINT('Ctrl Pts',(0.495812444326222,-1.,4.02084308851813));
#39847=CARTESIAN_POINT('Ctrl Pts',(0.495812444326222,1.,4.02084308851813));
#39848=CARTESIAN_POINT('Ctrl Pts',(0.499547962340889,-1.,4.0275581398015));
#39849=CARTESIAN_POINT('Ctrl Pts',(0.499547962340889,1.,4.0275581398015));
#39850=CARTESIAN_POINT('Ctrl Pts',(0.503321556915513,-1.,4.0342628417439));
#39851=CARTESIAN_POINT('Ctrl Pts',(0.503321556915513,1.,4.0342628417439));
#39852=CARTESIAN_POINT('Ctrl Pts',(0.507132823288361,-1.,4.04095715149074));
#39853=CARTESIAN_POINT('Ctrl Pts',(0.507132823288361,1.,4.04095715149074));
#39854=CARTESIAN_POINT('Ctrl Pts',(0.510981349219173,-1.,4.04764078815591));
#39855=CARTESIAN_POINT('Ctrl Pts',(0.510981349219173,1.,4.04764078815591));
#39856=CARTESIAN_POINT('Ctrl Pts',(0.514866728193103,-1.,4.05431335771261));
#39857=CARTESIAN_POINT('Ctrl Pts',(0.514866728193103,1.,4.05431335771261));
#39858=CARTESIAN_POINT('Ctrl Pts',(0.518788572336809,-1.,4.06097448037934));
#39859=CARTESIAN_POINT('Ctrl Pts',(0.518788572336809,1.,4.06097448037934));
#39860=CARTESIAN_POINT('Ctrl Pts',(0.522746528602767,-1.,4.06762394471075));
#39861=CARTESIAN_POINT('Ctrl Pts',(0.522746528602767,1.,4.06762394471075));
#39862=CARTESIAN_POINT('Ctrl Pts',(0.526740277226999,-1.,4.07426172299496));
#39863=CARTESIAN_POINT('Ctrl Pts',(0.526740277226999,1.,4.07426172299496));
#39864=CARTESIAN_POINT('Ctrl Pts',(0.530769518728075,-1.,4.08088789536488));
#39865=CARTESIAN_POINT('Ctrl Pts',(0.530769518728075,1.,4.08088789536488));
#39866=CARTESIAN_POINT('Ctrl Pts',(0.534833963476999,-1.,4.08750259988693));
#39867=CARTESIAN_POINT('Ctrl Pts',(0.534833963476999,1.,4.08750259988693));
#39868=CARTESIAN_POINT('Ctrl Pts',(0.53893332117992,-1.,4.09410597627116));
#39869=CARTESIAN_POINT('Ctrl Pts',(0.53893332117992,1.,4.09410597627116));
#39870=CARTESIAN_POINT('Ctrl Pts',(0.543067286878457,-1.,4.10069810244473));
#39871=CARTESIAN_POINT('Ctrl Pts',(0.543067286878457,1.,4.10069810244473));
#39872=CARTESIAN_POINT('Ctrl Pts',(0.547235539486759,-1.,4.1072789702877));
#39873=CARTESIAN_POINT('Ctrl Pts',(0.547235539486759,1.,4.1072789702877));
#39874=CARTESIAN_POINT('Ctrl Pts',(0.551437758498246,-1.,4.11384852025578));
#39875=CARTESIAN_POINT('Ctrl Pts',(0.551437758498246,1.,4.11384852025578));
#39876=CARTESIAN_POINT('Ctrl Pts',(0.555673636130778,-1.,4.1204066619623));
#39877=CARTESIAN_POINT('Ctrl Pts',(0.555673636130778,1.,4.1204066619623));
#39878=CARTESIAN_POINT('Ctrl Pts',(0.559942890594628,-1.,4.12695329951859));
#39879=CARTESIAN_POINT('Ctrl Pts',(0.559942890594628,1.,4.12695329951859));
#39880=CARTESIAN_POINT('Ctrl Pts',(0.564245279535705,-1.,4.13348835726086));
#39881=CARTESIAN_POINT('Ctrl Pts',(0.564245279535705,1.,4.13348835726086));
#39882=CARTESIAN_POINT('Ctrl Pts',(0.568580610187115,-1.,4.14001179828669));
#39883=CARTESIAN_POINT('Ctrl Pts',(0.568580610187115,1.,4.14001179828669));
#39884=CARTESIAN_POINT('Ctrl Pts',(0.572948736066276,-1.,4.14652361065787));
#39885=CARTESIAN_POINT('Ctrl Pts',(0.572948736066276,1.,4.14652361065787));
#39886=CARTESIAN_POINT('Ctrl Pts',(0.576469391673916,-1.,4.1517237611974));
#39887=CARTESIAN_POINT('Ctrl Pts',(0.576469391673916,1.,4.1517237611974));
#39888=CARTESIAN_POINT('Ctrl Pts',(0.579124568912543,-1.,4.15561864787379));
#39889=CARTESIAN_POINT('Ctrl Pts',(0.579124568912543,1.,4.15561864787379));
#39890=CARTESIAN_POINT('Ctrl Pts',(0.580901211462913,-1.,4.15821291712391));
#39891=CARTESIAN_POINT('Ctrl Pts',(0.580901211462913,1.,4.15821291712391));
#39892=CARTESIAN_POINT('Ctrl Pts',(0.581791163835814,-1.,4.15950947128175));
#39893=CARTESIAN_POINT('Ctrl Pts',(0.581791163835814,1.,4.15950947128175));
#39894=CARTESIAN_POINT('',(0.385112848332548,1.,3.73017266276632));
#39895=CARTESIAN_POINT('Ctrl Pts',(0.385112848332548,-1.,3.73017266276632));
#39896=CARTESIAN_POINT('Ctrl Pts',(0.385112848332548,-0.666666666666667,
3.73017266276632));
#39897=CARTESIAN_POINT('Ctrl Pts',(0.385112848332548,-0.333333333333333,
3.73017266276632));
#39898=CARTESIAN_POINT('Ctrl Pts',(0.385112848332548,0.333333333333333,
3.73017266276632));
#39899=CARTESIAN_POINT('Ctrl Pts',(0.385112848332548,0.666666666666667,
3.73017266276632));
#39900=CARTESIAN_POINT('Ctrl Pts',(0.385112848332548,1.,3.73017266276632));
#39901=CARTESIAN_POINT('',(0.581791163835814,1.,4.15950947128175));
#39902=CARTESIAN_POINT('',(0.581791163835814,0.,4.15950947128175));
#39903=CARTESIAN_POINT('Ctrl Pts',(0.385112848332549,1.,3.73017266276632));
#39904=CARTESIAN_POINT('Ctrl Pts',(0.385087139001608,1.,3.73021431755218));
#39905=CARTESIAN_POINT('Ctrl Pts',(0.385037797882046,1.,3.73040527620929));
#39906=CARTESIAN_POINT('Ctrl Pts',(0.385031656499141,1.,3.731060828624));
#39907=CARTESIAN_POINT('Ctrl Pts',(0.385187124633964,1.,3.73273893363318));
#39908=CARTESIAN_POINT('Ctrl Pts',(0.385670806454744,1.,3.73621371845475));
#39909=CARTESIAN_POINT('Ctrl Pts',(0.386519576222035,1.,3.74144965781088));
#39910=CARTESIAN_POINT('Ctrl Pts',(0.387663020050396,1.,3.74792651696269));
#39911=CARTESIAN_POINT('Ctrl Pts',(0.38905477589825,1.,3.75529302894757));
#39912=CARTESIAN_POINT('Ctrl Pts',(0.390642072979258,1.,3.76315635032993));
#39913=CARTESIAN_POINT('Ctrl Pts',(0.392372786223346,1.,3.77114011595892));
#39914=CARTESIAN_POINT('Ctrl Pts',(0.394202481011595,1.,3.77894173114368));
#39915=CARTESIAN_POINT('Ctrl Pts',(0.396103205335028,1.,3.78640521279479));
#39916=CARTESIAN_POINT('Ctrl Pts',(0.398064818684158,1.,3.79352887163457));
#39917=CARTESIAN_POINT('Ctrl Pts',(0.400088346504726,1.,3.80040370384659));
#39918=CARTESIAN_POINT('Ctrl Pts',(0.402181320148474,1.,3.80716881962763));
#39919=CARTESIAN_POINT('Ctrl Pts',(0.404352694628236,1.,3.81396374287762));
#39920=CARTESIAN_POINT('Ctrl Pts',(0.406607038258906,1.,3.82087303913741));
#39921=CARTESIAN_POINT('Ctrl Pts',(0.408942371447376,1.,3.82790724256397));
#39922=CARTESIAN_POINT('Ctrl Pts',(0.411353038798459,1.,3.83503345578645));
#39923=CARTESIAN_POINT('Ctrl Pts',(0.413831367016726,1.,3.84219403994742));
#39924=CARTESIAN_POINT('Ctrl Pts',(0.41636967805292,1.,3.8493286415751));
#39925=CARTESIAN_POINT('Ctrl Pts',(0.418962468086809,1.,3.85639825648031));
#39926=CARTESIAN_POINT('Ctrl Pts',(0.421607423177575,1.,3.86339652542749));
#39927=CARTESIAN_POINT('Ctrl Pts',(0.424304173195142,1.,3.87033643487882));
#39928=CARTESIAN_POINT('Ctrl Pts',(0.427053541173469,1.,3.87724240306609));
#39929=CARTESIAN_POINT('Ctrl Pts',(0.429856640579733,1.,3.88414070943334));
#39930=CARTESIAN_POINT('Ctrl Pts',(0.432713929544439,1.,3.89104947940592));
#39931=CARTESIAN_POINT('Ctrl Pts',(0.435624629433505,1.,3.8979725665544));
#39932=CARTESIAN_POINT('Ctrl Pts',(0.438587235458233,1.,3.90490512938546));
#39933=CARTESIAN_POINT('Ctrl Pts',(0.441599824524047,1.,3.91183704069146));
#39934=CARTESIAN_POINT('Ctrl Pts',(0.444660430230592,1.,3.91875701610721));
#39935=CARTESIAN_POINT('Ctrl Pts',(0.447767416837296,1.,3.92565674143424));
#39936=CARTESIAN_POINT('Ctrl Pts',(0.450919768356346,1.,3.93253407403128));
#39937=CARTESIAN_POINT('Ctrl Pts',(0.454116879027575,1.,3.93939080846298));
#39938=CARTESIAN_POINT('Ctrl Pts',(0.457358410451673,1.,3.94623117206675));
#39939=CARTESIAN_POINT('Ctrl Pts',(0.460644124429119,1.,3.95306005817363));
#39940=CARTESIAN_POINT('Ctrl Pts',(0.463973722115744,1.,3.95988133243543));
#39941=CARTESIAN_POINT('Ctrl Pts',(0.467346690880671,1.,3.96669622273946));
#39942=CARTESIAN_POINT('Ctrl Pts',(0.470762379613477,1.,3.97350414289415));
#39943=CARTESIAN_POINT('Ctrl Pts',(0.474220061019542,1.,3.9803033804443));
#39944=CARTESIAN_POINT('Ctrl Pts',(0.477718999122033,1.,3.98709184306743));
#39945=CARTESIAN_POINT('Ctrl Pts',(0.481258512209637,1.,3.99386775880655));
#39946=CARTESIAN_POINT('Ctrl Pts',(0.484838042421754,1.,4.00063045119234));
#39947=CARTESIAN_POINT('Ctrl Pts',(0.48845713042453,1.,4.0073800839092));
#39948=CARTESIAN_POINT('Ctrl Pts',(0.49211538341793,1.,4.01411733503486));
#39949=CARTESIAN_POINT('Ctrl Pts',(0.495812444326222,1.,4.02084308851813));
#39950=CARTESIAN_POINT('Ctrl Pts',(0.499547962340889,1.,4.0275581398015));
#39951=CARTESIAN_POINT('Ctrl Pts',(0.503321556915513,1.,4.0342628417439));
#39952=CARTESIAN_POINT('Ctrl Pts',(0.507132823288361,1.,4.04095715149074));
#39953=CARTESIAN_POINT('Ctrl Pts',(0.510981349219173,1.,4.04764078815591));
#39954=CARTESIAN_POINT('Ctrl Pts',(0.514866728193103,1.,4.05431335771261));
#39955=CARTESIAN_POINT('Ctrl Pts',(0.518788572336809,1.,4.06097448037934));
#39956=CARTESIAN_POINT('Ctrl Pts',(0.522746528602767,1.,4.06762394471075));
#39957=CARTESIAN_POINT('Ctrl Pts',(0.526740277226999,1.,4.07426172299496));
#39958=CARTESIAN_POINT('Ctrl Pts',(0.530769518728075,1.,4.08088789536488));
#39959=CARTESIAN_POINT('Ctrl Pts',(0.534833963476999,1.,4.08750259988693));
#39960=CARTESIAN_POINT('Ctrl Pts',(0.53893332117992,1.,4.09410597627116));
#39961=CARTESIAN_POINT('Ctrl Pts',(0.543067286878457,1.,4.10069810244473));
#39962=CARTESIAN_POINT('Ctrl Pts',(0.547235539486759,1.,4.1072789702877));
#39963=CARTESIAN_POINT('Ctrl Pts',(0.551437758498246,1.,4.11384852025578));
#39964=CARTESIAN_POINT('Ctrl Pts',(0.555673636130778,1.,4.1204066619623));
#39965=CARTESIAN_POINT('Ctrl Pts',(0.559942890594628,1.,4.12695329951859));
#39966=CARTESIAN_POINT('Ctrl Pts',(0.564245279535705,1.,4.13348835726086));
#39967=CARTESIAN_POINT('Ctrl Pts',(0.568580610187115,1.,4.14001179828669));
#39968=CARTESIAN_POINT('Ctrl Pts',(0.572948736066276,1.,4.14652361065787));
#39969=CARTESIAN_POINT('Ctrl Pts',(0.576469391673916,1.,4.1517237611974));
#39970=CARTESIAN_POINT('Ctrl Pts',(0.579124568912543,1.,4.15561864787379));
#39971=CARTESIAN_POINT('Ctrl Pts',(0.580901211462913,1.,4.15821291712391));
#39972=CARTESIAN_POINT('Ctrl Pts',(0.581791163835814,1.,4.15950947128175));
#39973=CARTESIAN_POINT('Origin',(0.581791163835814,0.,4.15950947128175));
#39974=CARTESIAN_POINT('',(0.732042837400619,1.,4.13571194405636));
#39975=CARTESIAN_POINT('Origin',(0.,0.,0.));
#39976=CARTESIAN_POINT('',(0.203156094897895,1.,3.74449296982994));
#39977=CARTESIAN_POINT('Origin',(0.,1.,0.));
#39978=CARTESIAN_POINT('Ctrl Pts',(0.203156094897895,1.,3.74449296982994));
#39979=CARTESIAN_POINT('Ctrl Pts',(0.203156094897895,0.666666666666667,
3.74449296982994));
#39980=CARTESIAN_POINT('Ctrl Pts',(0.203156094897895,0.333333333333333,
3.74449296982994));
#39981=CARTESIAN_POINT('Ctrl Pts',(0.203156094897895,-0.333333333333333,
3.74449296982994));
#39982=CARTESIAN_POINT('Ctrl Pts',(0.203156094897895,-0.666666666666667,
3.74449296982994));
#39983=CARTESIAN_POINT('Ctrl Pts',(0.203156094897895,-1.,3.74449296982994));
#39984=CARTESIAN_POINT('Ctrl Pts',(0.0760622897878233,-1.,4.19931119685982));
#39985=CARTESIAN_POINT('Ctrl Pts',(0.0760622897878233,1.,4.19931119685982));
#39986=CARTESIAN_POINT('Ctrl Pts',(0.0767384596142192,-1.,4.19789138621624));
#39987=CARTESIAN_POINT('Ctrl Pts',(0.0767384596142192,1.,4.19789138621624));
#39988=CARTESIAN_POINT('Ctrl Pts',(0.0780873956244399,-1.,4.19505112860624));
#39989=CARTESIAN_POINT('Ctrl Pts',(0.0780873956244399,1.,4.19505112860624));
#39990=CARTESIAN_POINT('Ctrl Pts',(0.08010058871176,-1.,4.19078883322483));
#39991=CARTESIAN_POINT('Ctrl Pts',(0.08010058871176,1.,4.19078883322483));
#39992=CARTESIAN_POINT('Ctrl Pts',(0.0827644164389507,-1.,4.1851019532944));
#39993=CARTESIAN_POINT('Ctrl Pts',(0.0827644164389507,1.,4.1851019532944));
#39994=CARTESIAN_POINT('Ctrl Pts',(0.0860600915552512,-1.,4.17798698669991));
#39995=CARTESIAN_POINT('Ctrl Pts',(0.0860600915552512,1.,4.17798698669991));
#39996=CARTESIAN_POINT('Ctrl Pts',(0.0893215560850325,-1.,4.17086566491823));
#39997=CARTESIAN_POINT('Ctrl Pts',(0.0893215560850325,1.,4.17086566491823));
#39998=CARTESIAN_POINT('Ctrl Pts',(0.0925486672167687,-1.,4.16373802265942));
#39999=CARTESIAN_POINT('Ctrl Pts',(0.0925486672167687,1.,4.16373802265942));
#40000=CARTESIAN_POINT('Ctrl Pts',(0.0957412403297065,-1.,4.15660412653006));
#40001=CARTESIAN_POINT('Ctrl Pts',(0.0957412403297065,1.,4.15660412653006));
#40002=CARTESIAN_POINT('Ctrl Pts',(0.0988990478899809,-1.,4.1494640891762));
#40003=CARTESIAN_POINT('Ctrl Pts',(0.0988990478899809,1.,4.1494640891762));
#40004=CARTESIAN_POINT('Ctrl Pts',(0.102021826577453,-1.,4.14231804938737));
#40005=CARTESIAN_POINT('Ctrl Pts',(0.102021826577453,1.,4.14231804938737));
#40006=CARTESIAN_POINT('Ctrl Pts',(0.105109286538864,-1.,4.13516614458396));
#40007=CARTESIAN_POINT('Ctrl Pts',(0.105109286538864,1.,4.13516614458396));
#40008=CARTESIAN_POINT('Ctrl Pts',(0.10816112052835,-1.,4.12800848371386));
#40009=CARTESIAN_POINT('Ctrl Pts',(0.10816112052835,1.,4.12800848371386));
#40010=CARTESIAN_POINT('Ctrl Pts',(0.111177012683377,-1.,4.12084512502444));
#40011=CARTESIAN_POINT('Ctrl Pts',(0.111177012683377,1.,4.12084512502444));
#40012=CARTESIAN_POINT('Ctrl Pts',(0.114156649609601,-1.,4.11367603925313));
#40013=CARTESIAN_POINT('Ctrl Pts',(0.114156649609601,1.,4.11367603925313));
#40014=CARTESIAN_POINT('Ctrl Pts',(0.117099722731704,-1.,4.10650113382187));
#40015=CARTESIAN_POINT('Ctrl Pts',(0.117099722731704,1.,4.10650113382187));
#40016=CARTESIAN_POINT('Ctrl Pts',(0.120005924388162,-1.,4.09932031767243));
#40017=CARTESIAN_POINT('Ctrl Pts',(0.120005924388162,1.,4.09932031767243));
#40018=CARTESIAN_POINT('Ctrl Pts',(0.122874946249119,-1.,4.09213355850836));
#40019=CARTESIAN_POINT('Ctrl Pts',(0.122874946249119,1.,4.09213355850836));
#40020=CARTESIAN_POINT('Ctrl Pts',(0.125706476822529,-1.,4.08494093372315));
#40021=CARTESIAN_POINT('Ctrl Pts',(0.125706476822529,1.,4.08494093372315));
#40022=CARTESIAN_POINT('Ctrl Pts',(0.128500200484813,-1.,4.07774270738809));
#40023=CARTESIAN_POINT('Ctrl Pts',(0.128500200484813,1.,4.07774270738809));
#40024=CARTESIAN_POINT('Ctrl Pts',(0.131255793548914,-1.,4.07053931528579));
#40025=CARTESIAN_POINT('Ctrl Pts',(0.131255793548914,1.,4.07053931528579));
#40026=CARTESIAN_POINT('Ctrl Pts',(0.133972916144225,-1.,4.06333121018476));
#40027=CARTESIAN_POINT('Ctrl Pts',(0.133972916144225,1.,4.06333121018476));
#40028=CARTESIAN_POINT('Ctrl Pts',(0.136651205046111,-1.,4.05611873400122));
#40029=CARTESIAN_POINT('Ctrl Pts',(0.136651205046111,1.,4.05611873400122));
#40030=CARTESIAN_POINT('Ctrl Pts',(0.139290267180059,-1.,4.04890199238056));
#40031=CARTESIAN_POINT('Ctrl Pts',(0.139290267180059,1.,4.04890199238056));
#40032=CARTESIAN_POINT('Ctrl Pts',(0.141889671485507,-1.,4.04168069633842));
#40033=CARTESIAN_POINT('Ctrl Pts',(0.141889671485507,1.,4.04168069633842));
#40034=CARTESIAN_POINT('Ctrl Pts',(0.144448947038352,-1.,4.03445411510403));
#40035=CARTESIAN_POINT('Ctrl Pts',(0.144448947038352,1.,4.03445411510403));
#40036=CARTESIAN_POINT('Ctrl Pts',(0.146967602878998,-1.,4.02722143147048));
#40037=CARTESIAN_POINT('Ctrl Pts',(0.146967602878998,1.,4.02722143147048));
#40038=CARTESIAN_POINT('Ctrl Pts',(0.149445144968707,-1.,4.01998203715588));
#40039=CARTESIAN_POINT('Ctrl Pts',(0.149445144968707,1.,4.01998203715588));
#40040=CARTESIAN_POINT('Ctrl Pts',(0.151881094022909,-1.,4.01273584234684));
#40041=CARTESIAN_POINT('Ctrl Pts',(0.151881094022909,1.,4.01273584234684));
#40042=CARTESIAN_POINT('Ctrl Pts',(0.154275004872309,-1.,4.00548360245297));
#40043=CARTESIAN_POINT('Ctrl Pts',(0.154275004872309,1.,4.00548360245297));
#40044=CARTESIAN_POINT('Ctrl Pts',(0.156626481393735,-1.,3.99822717425869));
#40045=CARTESIAN_POINT('Ctrl Pts',(0.156626481393735,1.,3.99822717425869));
#40046=CARTESIAN_POINT('Ctrl Pts',(0.158935123982796,-1.,3.99096873945862));
#40047=CARTESIAN_POINT('Ctrl Pts',(0.158935123982796,1.,3.99096873945862));
#40048=CARTESIAN_POINT('Ctrl Pts',(0.161200482186087,-1.,3.98371010319866));
#40049=CARTESIAN_POINT('Ctrl Pts',(0.161200482186087,1.,3.98371010319866));
#40050=CARTESIAN_POINT('Ctrl Pts',(0.163422004609998,-1.,3.97645194630944));
#40051=CARTESIAN_POINT('Ctrl Pts',(0.163422004609998,1.,3.97645194630944));
#40052=CARTESIAN_POINT('Ctrl Pts',(0.165598992851097,-1.,3.9691931362141));
#40053=CARTESIAN_POINT('Ctrl Pts',(0.165598992851097,1.,3.9691931362141));
#40054=CARTESIAN_POINT('Ctrl Pts',(0.167730547023312,-1.,3.96192990160296));
#40055=CARTESIAN_POINT('Ctrl Pts',(0.167730547023312,1.,3.96192990160296));
#40056=CARTESIAN_POINT('Ctrl Pts',(0.16981566637413,-1.,3.95465744665263));
#40057=CARTESIAN_POINT('Ctrl Pts',(0.16981566637413,1.,3.95465744665263));
#40058=CARTESIAN_POINT('Ctrl Pts',(0.171853355369232,-1.,3.94737164900861));
#40059=CARTESIAN_POINT('Ctrl Pts',(0.171853355369232,1.,3.94737164900861));
#40060=CARTESIAN_POINT('Ctrl Pts',(0.173842734974607,-1.,3.94007083096214));
#40061=CARTESIAN_POINT('Ctrl Pts',(0.173842734974607,1.,3.94007083096214));
#40062=CARTESIAN_POINT('Ctrl Pts',(0.175783136893872,-1.,3.93275726771049));
#40063=CARTESIAN_POINT('Ctrl Pts',(0.175783136893872,1.,3.93275726771049));
#40064=CARTESIAN_POINT('Ctrl Pts',(0.177674246152328,-1.,3.92543942697672));
#40065=CARTESIAN_POINT('Ctrl Pts',(0.177674246152328,1.,3.92543942697672));
#40066=CARTESIAN_POINT('Ctrl Pts',(0.179515885822894,-1.,3.91812876180948));
#40067=CARTESIAN_POINT('Ctrl Pts',(0.179515885822894,1.,3.91812876180948));
#40068=CARTESIAN_POINT('Ctrl Pts',(0.181307740731795,-1.,3.91083557557193));
#40069=CARTESIAN_POINT('Ctrl Pts',(0.181307740731795,1.,3.91083557557193));
#40070=CARTESIAN_POINT('Ctrl Pts',(0.183049081993193,-1.,3.90356488555138));
#40071=CARTESIAN_POINT('Ctrl Pts',(0.183049081993193,1.,3.90356488555138));
#40072=CARTESIAN_POINT('Ctrl Pts',(0.184738537728034,-1.,3.89631300742633));
#40073=CARTESIAN_POINT('Ctrl Pts',(0.184738537728034,1.,3.89631300742633));
#40074=CARTESIAN_POINT('Ctrl Pts',(0.186373724985263,-1.,3.88906196725817));
#40075=CARTESIAN_POINT('Ctrl Pts',(0.186373724985263,1.,3.88906196725817));
#40076=CARTESIAN_POINT('Ctrl Pts',(0.187951632512663,-1.,3.88178563496187));
#40077=CARTESIAN_POINT('Ctrl Pts',(0.187951632512663,1.,3.88178563496187));
#40078=CARTESIAN_POINT('Ctrl Pts',(0.189469253358254,-1.,3.87445976418377));
#40079=CARTESIAN_POINT('Ctrl Pts',(0.189469253358254,1.,3.87445976418377));
#40080=CARTESIAN_POINT('Ctrl Pts',(0.190924190418612,-1.,3.8670715862477));
#40081=CARTESIAN_POINT('Ctrl Pts',(0.190924190418612,1.,3.8670715862477));
#40082=CARTESIAN_POINT('Ctrl Pts',(0.192315153044979,-1.,3.85962774407652));
#40083=CARTESIAN_POINT('Ctrl Pts',(0.192315153044979,1.,3.85962774407652));
#40084=CARTESIAN_POINT('Ctrl Pts',(0.193642806777747,-1.,3.85216762264019));
#40085=CARTESIAN_POINT('Ctrl Pts',(0.193642806777747,1.,3.85216762264019));
#40086=CARTESIAN_POINT('Ctrl Pts',(0.194909009460254,-1.,3.84475203347052));
#40087=CARTESIAN_POINT('Ctrl Pts',(0.194909009460254,1.,3.84475203347052));
#40088=CARTESIAN_POINT('Ctrl Pts',(0.196115198971889,-1.,3.83743910616265));
#40089=CARTESIAN_POINT('Ctrl Pts',(0.196115198971889,1.,3.83743910616265));
#40090=CARTESIAN_POINT('Ctrl Pts',(0.197260935827375,-1.,3.83026221776488));
#40091=CARTESIAN_POINT('Ctrl Pts',(0.197260935827375,1.,3.83026221776488));
#40092=CARTESIAN_POINT('Ctrl Pts',(0.198342616900469,-1.,3.82321127348981));
#40093=CARTESIAN_POINT('Ctrl Pts',(0.198342616900469,1.,3.82321127348981));
#40094=CARTESIAN_POINT('Ctrl Pts',(0.199351525297396,-1.,3.81620203429702));
#40095=CARTESIAN_POINT('Ctrl Pts',(0.199351525297396,1.,3.81620203429702));
#40096=CARTESIAN_POINT('Ctrl Pts',(0.200274679433289,-1.,3.80909529318501));
#40097=CARTESIAN_POINT('Ctrl Pts',(0.200274679433289,1.,3.80909529318501));
#40098=CARTESIAN_POINT('Ctrl Pts',(0.201097756307251,-1.,3.80175247447171));
#40099=CARTESIAN_POINT('Ctrl Pts',(0.201097756307251,1.,3.80175247447171));
#40100=CARTESIAN_POINT('Ctrl Pts',(0.201807533800798,-1.,3.79408354187274));
#40101=CARTESIAN_POINT('Ctrl Pts',(0.201807533800798,1.,3.79408354187274));
#40102=CARTESIAN_POINT('Ctrl Pts',(0.202394260512192,-1.,3.78609175019317));
#40103=CARTESIAN_POINT('Ctrl Pts',(0.202394260512192,1.,3.78609175019317));
#40104=CARTESIAN_POINT('Ctrl Pts',(0.202854729699196,-1.,3.77793553476879));
#40105=CARTESIAN_POINT('Ctrl Pts',(0.202854729699196,1.,3.77793553476879));
#40106=CARTESIAN_POINT('Ctrl Pts',(0.203192390045337,-1.,3.76992071595267));
#40107=CARTESIAN_POINT('Ctrl Pts',(0.203192390045337,1.,3.76992071595267));
#40108=CARTESIAN_POINT('Ctrl Pts',(0.203414634707646,-1.,3.76242717937273));
#40109=CARTESIAN_POINT('Ctrl Pts',(0.203414634707646,1.,3.76242717937273));
#40110=CARTESIAN_POINT('Ctrl Pts',(0.203530796848403,-1.,3.75585118707924));
#40111=CARTESIAN_POINT('Ctrl Pts',(0.203530796848403,1.,3.75585118707924));
#40112=CARTESIAN_POINT('Ctrl Pts',(0.203550035479096,-1.,3.75054693397716));
#40113=CARTESIAN_POINT('Ctrl Pts',(0.203550035479096,1.,3.75054693397716));
#40114=CARTESIAN_POINT('Ctrl Pts',(0.203478844530229,-1.,3.74675472018582));
#40115=CARTESIAN_POINT('Ctrl Pts',(0.203478844530229,1.,3.74675472018582));
#40116=CARTESIAN_POINT('Ctrl Pts',(0.203352057956055,-1.,3.7450208092684));
#40117=CARTESIAN_POINT('Ctrl Pts',(0.203352057956055,1.,3.7450208092684));
#40118=CARTESIAN_POINT('Ctrl Pts',(0.203218215747894,-1.,3.74446880195845));
#40119=CARTESIAN_POINT('Ctrl Pts',(0.203218215747894,1.,3.74446880195845));
#40120=CARTESIAN_POINT('Ctrl Pts',(0.20311176758786,-1.,3.74443319346666));
#40121=CARTESIAN_POINT('Ctrl Pts',(0.20311176758786,1.,3.74443319346666));
#40122=CARTESIAN_POINT('Ctrl Pts',(0.203054238699719,-1.,3.74449849461127));
#40123=CARTESIAN_POINT('Ctrl Pts',(0.203054238699719,1.,3.74449849461127));
#40124=CARTESIAN_POINT('',(0.0760622897878233,1.,4.19931119685982));
#40125=CARTESIAN_POINT('Ctrl Pts',(0.0760622897878233,1.,4.19931119685982));
#40126=CARTESIAN_POINT('Ctrl Pts',(0.0767384596142192,1.,4.19789138621624));
#40127=CARTESIAN_POINT('Ctrl Pts',(0.0780873956244399,1.,4.19505112860624));
#40128=CARTESIAN_POINT('Ctrl Pts',(0.08010058871176,1.,4.19078883322483));
#40129=CARTESIAN_POINT('Ctrl Pts',(0.0827644164389507,1.,4.1851019532944));
#40130=CARTESIAN_POINT('Ctrl Pts',(0.0860600915552512,1.,4.17798698669991));
#40131=CARTESIAN_POINT('Ctrl Pts',(0.0893215560850325,1.,4.17086566491823));
#40132=CARTESIAN_POINT('Ctrl Pts',(0.0925486672167687,1.,4.16373802265942));
#40133=CARTESIAN_POINT('Ctrl Pts',(0.0957412403297065,1.,4.15660412653006));
#40134=CARTESIAN_POINT('Ctrl Pts',(0.0988990478899809,1.,4.1494640891762));
#40135=CARTESIAN_POINT('Ctrl Pts',(0.102021826577453,1.,4.14231804938737));
#40136=CARTESIAN_POINT('Ctrl Pts',(0.105109286538864,1.,4.13516614458396));
#40137=CARTESIAN_POINT('Ctrl Pts',(0.10816112052835,1.,4.12800848371386));
#40138=CARTESIAN_POINT('Ctrl Pts',(0.111177012683377,1.,4.12084512502444));
#40139=CARTESIAN_POINT('Ctrl Pts',(0.114156649609601,1.,4.11367603925313));
#40140=CARTESIAN_POINT('Ctrl Pts',(0.117099722731704,1.,4.10650113382187));
#40141=CARTESIAN_POINT('Ctrl Pts',(0.120005924388162,1.,4.09932031767243));
#40142=CARTESIAN_POINT('Ctrl Pts',(0.122874946249119,1.,4.09213355850836));
#40143=CARTESIAN_POINT('Ctrl Pts',(0.125706476822529,1.,4.08494093372315));
#40144=CARTESIAN_POINT('Ctrl Pts',(0.128500200484813,1.,4.07774270738809));
#40145=CARTESIAN_POINT('Ctrl Pts',(0.131255793548914,1.,4.07053931528579));
#40146=CARTESIAN_POINT('Ctrl Pts',(0.133972916144225,1.,4.06333121018476));
#40147=CARTESIAN_POINT('Ctrl Pts',(0.136651205046111,1.,4.05611873400122));
#40148=CARTESIAN_POINT('Ctrl Pts',(0.139290267180059,1.,4.04890199238056));
#40149=CARTESIAN_POINT('Ctrl Pts',(0.141889671485507,1.,4.04168069633842));
#40150=CARTESIAN_POINT('Ctrl Pts',(0.144448947038352,1.,4.03445411510403));
#40151=CARTESIAN_POINT('Ctrl Pts',(0.146967602878998,1.,4.02722143147048));
#40152=CARTESIAN_POINT('Ctrl Pts',(0.149445144968707,1.,4.01998203715588));
#40153=CARTESIAN_POINT('Ctrl Pts',(0.151881094022909,1.,4.01273584234684));
#40154=CARTESIAN_POINT('Ctrl Pts',(0.154275004872309,1.,4.00548360245297));
#40155=CARTESIAN_POINT('Ctrl Pts',(0.156626481393735,1.,3.99822717425869));
#40156=CARTESIAN_POINT('Ctrl Pts',(0.158935123982796,1.,3.99096873945862));
#40157=CARTESIAN_POINT('Ctrl Pts',(0.161200482186087,1.,3.98371010319866));
#40158=CARTESIAN_POINT('Ctrl Pts',(0.163422004609998,1.,3.97645194630944));
#40159=CARTESIAN_POINT('Ctrl Pts',(0.165598992851097,1.,3.9691931362141));
#40160=CARTESIAN_POINT('Ctrl Pts',(0.167730547023312,1.,3.96192990160296));
#40161=CARTESIAN_POINT('Ctrl Pts',(0.16981566637413,1.,3.95465744665263));
#40162=CARTESIAN_POINT('Ctrl Pts',(0.171853355369232,1.,3.94737164900861));
#40163=CARTESIAN_POINT('Ctrl Pts',(0.173842734974607,1.,3.94007083096214));
#40164=CARTESIAN_POINT('Ctrl Pts',(0.175783136893872,1.,3.93275726771049));
#40165=CARTESIAN_POINT('Ctrl Pts',(0.177674246152328,1.,3.92543942697672));
#40166=CARTESIAN_POINT('Ctrl Pts',(0.179515885822894,1.,3.91812876180948));
#40167=CARTESIAN_POINT('Ctrl Pts',(0.181307740731795,1.,3.91083557557193));
#40168=CARTESIAN_POINT('Ctrl Pts',(0.183049081993193,1.,3.90356488555138));
#40169=CARTESIAN_POINT('Ctrl Pts',(0.184738537728034,1.,3.89631300742633));
#40170=CARTESIAN_POINT('Ctrl Pts',(0.186373724985263,1.,3.88906196725817));
#40171=CARTESIAN_POINT('Ctrl Pts',(0.187951632512663,1.,3.88178563496187));
#40172=CARTESIAN_POINT('Ctrl Pts',(0.189469253358254,1.,3.87445976418377));
#40173=CARTESIAN_POINT('Ctrl Pts',(0.190924190418612,1.,3.8670715862477));
#40174=CARTESIAN_POINT('Ctrl Pts',(0.192315153044979,1.,3.85962774407652));
#40175=CARTESIAN_POINT('Ctrl Pts',(0.193642806777747,1.,3.85216762264019));
#40176=CARTESIAN_POINT('Ctrl Pts',(0.194909009460254,1.,3.84475203347052));
#40177=CARTESIAN_POINT('Ctrl Pts',(0.196115198971889,1.,3.83743910616265));
#40178=CARTESIAN_POINT('Ctrl Pts',(0.197260935827375,1.,3.83026221776488));
#40179=CARTESIAN_POINT('Ctrl Pts',(0.198342616900469,1.,3.82321127348981));
#40180=CARTESIAN_POINT('Ctrl Pts',(0.199351525297396,1.,3.81620203429702));
#40181=CARTESIAN_POINT('Ctrl Pts',(0.200274679433289,1.,3.80909529318501));
#40182=CARTESIAN_POINT('Ctrl Pts',(0.201097756307251,1.,3.80175247447171));
#40183=CARTESIAN_POINT('Ctrl Pts',(0.201807533800798,1.,3.79408354187274));
#40184=CARTESIAN_POINT('Ctrl Pts',(0.202394260512192,1.,3.78609175019317));
#40185=CARTESIAN_POINT('Ctrl Pts',(0.202854729699196,1.,3.77793553476879));
#40186=CARTESIAN_POINT('Ctrl Pts',(0.203192390045337,1.,3.76992071595267));
#40187=CARTESIAN_POINT('Ctrl Pts',(0.203414634707646,1.,3.76242717937273));
#40188=CARTESIAN_POINT('Ctrl Pts',(0.203530796848403,1.,3.75585118707924));
#40189=CARTESIAN_POINT('Ctrl Pts',(0.203550035479096,1.,3.75054693397716));
#40190=CARTESIAN_POINT('Ctrl Pts',(0.203484186269314,1.,3.74703926501843));
#40191=CARTESIAN_POINT('Ctrl Pts',(0.203375226874331,1.,3.74535749969262));
#40192=CARTESIAN_POINT('Ctrl Pts',(0.203266610111263,1.,3.74471097893961));
#40193=CARTESIAN_POINT('Ctrl Pts',(0.203188003947964,1.,3.74453008995129));
#40194=CARTESIAN_POINT('Ctrl Pts',(0.203156094897895,1.,3.74449296982994));
#40195=CARTESIAN_POINT('',(0.0760622897878233,0.,4.19931119685982));
#40196=CARTESIAN_POINT('Ctrl Pts',(-0.20305423869972,-1.,3.74449849461127));
#40197=CARTESIAN_POINT('Ctrl Pts',(-0.20305423869972,1.,3.74449849461127));
#40198=CARTESIAN_POINT('Ctrl Pts',(-0.203111767587923,-1.,3.7444331934681));
#40199=CARTESIAN_POINT('Ctrl Pts',(-0.203111767587923,1.,3.7444331934681));
#40200=CARTESIAN_POINT('Ctrl Pts',(-0.203218215748059,-1.,3.7444688019622));
#40201=CARTESIAN_POINT('Ctrl Pts',(-0.203218215748059,1.,3.7444688019622));
#40202=CARTESIAN_POINT('Ctrl Pts',(-0.203352057956297,-1.,3.74502080927395));
#40203=CARTESIAN_POINT('Ctrl Pts',(-0.203352057956297,1.,3.74502080927395));
#40204=CARTESIAN_POINT('Ctrl Pts',(-0.203478844530447,-1.,3.7467547201908));
#40205=CARTESIAN_POINT('Ctrl Pts',(-0.203478844530447,1.,3.7467547201908));
#40206=CARTESIAN_POINT('Ctrl Pts',(-0.203550035479166,-1.,3.75054693397875));
#40207=CARTESIAN_POINT('Ctrl Pts',(-0.203550035479166,1.,3.75054693397875));
#40208=CARTESIAN_POINT('Ctrl Pts',(-0.203530796848322,-1.,3.75585118707734));
#40209=CARTESIAN_POINT('Ctrl Pts',(-0.203530796848322,1.,3.75585118707734));
#40210=CARTESIAN_POINT('Ctrl Pts',(-0.203414634707479,-1.,3.76242717936885));
#40211=CARTESIAN_POINT('Ctrl Pts',(-0.203414634707479,1.,3.76242717936885));
#40212=CARTESIAN_POINT('Ctrl Pts',(-0.203192390045165,-1.,3.7699207159487));
#40213=CARTESIAN_POINT('Ctrl Pts',(-0.203192390045165,1.,3.7699207159487));
#40214=CARTESIAN_POINT('Ctrl Pts',(-0.202854729699081,-1.,3.77793553476614));
#40215=CARTESIAN_POINT('Ctrl Pts',(-0.202854729699081,1.,3.77793553476614));
#40216=CARTESIAN_POINT('Ctrl Pts',(-0.20239426051216,-1.,3.78609175019242));
#40217=CARTESIAN_POINT('Ctrl Pts',(-0.20239426051216,1.,3.78609175019242));
#40218=CARTESIAN_POINT('Ctrl Pts',(-0.201807533800837,-1.,3.7940835418736));
#40219=CARTESIAN_POINT('Ctrl Pts',(-0.201807533800837,1.,3.7940835418736));
#40220=CARTESIAN_POINT('Ctrl Pts',(-0.201097756307326,-1.,3.80175247447337));
#40221=CARTESIAN_POINT('Ctrl Pts',(-0.201097756307326,1.,3.80175247447337));
#40222=CARTESIAN_POINT('Ctrl Pts',(-0.200274679433365,-1.,3.80909529318669));
#40223=CARTESIAN_POINT('Ctrl Pts',(-0.200274679433365,1.,3.80909529318669));
#40224=CARTESIAN_POINT('Ctrl Pts',(-0.199351525297447,-1.,3.81620203429815));
#40225=CARTESIAN_POINT('Ctrl Pts',(-0.199351525297447,1.,3.81620203429815));
#40226=CARTESIAN_POINT('Ctrl Pts',(-0.198342616900487,-1.,3.82321127349016));
#40227=CARTESIAN_POINT('Ctrl Pts',(-0.198342616900487,1.,3.82321127349016));
#40228=CARTESIAN_POINT('Ctrl Pts',(-0.197260935827362,-1.,3.83026221776456));
#40229=CARTESIAN_POINT('Ctrl Pts',(-0.197260935827362,1.,3.83026221776456));
#40230=CARTESIAN_POINT('Ctrl Pts',(-0.196115198971859,-1.,3.83743910616195));
#40231=CARTESIAN_POINT('Ctrl Pts',(-0.196115198971859,1.,3.83743910616195));
#40232=CARTESIAN_POINT('Ctrl Pts',(-0.194909009460221,-1.,3.84475203346977));
#40233=CARTESIAN_POINT('Ctrl Pts',(-0.194909009460221,1.,3.84475203346977));
#40234=CARTESIAN_POINT('Ctrl Pts',(-0.193642806777723,-1.,3.85216762263966));
#40235=CARTESIAN_POINT('Ctrl Pts',(-0.193642806777723,1.,3.85216762263966));
#40236=CARTESIAN_POINT('Ctrl Pts',(-0.192315153044971,-1.,3.85962774407633));
#40237=CARTESIAN_POINT('Ctrl Pts',(-0.192315153044971,1.,3.85962774407633));
#40238=CARTESIAN_POINT('Ctrl Pts',(-0.19092419041862,-1.,3.86707158624783));
#40239=CARTESIAN_POINT('Ctrl Pts',(-0.19092419041862,1.,3.86707158624783));
#40240=CARTESIAN_POINT('Ctrl Pts',(-0.189469253358273,-1.,3.87445976418412));
#40241=CARTESIAN_POINT('Ctrl Pts',(-0.189469253358273,1.,3.87445976418412));
#40242=CARTESIAN_POINT('Ctrl Pts',(-0.187951632512685,-1.,3.88178563496228));
#40243=CARTESIAN_POINT('Ctrl Pts',(-0.187951632512685,1.,3.88178563496228));
#40244=CARTESIAN_POINT('Ctrl Pts',(-0.186373724985281,-1.,3.88906196725848));
#40245=CARTESIAN_POINT('Ctrl Pts',(-0.186373724985281,1.,3.88906196725848));
#40246=CARTESIAN_POINT('Ctrl Pts',(-0.184738537728043,-1.,3.89631300742646));
#40247=CARTESIAN_POINT('Ctrl Pts',(-0.184738537728043,1.,3.89631300742646));
#40248=CARTESIAN_POINT('Ctrl Pts',(-0.183049081993191,-1.,3.90356488555132));
#40249=CARTESIAN_POINT('Ctrl Pts',(-0.183049081993191,1.,3.90356488555132));
#40250=CARTESIAN_POINT('Ctrl Pts',(-0.181307740731786,-1.,3.91083557557175));
#40251=CARTESIAN_POINT('Ctrl Pts',(-0.181307740731786,1.,3.91083557557175));
#40252=CARTESIAN_POINT('Ctrl Pts',(-0.179515885822882,-1.,3.91812876180926));
#40253=CARTESIAN_POINT('Ctrl Pts',(-0.179515885822882,1.,3.91812876180926));
#40254=CARTESIAN_POINT('Ctrl Pts',(-0.177674246152318,-1.,3.92543942697655));
#40255=CARTESIAN_POINT('Ctrl Pts',(-0.177674246152318,1.,3.92543942697655));
#40256=CARTESIAN_POINT('Ctrl Pts',(-0.175783136893868,-1.,3.93275726771042));
#40257=CARTESIAN_POINT('Ctrl Pts',(-0.175783136893868,1.,3.93275726771042));
#40258=CARTESIAN_POINT('Ctrl Pts',(-0.17384273497461,-1.,3.94007083096217));
#40259=CARTESIAN_POINT('Ctrl Pts',(-0.17384273497461,1.,3.94007083096217));
#40260=CARTESIAN_POINT('Ctrl Pts',(-0.17185335536924,-1.,3.94737164900868));
#40261=CARTESIAN_POINT('Ctrl Pts',(-0.17185335536924,1.,3.94737164900868));
#40262=CARTESIAN_POINT('Ctrl Pts',(-0.169815666374139,-1.,3.95465744665268));
#40263=CARTESIAN_POINT('Ctrl Pts',(-0.169815666374139,1.,3.95465744665268));
#40264=CARTESIAN_POINT('Ctrl Pts',(-0.16773054702332,-1.,3.96192990160296));
#40265=CARTESIAN_POINT('Ctrl Pts',(-0.16773054702332,1.,3.96192990160296));
#40266=CARTESIAN_POINT('Ctrl Pts',(-0.165598992851102,-1.,3.96919313621407));
#40267=CARTESIAN_POINT('Ctrl Pts',(-0.165598992851102,1.,3.96919313621407));
#40268=CARTESIAN_POINT('Ctrl Pts',(-0.163422004609999,-1.,3.97645194630943));
#40269=CARTESIAN_POINT('Ctrl Pts',(-0.163422004609999,1.,3.97645194630943));
#40270=CARTESIAN_POINT('Ctrl Pts',(-0.161200482186085,-1.,3.98371010319872));
#40271=CARTESIAN_POINT('Ctrl Pts',(-0.161200482186085,1.,3.98371010319872));
#40272=CARTESIAN_POINT('Ctrl Pts',(-0.158935123982793,-1.,3.99096873945878));
#40273=CARTESIAN_POINT('Ctrl Pts',(-0.158935123982793,1.,3.99096873945878));
#40274=CARTESIAN_POINT('Ctrl Pts',(-0.156626481393734,-1.,3.99822717425893));
#40275=CARTESIAN_POINT('Ctrl Pts',(-0.156626481393734,1.,3.99822717425893));
#40276=CARTESIAN_POINT('Ctrl Pts',(-0.154275004872311,-1.,4.00548360245319));
#40277=CARTESIAN_POINT('Ctrl Pts',(-0.154275004872311,1.,4.00548360245319));
#40278=CARTESIAN_POINT('Ctrl Pts',(-0.151881094022911,-1.,4.01273584234689));
#40279=CARTESIAN_POINT('Ctrl Pts',(-0.151881094022911,1.,4.01273584234689));
#40280=CARTESIAN_POINT('Ctrl Pts',(-0.149445144968707,-1.,4.01998203715564));
#40281=CARTESIAN_POINT('Ctrl Pts',(-0.149445144968707,1.,4.01998203715564));
#40282=CARTESIAN_POINT('Ctrl Pts',(-0.146967602878994,-1.,4.02722143146994));
#40283=CARTESIAN_POINT('Ctrl Pts',(-0.146967602878994,1.,4.02722143146994));
#40284=CARTESIAN_POINT('Ctrl Pts',(-0.144448947038345,-1.,4.03445411510333));
#40285=CARTESIAN_POINT('Ctrl Pts',(-0.144448947038345,1.,4.03445411510333));
#40286=CARTESIAN_POINT('Ctrl Pts',(-0.1418896714855,-1.,4.04168069633781));
#40287=CARTESIAN_POINT('Ctrl Pts',(-0.1418896714855,1.,4.04168069633781));
#40288=CARTESIAN_POINT('Ctrl Pts',(-0.139290267180057,-1.,4.04890199238036));
#40289=CARTESIAN_POINT('Ctrl Pts',(-0.139290267180057,1.,4.04890199238036));
#40290=CARTESIAN_POINT('Ctrl Pts',(-0.136651205046119,-1.,4.05611873400172));
#40291=CARTESIAN_POINT('Ctrl Pts',(-0.136651205046119,1.,4.05611873400172));
#40292=CARTESIAN_POINT('Ctrl Pts',(-0.133972916144245,-1.,4.06333121018596));
#40293=CARTESIAN_POINT('Ctrl Pts',(-0.133972916144245,1.,4.06333121018596));
#40294=CARTESIAN_POINT('Ctrl Pts',(-0.131255793548941,-1.,4.0705393152874));
#40295=CARTESIAN_POINT('Ctrl Pts',(-0.131255793548941,1.,4.0705393152874));
#40296=CARTESIAN_POINT('Ctrl Pts',(-0.128500200484838,-1.,4.07774270738954));
#40297=CARTESIAN_POINT('Ctrl Pts',(-0.128500200484838,1.,4.07774270738954));
#40298=CARTESIAN_POINT('Ctrl Pts',(-0.12570647682254,-1.,4.08494093372377));
#40299=CARTESIAN_POINT('Ctrl Pts',(-0.12570647682254,1.,4.08494093372377));
#40300=CARTESIAN_POINT('Ctrl Pts',(-0.122874946249107,-1.,4.09213355850756));
#40301=CARTESIAN_POINT('Ctrl Pts',(-0.122874946249107,1.,4.09213355850756));
#40302=CARTESIAN_POINT('Ctrl Pts',(-0.120005924388124,-1.,4.09932031767002));
#40303=CARTESIAN_POINT('Ctrl Pts',(-0.120005924388124,1.,4.09932031767002));
#40304=CARTESIAN_POINT('Ctrl Pts',(-0.117099722731648,-1.,4.10650113381833));
#40305=CARTESIAN_POINT('Ctrl Pts',(-0.117099722731648,1.,4.10650113381833));
#40306=CARTESIAN_POINT('Ctrl Pts',(-0.114156649609546,-1.,4.11367603924961));
#40307=CARTESIAN_POINT('Ctrl Pts',(-0.114156649609546,1.,4.11367603924961));
#40308=CARTESIAN_POINT('Ctrl Pts',(-0.111177012683347,-1.,4.1208451250225));
#40309=CARTESIAN_POINT('Ctrl Pts',(-0.111177012683347,1.,4.1208451250225));
#40310=CARTESIAN_POINT('Ctrl Pts',(-0.10816112052837,-1.,4.12800848371504));
#40311=CARTESIAN_POINT('Ctrl Pts',(-0.10816112052837,1.,4.12800848371504));
#40312=CARTESIAN_POINT('Ctrl Pts',(-0.105109286538945,-1.,4.13516614458895));
#40313=CARTESIAN_POINT('Ctrl Pts',(-0.105109286538945,1.,4.13516614458895));
#40314=CARTESIAN_POINT('Ctrl Pts',(-0.102021826577584,-1.,4.14231804939538));
#40315=CARTESIAN_POINT('Ctrl Pts',(-0.102021826577584,1.,4.14231804939538));
#40316=CARTESIAN_POINT('Ctrl Pts',(-0.0988990478901228,-1.,4.14946408918485));
#40317=CARTESIAN_POINT('Ctrl Pts',(-0.0988990478901228,1.,4.14946408918485));
#40318=CARTESIAN_POINT('Ctrl Pts',(-0.0957412403298009,-1.,4.15660412653577));
#40319=CARTESIAN_POINT('Ctrl Pts',(-0.0957412403298009,1.,4.15660412653577));
#40320=CARTESIAN_POINT('Ctrl Pts',(-0.0925486672167534,-1.,4.16373802265839));
#40321=CARTESIAN_POINT('Ctrl Pts',(-0.0925486672167534,1.,4.16373802265839));
#40322=CARTESIAN_POINT('Ctrl Pts',(-0.0893215560848652,-1.,4.17086566490794));
#40323=CARTESIAN_POINT('Ctrl Pts',(-0.0893215560848652,1.,4.17086566490794));
#40324=CARTESIAN_POINT('Ctrl Pts',(-0.0860600915549399,-1.,4.17798698668094));
#40325=CARTESIAN_POINT('Ctrl Pts',(-0.0860600915549399,1.,4.17798698668094));
#40326=CARTESIAN_POINT('Ctrl Pts',(-0.0827644164385681,-1.,4.18510195327123));
#40327=CARTESIAN_POINT('Ctrl Pts',(-0.0827644164385681,1.,4.18510195327123));
#40328=CARTESIAN_POINT('Ctrl Pts',(-0.0801005887114322,-1.,4.19078883320504));
#40329=CARTESIAN_POINT('Ctrl Pts',(-0.0801005887114322,1.,4.19078883320504));
#40330=CARTESIAN_POINT('Ctrl Pts',(-0.07808739562424,-1.,4.19505112859416));
#40331=CARTESIAN_POINT('Ctrl Pts',(-0.07808739562424,1.,4.19505112859416));
#40332=CARTESIAN_POINT('Ctrl Pts',(-0.0767384596141467,-1.,4.1978913862118));
#40333=CARTESIAN_POINT('Ctrl Pts',(-0.0767384596141467,1.,4.1978913862118));
#40334=CARTESIAN_POINT('Ctrl Pts',(-0.0760622897878249,-1.,4.19931119685982));
#40335=CARTESIAN_POINT('Ctrl Pts',(-0.0760622897878249,1.,4.19931119685982));
#40336=CARTESIAN_POINT('',(-0.203156094896102,1.,3.74449296983004));
#40337=CARTESIAN_POINT('Ctrl Pts',(-0.203156094896101,-1.,3.74449296983004));
#40338=CARTESIAN_POINT('Ctrl Pts',(-0.203156094896101,-0.666666666666667,
3.74449296983004));
#40339=CARTESIAN_POINT('Ctrl Pts',(-0.203156094896101,-0.333333333333333,
3.74449296983004));
#40340=CARTESIAN_POINT('Ctrl Pts',(-0.203156094896101,0.333333333333333,
3.74449296983004));
#40341=CARTESIAN_POINT('Ctrl Pts',(-0.203156094896101,0.666666666666667,
3.74449296983004));
#40342=CARTESIAN_POINT('Ctrl Pts',(-0.203156094896101,1.,3.74449296983004));
#40343=CARTESIAN_POINT('',(-0.0760622897878249,1.,4.19931119685982));
#40344=CARTESIAN_POINT('',(-0.0760622897878249,0.,4.19931119685982));
#40345=CARTESIAN_POINT('Ctrl Pts',(-0.203156094896101,1.,3.74449296983004));
#40346=CARTESIAN_POINT('Ctrl Pts',(-0.203188003946657,1.,3.74453008995092));
#40347=CARTESIAN_POINT('Ctrl Pts',(-0.203266610110531,1.,3.74471097893845));
#40348=CARTESIAN_POINT('Ctrl Pts',(-0.203375226874122,1.,3.74535749969115));
#40349=CARTESIAN_POINT('Ctrl Pts',(-0.203484186269415,1.,3.74703926501752));
#40350=CARTESIAN_POINT('Ctrl Pts',(-0.203550035479166,1.,3.75054693397875));
#40351=CARTESIAN_POINT('Ctrl Pts',(-0.203530796848322,1.,3.75585118707734));
#40352=CARTESIAN_POINT('Ctrl Pts',(-0.203414634707479,1.,3.76242717936885));
#40353=CARTESIAN_POINT('Ctrl Pts',(-0.203192390045165,1.,3.7699207159487));
#40354=CARTESIAN_POINT('Ctrl Pts',(-0.202854729699081,1.,3.77793553476614));
#40355=CARTESIAN_POINT('Ctrl Pts',(-0.20239426051216,1.,3.78609175019242));
#40356=CARTESIAN_POINT('Ctrl Pts',(-0.201807533800837,1.,3.7940835418736));
#40357=CARTESIAN_POINT('Ctrl Pts',(-0.201097756307326,1.,3.80175247447337));
#40358=CARTESIAN_POINT('Ctrl Pts',(-0.200274679433365,1.,3.80909529318669));
#40359=CARTESIAN_POINT('Ctrl Pts',(-0.199351525297447,1.,3.81620203429815));
#40360=CARTESIAN_POINT('Ctrl Pts',(-0.198342616900487,1.,3.82321127349016));
#40361=CARTESIAN_POINT('Ctrl Pts',(-0.197260935827362,1.,3.83026221776456));
#40362=CARTESIAN_POINT('Ctrl Pts',(-0.196115198971859,1.,3.83743910616195));
#40363=CARTESIAN_POINT('Ctrl Pts',(-0.194909009460221,1.,3.84475203346977));
#40364=CARTESIAN_POINT('Ctrl Pts',(-0.193642806777723,1.,3.85216762263966));
#40365=CARTESIAN_POINT('Ctrl Pts',(-0.192315153044971,1.,3.85962774407633));
#40366=CARTESIAN_POINT('Ctrl Pts',(-0.19092419041862,1.,3.86707158624783));
#40367=CARTESIAN_POINT('Ctrl Pts',(-0.189469253358273,1.,3.87445976418412));
#40368=CARTESIAN_POINT('Ctrl Pts',(-0.187951632512685,1.,3.88178563496228));
#40369=CARTESIAN_POINT('Ctrl Pts',(-0.186373724985281,1.,3.88906196725848));
#40370=CARTESIAN_POINT('Ctrl Pts',(-0.184738537728043,1.,3.89631300742646));
#40371=CARTESIAN_POINT('Ctrl Pts',(-0.183049081993191,1.,3.90356488555132));
#40372=CARTESIAN_POINT('Ctrl Pts',(-0.181307740731786,1.,3.91083557557175));
#40373=CARTESIAN_POINT('Ctrl Pts',(-0.179515885822882,1.,3.91812876180926));
#40374=CARTESIAN_POINT('Ctrl Pts',(-0.177674246152318,1.,3.92543942697655));
#40375=CARTESIAN_POINT('Ctrl Pts',(-0.175783136893868,1.,3.93275726771042));
#40376=CARTESIAN_POINT('Ctrl Pts',(-0.17384273497461,1.,3.94007083096217));
#40377=CARTESIAN_POINT('Ctrl Pts',(-0.17185335536924,1.,3.94737164900868));
#40378=CARTESIAN_POINT('Ctrl Pts',(-0.169815666374139,1.,3.95465744665268));
#40379=CARTESIAN_POINT('Ctrl Pts',(-0.16773054702332,1.,3.96192990160296));
#40380=CARTESIAN_POINT('Ctrl Pts',(-0.165598992851102,1.,3.96919313621407));
#40381=CARTESIAN_POINT('Ctrl Pts',(-0.163422004609999,1.,3.97645194630943));
#40382=CARTESIAN_POINT('Ctrl Pts',(-0.161200482186085,1.,3.98371010319872));
#40383=CARTESIAN_POINT('Ctrl Pts',(-0.158935123982793,1.,3.99096873945878));
#40384=CARTESIAN_POINT('Ctrl Pts',(-0.156626481393734,1.,3.99822717425893));
#40385=CARTESIAN_POINT('Ctrl Pts',(-0.154275004872311,1.,4.00548360245319));
#40386=CARTESIAN_POINT('Ctrl Pts',(-0.151881094022911,1.,4.01273584234689));
#40387=CARTESIAN_POINT('Ctrl Pts',(-0.149445144968707,1.,4.01998203715564));
#40388=CARTESIAN_POINT('Ctrl Pts',(-0.146967602878994,1.,4.02722143146994));
#40389=CARTESIAN_POINT('Ctrl Pts',(-0.144448947038345,1.,4.03445411510333));
#40390=CARTESIAN_POINT('Ctrl Pts',(-0.1418896714855,1.,4.04168069633781));
#40391=CARTESIAN_POINT('Ctrl Pts',(-0.139290267180057,1.,4.04890199238036));
#40392=CARTESIAN_POINT('Ctrl Pts',(-0.136651205046119,1.,4.05611873400172));
#40393=CARTESIAN_POINT('Ctrl Pts',(-0.133972916144245,1.,4.06333121018596));
#40394=CARTESIAN_POINT('Ctrl Pts',(-0.131255793548941,1.,4.0705393152874));
#40395=CARTESIAN_POINT('Ctrl Pts',(-0.128500200484838,1.,4.07774270738954));
#40396=CARTESIAN_POINT('Ctrl Pts',(-0.12570647682254,1.,4.08494093372377));
#40397=CARTESIAN_POINT('Ctrl Pts',(-0.122874946249107,1.,4.09213355850756));
#40398=CARTESIAN_POINT('Ctrl Pts',(-0.120005924388124,1.,4.09932031767002));
#40399=CARTESIAN_POINT('Ctrl Pts',(-0.117099722731648,1.,4.10650113381833));
#40400=CARTESIAN_POINT('Ctrl Pts',(-0.114156649609546,1.,4.11367603924961));
#40401=CARTESIAN_POINT('Ctrl Pts',(-0.111177012683347,1.,4.1208451250225));
#40402=CARTESIAN_POINT('Ctrl Pts',(-0.10816112052837,1.,4.12800848371504));
#40403=CARTESIAN_POINT('Ctrl Pts',(-0.105109286538945,1.,4.13516614458895));
#40404=CARTESIAN_POINT('Ctrl Pts',(-0.102021826577584,1.,4.14231804939538));
#40405=CARTESIAN_POINT('Ctrl Pts',(-0.0988990478901228,1.,4.14946408918485));
#40406=CARTESIAN_POINT('Ctrl Pts',(-0.0957412403298009,1.,4.15660412653577));
#40407=CARTESIAN_POINT('Ctrl Pts',(-0.0925486672167534,1.,4.16373802265839));
#40408=CARTESIAN_POINT('Ctrl Pts',(-0.0893215560848652,1.,4.17086566490794));
#40409=CARTESIAN_POINT('Ctrl Pts',(-0.0860600915549399,1.,4.17798698668094));
#40410=CARTESIAN_POINT('Ctrl Pts',(-0.0827644164385681,1.,4.18510195327123));
#40411=CARTESIAN_POINT('Ctrl Pts',(-0.0801005887114322,1.,4.19078883320504));
#40412=CARTESIAN_POINT('Ctrl Pts',(-0.07808739562424,1.,4.19505112859416));
#40413=CARTESIAN_POINT('Ctrl Pts',(-0.0767384596141467,1.,4.1978913862118));
#40414=CARTESIAN_POINT('Ctrl Pts',(-0.0760622897878249,1.,4.19931119685982));
#40415=CARTESIAN_POINT('Origin',(-0.0760622897878249,0.,4.19931119685982));
#40416=CARTESIAN_POINT('',(0.0760622897878233,1.,4.19931119685982));
#40417=CARTESIAN_POINT('Origin',(0.,0.,0.));
#40418=CARTESIAN_POINT('',(-0.385112848330762,1.,3.73017266276651));
#40419=CARTESIAN_POINT('Origin',(0.,1.,0.));
#40420=CARTESIAN_POINT('Ctrl Pts',(-0.385112848330762,1.,3.73017266276651));
#40421=CARTESIAN_POINT('Ctrl Pts',(-0.385112848330762,0.666666666666667,
3.73017266276651));
#40422=CARTESIAN_POINT('Ctrl Pts',(-0.385112848330762,0.333333333333333,
3.73017266276651));
#40423=CARTESIAN_POINT('Ctrl Pts',(-0.385112848330762,-0.333333333333333,
3.73017266276651));
#40424=CARTESIAN_POINT('Ctrl Pts',(-0.385112848330762,-0.666666666666667,
3.73017266276651));
#40425=CARTESIAN_POINT('Ctrl Pts',(-0.385112848330762,-1.,3.73017266276651));
#40426=CARTESIAN_POINT('Ctrl Pts',(-0.581791163835815,-1.,4.15950947128175));
#40427=CARTESIAN_POINT('Ctrl Pts',(-0.581791163835815,1.,4.15950947128175));
#40428=CARTESIAN_POINT('Ctrl Pts',(-0.580901211463535,-1.,4.1582129171283));
#40429=CARTESIAN_POINT('Ctrl Pts',(-0.580901211463535,1.,4.1582129171283));
#40430=CARTESIAN_POINT('Ctrl Pts',(-0.579124568914235,-1.,4.15561864788576));
#40431=CARTESIAN_POINT('Ctrl Pts',(-0.579124568914235,1.,4.15561864788576));
#40432=CARTESIAN_POINT('Ctrl Pts',(-0.576469391676688,-1.,4.151723761217));
#40433=CARTESIAN_POINT('Ctrl Pts',(-0.576469391676688,1.,4.151723761217));
#40434=CARTESIAN_POINT('Ctrl Pts',(-0.572948736069522,-1.,4.14652361068081));
#40435=CARTESIAN_POINT('Ctrl Pts',(-0.572948736069522,1.,4.14652361068081));
#40436=CARTESIAN_POINT('Ctrl Pts',(-0.568580610189775,-1.,4.14001179830547));
#40437=CARTESIAN_POINT('Ctrl Pts',(-0.568580610189775,1.,4.14001179830547));
#40438=CARTESIAN_POINT('Ctrl Pts',(-0.564245279537149,-1.,4.13348835727104));
#40439=CARTESIAN_POINT('Ctrl Pts',(-0.564245279537149,1.,4.13348835727104));
#40440=CARTESIAN_POINT('Ctrl Pts',(-0.559942890594774,-1.,4.12695329951961));
#40441=CARTESIAN_POINT('Ctrl Pts',(-0.559942890594774,1.,4.12695329951961));
#40442=CARTESIAN_POINT('Ctrl Pts',(-0.555673636129977,-1.,4.12040666195664));
#40443=CARTESIAN_POINT('Ctrl Pts',(-0.555673636129977,1.,4.12040666195664));
#40444=CARTESIAN_POINT('Ctrl Pts',(-0.551437758497033,-1.,4.11384852024721));
#40445=CARTESIAN_POINT('Ctrl Pts',(-0.551437758497033,1.,4.11384852024721));
#40446=CARTESIAN_POINT('Ctrl Pts',(-0.547235539485637,-1.,4.10727897027977));
#40447=CARTESIAN_POINT('Ctrl Pts',(-0.547235539485637,1.,4.10727897027977));
#40448=CARTESIAN_POINT('Ctrl Pts',(-0.543067286877757,-1.,4.10069810243979));
#40449=CARTESIAN_POINT('Ctrl Pts',(-0.543067286877757,1.,4.10069810243979));
#40450=CARTESIAN_POINT('Ctrl Pts',(-0.538933321179756,-1.,4.09410597627));
#40451=CARTESIAN_POINT('Ctrl Pts',(-0.538933321179756,1.,4.09410597627));
#40452=CARTESIAN_POINT('Ctrl Pts',(-0.534833963477273,-1.,4.08750259988885));
#40453=CARTESIAN_POINT('Ctrl Pts',(-0.534833963477273,1.,4.08750259988885));
#40454=CARTESIAN_POINT('Ctrl Pts',(-0.530769518728571,-1.,4.08088789536836));
#40455=CARTESIAN_POINT('Ctrl Pts',(-0.530769518728571,1.,4.08088789536836));
#40456=CARTESIAN_POINT('Ctrl Pts',(-0.526740277227498,-1.,4.07426172299847));
#40457=CARTESIAN_POINT('Ctrl Pts',(-0.526740277227498,1.,4.07426172299847));
#40458=CARTESIAN_POINT('Ctrl Pts',(-0.522746528603107,-1.,4.06762394471314));
#40459=CARTESIAN_POINT('Ctrl Pts',(-0.522746528603107,1.,4.06762394471314));
#40460=CARTESIAN_POINT('Ctrl Pts',(-0.518788572336924,-1.,4.06097448038013));
#40461=CARTESIAN_POINT('Ctrl Pts',(-0.518788572336924,1.,4.06097448038013));
#40462=CARTESIAN_POINT('Ctrl Pts',(-0.514866728193017,-1.,4.05431335771199));
#40463=CARTESIAN_POINT('Ctrl Pts',(-0.514866728193017,1.,4.05431335771199));
#40464=CARTESIAN_POINT('Ctrl Pts',(-0.51098134921897,-1.,4.04764078815447));
#40465=CARTESIAN_POINT('Ctrl Pts',(-0.51098134921897,1.,4.04764078815447));
#40466=CARTESIAN_POINT('Ctrl Pts',(-0.507132823288136,-1.,4.04095715148915));
#40467=CARTESIAN_POINT('Ctrl Pts',(-0.507132823288136,1.,4.04095715148915));
#40468=CARTESIAN_POINT('Ctrl Pts',(-0.503321556915346,-1.,4.03426284174272));
#40469=CARTESIAN_POINT('Ctrl Pts',(-0.503321556915346,1.,4.03426284174272));
#40470=CARTESIAN_POINT('Ctrl Pts',(-0.499547962340821,-1.,4.02755813980101));
#40471=CARTESIAN_POINT('Ctrl Pts',(-0.499547962340821,1.,4.02755813980101));
#40472=CARTESIAN_POINT('Ctrl Pts',(-0.495812444326251,-1.,4.02084308851832));
#40473=CARTESIAN_POINT('Ctrl Pts',(-0.495812444326251,1.,4.02084308851832));
#40474=CARTESIAN_POINT('Ctrl Pts',(-0.492115383418018,-1.,4.01411733503546));
#40475=CARTESIAN_POINT('Ctrl Pts',(-0.492115383418018,1.,4.01411733503546));
#40476=CARTESIAN_POINT('Ctrl Pts',(-0.488457130424633,-1.,4.0073800839099));
#40477=CARTESIAN_POINT('Ctrl Pts',(-0.488457130424633,1.,4.0073800839099));
#40478=CARTESIAN_POINT('Ctrl Pts',(-0.484838042421835,-1.,4.00063045119288));
#40479=CARTESIAN_POINT('Ctrl Pts',(-0.484838042421835,1.,4.00063045119288));
#40480=CARTESIAN_POINT('Ctrl Pts',(-0.481258512209675,-1.,3.99386775880679));
#40481=CARTESIAN_POINT('Ctrl Pts',(-0.481258512209675,1.,3.99386775880679));
#40482=CARTESIAN_POINT('Ctrl Pts',(-0.477718999122027,-1.,3.98709184306738));
#40483=CARTESIAN_POINT('Ctrl Pts',(-0.477718999122027,1.,3.98709184306738));
#40484=CARTESIAN_POINT('Ctrl Pts',(-0.47422006101951,-1.,3.98030338044409));
#40485=CARTESIAN_POINT('Ctrl Pts',(-0.47422006101951,1.,3.98030338044409));
#40486=CARTESIAN_POINT('Ctrl Pts',(-0.470762379613439,-1.,3.97350414289392));
#40487=CARTESIAN_POINT('Ctrl Pts',(-0.470762379613439,1.,3.97350414289392));
#40488=CARTESIAN_POINT('Ctrl Pts',(-0.467346690880643,-1.,3.9666962227393));
#40489=CARTESIAN_POINT('Ctrl Pts',(-0.467346690880643,1.,3.9666962227393));
#40490=CARTESIAN_POINT('Ctrl Pts',(-0.463973722115733,-1.,3.95988133243538));
#40491=CARTESIAN_POINT('Ctrl Pts',(-0.463973722115733,1.,3.95988133243538));
#40492=CARTESIAN_POINT('Ctrl Pts',(-0.460644124429121,-1.,3.95306005817364));
#40493=CARTESIAN_POINT('Ctrl Pts',(-0.460644124429121,1.,3.95306005817364));
#40494=CARTESIAN_POINT('Ctrl Pts',(-0.457358410451683,-1.,3.94623117206678));
#40495=CARTESIAN_POINT('Ctrl Pts',(-0.457358410451683,1.,3.94623117206678));
#40496=CARTESIAN_POINT('Ctrl Pts',(-0.454116879027584,-1.,3.93939080846298));
#40497=CARTESIAN_POINT('Ctrl Pts',(-0.454116879027584,1.,3.93939080846298));
#40498=CARTESIAN_POINT('Ctrl Pts',(-0.450919768356348,-1.,3.93253407403123));
#40499=CARTESIAN_POINT('Ctrl Pts',(-0.450919768356348,1.,3.93253407403123));
#40500=CARTESIAN_POINT('Ctrl Pts',(-0.447767416837293,-1.,3.92565674143416));
#40501=CARTESIAN_POINT('Ctrl Pts',(-0.447767416837293,1.,3.92565674143416));
#40502=CARTESIAN_POINT('Ctrl Pts',(-0.444660430230591,-1.,3.91875701610719));
#40503=CARTESIAN_POINT('Ctrl Pts',(-0.444660430230591,1.,3.91875701610719));
#40504=CARTESIAN_POINT('Ctrl Pts',(-0.441599824524054,-1.,3.91183704069153));
#40505=CARTESIAN_POINT('Ctrl Pts',(-0.441599824524054,1.,3.91183704069153));
#40506=CARTESIAN_POINT('Ctrl Pts',(-0.43858723545825,-1.,3.90490512938563));
#40507=CARTESIAN_POINT('Ctrl Pts',(-0.43858723545825,1.,3.90490512938563));
#40508=CARTESIAN_POINT('Ctrl Pts',(-0.435624629433528,-1.,3.89797256655462));
#40509=CARTESIAN_POINT('Ctrl Pts',(-0.435624629433528,1.,3.89797256655462));
#40510=CARTESIAN_POINT('Ctrl Pts',(-0.432713929544458,-1.,3.89104947940611));
#40511=CARTESIAN_POINT('Ctrl Pts',(-0.432713929544458,1.,3.89104947940611));
#40512=CARTESIAN_POINT('Ctrl Pts',(-0.429856640579741,-1.,3.88414070943341));
#40513=CARTESIAN_POINT('Ctrl Pts',(-0.429856640579741,1.,3.88414070943341));
#40514=CARTESIAN_POINT('Ctrl Pts',(-0.427053541173457,-1.,3.87724240306597));
#40515=CARTESIAN_POINT('Ctrl Pts',(-0.427053541173457,1.,3.87724240306597));
#40516=CARTESIAN_POINT('Ctrl Pts',(-0.424304173195111,-1.,3.87033643487851));
#40517=CARTESIAN_POINT('Ctrl Pts',(-0.424304173195111,1.,3.87033643487851));
#40518=CARTESIAN_POINT('Ctrl Pts',(-0.421607423177534,-1.,3.86339652542709));
#40519=CARTESIAN_POINT('Ctrl Pts',(-0.421607423177534,1.,3.86339652542709));
#40520=CARTESIAN_POINT('Ctrl Pts',(-0.418962468086773,-1.,3.85639825647996));
#40521=CARTESIAN_POINT('Ctrl Pts',(-0.418962468086773,1.,3.85639825647996));
#40522=CARTESIAN_POINT('Ctrl Pts',(-0.416369678052907,-1.,3.84932864157497));
#40523=CARTESIAN_POINT('Ctrl Pts',(-0.416369678052907,1.,3.84932864157497));
#40524=CARTESIAN_POINT('Ctrl Pts',(-0.413831367016748,-1.,3.84219403994762));
#40525=CARTESIAN_POINT('Ctrl Pts',(-0.413831367016748,1.,3.84219403994762));
#40526=CARTESIAN_POINT('Ctrl Pts',(-0.411353038798519,-1.,3.83503345578698));
#40527=CARTESIAN_POINT('Ctrl Pts',(-0.411353038798519,1.,3.83503345578698));
#40528=CARTESIAN_POINT('Ctrl Pts',(-0.40894237144746,-1.,3.82790724256471));
#40529=CARTESIAN_POINT('Ctrl Pts',(-0.40894237144746,1.,3.82790724256471));
#40530=CARTESIAN_POINT('Ctrl Pts',(-0.406607038258985,-1.,3.8208730391381));
#40531=CARTESIAN_POINT('Ctrl Pts',(-0.406607038258985,1.,3.8208730391381));
#40532=CARTESIAN_POINT('Ctrl Pts',(-0.404352694628273,-1.,3.81396374287793));
#40533=CARTESIAN_POINT('Ctrl Pts',(-0.404352694628273,1.,3.81396374287793));
#40534=CARTESIAN_POINT('Ctrl Pts',(-0.402181320148436,-1.,3.80716881962728));
#40535=CARTESIAN_POINT('Ctrl Pts',(-0.402181320148436,1.,3.80716881962728));
#40536=CARTESIAN_POINT('Ctrl Pts',(-0.4000883465046,-1.,3.80040370384546));
#40537=CARTESIAN_POINT('Ctrl Pts',(-0.4000883465046,1.,3.80040370384546));
#40538=CARTESIAN_POINT('Ctrl Pts',(-0.39806481868397,-1.,3.7935288716329));
#40539=CARTESIAN_POINT('Ctrl Pts',(-0.39806481868397,1.,3.7935288716329));
#40540=CARTESIAN_POINT('Ctrl Pts',(-0.396103205334841,-1.,3.78640521279313));
#40541=CARTESIAN_POINT('Ctrl Pts',(-0.396103205334841,1.,3.78640521279313));
#40542=CARTESIAN_POINT('Ctrl Pts',(-0.394202481011499,-1.,3.77894173114283));
#40543=CARTESIAN_POINT('Ctrl Pts',(-0.394202481011499,1.,3.77894173114283));
#40544=CARTESIAN_POINT('Ctrl Pts',(-0.392372786223433,-1.,3.77114011595967));
#40545=CARTESIAN_POINT('Ctrl Pts',(-0.392372786223433,1.,3.77114011595967));
#40546=CARTESIAN_POINT('Ctrl Pts',(-0.39064207297956,-1.,3.76315635033257));
#40547=CARTESIAN_POINT('Ctrl Pts',(-0.39064207297956,1.,3.76315635033257));
#40548=CARTESIAN_POINT('Ctrl Pts',(-0.389054775898702,-1.,3.75529302895152));
#40549=CARTESIAN_POINT('Ctrl Pts',(-0.389054775898702,1.,3.75529302895152));
#40550=CARTESIAN_POINT('Ctrl Pts',(-0.387663020050836,-1.,3.74792651696654));
#40551=CARTESIAN_POINT('Ctrl Pts',(-0.387663020050836,1.,3.74792651696654));
#40552=CARTESIAN_POINT('Ctrl Pts',(-0.386519576222251,-1.,3.74144965781276));
#40553=CARTESIAN_POINT('Ctrl Pts',(-0.386519576222251,1.,3.74144965781276));
#40554=CARTESIAN_POINT('Ctrl Pts',(-0.385670806454566,-1.,3.73621371845318));
#40555=CARTESIAN_POINT('Ctrl Pts',(-0.385670806454566,1.,3.73621371845318));
#40556=CARTESIAN_POINT('Ctrl Pts',(-0.385147887988951,-1.,3.73245705638843));
#40557=CARTESIAN_POINT('Ctrl Pts',(-0.385147887988951,1.,3.73245705638843));
#40558=CARTESIAN_POINT('Ctrl Pts',(-0.385001870183213,-1.,3.73072465900175));
#40559=CARTESIAN_POINT('Ctrl Pts',(-0.385001870183213,1.,3.73072465900175));
#40560=CARTESIAN_POINT('Ctrl Pts',(-0.385047711603462,-1.,3.73015851028356));
#40561=CARTESIAN_POINT('Ctrl Pts',(-0.385047711603462,1.,3.73015851028356));
#40562=CARTESIAN_POINT('Ctrl Pts',(-0.385147278814642,-1.,3.73010668803042));
#40563=CARTESIAN_POINT('Ctrl Pts',(-0.385147278814642,1.,3.73010668803042));
#40564=CARTESIAN_POINT('Ctrl Pts',(-0.38521431477633,-1.,3.73016218570874));
#40565=CARTESIAN_POINT('Ctrl Pts',(-0.38521431477633,1.,3.73016218570874));
#40566=CARTESIAN_POINT('',(-0.581791163835815,1.,4.15950947128175));
#40567=CARTESIAN_POINT('Ctrl Pts',(-0.581791163835815,1.,4.15950947128175));
#40568=CARTESIAN_POINT('Ctrl Pts',(-0.580901211463535,1.,4.1582129171283));
#40569=CARTESIAN_POINT('Ctrl Pts',(-0.579124568914235,1.,4.15561864788576));
#40570=CARTESIAN_POINT('Ctrl Pts',(-0.576469391676688,1.,4.151723761217));
#40571=CARTESIAN_POINT('Ctrl Pts',(-0.572948736069522,1.,4.14652361068081));
#40572=CARTESIAN_POINT('Ctrl Pts',(-0.568580610189775,1.,4.14001179830547));
#40573=CARTESIAN_POINT('Ctrl Pts',(-0.564245279537149,1.,4.13348835727104));
#40574=CARTESIAN_POINT('Ctrl Pts',(-0.559942890594774,1.,4.12695329951961));
#40575=CARTESIAN_POINT('Ctrl Pts',(-0.555673636129977,1.,4.12040666195664));
#40576=CARTESIAN_POINT('Ctrl Pts',(-0.551437758497033,1.,4.11384852024721));
#40577=CARTESIAN_POINT('Ctrl Pts',(-0.547235539485637,1.,4.10727897027977));
#40578=CARTESIAN_POINT('Ctrl Pts',(-0.543067286877757,1.,4.10069810243979));
#40579=CARTESIAN_POINT('Ctrl Pts',(-0.538933321179756,1.,4.09410597627));
#40580=CARTESIAN_POINT('Ctrl Pts',(-0.534833963477273,1.,4.08750259988885));
#40581=CARTESIAN_POINT('Ctrl Pts',(-0.530769518728571,1.,4.08088789536836));
#40582=CARTESIAN_POINT('Ctrl Pts',(-0.526740277227498,1.,4.07426172299847));
#40583=CARTESIAN_POINT('Ctrl Pts',(-0.522746528603107,1.,4.06762394471314));
#40584=CARTESIAN_POINT('Ctrl Pts',(-0.518788572336924,1.,4.06097448038013));
#40585=CARTESIAN_POINT('Ctrl Pts',(-0.514866728193017,1.,4.05431335771199));
#40586=CARTESIAN_POINT('Ctrl Pts',(-0.51098134921897,1.,4.04764078815447));
#40587=CARTESIAN_POINT('Ctrl Pts',(-0.507132823288136,1.,4.04095715148915));
#40588=CARTESIAN_POINT('Ctrl Pts',(-0.503321556915346,1.,4.03426284174272));
#40589=CARTESIAN_POINT('Ctrl Pts',(-0.499547962340821,1.,4.02755813980101));
#40590=CARTESIAN_POINT('Ctrl Pts',(-0.495812444326251,1.,4.02084308851832));
#40591=CARTESIAN_POINT('Ctrl Pts',(-0.492115383418018,1.,4.01411733503546));
#40592=CARTESIAN_POINT('Ctrl Pts',(-0.488457130424633,1.,4.0073800839099));
#40593=CARTESIAN_POINT('Ctrl Pts',(-0.484838042421835,1.,4.00063045119288));
#40594=CARTESIAN_POINT('Ctrl Pts',(-0.481258512209675,1.,3.99386775880679));
#40595=CARTESIAN_POINT('Ctrl Pts',(-0.477718999122027,1.,3.98709184306738));
#40596=CARTESIAN_POINT('Ctrl Pts',(-0.47422006101951,1.,3.98030338044409));
#40597=CARTESIAN_POINT('Ctrl Pts',(-0.470762379613439,1.,3.97350414289392));
#40598=CARTESIAN_POINT('Ctrl Pts',(-0.467346690880643,1.,3.9666962227393));
#40599=CARTESIAN_POINT('Ctrl Pts',(-0.463973722115733,1.,3.95988133243538));
#40600=CARTESIAN_POINT('Ctrl Pts',(-0.460644124429121,1.,3.95306005817364));
#40601=CARTESIAN_POINT('Ctrl Pts',(-0.457358410451683,1.,3.94623117206678));
#40602=CARTESIAN_POINT('Ctrl Pts',(-0.454116879027584,1.,3.93939080846298));
#40603=CARTESIAN_POINT('Ctrl Pts',(-0.450919768356348,1.,3.93253407403123));
#40604=CARTESIAN_POINT('Ctrl Pts',(-0.447767416837293,1.,3.92565674143416));
#40605=CARTESIAN_POINT('Ctrl Pts',(-0.444660430230591,1.,3.91875701610719));
#40606=CARTESIAN_POINT('Ctrl Pts',(-0.441599824524054,1.,3.91183704069153));
#40607=CARTESIAN_POINT('Ctrl Pts',(-0.43858723545825,1.,3.90490512938563));
#40608=CARTESIAN_POINT('Ctrl Pts',(-0.435624629433528,1.,3.89797256655462));
#40609=CARTESIAN_POINT('Ctrl Pts',(-0.432713929544458,1.,3.89104947940611));
#40610=CARTESIAN_POINT('Ctrl Pts',(-0.429856640579741,1.,3.88414070943341));
#40611=CARTESIAN_POINT('Ctrl Pts',(-0.427053541173457,1.,3.87724240306597));
#40612=CARTESIAN_POINT('Ctrl Pts',(-0.424304173195111,1.,3.87033643487851));
#40613=CARTESIAN_POINT('Ctrl Pts',(-0.421607423177534,1.,3.86339652542709));
#40614=CARTESIAN_POINT('Ctrl Pts',(-0.418962468086773,1.,3.85639825647996));
#40615=CARTESIAN_POINT('Ctrl Pts',(-0.416369678052907,1.,3.84932864157497));
#40616=CARTESIAN_POINT('Ctrl Pts',(-0.413831367016748,1.,3.84219403994762));
#40617=CARTESIAN_POINT('Ctrl Pts',(-0.411353038798519,1.,3.83503345578698));
#40618=CARTESIAN_POINT('Ctrl Pts',(-0.40894237144746,1.,3.82790724256471));
#40619=CARTESIAN_POINT('Ctrl Pts',(-0.406607038258985,1.,3.8208730391381));
#40620=CARTESIAN_POINT('Ctrl Pts',(-0.404352694628273,1.,3.81396374287793));
#40621=CARTESIAN_POINT('Ctrl Pts',(-0.402181320148436,1.,3.80716881962728));
#40622=CARTESIAN_POINT('Ctrl Pts',(-0.4000883465046,1.,3.80040370384546));
#40623=CARTESIAN_POINT('Ctrl Pts',(-0.39806481868397,1.,3.7935288716329));
#40624=CARTESIAN_POINT('Ctrl Pts',(-0.396103205334841,1.,3.78640521279313));
#40625=CARTESIAN_POINT('Ctrl Pts',(-0.394202481011499,1.,3.77894173114283));
#40626=CARTESIAN_POINT('Ctrl Pts',(-0.392372786223433,1.,3.77114011595967));
#40627=CARTESIAN_POINT('Ctrl Pts',(-0.39064207297956,1.,3.76315635033257));
#40628=CARTESIAN_POINT('Ctrl Pts',(-0.389054775898702,1.,3.75529302895152));
#40629=CARTESIAN_POINT('Ctrl Pts',(-0.387663020050836,1.,3.74792651696654));
#40630=CARTESIAN_POINT('Ctrl Pts',(-0.386519576222251,1.,3.74144965781276));
#40631=CARTESIAN_POINT('Ctrl Pts',(-0.385670806454566,1.,3.73621371845318));
#40632=CARTESIAN_POINT('Ctrl Pts',(-0.385187124634206,1.,3.73273893363406));
#40633=CARTESIAN_POINT('Ctrl Pts',(-0.385031656499164,1.,3.73106082862548));
#40634=CARTESIAN_POINT('Ctrl Pts',(-0.385037797881504,1.,3.73040527621055));
#40635=CARTESIAN_POINT('Ctrl Pts',(-0.385087139000375,1.,3.73021431755274));
#40636=CARTESIAN_POINT('Ctrl Pts',(-0.385112848330762,1.,3.73017266276651));
#40637=CARTESIAN_POINT('',(-0.581791163835815,0.,4.15950947128175));
#40638=CARTESIAN_POINT('Ctrl Pts',(-0.7863229229206,-1.,3.66663282329846));
#40639=CARTESIAN_POINT('Ctrl Pts',(-0.7863229229206,1.,3.66663282329846));
#40640=CARTESIAN_POINT('Ctrl Pts',(-0.786369528183326,-1.,3.66655932661986));
#40641=CARTESIAN_POINT('Ctrl Pts',(-0.786369528183326,1.,3.66655932661986));
#40642=CARTESIAN_POINT('Ctrl Pts',(-0.786480236185697,-1.,3.66657784455334));
#40643=CARTESIAN_POINT('Ctrl Pts',(-0.786480236185697,1.,3.66657784455334));
#40644=CARTESIAN_POINT('Ctrl Pts',(-0.786698783542764,-1.,3.66710211820482));
#40645=CARTESIAN_POINT('Ctrl Pts',(-0.786698783542764,1.,3.66710211820482));
#40646=CARTESIAN_POINT('Ctrl Pts',(-0.787095252590501,-1.,3.66879484801113));
#40647=CARTESIAN_POINT('Ctrl Pts',(-0.787095252590501,1.,3.66879484801113));
#40648=CARTESIAN_POINT('Ctrl Pts',(-0.787758799995743,-1.,3.67252923663655));
#40649=CARTESIAN_POINT('Ctrl Pts',(-0.787758799995743,1.,3.67252923663655));
#40650=CARTESIAN_POINT('Ctrl Pts',(-0.788569566220285,-1.,3.67777119516252));
#40651=CARTESIAN_POINT('Ctrl Pts',(-0.788569566220285,1.,3.67777119516252));
#40652=CARTESIAN_POINT('Ctrl Pts',(-0.789483546064387,-1.,3.68428439783905));
#40653=CARTESIAN_POINT('Ctrl Pts',(-0.789483546064387,1.,3.68428439783905));
#40654=CARTESIAN_POINT('Ctrl Pts',(-0.790436284988788,-1.,3.69172044327364));
#40655=CARTESIAN_POINT('Ctrl Pts',(-0.790436284988788,1.,3.69172044327364));
#40656=CARTESIAN_POINT('Ctrl Pts',(-0.79135657569598,-1.,3.69968940808721));
#40657=CARTESIAN_POINT('Ctrl Pts',(-0.79135657569598,1.,3.69968940808721));
#40658=CARTESIAN_POINT('Ctrl Pts',(-0.792177688845818,-1.,3.70781724021806));
#40659=CARTESIAN_POINT('Ctrl Pts',(-0.792177688845818,1.,3.70781724021806));
#40660=CARTESIAN_POINT('Ctrl Pts',(-0.792848377370287,-1.,3.71580242396124));
#40661=CARTESIAN_POINT('Ctrl Pts',(-0.792848377370287,1.,3.71580242396124));
#40662=CARTESIAN_POINT('Ctrl Pts',(-0.793347023784205,-1.,3.72348797293734));
#40663=CARTESIAN_POINT('Ctrl Pts',(-0.793347023784205,1.,3.72348797293734));
#40664=CARTESIAN_POINT('Ctrl Pts',(-0.793682750269684,-1.,3.73086914695805));
#40665=CARTESIAN_POINT('Ctrl Pts',(-0.793682750269684,1.,3.73086914695805));
#40666=CARTESIAN_POINT('Ctrl Pts',(-0.793882700937017,-1.,3.73803280541687));
#40667=CARTESIAN_POINT('Ctrl Pts',(-0.793882700937017,1.,3.73803280541687));
#40668=CARTESIAN_POINT('Ctrl Pts',(-0.793982700459952,-1.,3.74511357728861));
#40669=CARTESIAN_POINT('Ctrl Pts',(-0.793982700459952,1.,3.74511357728861));
#40670=CARTESIAN_POINT('Ctrl Pts',(-0.794017347371377,-1.,3.75224692493864));
#40671=CARTESIAN_POINT('Ctrl Pts',(-0.794017347371377,1.,3.75224692493864));
#40672=CARTESIAN_POINT('Ctrl Pts',(-0.794008429134907,-1.,3.75951468666257));
#40673=CARTESIAN_POINT('Ctrl Pts',(-0.794008429134907,1.,3.75951468666257));
#40674=CARTESIAN_POINT('Ctrl Pts',(-0.793961083688992,-1.,3.76692626931111));
#40675=CARTESIAN_POINT('Ctrl Pts',(-0.793961083688992,1.,3.76692626931111));
#40676=CARTESIAN_POINT('Ctrl Pts',(-0.793870523787408,-1.,3.77444863801212));
#40677=CARTESIAN_POINT('Ctrl Pts',(-0.793870523787408,1.,3.77444863801212));
#40678=CARTESIAN_POINT('Ctrl Pts',(-0.7937262357813,-1.,3.78202460377598));
#40679=CARTESIAN_POINT('Ctrl Pts',(-0.7937262357813,1.,3.78202460377598));
#40680=CARTESIAN_POINT('Ctrl Pts',(-0.793516871680993,-1.,3.78959439439235));
#40681=CARTESIAN_POINT('Ctrl Pts',(-0.793516871680993,1.,3.78959439439235));
#40682=CARTESIAN_POINT('Ctrl Pts',(-0.793235612973273,-1.,3.79711921389897));
#40683=CARTESIAN_POINT('Ctrl Pts',(-0.793235612973273,1.,3.79711921389897));
#40684=CARTESIAN_POINT('Ctrl Pts',(-0.792882695234778,-1.,3.80459229925637));
#40685=CARTESIAN_POINT('Ctrl Pts',(-0.792882695234778,1.,3.80459229925637));
#40686=CARTESIAN_POINT('Ctrl Pts',(-0.792462483517634,-1.,3.81202588694756));
#40687=CARTESIAN_POINT('Ctrl Pts',(-0.792462483517634,1.,3.81202588694756));
#40688=CARTESIAN_POINT('Ctrl Pts',(-0.791981740718635,-1.,3.81944345442249));
#40689=CARTESIAN_POINT('Ctrl Pts',(-0.791981740718635,1.,3.81944345442249));
#40690=CARTESIAN_POINT('Ctrl Pts',(-0.791447528662369,-1.,3.82687033899792));
#40691=CARTESIAN_POINT('Ctrl Pts',(-0.791447528662369,1.,3.82687033899792));
#40692=CARTESIAN_POINT('Ctrl Pts',(-0.790865012705301,-1.,3.83432392054786));
#40693=CARTESIAN_POINT('Ctrl Pts',(-0.790865012705301,1.,3.83432392054786));
#40694=CARTESIAN_POINT('Ctrl Pts',(-0.790236124191242,-1.,3.84180762342454));
#40695=CARTESIAN_POINT('Ctrl Pts',(-0.790236124191242,1.,3.84180762342454));
#40696=CARTESIAN_POINT('Ctrl Pts',(-0.789560798155582,-1.,3.84931637808894));
#40697=CARTESIAN_POINT('Ctrl Pts',(-0.789560798155582,1.,3.84931637808894));
#40698=CARTESIAN_POINT('Ctrl Pts',(-0.788837734090672,-1.,3.85683995872529));
#40699=CARTESIAN_POINT('Ctrl Pts',(-0.788837734090672,1.,3.85683995872529));
#40700=CARTESIAN_POINT('Ctrl Pts',(-0.788065315093778,-1.,3.86436702561345));
#40701=CARTESIAN_POINT('Ctrl Pts',(-0.788065315093778,1.,3.86436702561345));
#40702=CARTESIAN_POINT('Ctrl Pts',(-0.787242527617999,-1.,3.87188916600912));
#40703=CARTESIAN_POINT('Ctrl Pts',(-0.787242527617999,1.,3.87188916600912));
#40704=CARTESIAN_POINT('Ctrl Pts',(-0.786369675812609,-1.,3.8794040281819));
#40705=CARTESIAN_POINT('Ctrl Pts',(-0.786369675812609,1.,3.8794040281819));
#40706=CARTESIAN_POINT('Ctrl Pts',(-0.78544789034073,-1.,3.88691313167398));
#40707=CARTESIAN_POINT('Ctrl Pts',(-0.78544789034073,1.,3.88691313167398));
#40708=CARTESIAN_POINT('Ctrl Pts',(-0.784478799358336,-1.,3.89442039235103));
#40709=CARTESIAN_POINT('Ctrl Pts',(-0.784478799358336,1.,3.89442039235103));
#40710=CARTESIAN_POINT('Ctrl Pts',(-0.783464141529081,-1.,3.9019303904397));
#40711=CARTESIAN_POINT('Ctrl Pts',(-0.783464141529081,1.,3.9019303904397));
#40712=CARTESIAN_POINT('Ctrl Pts',(-0.782405395622764,-1.,3.90944671004542));
#40713=CARTESIAN_POINT('Ctrl Pts',(-0.782405395622764,1.,3.90944671004542));
#40714=CARTESIAN_POINT('Ctrl Pts',(-0.781303428618367,-1.,3.91697036054676));
#40715=CARTESIAN_POINT('Ctrl Pts',(-0.781303428618367,1.,3.91697036054676));
#40716=CARTESIAN_POINT('Ctrl Pts',(-0.780158678615543,-1.,3.92450058323823));
#40717=CARTESIAN_POINT('Ctrl Pts',(-0.780158678615543,1.,3.92450058323823));
#40718=CARTESIAN_POINT('Ctrl Pts',(-0.778971308134821,-1.,3.93203552473174));
#40719=CARTESIAN_POINT('Ctrl Pts',(-0.778971308134821,1.,3.93203552473174));
#40720=CARTESIAN_POINT('Ctrl Pts',(-0.777741370568559,-1.,3.93957296768103));
#40721=CARTESIAN_POINT('Ctrl Pts',(-0.777741370568559,1.,3.93957296768103));
#40722=CARTESIAN_POINT('Ctrl Pts',(-0.776468966697921,-1.,3.94711101619447));
#40723=CARTESIAN_POINT('Ctrl Pts',(-0.776468966697921,1.,3.94711101619447));
#40724=CARTESIAN_POINT('Ctrl Pts',(-0.775154418039352,-1.,3.9546488545231));
#40725=CARTESIAN_POINT('Ctrl Pts',(-0.775154418039352,1.,3.9546488545231));
#40726=CARTESIAN_POINT('Ctrl Pts',(-0.773798212026566,-1.,3.96218649639807));
#40727=CARTESIAN_POINT('Ctrl Pts',(-0.773798212026566,1.,3.96218649639807));
#40728=CARTESIAN_POINT('Ctrl Pts',(-0.772400931772136,-1.,3.96972446532772));
#40729=CARTESIAN_POINT('Ctrl Pts',(-0.772400931772136,1.,3.96972446532772));
#40730=CARTESIAN_POINT('Ctrl Pts',(-0.770963190030471,-1.,3.97726349165488));
#40731=CARTESIAN_POINT('Ctrl Pts',(-0.770963190030471,1.,3.97726349165488));
#40732=CARTESIAN_POINT('Ctrl Pts',(-0.769485566245544,-1.,3.98480422348451));
#40733=CARTESIAN_POINT('Ctrl Pts',(-0.769485566245544,1.,3.98480422348451));
#40734=CARTESIAN_POINT('Ctrl Pts',(-0.767968531377915,-1.,3.9923468788101));
#40735=CARTESIAN_POINT('Ctrl Pts',(-0.767968531377915,1.,3.9923468788101));
#40736=CARTESIAN_POINT('Ctrl Pts',(-0.766412457136064,-1.,3.99989129179622));
#40737=CARTESIAN_POINT('Ctrl Pts',(-0.766412457136064,1.,3.99989129179622));
#40738=CARTESIAN_POINT('Ctrl Pts',(-0.764817648785198,-1.,4.00743706791509));
#40739=CARTESIAN_POINT('Ctrl Pts',(-0.764817648785198,1.,4.00743706791509));
#40740=CARTESIAN_POINT('Ctrl Pts',(-0.763184371182935,-1.,4.01498370680496));
#40741=CARTESIAN_POINT('Ctrl Pts',(-0.763184371182935,1.,4.01498370680496));
#40742=CARTESIAN_POINT('Ctrl Pts',(-0.761512875859804,-1.,4.02253072741268));
#40743=CARTESIAN_POINT('Ctrl Pts',(-0.761512875859804,1.,4.02253072741268));
#40744=CARTESIAN_POINT('Ctrl Pts',(-0.759803433243752,-1.,4.03007781954412));
#40745=CARTESIAN_POINT('Ctrl Pts',(-0.759803433243752,1.,4.03007781954412));
#40746=CARTESIAN_POINT('Ctrl Pts',(-0.758056338884944,-1.,4.03762485803119));
#40747=CARTESIAN_POINT('Ctrl Pts',(-0.758056338884944,1.,4.03762485803119));
#40748=CARTESIAN_POINT('Ctrl Pts',(-0.756271902369581,-1.,4.04517182653997));
#40749=CARTESIAN_POINT('Ctrl Pts',(-0.756271902369581,1.,4.04517182653997));
#40750=CARTESIAN_POINT('Ctrl Pts',(-0.754450441816078,-1.,4.05271876687915));
#40751=CARTESIAN_POINT('Ctrl Pts',(-0.754450441816078,1.,4.05271876687915));
#40752=CARTESIAN_POINT('Ctrl Pts',(-0.752592276483072,-1.,4.06026572221515));
#40753=CARTESIAN_POINT('Ctrl Pts',(-0.752592276483072,1.,4.06026572221515));
#40754=CARTESIAN_POINT('Ctrl Pts',(-0.750697720484036,-1.,4.06781267242378));
#40755=CARTESIAN_POINT('Ctrl Pts',(-0.750697720484036,1.,4.06781267242378));
#40756=CARTESIAN_POINT('Ctrl Pts',(-0.748767076680557,-1.,4.07535951056152));
#40757=CARTESIAN_POINT('Ctrl Pts',(-0.748767076680557,1.,4.07535951056152));
#40758=CARTESIAN_POINT('Ctrl Pts',(-0.746800631492315,-1.,4.08290608095642));
#40759=CARTESIAN_POINT('Ctrl Pts',(-0.746800631492315,1.,4.08290608095642));
#40760=CARTESIAN_POINT('Ctrl Pts',(-0.7447986497065,-1.,4.09045220253573));
#40761=CARTESIAN_POINT('Ctrl Pts',(-0.7447986497065,1.,4.09045220253573));
#40762=CARTESIAN_POINT('Ctrl Pts',(-0.742761369689841,-1.,4.09799769702611));
#40763=CARTESIAN_POINT('Ctrl Pts',(-0.742761369689841,1.,4.09799769702611));
#40764=CARTESIAN_POINT('Ctrl Pts',(-0.740688998553377,-1.,4.10554241757547));
#40765=CARTESIAN_POINT('Ctrl Pts',(-0.740688998553377,1.,4.10554241757547));
#40766=CARTESIAN_POINT('Ctrl Pts',(-0.738581708225844,-1.,4.11308626951927));
#40767=CARTESIAN_POINT('Ctrl Pts',(-0.738581708225844,1.,4.11308626951927));
#40768=CARTESIAN_POINT('Ctrl Pts',(-0.736439634331345,-1.,4.120629196238));
#40769=CARTESIAN_POINT('Ctrl Pts',(-0.736439634331345,1.,4.120629196238));
#40770=CARTESIAN_POINT('Ctrl Pts',(-0.734698226764092,-1.,4.12666277570844));
#40771=CARTESIAN_POINT('Ctrl Pts',(-0.734698226764092,1.,4.12666277570844));
#40772=CARTESIAN_POINT('Ctrl Pts',(-0.733376589323546,-1.,4.13118752795207));
#40773=CARTESIAN_POINT('Ctrl Pts',(-0.733376589323546,1.,4.13118752795207));
#40774=CARTESIAN_POINT('Ctrl Pts',(-0.73248857513516,-1.,4.1342038373684));
#40775=CARTESIAN_POINT('Ctrl Pts',(-0.73248857513516,1.,4.1342038373684));
#40776=CARTESIAN_POINT('Ctrl Pts',(-0.73204283740062,-1.,4.13571194405636));
#40777=CARTESIAN_POINT('Ctrl Pts',(-0.73204283740062,1.,4.13571194405636));
#40778=CARTESIAN_POINT('',(-0.786422660831985,1.,3.66661143271685));
#40779=CARTESIAN_POINT('Ctrl Pts',(-0.786422660831985,-1.,3.66661143271685));
#40780=CARTESIAN_POINT('Ctrl Pts',(-0.786422660831985,-0.666666666666667,
3.66661143271685));
#40781=CARTESIAN_POINT('Ctrl Pts',(-0.786422660831985,-0.333333333333333,
3.66661143271685));
#40782=CARTESIAN_POINT('Ctrl Pts',(-0.786422660831985,0.333333333333333,
3.66661143271685));
#40783=CARTESIAN_POINT('Ctrl Pts',(-0.786422660831985,0.666666666666667,
3.66661143271685));
#40784=CARTESIAN_POINT('Ctrl Pts',(-0.786422660831985,1.,3.66661143271685));
#40785=CARTESIAN_POINT('',(-0.73204283740062,1.,4.13571194405636));
#40786=CARTESIAN_POINT('',(-0.73204283740062,0.,4.13571194405636));
#40787=CARTESIAN_POINT('Ctrl Pts',(-0.786422660831985,1.,3.66661143271685));
#40788=CARTESIAN_POINT('Ctrl Pts',(-0.786459983895432,1.,3.6666431041522));
#40789=CARTESIAN_POINT('Ctrl Pts',(-0.786565919558984,1.,3.66680946938292));
#40790=CARTESIAN_POINT('Ctrl Pts',(-0.786774337198062,1.,3.66743103898702));
#40791=CARTESIAN_POINT('Ctrl Pts',(-0.787145041181546,1.,3.66907505398677));
#40792=CARTESIAN_POINT('Ctrl Pts',(-0.787758799995743,1.,3.67252923663655));
#40793=CARTESIAN_POINT('Ctrl Pts',(-0.788569566220285,1.,3.67777119516252));
#40794=CARTESIAN_POINT('Ctrl Pts',(-0.789483546064387,1.,3.68428439783905));
#40795=CARTESIAN_POINT('Ctrl Pts',(-0.790436284988788,1.,3.69172044327364));
#40796=CARTESIAN_POINT('Ctrl Pts',(-0.79135657569598,1.,3.69968940808721));
#40797=CARTESIAN_POINT('Ctrl Pts',(-0.792177688845818,1.,3.70781724021806));
#40798=CARTESIAN_POINT('Ctrl Pts',(-0.792848377370287,1.,3.71580242396124));
#40799=CARTESIAN_POINT('Ctrl Pts',(-0.793347023784205,1.,3.72348797293734));
#40800=CARTESIAN_POINT('Ctrl Pts',(-0.793682750269684,1.,3.73086914695805));
#40801=CARTESIAN_POINT('Ctrl Pts',(-0.793882700937017,1.,3.73803280541687));
#40802=CARTESIAN_POINT('Ctrl Pts',(-0.793982700459952,1.,3.74511357728861));
#40803=CARTESIAN_POINT('Ctrl Pts',(-0.794017347371377,1.,3.75224692493864));
#40804=CARTESIAN_POINT('Ctrl Pts',(-0.794008429134907,1.,3.75951468666257));
#40805=CARTESIAN_POINT('Ctrl Pts',(-0.793961083688992,1.,3.76692626931111));
#40806=CARTESIAN_POINT('Ctrl Pts',(-0.793870523787408,1.,3.77444863801212));
#40807=CARTESIAN_POINT('Ctrl Pts',(-0.7937262357813,1.,3.78202460377598));
#40808=CARTESIAN_POINT('Ctrl Pts',(-0.793516871680993,1.,3.78959439439235));
#40809=CARTESIAN_POINT('Ctrl Pts',(-0.793235612973273,1.,3.79711921389897));
#40810=CARTESIAN_POINT('Ctrl Pts',(-0.792882695234778,1.,3.80459229925637));
#40811=CARTESIAN_POINT('Ctrl Pts',(-0.792462483517634,1.,3.81202588694756));
#40812=CARTESIAN_POINT('Ctrl Pts',(-0.791981740718635,1.,3.81944345442249));
#40813=CARTESIAN_POINT('Ctrl Pts',(-0.791447528662369,1.,3.82687033899792));
#40814=CARTESIAN_POINT('Ctrl Pts',(-0.790865012705301,1.,3.83432392054786));
#40815=CARTESIAN_POINT('Ctrl Pts',(-0.790236124191242,1.,3.84180762342454));
#40816=CARTESIAN_POINT('Ctrl Pts',(-0.789560798155582,1.,3.84931637808894));
#40817=CARTESIAN_POINT('Ctrl Pts',(-0.788837734090672,1.,3.85683995872529));
#40818=CARTESIAN_POINT('Ctrl Pts',(-0.788065315093778,1.,3.86436702561345));
#40819=CARTESIAN_POINT('Ctrl Pts',(-0.787242527617999,1.,3.87188916600912));
#40820=CARTESIAN_POINT('Ctrl Pts',(-0.786369675812609,1.,3.8794040281819));
#40821=CARTESIAN_POINT('Ctrl Pts',(-0.78544789034073,1.,3.88691313167398));
#40822=CARTESIAN_POINT('Ctrl Pts',(-0.784478799358336,1.,3.89442039235103));
#40823=CARTESIAN_POINT('Ctrl Pts',(-0.783464141529081,1.,3.9019303904397));
#40824=CARTESIAN_POINT('Ctrl Pts',(-0.782405395622764,1.,3.90944671004542));
#40825=CARTESIAN_POINT('Ctrl Pts',(-0.781303428618367,1.,3.91697036054676));
#40826=CARTESIAN_POINT('Ctrl Pts',(-0.780158678615543,1.,3.92450058323823));
#40827=CARTESIAN_POINT('Ctrl Pts',(-0.778971308134821,1.,3.93203552473174));
#40828=CARTESIAN_POINT('Ctrl Pts',(-0.777741370568559,1.,3.93957296768103));
#40829=CARTESIAN_POINT('Ctrl Pts',(-0.776468966697921,1.,3.94711101619447));
#40830=CARTESIAN_POINT('Ctrl Pts',(-0.775154418039352,1.,3.9546488545231));
#40831=CARTESIAN_POINT('Ctrl Pts',(-0.773798212026566,1.,3.96218649639807));
#40832=CARTESIAN_POINT('Ctrl Pts',(-0.772400931772136,1.,3.96972446532772));
#40833=CARTESIAN_POINT('Ctrl Pts',(-0.770963190030471,1.,3.97726349165488));
#40834=CARTESIAN_POINT('Ctrl Pts',(-0.769485566245544,1.,3.98480422348451));
#40835=CARTESIAN_POINT('Ctrl Pts',(-0.767968531377915,1.,3.9923468788101));
#40836=CARTESIAN_POINT('Ctrl Pts',(-0.766412457136064,1.,3.99989129179622));
#40837=CARTESIAN_POINT('Ctrl Pts',(-0.764817648785198,1.,4.00743706791509));
#40838=CARTESIAN_POINT('Ctrl Pts',(-0.763184371182935,1.,4.01498370680496));
#40839=CARTESIAN_POINT('Ctrl Pts',(-0.761512875859804,1.,4.02253072741268));
#40840=CARTESIAN_POINT('Ctrl Pts',(-0.759803433243752,1.,4.03007781954412));
#40841=CARTESIAN_POINT('Ctrl Pts',(-0.758056338884944,1.,4.03762485803119));
#40842=CARTESIAN_POINT('Ctrl Pts',(-0.756271902369581,1.,4.04517182653997));
#40843=CARTESIAN_POINT('Ctrl Pts',(-0.754450441816078,1.,4.05271876687915));
#40844=CARTESIAN_POINT('Ctrl Pts',(-0.752592276483072,1.,4.06026572221515));
#40845=CARTESIAN_POINT('Ctrl Pts',(-0.750697720484036,1.,4.06781267242378));
#40846=CARTESIAN_POINT('Ctrl Pts',(-0.748767076680557,1.,4.07535951056152));
#40847=CARTESIAN_POINT('Ctrl Pts',(-0.746800631492315,1.,4.08290608095642));
#40848=CARTESIAN_POINT('Ctrl Pts',(-0.7447986497065,1.,4.09045220253573));
#40849=CARTESIAN_POINT('Ctrl Pts',(-0.742761369689841,1.,4.09799769702611));
#40850=CARTESIAN_POINT('Ctrl Pts',(-0.740688998553377,1.,4.10554241757547));
#40851=CARTESIAN_POINT('Ctrl Pts',(-0.738581708225844,1.,4.11308626951927));
#40852=CARTESIAN_POINT('Ctrl Pts',(-0.736439634331345,1.,4.120629196238));
#40853=CARTESIAN_POINT('Ctrl Pts',(-0.734698226764092,1.,4.12666277570844));
#40854=CARTESIAN_POINT('Ctrl Pts',(-0.733376589323546,1.,4.13118752795207));
#40855=CARTESIAN_POINT('Ctrl Pts',(-0.73248857513516,1.,4.1342038373684));
#40856=CARTESIAN_POINT('Ctrl Pts',(-0.73204283740062,1.,4.13571194405636));
#40857=CARTESIAN_POINT('Origin',(-0.73204283740062,0.,4.13571194405636));
#40858=CARTESIAN_POINT('',(-0.581791163835815,1.,4.15950947128175));
#40859=CARTESIAN_POINT('Origin',(0.,0.,0.));
#40860=CARTESIAN_POINT('',(-0.963899035117249,1.,3.62400312501245));
#40861=CARTESIAN_POINT('Origin',(0.,1.,0.));
#40862=CARTESIAN_POINT('Ctrl Pts',(-0.963899035117249,1.,3.62400312501245));
#40863=CARTESIAN_POINT('Ctrl Pts',(-0.963899035117249,0.666666666666667,
3.62400312501245));
#40864=CARTESIAN_POINT('Ctrl Pts',(-0.963899035117249,0.333333333333333,
3.62400312501245));
#40865=CARTESIAN_POINT('Ctrl Pts',(-0.963899035117249,-0.333333333333333,
3.62400312501245));
#40866=CARTESIAN_POINT('Ctrl Pts',(-0.963899035117249,-0.666666666666667,
3.62400312501245));
#40867=CARTESIAN_POINT('Ctrl Pts',(-0.963899035117249,-1.,3.62400312501245));
#40868=CARTESIAN_POINT('Ctrl Pts',(-1.22531898815164,-1.,4.01728681790024));
#40869=CARTESIAN_POINT('Ctrl Pts',(-1.22531898815164,1.,4.01728681790024));
#40870=CARTESIAN_POINT('Ctrl Pts',(-1.22423716681447,-1.,4.0161454457032));
#40871=CARTESIAN_POINT('Ctrl Pts',(-1.22423716681447,1.,4.0161454457032));
#40872=CARTESIAN_POINT('Ctrl Pts',(-1.22207656456199,-1.,4.01386104434674));
#40873=CARTESIAN_POINT('Ctrl Pts',(-1.22207656456199,1.,4.01386104434674));
#40874=CARTESIAN_POINT('Ctrl Pts',(-1.21884478244983,-1.,4.01042947142681));
#40875=CARTESIAN_POINT('Ctrl Pts',(-1.21884478244983,1.,4.01042947142681));
#40876=CARTESIAN_POINT('Ctrl Pts',(-1.21455398918813,-1.,4.00584409524937));
#40877=CARTESIAN_POINT('Ctrl Pts',(-1.21455398918813,1.,4.00584409524937));
#40878=CARTESIAN_POINT('Ctrl Pts',(-1.20922097030107,-1.,4.00009577952534));
#40879=CARTESIAN_POINT('Ctrl Pts',(-1.20922097030107,1.,4.00009577952534));
#40880=CARTESIAN_POINT('Ctrl Pts',(-1.2039185237544,-1.,3.99433084800649));
#40881=CARTESIAN_POINT('Ctrl Pts',(-1.2039185237544,1.,3.99433084800649));
#40882=CARTESIAN_POINT('Ctrl Pts',(-1.19864679609596,-1.,3.98854928957287));
#40883=CARTESIAN_POINT('Ctrl Pts',(-1.19864679609596,1.,3.98854928957287));
#40884=CARTESIAN_POINT('Ctrl Pts',(-1.19340598349307,-1.,3.98275111052015));
#40885=CARTESIAN_POINT('Ctrl Pts',(-1.19340598349307,1.,3.98275111052015));
#40886=CARTESIAN_POINT('Ctrl Pts',(-1.18819633715285,-1.,3.97693634766926));
#40887=CARTESIAN_POINT('Ctrl Pts',(-1.18819633715285,1.,3.97693634766926));
#40888=CARTESIAN_POINT('Ctrl Pts',(-1.18301815039596,-1.,3.9711050516465));
#40889=CARTESIAN_POINT('Ctrl Pts',(-1.18301815039596,1.,3.9711050516465));
#40890=CARTESIAN_POINT('Ctrl Pts',(-1.17787174135445,-1.,3.96525726357682));
#40891=CARTESIAN_POINT('Ctrl Pts',(-1.17787174135445,1.,3.96525726357682));
#40892=CARTESIAN_POINT('Ctrl Pts',(-1.17275743590327,-1.,3.95939299213164));
#40893=CARTESIAN_POINT('Ctrl Pts',(-1.17275743590327,1.,3.95939299213164));
#40894=CARTESIAN_POINT('Ctrl Pts',(-1.16767555244495,-1.,3.95351219510062));
#40895=CARTESIAN_POINT('Ctrl Pts',(-1.16767555244495,1.,3.95351219510062));
#40896=CARTESIAN_POINT('Ctrl Pts',(-1.16262637999261,-1.,3.9476147478092));
#40897=CARTESIAN_POINT('Ctrl Pts',(-1.16262637999261,1.,3.9476147478092));
#40898=CARTESIAN_POINT('Ctrl Pts',(-1.1576101834106,-1.,3.94170046685542));
#40899=CARTESIAN_POINT('Ctrl Pts',(-1.1576101834106,1.,3.94170046685542));
#40900=CARTESIAN_POINT('Ctrl Pts',(-1.15262722716391,-1.,3.9357691705651));
#40901=CARTESIAN_POINT('Ctrl Pts',(-1.15262722716391,1.,3.9357691705651));
#40902=CARTESIAN_POINT('Ctrl Pts',(-1.14767779451147,-1.,3.92982073294334));
#40903=CARTESIAN_POINT('Ctrl Pts',(-1.14767779451147,1.,3.92982073294334));
#40904=CARTESIAN_POINT('Ctrl Pts',(-1.14276220561575,-1.,3.92385513133937));
#40905=CARTESIAN_POINT('Ctrl Pts',(-1.14276220561575,1.,3.92385513133937));
#40906=CARTESIAN_POINT('Ctrl Pts',(-1.13788084225511,-1.,3.91787251936688));
#40907=CARTESIAN_POINT('Ctrl Pts',(-1.13788084225511,1.,3.91787251936688));
#40908=CARTESIAN_POINT('Ctrl Pts',(-1.13303414693849,-1.,3.91187321145495));
#40909=CARTESIAN_POINT('Ctrl Pts',(-1.13303414693849,1.,3.91187321145495));
#40910=CARTESIAN_POINT('Ctrl Pts',(-1.12822258281518,-1.,3.90585753318622));
#40911=CARTESIAN_POINT('Ctrl Pts',(-1.12822258281518,1.,3.90585753318622));
#40912=CARTESIAN_POINT('Ctrl Pts',(-1.12344660099029,-1.,3.89982569749978));
#40913=CARTESIAN_POINT('Ctrl Pts',(-1.12344660099029,1.,3.89982569749978));
#40914=CARTESIAN_POINT('Ctrl Pts',(-1.11870660794609,-1.,3.89377768340362));
#40915=CARTESIAN_POINT('Ctrl Pts',(-1.11870660794609,1.,3.89377768340362));
#40916=CARTESIAN_POINT('Ctrl Pts',(-1.11400292434447,-1.,3.88771308285229));
#40917=CARTESIAN_POINT('Ctrl Pts',(-1.11400292434447,1.,3.88771308285229));
#40918=CARTESIAN_POINT('Ctrl Pts',(-1.10933577224029,-1.,3.88163105531791));
#40919=CARTESIAN_POINT('Ctrl Pts',(-1.10933577224029,1.,3.88163105531791));
#40920=CARTESIAN_POINT('Ctrl Pts',(-1.10470536603303,-1.,3.87553067187566));
#40921=CARTESIAN_POINT('Ctrl Pts',(-1.10470536603303,1.,3.87553067187566));
#40922=CARTESIAN_POINT('Ctrl Pts',(-1.10011198761202,-1.,3.86941120134872));
#40923=CARTESIAN_POINT('Ctrl Pts',(-1.10011198761202,1.,3.86941120134872));
#40924=CARTESIAN_POINT('Ctrl Pts',(-1.09555606505012,-1.,3.86327241021242));
#40925=CARTESIAN_POINT('Ctrl Pts',(-1.09555606505012,1.,3.86327241021242));
#40926=CARTESIAN_POINT('Ctrl Pts',(-1.09103825516288,-1.,3.85711487933911));
#40927=CARTESIAN_POINT('Ctrl Pts',(-1.09103825516288,1.,3.85711487933911));
#40928=CARTESIAN_POINT('Ctrl Pts',(-1.08655950846377,-1.,3.8509402522269));
#40929=CARTESIAN_POINT('Ctrl Pts',(-1.08655950846377,1.,3.8509402522269));
#40930=CARTESIAN_POINT('Ctrl Pts',(-1.08212087917986,-1.,3.84475048030615));
#40931=CARTESIAN_POINT('Ctrl Pts',(-1.08212087917986,1.,3.84475048030615));
#40932=CARTESIAN_POINT('Ctrl Pts',(-1.07772335353856,-1.,3.83854714117486));
#40933=CARTESIAN_POINT('Ctrl Pts',(-1.07772335353856,1.,3.83854714117486));
#40934=CARTESIAN_POINT('Ctrl Pts',(-1.0733676663346,-1.,3.83233071195145));
#40935=CARTESIAN_POINT('Ctrl Pts',(-1.0733676663346,1.,3.83233071195145));
#40936=CARTESIAN_POINT('Ctrl Pts',(-1.0690541318036,-1.,3.82609989967278));
#40937=CARTESIAN_POINT('Ctrl Pts',(-1.0690541318036,1.,3.82609989967278));
#40938=CARTESIAN_POINT('Ctrl Pts',(-1.06478244038931,-1.,3.81985083953012));
#40939=CARTESIAN_POINT('Ctrl Pts',(-1.06478244038931,1.,3.81985083953012));
#40940=CARTESIAN_POINT('Ctrl Pts',(-1.06055206187298,-1.,3.81357866117485));
#40941=CARTESIAN_POINT('Ctrl Pts',(-1.06055206187298,1.,3.81357866117485));
#40942=CARTESIAN_POINT('Ctrl Pts',(-1.05636266918643,-1.,3.80727913637784));
#40943=CARTESIAN_POINT('Ctrl Pts',(-1.05636266918643,1.,3.80727913637784));
#40944=CARTESIAN_POINT('Ctrl Pts',(-1.05221457990015,-1.,3.80095039790678));
#40945=CARTESIAN_POINT('Ctrl Pts',(-1.05221457990015,1.,3.80095039790678));
#40946=CARTESIAN_POINT('Ctrl Pts',(-1.04810913267641,-1.,3.79459440308793));
#40947=CARTESIAN_POINT('Ctrl Pts',(-1.04810913267641,1.,3.79459440308793));
#40948=CARTESIAN_POINT('Ctrl Pts',(-1.04404924374426,-1.,3.78821910787195));
#40949=CARTESIAN_POINT('Ctrl Pts',(-1.04404924374426,1.,3.78821910787195));
#40950=CARTESIAN_POINT('Ctrl Pts',(-1.04003862055804,-1.,3.78183535008192));
#40951=CARTESIAN_POINT('Ctrl Pts',(-1.04003862055804,1.,3.78183535008192));
#40952=CARTESIAN_POINT('Ctrl Pts',(-1.03608074678013,-1.,3.77545283140445));
#40953=CARTESIAN_POINT('Ctrl Pts',(-1.03608074678013,1.,3.77545283140445));
#40954=CARTESIAN_POINT('Ctrl Pts',(-1.0321778660492,-1.,3.76907609832522));
#40955=CARTESIAN_POINT('Ctrl Pts',(-1.0321778660492,1.,3.76907609832522));
#40956=CARTESIAN_POINT('Ctrl Pts',(-1.02833014458181,-1.,3.76270122291232));
#40957=CARTESIAN_POINT('Ctrl Pts',(-1.02833014458181,1.,3.76270122291232));
#40958=CARTESIAN_POINT('Ctrl Pts',(-1.0245342944466,-1.,3.75631037456194));
#40959=CARTESIAN_POINT('Ctrl Pts',(-1.0245342944466,1.,3.75631037456194));
#40960=CARTESIAN_POINT('Ctrl Pts',(-1.02078510487428,-1.,3.74987777155834));
#40961=CARTESIAN_POINT('Ctrl Pts',(-1.02078510487428,1.,3.74987777155834));
#40962=CARTESIAN_POINT('Ctrl Pts',(-1.01707794311079,-1.,3.74337942504959));
#40963=CARTESIAN_POINT('Ctrl Pts',(-1.01707794311079,1.,3.74337942504959));
#40964=CARTESIAN_POINT('Ctrl Pts',(-1.01341114319903,-1.,3.73680245055734));
#40965=CARTESIAN_POINT('Ctrl Pts',(-1.01341114319903,1.,3.73680245055734));
#40966=CARTESIAN_POINT('Ctrl Pts',(-1.00978798539496,-1.,3.73015276704426));
#40967=CARTESIAN_POINT('Ctrl Pts',(-1.00978798539496,1.,3.73015276704426));
#40968=CARTESIAN_POINT('Ctrl Pts',(-1.0062200073571,-1.,3.72346803750595));
#40969=CARTESIAN_POINT('Ctrl Pts',(-1.0062200073571,1.,3.72346803750595));
#40970=CARTESIAN_POINT('Ctrl Pts',(-1.00272423396822,-1.,3.71680667125118));
#40971=CARTESIAN_POINT('Ctrl Pts',(-1.00272423396822,1.,3.71680667125118));
#40972=CARTESIAN_POINT('Ctrl Pts',(-0.999317260756531,-1.,3.71022439713938));
#40973=CARTESIAN_POINT('Ctrl Pts',(-0.999317260756531,1.,3.71022439713938));
#40974=CARTESIAN_POINT('Ctrl Pts',(-0.996009819772518,-1.,3.70375282282138));
#40975=CARTESIAN_POINT('Ctrl Pts',(-0.996009819772518,1.,3.70375282282138));
#40976=CARTESIAN_POINT('Ctrl Pts',(-0.99280221833201,-1.,3.69738123415662));
#40977=CARTESIAN_POINT('Ctrl Pts',(-0.99280221833201,1.,3.69738123415662));
#40978=CARTESIAN_POINT('Ctrl Pts',(-0.989676715398558,-1.,3.69102682138846));
#40979=CARTESIAN_POINT('Ctrl Pts',(-0.989676715398558,1.,3.69102682138846));
#40980=CARTESIAN_POINT('Ctrl Pts',(-0.986602639863838,-1.,3.68455317926068));
#40981=CARTESIAN_POINT('Ctrl Pts',(-0.986602639863838,1.,3.68455317926068));
#40982=CARTESIAN_POINT('Ctrl Pts',(-0.983550791470419,-1.,3.67782408841715));
#40983=CARTESIAN_POINT('Ctrl Pts',(-0.983550791470419,1.,3.67782408841715));
#40984=CARTESIAN_POINT('Ctrl Pts',(-0.980505922458267,-1.,3.67074983340361));
#40985=CARTESIAN_POINT('Ctrl Pts',(-0.980505922458267,1.,3.67074983340361));
#40986=CARTESIAN_POINT('Ctrl Pts',(-0.977478312751618,-1.,3.66333049637475));
#40987=CARTESIAN_POINT('Ctrl Pts',(-0.977478312751618,1.,3.66333049637475));
#40988=CARTESIAN_POINT('Ctrl Pts',(-0.974519971354848,-1.,3.65571576735126));
#40989=CARTESIAN_POINT('Ctrl Pts',(-0.974519971354848,1.,3.65571576735126));
#40990=CARTESIAN_POINT('Ctrl Pts',(-0.971722122061341,-1.,3.64819756447455));
#40991=CARTESIAN_POINT('Ctrl Pts',(-0.971722122061341,1.,3.64819756447455));
#40992=CARTESIAN_POINT('Ctrl Pts',(-0.969195124675866,-1.,3.64113946505766));
#40993=CARTESIAN_POINT('Ctrl Pts',(-0.969195124675866,1.,3.64113946505766));
#40994=CARTESIAN_POINT('Ctrl Pts',(-0.967052554541386,-1.,3.63492122081143));
#40995=CARTESIAN_POINT('Ctrl Pts',(-0.967052554541386,1.,3.63492122081143));
#40996=CARTESIAN_POINT('Ctrl Pts',(-0.965395153165293,-1.,3.62988252139846));
#40997=CARTESIAN_POINT('Ctrl Pts',(-0.965395153165293,1.,3.62988252139846));
#40998=CARTESIAN_POINT('Ctrl Pts',(-0.964291001273288,-1.,3.62625391254797));
#40999=CARTESIAN_POINT('Ctrl Pts',(-0.964291001273288,1.,3.62625391254797));
#41000=CARTESIAN_POINT('Ctrl Pts',(-0.963875774530619,-1.,3.6245656860652));
#41001=CARTESIAN_POINT('Ctrl Pts',(-0.963875774530619,1.,3.6245656860652));
#41002=CARTESIAN_POINT('Ctrl Pts',(-0.963832486395051,-1.,3.62399933639914));
#41003=CARTESIAN_POINT('Ctrl Pts',(-0.963832486395051,1.,3.62399933639914));
#41004=CARTESIAN_POINT('Ctrl Pts',(-0.963922720982193,-1.,3.62393257642052));
#41005=CARTESIAN_POINT('Ctrl Pts',(-0.963922720982193,1.,3.62393257642052));
#41006=CARTESIAN_POINT('Ctrl Pts',(-0.963997613369571,-1.,3.62397690409552));
#41007=CARTESIAN_POINT('Ctrl Pts',(-0.963997613369571,1.,3.62397690409552));
#41008=CARTESIAN_POINT('',(-1.22531898815164,1.,4.01728681790024));
#41009=CARTESIAN_POINT('Ctrl Pts',(-1.22531898815164,1.,4.01728681790024));
#41010=CARTESIAN_POINT('Ctrl Pts',(-1.22423716681447,1.,4.0161454457032));
#41011=CARTESIAN_POINT('Ctrl Pts',(-1.22207656456199,1.,4.01386104434674));
#41012=CARTESIAN_POINT('Ctrl Pts',(-1.21884478244983,1.,4.01042947142681));
#41013=CARTESIAN_POINT('Ctrl Pts',(-1.21455398918813,1.,4.00584409524937));
#41014=CARTESIAN_POINT('Ctrl Pts',(-1.20922097030107,1.,4.00009577952534));
#41015=CARTESIAN_POINT('Ctrl Pts',(-1.2039185237544,1.,3.99433084800649));
#41016=CARTESIAN_POINT('Ctrl Pts',(-1.19864679609596,1.,3.98854928957287));
#41017=CARTESIAN_POINT('Ctrl Pts',(-1.19340598349307,1.,3.98275111052015));
#41018=CARTESIAN_POINT('Ctrl Pts',(-1.18819633715285,1.,3.97693634766926));
#41019=CARTESIAN_POINT('Ctrl Pts',(-1.18301815039596,1.,3.9711050516465));
#41020=CARTESIAN_POINT('Ctrl Pts',(-1.17787174135445,1.,3.96525726357682));
#41021=CARTESIAN_POINT('Ctrl Pts',(-1.17275743590327,1.,3.95939299213164));
#41022=CARTESIAN_POINT('Ctrl Pts',(-1.16767555244495,1.,3.95351219510062));
#41023=CARTESIAN_POINT('Ctrl Pts',(-1.16262637999261,1.,3.9476147478092));
#41024=CARTESIAN_POINT('Ctrl Pts',(-1.1576101834106,1.,3.94170046685542));
#41025=CARTESIAN_POINT('Ctrl Pts',(-1.15262722716391,1.,3.9357691705651));
#41026=CARTESIAN_POINT('Ctrl Pts',(-1.14767779451147,1.,3.92982073294334));
#41027=CARTESIAN_POINT('Ctrl Pts',(-1.14276220561575,1.,3.92385513133937));
#41028=CARTESIAN_POINT('Ctrl Pts',(-1.13788084225511,1.,3.91787251936688));
#41029=CARTESIAN_POINT('Ctrl Pts',(-1.13303414693849,1.,3.91187321145495));
#41030=CARTESIAN_POINT('Ctrl Pts',(-1.12822258281518,1.,3.90585753318622));
#41031=CARTESIAN_POINT('Ctrl Pts',(-1.12344660099029,1.,3.89982569749978));
#41032=CARTESIAN_POINT('Ctrl Pts',(-1.11870660794609,1.,3.89377768340362));
#41033=CARTESIAN_POINT('Ctrl Pts',(-1.11400292434447,1.,3.88771308285229));
#41034=CARTESIAN_POINT('Ctrl Pts',(-1.10933577224029,1.,3.88163105531791));
#41035=CARTESIAN_POINT('Ctrl Pts',(-1.10470536603303,1.,3.87553067187566));
#41036=CARTESIAN_POINT('Ctrl Pts',(-1.10011198761202,1.,3.86941120134872));
#41037=CARTESIAN_POINT('Ctrl Pts',(-1.09555606505012,1.,3.86327241021242));
#41038=CARTESIAN_POINT('Ctrl Pts',(-1.09103825516288,1.,3.85711487933911));
#41039=CARTESIAN_POINT('Ctrl Pts',(-1.08655950846377,1.,3.8509402522269));
#41040=CARTESIAN_POINT('Ctrl Pts',(-1.08212087917986,1.,3.84475048030615));
#41041=CARTESIAN_POINT('Ctrl Pts',(-1.07772335353856,1.,3.83854714117486));
#41042=CARTESIAN_POINT('Ctrl Pts',(-1.0733676663346,1.,3.83233071195145));
#41043=CARTESIAN_POINT('Ctrl Pts',(-1.0690541318036,1.,3.82609989967278));
#41044=CARTESIAN_POINT('Ctrl Pts',(-1.06478244038931,1.,3.81985083953012));
#41045=CARTESIAN_POINT('Ctrl Pts',(-1.06055206187298,1.,3.81357866117485));
#41046=CARTESIAN_POINT('Ctrl Pts',(-1.05636266918643,1.,3.80727913637784));
#41047=CARTESIAN_POINT('Ctrl Pts',(-1.05221457990015,1.,3.80095039790678));
#41048=CARTESIAN_POINT('Ctrl Pts',(-1.04810913267641,1.,3.79459440308793));
#41049=CARTESIAN_POINT('Ctrl Pts',(-1.04404924374426,1.,3.78821910787195));
#41050=CARTESIAN_POINT('Ctrl Pts',(-1.04003862055804,1.,3.78183535008192));
#41051=CARTESIAN_POINT('Ctrl Pts',(-1.03608074678013,1.,3.77545283140445));
#41052=CARTESIAN_POINT('Ctrl Pts',(-1.0321778660492,1.,3.76907609832522));
#41053=CARTESIAN_POINT('Ctrl Pts',(-1.02833014458181,1.,3.76270122291232));
#41054=CARTESIAN_POINT('Ctrl Pts',(-1.0245342944466,1.,3.75631037456194));
#41055=CARTESIAN_POINT('Ctrl Pts',(-1.02078510487428,1.,3.74987777155834));
#41056=CARTESIAN_POINT('Ctrl Pts',(-1.01707794311079,1.,3.74337942504959));
#41057=CARTESIAN_POINT('Ctrl Pts',(-1.01341114319903,1.,3.73680245055734));
#41058=CARTESIAN_POINT('Ctrl Pts',(-1.00978798539496,1.,3.73015276704426));
#41059=CARTESIAN_POINT('Ctrl Pts',(-1.0062200073571,1.,3.72346803750595));
#41060=CARTESIAN_POINT('Ctrl Pts',(-1.00272423396822,1.,3.71680667125118));
#41061=CARTESIAN_POINT('Ctrl Pts',(-0.999317260756531,1.,3.71022439713938));
#41062=CARTESIAN_POINT('Ctrl Pts',(-0.996009819772518,1.,3.70375282282138));
#41063=CARTESIAN_POINT('Ctrl Pts',(-0.99280221833201,1.,3.69738123415662));
#41064=CARTESIAN_POINT('Ctrl Pts',(-0.989676715398558,1.,3.69102682138846));
#41065=CARTESIAN_POINT('Ctrl Pts',(-0.986602639863838,1.,3.68455317926068));
#41066=CARTESIAN_POINT('Ctrl Pts',(-0.983550791470419,1.,3.67782408841715));
#41067=CARTESIAN_POINT('Ctrl Pts',(-0.980505922458267,1.,3.67074983340361));
#41068=CARTESIAN_POINT('Ctrl Pts',(-0.977478312751618,1.,3.66333049637475));
#41069=CARTESIAN_POINT('Ctrl Pts',(-0.974519971354848,1.,3.65571576735126));
#41070=CARTESIAN_POINT('Ctrl Pts',(-0.971722122061341,1.,3.64819756447455));
#41071=CARTESIAN_POINT('Ctrl Pts',(-0.969195124675866,1.,3.64113946505766));
#41072=CARTESIAN_POINT('Ctrl Pts',(-0.967052554541386,1.,3.63492122081143));
#41073=CARTESIAN_POINT('Ctrl Pts',(-0.965395153165293,1.,3.62988252139846));
#41074=CARTESIAN_POINT('Ctrl Pts',(-0.964373850166457,1.,3.62652618145335));
#41075=CARTESIAN_POINT('Ctrl Pts',(-0.963957782642843,1.,3.62489305727662));
#41076=CARTESIAN_POINT('Ctrl Pts',(-0.963861297423241,1.,3.62424461507588));
#41077=CARTESIAN_POINT('Ctrl Pts',(-0.963880158555582,1.,3.6240482887845));
#41078=CARTESIAN_POINT('Ctrl Pts',(-0.963899035117249,1.,3.62400312501245));
#41079=CARTESIAN_POINT('',(-1.22531898815164,0.,4.01728681790024));
#41080=CARTESIAN_POINT('Ctrl Pts',(-1.35022972712301,-1.,3.49848248301936));
#41081=CARTESIAN_POINT('Ctrl Pts',(-1.35022972712301,1.,3.49848248301936));
#41082=CARTESIAN_POINT('Ctrl Pts',(-1.35026426118402,-1.,3.4984026005375));
#41083=CARTESIAN_POINT('Ctrl Pts',(-1.35026426118402,1.,3.4984026005375));
#41084=CARTESIAN_POINT('Ctrl Pts',(-1.35037650303019,-1.,3.49840357193736));
#41085=CARTESIAN_POINT('Ctrl Pts',(-1.35037650303019,1.,3.49840357193736));
#41086=CARTESIAN_POINT('Ctrl Pts',(-1.35067437417483,-1.,3.49888720257132));
#41087=CARTESIAN_POINT('Ctrl Pts',(-1.35067437417483,1.,3.49888720257132));
#41088=CARTESIAN_POINT('Ctrl Pts',(-1.3513307633124,-1.,3.5004970706414));
#41089=CARTESIAN_POINT('Ctrl Pts',(-1.3513307633124,1.,3.5004970706414));
#41090=CARTESIAN_POINT('Ctrl Pts',(-1.35257032843486,-1.,3.50408168106261));
#41091=CARTESIAN_POINT('Ctrl Pts',(-1.35257032843486,1.,3.50408168106261));
#41092=CARTESIAN_POINT('Ctrl Pts',(-1.35419113575956,-1.,3.50913227059999));
#41093=CARTESIAN_POINT('Ctrl Pts',(-1.35419113575956,1.,3.50913227059999));
#41094=CARTESIAN_POINT('Ctrl Pts',(-1.35611275237152,-1.,3.51542230699556));
#41095=CARTESIAN_POINT('Ctrl Pts',(-1.35611275237152,1.,3.51542230699556));
#41096=CARTESIAN_POINT('Ctrl Pts',(-1.35821701528836,-1.,3.52261776116748));
#41097=CARTESIAN_POINT('Ctrl Pts',(-1.35821701528836,1.,3.52261776116748));
#41098=CARTESIAN_POINT('Ctrl Pts',(-1.36037259643734,-1.,3.530344649616));
#41099=CARTESIAN_POINT('Ctrl Pts',(-1.36037259643734,1.,3.530344649616));
#41100=CARTESIAN_POINT('Ctrl Pts',(-1.36245507339307,-1.,3.53824396424961));
#41101=CARTESIAN_POINT('Ctrl Pts',(-1.36245507339307,1.,3.53824396424961));
#41102=CARTESIAN_POINT('Ctrl Pts',(-1.36436666257598,-1.,3.54602591832973));
#41103=CARTESIAN_POINT('Ctrl Pts',(-1.36436666257598,1.,3.54602591832973));
#41104=CARTESIAN_POINT('Ctrl Pts',(-1.3660614545677,-1.,3.55353883995949));
#41105=CARTESIAN_POINT('Ctrl Pts',(-1.3660614545677,1.,3.55353883995949));
#41106=CARTESIAN_POINT('Ctrl Pts',(-1.36754771771233,-1.,3.56077662028649));
#41107=CARTESIAN_POINT('Ctrl Pts',(-1.36754771771233,1.,3.56077662028649));
#41108=CARTESIAN_POINT('Ctrl Pts',(-1.36886584973389,-1.,3.5678208030466));
#41109=CARTESIAN_POINT('Ctrl Pts',(-1.36886584973389,1.,3.5678208030466));
#41110=CARTESIAN_POINT('Ctrl Pts',(-1.37007229485659,-1.,3.57479875549486));
#41111=CARTESIAN_POINT('Ctrl Pts',(-1.37007229485659,1.,3.57479875549486));
#41112=CARTESIAN_POINT('Ctrl Pts',(-1.37122241663062,-1.,3.58183885982715));
#41113=CARTESIAN_POINT('Ctrl Pts',(-1.37122241663062,1.,3.58183885982715));
#41114=CARTESIAN_POINT('Ctrl Pts',(-1.37235053660976,-1.,3.58901853846365));
#41115=CARTESIAN_POINT('Ctrl Pts',(-1.37235053660976,1.,3.58901853846365));
#41116=CARTESIAN_POINT('Ctrl Pts',(-1.37346320103157,-1.,3.59634627869048));
#41117=CARTESIAN_POINT('Ctrl Pts',(-1.37346320103157,1.,3.59634627869048));
#41118=CARTESIAN_POINT('Ctrl Pts',(-1.37455051379623,-1.,3.60379020123988));
#41119=CARTESIAN_POINT('Ctrl Pts',(-1.37455051379623,1.,3.60379020123988));
#41120=CARTESIAN_POINT('Ctrl Pts',(-1.37559314436634,-1.,3.61129546591064));
#41121=CARTESIAN_POINT('Ctrl Pts',(-1.37559314436634,1.,3.61129546591064));
#41122=CARTESIAN_POINT('Ctrl Pts',(-1.37657053403107,-1.,3.6188048116042));
#41123=CARTESIAN_POINT('Ctrl Pts',(-1.37657053403107,1.,3.6188048116042));
#41124=CARTESIAN_POINT('Ctrl Pts',(-1.37746987919881,-1.,3.62628098665145));
#41125=CARTESIAN_POINT('Ctrl Pts',(-1.37746987919881,1.,3.62628098665145));
#41126=CARTESIAN_POINT('Ctrl Pts',(-1.37829035457339,-1.,3.63371727442486));
#41127=CARTESIAN_POINT('Ctrl Pts',(-1.37829035457339,1.,3.63371727442486));
#41128=CARTESIAN_POINT('Ctrl Pts',(-1.37903818567359,-1.,3.64112507791141));
#41129=CARTESIAN_POINT('Ctrl Pts',(-1.37903818567359,1.,3.64112507791141));
#41130=CARTESIAN_POINT('Ctrl Pts',(-1.37972372481603,-1.,3.64852652756456));
#41131=CARTESIAN_POINT('Ctrl Pts',(-1.37972372481603,1.,3.64852652756456));
#41132=CARTESIAN_POINT('Ctrl Pts',(-1.38035791051213,-1.,3.6559455440439));
#41133=CARTESIAN_POINT('Ctrl Pts',(-1.38035791051213,1.,3.6559455440439));
#41134=CARTESIAN_POINT('Ctrl Pts',(-1.38094856333552,-1.,3.66339848520857));
#41135=CARTESIAN_POINT('Ctrl Pts',(-1.38094856333552,1.,3.66339848520857));
#41136=CARTESIAN_POINT('Ctrl Pts',(-1.38149812653868,-1.,3.67088843112262));
#41137=CARTESIAN_POINT('Ctrl Pts',(-1.38149812653868,1.,3.67088843112262));
#41138=CARTESIAN_POINT('Ctrl Pts',(-1.3820057429062,-1.,3.67841038482414));
#41139=CARTESIAN_POINT('Ctrl Pts',(-1.3820057429062,1.,3.67841038482414));
#41140=CARTESIAN_POINT('Ctrl Pts',(-1.38246852827182,-1.,3.68595444983837));
#41141=CARTESIAN_POINT('Ctrl Pts',(-1.38246852827182,1.,3.68595444983837));
#41142=CARTESIAN_POINT('Ctrl Pts',(-1.38288311171651,-1.,3.69350967899526));
#41143=CARTESIAN_POINT('Ctrl Pts',(-1.38288311171651,1.,3.69350967899526));
#41144=CARTESIAN_POINT('Ctrl Pts',(-1.38324717612865,-1.,3.701067921679));
#41145=CARTESIAN_POINT('Ctrl Pts',(-1.38324717612865,1.,3.701067921679));
#41146=CARTESIAN_POINT('Ctrl Pts',(-1.38356065402124,-1.,3.70862680753347));
#41147=CARTESIAN_POINT('Ctrl Pts',(-1.38356065402124,1.,3.70862680753347));
#41148=CARTESIAN_POINT('Ctrl Pts',(-1.38382489984586,-1.,3.7161876605181));
#41149=CARTESIAN_POINT('Ctrl Pts',(-1.38382489984586,1.,3.7161876605181));
#41150=CARTESIAN_POINT('Ctrl Pts',(-1.3840421342895,-1.,3.72375409358803));
#41151=CARTESIAN_POINT('Ctrl Pts',(-1.3840421342895,1.,3.72375409358803));
#41152=CARTESIAN_POINT('Ctrl Pts',(-1.38421479111531,-1.,3.73133035859282));
#41153=CARTESIAN_POINT('Ctrl Pts',(-1.38421479111531,1.,3.73133035859282));
#41154=CARTESIAN_POINT('Ctrl Pts',(-1.38434489156458,-1.,3.73891976418104));
#41155=CARTESIAN_POINT('Ctrl Pts',(-1.38434489156458,1.,3.73891976418104));
#41156=CARTESIAN_POINT('Ctrl Pts',(-1.38443344984394,-1.,3.74652317167876));
#41157=CARTESIAN_POINT('Ctrl Pts',(-1.38443344984394,1.,3.74652317167876));
#41158=CARTESIAN_POINT('Ctrl Pts',(-1.38448077997163,-1.,3.7541397631875));
#41159=CARTESIAN_POINT('Ctrl Pts',(-1.38448077997163,1.,3.7541397631875));
#41160=CARTESIAN_POINT('Ctrl Pts',(-1.3844867525335,-1.,3.76176768271367));
#41161=CARTESIAN_POINT('Ctrl Pts',(-1.3844867525335,1.,3.76176768271367));
#41162=CARTESIAN_POINT('Ctrl Pts',(-1.38445107339518,-1.,3.76940473185779));
#41163=CARTESIAN_POINT('Ctrl Pts',(-1.38445107339518,1.,3.76940473185779));
#41164=CARTESIAN_POINT('Ctrl Pts',(-1.38437354551428,-1.,3.77704902230418));
#41165=CARTESIAN_POINT('Ctrl Pts',(-1.38437354551428,1.,3.77704902230418));
#41166=CARTESIAN_POINT('Ctrl Pts',(-1.38425435883756,-1.,3.78469969805082));
#41167=CARTESIAN_POINT('Ctrl Pts',(-1.38425435883756,1.,3.78469969805082));
#41168=CARTESIAN_POINT('Ctrl Pts',(-1.38409399694566,-1.,3.79235669640841));
#41169=CARTESIAN_POINT('Ctrl Pts',(-1.38409399694566,1.,3.79235669640841));
#41170=CARTESIAN_POINT('Ctrl Pts',(-1.38389311766682,-1.,3.80002044322111));
#41171=CARTESIAN_POINT('Ctrl Pts',(-1.38389311766682,1.,3.80002044322111));
#41172=CARTESIAN_POINT('Ctrl Pts',(-1.3836524404622,-1.,3.80769156398411));
#41173=CARTESIAN_POINT('Ctrl Pts',(-1.3836524404622,1.,3.80769156398411));
#41174=CARTESIAN_POINT('Ctrl Pts',(-1.38337263902782,-1.,3.81537060817811));
#41175=CARTESIAN_POINT('Ctrl Pts',(-1.38337263902782,1.,3.81537060817811));
#41176=CARTESIAN_POINT('Ctrl Pts',(-1.38305421262763,-1.,3.82305771743829));
#41177=CARTESIAN_POINT('Ctrl Pts',(-1.38305421262763,1.,3.82305771743829));
#41178=CARTESIAN_POINT('Ctrl Pts',(-1.38269750245138,-1.,3.8307526698229));
#41179=CARTESIAN_POINT('Ctrl Pts',(-1.38269750245138,1.,3.8307526698229));
#41180=CARTESIAN_POINT('Ctrl Pts',(-1.38230274828822,-1.,3.83845502790746));
#41181=CARTESIAN_POINT('Ctrl Pts',(-1.38230274828822,1.,3.83845502790746));
#41182=CARTESIAN_POINT('Ctrl Pts',(-1.38187013346109,-1.,3.84616425605764));
#41183=CARTESIAN_POINT('Ctrl Pts',(-1.38187013346109,1.,3.84616425605764));
#41184=CARTESIAN_POINT('Ctrl Pts',(-1.38139983115049,-1.,3.85387983979481));
#41185=CARTESIAN_POINT('Ctrl Pts',(-1.38139983115049,1.,3.85387983979481));
#41186=CARTESIAN_POINT('Ctrl Pts',(-1.38089205992989,-1.,3.86160143043959));
#41187=CARTESIAN_POINT('Ctrl Pts',(-1.38089205992989,1.,3.86160143043959));
#41188=CARTESIAN_POINT('Ctrl Pts',(-1.38034709213014,-1.,3.86932885813068));
#41189=CARTESIAN_POINT('Ctrl Pts',(-1.38034709213014,1.,3.86932885813068));
#41190=CARTESIAN_POINT('Ctrl Pts',(-1.37976523097073,-1.,3.87706205830532));
#41191=CARTESIAN_POINT('Ctrl Pts',(-1.37976523097073,1.,3.87706205830532));
#41192=CARTESIAN_POINT('Ctrl Pts',(-1.37914679719383,-1.,3.88480102249277));
#41193=CARTESIAN_POINT('Ctrl Pts',(-1.37914679719383,1.,3.88480102249277));
#41194=CARTESIAN_POINT('Ctrl Pts',(-1.3784921128802,-1.,3.89254574338496));
#41195=CARTESIAN_POINT('Ctrl Pts',(-1.3784921128802,1.,3.89254574338496));
#41196=CARTESIAN_POINT('Ctrl Pts',(-1.37780148512792,-1.,3.90029615196727));
#41197=CARTESIAN_POINT('Ctrl Pts',(-1.37780148512792,1.,3.90029615196727));
#41198=CARTESIAN_POINT('Ctrl Pts',(-1.3770751963402,-1.,3.90805209523486));
#41199=CARTESIAN_POINT('Ctrl Pts',(-1.3770751963402,1.,3.90805209523486));
#41200=CARTESIAN_POINT('Ctrl Pts',(-1.37631350505797,-1.,3.91581337462644));
#41201=CARTESIAN_POINT('Ctrl Pts',(-1.37631350505797,1.,3.91581337462644));
#41202=CARTESIAN_POINT('Ctrl Pts',(-1.37551664448242,-1.,3.92357976987672));
#41203=CARTESIAN_POINT('Ctrl Pts',(-1.37551664448242,1.,3.92357976987672));
#41204=CARTESIAN_POINT('Ctrl Pts',(-1.37468482215751,-1.,3.93135106761844));
#41205=CARTESIAN_POINT('Ctrl Pts',(-1.37468482215751,1.,3.93135106761844));
#41206=CARTESIAN_POINT('Ctrl Pts',(-1.37381821967165,-1.,3.93912709040818));
#41207=CARTESIAN_POINT('Ctrl Pts',(-1.37381821967165,1.,3.93912709040818));
#41208=CARTESIAN_POINT('Ctrl Pts',(-1.37291699202807,-1.,3.94690771785133));
#41209=CARTESIAN_POINT('Ctrl Pts',(-1.37291699202807,1.,3.94690771785133));
#41210=CARTESIAN_POINT('Ctrl Pts',(-1.37198126432386,-1.,3.95469287280914));
#41211=CARTESIAN_POINT('Ctrl Pts',(-1.37198126432386,1.,3.95469287280914));
#41212=CARTESIAN_POINT('Ctrl Pts',(-1.3712051561502,-1.,3.96092458506535));
#41213=CARTESIAN_POINT('Ctrl Pts',(-1.3712051561502,1.,3.96092458506535));
#41214=CARTESIAN_POINT('Ctrl Pts',(-1.37060761745635,-1.,3.96560037974645));
#41215=CARTESIAN_POINT('Ctrl Pts',(-1.37060761745635,1.,3.96560037974645));
#41216=CARTESIAN_POINT('Ctrl Pts',(-1.37020239094614,-1.,3.9687184694131));
#41217=CARTESIAN_POINT('Ctrl Pts',(-1.37020239094614,1.,3.9687184694131));
#41218=CARTESIAN_POINT('Ctrl Pts',(-1.36999806084572,-1.,3.97027773754922));
#41219=CARTESIAN_POINT('Ctrl Pts',(-1.36999806084572,1.,3.97027773754922));
#41220=CARTESIAN_POINT('',(-1.35032489087101,1.,3.4984457533445));
#41221=CARTESIAN_POINT('Ctrl Pts',(-1.35032489087101,-1.,3.4984457533445));
#41222=CARTESIAN_POINT('Ctrl Pts',(-1.35032489087101,-0.666666666666667,
3.4984457533445));
#41223=CARTESIAN_POINT('Ctrl Pts',(-1.35032489087101,-0.333333333333333,
3.4984457533445));
#41224=CARTESIAN_POINT('Ctrl Pts',(-1.35032489087101,0.333333333333333,
3.4984457533445));
#41225=CARTESIAN_POINT('Ctrl Pts',(-1.35032489087101,0.666666666666667,
3.4984457533445));
#41226=CARTESIAN_POINT('Ctrl Pts',(-1.35032489087101,1.,3.4984457533445));
#41227=CARTESIAN_POINT('',(-1.36999806084572,1.,3.97027773754922));
#41228=CARTESIAN_POINT('',(-1.36999806084572,0.,3.97027773754922));
#41229=CARTESIAN_POINT('Ctrl Pts',(-1.35032489087101,1.,3.4984457533445));
#41230=CARTESIAN_POINT('Ctrl Pts',(-1.35036670892966,1.,3.49847119623846));
#41231=CARTESIAN_POINT('Ctrl Pts',(-1.35049736560527,1.,3.49861894124827));
#41232=CARTESIAN_POINT('Ctrl Pts',(-1.35080045218587,1.,3.49920025459723));
#41233=CARTESIAN_POINT('Ctrl Pts',(-1.35142377279517,1.,3.5007660381649));
#41234=CARTESIAN_POINT('Ctrl Pts',(-1.35257032843486,1.,3.50408168106261));
#41235=CARTESIAN_POINT('Ctrl Pts',(-1.35419113575956,1.,3.50913227059999));
#41236=CARTESIAN_POINT('Ctrl Pts',(-1.35611275237152,1.,3.51542230699556));
#41237=CARTESIAN_POINT('Ctrl Pts',(-1.35821701528836,1.,3.52261776116748));
#41238=CARTESIAN_POINT('Ctrl Pts',(-1.36037259643734,1.,3.530344649616));
#41239=CARTESIAN_POINT('Ctrl Pts',(-1.36245507339307,1.,3.53824396424961));
#41240=CARTESIAN_POINT('Ctrl Pts',(-1.36436666257598,1.,3.54602591832973));
#41241=CARTESIAN_POINT('Ctrl Pts',(-1.3660614545677,1.,3.55353883995949));
#41242=CARTESIAN_POINT('Ctrl Pts',(-1.36754771771233,1.,3.56077662028649));
#41243=CARTESIAN_POINT('Ctrl Pts',(-1.36886584973389,1.,3.5678208030466));
#41244=CARTESIAN_POINT('Ctrl Pts',(-1.37007229485659,1.,3.57479875549486));
#41245=CARTESIAN_POINT('Ctrl Pts',(-1.37122241663062,1.,3.58183885982715));
#41246=CARTESIAN_POINT('Ctrl Pts',(-1.37235053660976,1.,3.58901853846365));
#41247=CARTESIAN_POINT('Ctrl Pts',(-1.37346320103157,1.,3.59634627869048));
#41248=CARTESIAN_POINT('Ctrl Pts',(-1.37455051379623,1.,3.60379020123988));
#41249=CARTESIAN_POINT('Ctrl Pts',(-1.37559314436634,1.,3.61129546591064));
#41250=CARTESIAN_POINT('Ctrl Pts',(-1.37657053403107,1.,3.6188048116042));
#41251=CARTESIAN_POINT('Ctrl Pts',(-1.37746987919881,1.,3.62628098665145));
#41252=CARTESIAN_POINT('Ctrl Pts',(-1.37829035457339,1.,3.63371727442486));
#41253=CARTESIAN_POINT('Ctrl Pts',(-1.37903818567359,1.,3.64112507791141));
#41254=CARTESIAN_POINT('Ctrl Pts',(-1.37972372481603,1.,3.64852652756456));
#41255=CARTESIAN_POINT('Ctrl Pts',(-1.38035791051213,1.,3.6559455440439));
#41256=CARTESIAN_POINT('Ctrl Pts',(-1.38094856333552,1.,3.66339848520857));
#41257=CARTESIAN_POINT('Ctrl Pts',(-1.38149812653868,1.,3.67088843112262));
#41258=CARTESIAN_POINT('Ctrl Pts',(-1.3820057429062,1.,3.67841038482414));
#41259=CARTESIAN_POINT('Ctrl Pts',(-1.38246852827182,1.,3.68595444983837));
#41260=CARTESIAN_POINT('Ctrl Pts',(-1.38288311171651,1.,3.69350967899526));
#41261=CARTESIAN_POINT('Ctrl Pts',(-1.38324717612865,1.,3.701067921679));
#41262=CARTESIAN_POINT('Ctrl Pts',(-1.38356065402124,1.,3.70862680753347));
#41263=CARTESIAN_POINT('Ctrl Pts',(-1.38382489984586,1.,3.7161876605181));
#41264=CARTESIAN_POINT('Ctrl Pts',(-1.3840421342895,1.,3.72375409358803));
#41265=CARTESIAN_POINT('Ctrl Pts',(-1.38421479111531,1.,3.73133035859282));
#41266=CARTESIAN_POINT('Ctrl Pts',(-1.38434489156458,1.,3.73891976418104));
#41267=CARTESIAN_POINT('Ctrl Pts',(-1.38443344984394,1.,3.74652317167876));
#41268=CARTESIAN_POINT('Ctrl Pts',(-1.38448077997163,1.,3.7541397631875));
#41269=CARTESIAN_POINT('Ctrl Pts',(-1.3844867525335,1.,3.76176768271367));
#41270=CARTESIAN_POINT('Ctrl Pts',(-1.38445107339518,1.,3.76940473185779));
#41271=CARTESIAN_POINT('Ctrl Pts',(-1.38437354551428,1.,3.77704902230418));
#41272=CARTESIAN_POINT('Ctrl Pts',(-1.38425435883756,1.,3.78469969805082));
#41273=CARTESIAN_POINT('Ctrl Pts',(-1.38409399694566,1.,3.79235669640841));
#41274=CARTESIAN_POINT('Ctrl Pts',(-1.38389311766682,1.,3.80002044322111));
#41275=CARTESIAN_POINT('Ctrl Pts',(-1.3836524404622,1.,3.80769156398411));
#41276=CARTESIAN_POINT('Ctrl Pts',(-1.38337263902782,1.,3.81537060817811));
#41277=CARTESIAN_POINT('Ctrl Pts',(-1.38305421262763,1.,3.82305771743829));
#41278=CARTESIAN_POINT('Ctrl Pts',(-1.38269750245138,1.,3.8307526698229));
#41279=CARTESIAN_POINT('Ctrl Pts',(-1.38230274828822,1.,3.83845502790746));
#41280=CARTESIAN_POINT('Ctrl Pts',(-1.38187013346109,1.,3.84616425605764));
#41281=CARTESIAN_POINT('Ctrl Pts',(-1.38139983115049,1.,3.85387983979481));
#41282=CARTESIAN_POINT('Ctrl Pts',(-1.38089205992989,1.,3.86160143043959));
#41283=CARTESIAN_POINT('Ctrl Pts',(-1.38034709213014,1.,3.86932885813068));
#41284=CARTESIAN_POINT('Ctrl Pts',(-1.37976523097073,1.,3.87706205830532));
#41285=CARTESIAN_POINT('Ctrl Pts',(-1.37914679719383,1.,3.88480102249277));
#41286=CARTESIAN_POINT('Ctrl Pts',(-1.3784921128802,1.,3.89254574338496));
#41287=CARTESIAN_POINT('Ctrl Pts',(-1.37780148512792,1.,3.90029615196727));
#41288=CARTESIAN_POINT('Ctrl Pts',(-1.3770751963402,1.,3.90805209523486));
#41289=CARTESIAN_POINT('Ctrl Pts',(-1.37631350505797,1.,3.91581337462644));
#41290=CARTESIAN_POINT('Ctrl Pts',(-1.37551664448242,1.,3.92357976987672));
#41291=CARTESIAN_POINT('Ctrl Pts',(-1.37468482215751,1.,3.93135106761844));
#41292=CARTESIAN_POINT('Ctrl Pts',(-1.37381821967165,1.,3.93912709040818));
#41293=CARTESIAN_POINT('Ctrl Pts',(-1.37291699202807,1.,3.94690771785133));
#41294=CARTESIAN_POINT('Ctrl Pts',(-1.37198126432386,1.,3.95469287280914));
#41295=CARTESIAN_POINT('Ctrl Pts',(-1.3712051561502,1.,3.96092458506535));
#41296=CARTESIAN_POINT('Ctrl Pts',(-1.37060761745635,1.,3.96560037974645));
#41297=CARTESIAN_POINT('Ctrl Pts',(-1.37020239094614,1.,3.9687184694131));
#41298=CARTESIAN_POINT('Ctrl Pts',(-1.36999806084572,1.,3.97027773754922));
#41299=CARTESIAN_POINT('Origin',(-1.36999806084572,0.,3.97027773754922));
#41300=CARTESIAN_POINT('',(-1.22531898815164,1.,4.01728681790024));
#41301=CARTESIAN_POINT('Origin',(0.,0.,0.));
#41302=CARTESIAN_POINT('',(-1.51895082866166,1.,3.42859860294378));
#41303=CARTESIAN_POINT('Origin',(0.,1.,0.));
#41304=CARTESIAN_POINT('Ctrl Pts',(-1.51895082866166,1.,3.42859860294378));
#41305=CARTESIAN_POINT('Ctrl Pts',(-1.51895082866166,0.666666666666667,
3.42859860294378));
#41306=CARTESIAN_POINT('Ctrl Pts',(-1.51895082866166,0.333333333333333,
3.42859860294378));
#41307=CARTESIAN_POINT('Ctrl Pts',(-1.51895082866166,-0.333333333333333,
3.42859860294378));
#41308=CARTESIAN_POINT('Ctrl Pts',(-1.51895082866166,-0.666666666666667,
3.42859860294378));
#41309=CARTESIAN_POINT('Ctrl Pts',(-1.51895082866166,-1.,3.42859860294378));
#41310=CARTESIAN_POINT('Ctrl Pts',(-1.83867539237861,-1.,3.77614523045147));
#41311=CARTESIAN_POINT('Ctrl Pts',(-1.83867539237861,1.,3.77614523045147));
#41312=CARTESIAN_POINT('Ctrl Pts',(-1.83742834010821,-1.,3.77518714458232));
#41313=CARTESIAN_POINT('Ctrl Pts',(-1.83742834010821,1.,3.77518714458232));
#41314=CARTESIAN_POINT('Ctrl Pts',(-1.83493697935064,-1.,3.77326886065484));
#41315=CARTESIAN_POINT('Ctrl Pts',(-1.83493697935064,1.,3.77326886065484));
#41316=CARTESIAN_POINT('Ctrl Pts',(-1.83120816956515,-1.,3.77038509819777));
#41317=CARTESIAN_POINT('Ctrl Pts',(-1.83120816956515,1.,3.77038509819777));
#41318=CARTESIAN_POINT('Ctrl Pts',(-1.82625289221933,-1.,3.76652740355856));
#41319=CARTESIAN_POINT('Ctrl Pts',(-1.82625289221933,1.,3.76652740355856));
#41320=CARTESIAN_POINT('Ctrl Pts',(-1.82008629694924,-1.,3.76168412709652));
#41321=CARTESIAN_POINT('Ctrl Pts',(-1.82008629694924,1.,3.76168412709652));
#41322=CARTESIAN_POINT('Ctrl Pts',(-1.81394729834032,-1.,3.75681965683995));
#41323=CARTESIAN_POINT('Ctrl Pts',(-1.81394729834032,1.,3.75681965683995));
#41324=CARTESIAN_POINT('Ctrl Pts',(-1.80783603939662,-1.,3.75193395888069));
#41325=CARTESIAN_POINT('Ctrl Pts',(-1.80783603939662,1.,3.75193395888069));
#41326=CARTESIAN_POINT('Ctrl Pts',(-1.80175271485519,-1.,3.74702700874954));
#41327=CARTESIAN_POINT('Ctrl Pts',(-1.80175271485519,1.,3.74702700874954));
#41328=CARTESIAN_POINT('Ctrl Pts',(-1.79569757859041,-1.,3.74209880351667));
#41329=CARTESIAN_POINT('Ctrl Pts',(-1.79569757859041,1.,3.74209880351667));
#41330=CARTESIAN_POINT('Ctrl Pts',(-1.78967092823139,-1.,3.73714934729962));
#41331=CARTESIAN_POINT('Ctrl Pts',(-1.78967092823139,1.,3.73714934729962));
#41332=CARTESIAN_POINT('Ctrl Pts',(-1.78367308442682,-1.,3.73217863095022));
#41333=CARTESIAN_POINT('Ctrl Pts',(-1.78367308442682,1.,3.73217863095022));
#41334=CARTESIAN_POINT('Ctrl Pts',(-1.77770437039606,-1.,3.72718661205504));
#41335=CARTESIAN_POINT('Ctrl Pts',(-1.77770437039606,1.,3.72718661205504));
#41336=CARTESIAN_POINT('Ctrl Pts',(-1.77176509401846,-1.,3.72217319911429));
#41337=CARTESIAN_POINT('Ctrl Pts',(-1.77176509401846,1.,3.72217319911429));
#41338=CARTESIAN_POINT('Ctrl Pts',(-1.76585552124549,-1.,3.71713822377675));
#41339=CARTESIAN_POINT('Ctrl Pts',(-1.76585552124549,1.,3.71713822377675));
#41340=CARTESIAN_POINT('Ctrl Pts',(-1.75997588499021,-1.,3.71208146346454));
#41341=CARTESIAN_POINT('Ctrl Pts',(-1.75997588499021,1.,3.71208146346454));
#41342=CARTESIAN_POINT('Ctrl Pts',(-1.75412641804148,-1.,3.70700269736876));
#41343=CARTESIAN_POINT('Ctrl Pts',(-1.75412641804148,1.,3.70700269736876));
#41344=CARTESIAN_POINT('Ctrl Pts',(-1.74830738046092,-1.,3.70190175673422));
#41345=CARTESIAN_POINT('Ctrl Pts',(-1.74830738046092,1.,3.70190175673422));
#41346=CARTESIAN_POINT('Ctrl Pts',(-1.74251908492589,-1.,3.6967785691046));
#41347=CARTESIAN_POINT('Ctrl Pts',(-1.74251908492589,1.,3.6967785691046));
#41348=CARTESIAN_POINT('Ctrl Pts',(-1.73676193254493,-1.,3.69163322647906));
#41349=CARTESIAN_POINT('Ctrl Pts',(-1.73676193254493,1.,3.69163322647906));
#41350=CARTESIAN_POINT('Ctrl Pts',(-1.73103640956647,-1.,3.68646597019188));
#41351=CARTESIAN_POINT('Ctrl Pts',(-1.73103640956647,1.,3.68646597019188));
#41352=CARTESIAN_POINT('Ctrl Pts',(-1.72534302437003,-1.,3.68127704936472));
#41353=CARTESIAN_POINT('Ctrl Pts',(-1.72534302437003,1.,3.68127704936472));
#41354=CARTESIAN_POINT('Ctrl Pts',(-1.71968225581787,-1.,3.67606660374665));
#41355=CARTESIAN_POINT('Ctrl Pts',(-1.71968225581787,1.,3.67606660374665));
#41356=CARTESIAN_POINT('Ctrl Pts',(-1.71405450210392,-1.,3.67083454901629));
#41357=CARTESIAN_POINT('Ctrl Pts',(-1.71405450210392,1.,3.67083454901629));
#41358=CARTESIAN_POINT('Ctrl Pts',(-1.70846001610983,-1.,3.6655804319893));
#41359=CARTESIAN_POINT('Ctrl Pts',(-1.70846001610983,1.,3.6655804319893));
#41360=CARTESIAN_POINT('Ctrl Pts',(-1.70289888566904,-1.,3.6603033877491));
#41361=CARTESIAN_POINT('Ctrl Pts',(-1.70289888566904,1.,3.6603033877491));
#41362=CARTESIAN_POINT('Ctrl Pts',(-1.69737117722559,-1.,3.65500246526798));
#41363=CARTESIAN_POINT('Ctrl Pts',(-1.69737117722559,1.,3.65500246526798));
#41364=CARTESIAN_POINT('Ctrl Pts',(-1.691877054817,-1.,3.64967689827393));
#41365=CARTESIAN_POINT('Ctrl Pts',(-1.691877054817,1.,3.64967689827393));
#41366=CARTESIAN_POINT('Ctrl Pts',(-1.68641690471455,-1.,3.64432638915199));
#41367=CARTESIAN_POINT('Ctrl Pts',(-1.68641690471455,1.,3.64432638915199));
#41368=CARTESIAN_POINT('Ctrl Pts',(-1.68099146651577,-1.,3.63895140887443));
#41369=CARTESIAN_POINT('Ctrl Pts',(-1.68099146651577,1.,3.63895140887443));
#41370=CARTESIAN_POINT('Ctrl Pts',(-1.67560193613145,-1.,3.63355343201211));
#41371=CARTESIAN_POINT('Ctrl Pts',(-1.67560193613145,1.,3.63355343201211));
#41372=CARTESIAN_POINT('Ctrl Pts',(-1.67024966008037,-1.,3.62813422105257));
#41373=CARTESIAN_POINT('Ctrl Pts',(-1.67024966008037,1.,3.62813422105257));
#41374=CARTESIAN_POINT('Ctrl Pts',(-1.66493585923853,-1.,3.62269517989104));
#41375=CARTESIAN_POINT('Ctrl Pts',(-1.66493585923853,1.,3.62269517989104));
#41376=CARTESIAN_POINT('Ctrl Pts',(-1.65966133399186,-1.,3.61723666482457));
#41377=CARTESIAN_POINT('Ctrl Pts',(-1.65966133399186,1.,3.61723666482457));
#41378=CARTESIAN_POINT('Ctrl Pts',(-1.65442619244327,-1.,3.61175734965129));
#41379=CARTESIAN_POINT('Ctrl Pts',(-1.65442619244327,1.,3.61175734965129));
#41380=CARTESIAN_POINT('Ctrl Pts',(-1.64922952425833,-1.,3.60625346556992));
#41381=CARTESIAN_POINT('Ctrl Pts',(-1.64922952425833,1.,3.60625346556992));
#41382=CARTESIAN_POINT('Ctrl Pts',(-1.6440700438558,-1.,3.6007202851384));
#41383=CARTESIAN_POINT('Ctrl Pts',(-1.6440700438558,1.,3.6007202851384));
#41384=CARTESIAN_POINT('Ctrl Pts',(-1.63894676675349,-1.,3.59515368334887));
#41385=CARTESIAN_POINT('Ctrl Pts',(-1.63894676675349,1.,3.59515368334887));
#41386=CARTESIAN_POINT('Ctrl Pts',(-1.63385971451259,-1.,3.58955176627876));
#41387=CARTESIAN_POINT('Ctrl Pts',(-1.63385971451259,1.,3.58955176627876));
#41388=CARTESIAN_POINT('Ctrl Pts',(-1.62881051550748,-1.,3.5839162577435));
#41389=CARTESIAN_POINT('Ctrl Pts',(-1.62881051550748,1.,3.5839162577435));
#41390=CARTESIAN_POINT('Ctrl Pts',(-1.62380329464851,-1.,3.57825455954405));
#41391=CARTESIAN_POINT('Ctrl Pts',(-1.62380329464851,1.,3.57825455954405));
#41392=CARTESIAN_POINT('Ctrl Pts',(-1.61884340915412,-1.,3.57257679609826));
#41393=CARTESIAN_POINT('Ctrl Pts',(-1.61884340915412,1.,3.57257679609826));
#41394=CARTESIAN_POINT('Ctrl Pts',(-1.61393581747522,-1.,3.56689200468404));
#41395=CARTESIAN_POINT('Ctrl Pts',(-1.61393581747522,1.,3.56689200468404));
#41396=CARTESIAN_POINT('Ctrl Pts',(-1.60908344685459,-1.,3.56120432482986));
#41397=CARTESIAN_POINT('Ctrl Pts',(-1.60908344685459,1.,3.56120432482986));
#41398=CARTESIAN_POINT('Ctrl Pts',(-1.60428584699848,-1.,3.55550985096117));
#41399=CARTESIAN_POINT('Ctrl Pts',(-1.60428584699848,1.,3.55550985096117));
#41400=CARTESIAN_POINT('Ctrl Pts',(-1.59953698113444,-1.,3.54979148634426));
#41401=CARTESIAN_POINT('Ctrl Pts',(-1.59953698113444,1.,3.54979148634426));
#41402=CARTESIAN_POINT('Ctrl Pts',(-1.5948276694975,-1.,3.544024581823));
#41403=CARTESIAN_POINT('Ctrl Pts',(-1.5948276694975,1.,3.544024581823));
#41404=CARTESIAN_POINT('Ctrl Pts',(-1.59014958368725,-1.,3.53818616861045));
#41405=CARTESIAN_POINT('Ctrl Pts',(-1.59014958368725,1.,3.53818616861045));
#41406=CARTESIAN_POINT('Ctrl Pts',(-1.58549906268083,-1.,3.53226378147068));
#41407=CARTESIAN_POINT('Ctrl Pts',(-1.58549906268083,1.,3.53226378147068));
#41408=CARTESIAN_POINT('Ctrl Pts',(-1.58088027227856,-1.,3.52626275334899));
#41409=CARTESIAN_POINT('Ctrl Pts',(-1.58088027227856,1.,3.52626275334899));
#41410=CARTESIAN_POINT('Ctrl Pts',(-1.5763104998818,-1.,3.52021847865961));
#41411=CARTESIAN_POINT('Ctrl Pts',(-1.5763104998818,1.,3.52021847865961));
#41412=CARTESIAN_POINT('Ctrl Pts',(-1.57181569799774,-1.,3.51418598431733));
#41413=CARTESIAN_POINT('Ctrl Pts',(-1.57181569799774,1.,3.51418598431733));
#41414=CARTESIAN_POINT('Ctrl Pts',(-1.56742097575041,-1.,3.50821771695427));
#41415=CARTESIAN_POINT('Ctrl Pts',(-1.56742097575041,1.,3.50821771695427));
#41416=CARTESIAN_POINT('Ctrl Pts',(-1.56314187758689,-1.,3.50234321621607));
#41417=CARTESIAN_POINT('Ctrl Pts',(-1.56314187758689,1.,3.50234321621607));
#41418=CARTESIAN_POINT('Ctrl Pts',(-1.55897703097859,-1.,3.49655185179623));
#41419=CARTESIAN_POINT('Ctrl Pts',(-1.55897703097859,1.,3.49655185179623));
#41420=CARTESIAN_POINT('Ctrl Pts',(-1.5548959590107,-1.,3.49076460877317));
#41421=CARTESIAN_POINT('Ctrl Pts',(-1.5548959590107,1.,3.49076460877317));
#41422=CARTESIAN_POINT('Ctrl Pts',(-1.55084702970382,-1.,3.48485155928414));
#41423=CARTESIAN_POINT('Ctrl Pts',(-1.55084702970382,1.,3.48485155928414));
#41424=CARTESIAN_POINT('Ctrl Pts',(-1.54678009290207,-1.,3.47868272898599));
#41425=CARTESIAN_POINT('Ctrl Pts',(-1.54678009290207,1.,3.47868272898599));
#41426=CARTESIAN_POINT('Ctrl Pts',(-1.54266605398152,-1.,3.47217189224576));
#41427=CARTESIAN_POINT('Ctrl Pts',(-1.54266605398152,1.,3.47217189224576));
#41428=CARTESIAN_POINT('Ctrl Pts',(-1.53851507915533,-1.,3.46531752207222));
#41429=CARTESIAN_POINT('Ctrl Pts',(-1.53851507915533,1.,3.46531752207222));
#41430=CARTESIAN_POINT('Ctrl Pts',(-1.53440195378902,-1.,3.45825932955273));
#41431=CARTESIAN_POINT('Ctrl Pts',(-1.53440195378902,1.,3.45825932955273));
#41432=CARTESIAN_POINT('Ctrl Pts',(-1.530462444618,-1.,3.45127136828667));
#41433=CARTESIAN_POINT('Ctrl Pts',(-1.530462444618,1.,3.45127136828667));
#41434=CARTESIAN_POINT('Ctrl Pts',(-1.52686242875717,-1.,3.44469547527));
#41435=CARTESIAN_POINT('Ctrl Pts',(-1.52686242875717,1.,3.44469547527));
#41436=CARTESIAN_POINT('Ctrl Pts',(-1.52377348950429,-1.,3.43888895974182));
#41437=CARTESIAN_POINT('Ctrl Pts',(-1.52377348950429,1.,3.43888895974182));
#41438=CARTESIAN_POINT('Ctrl Pts',(-1.52134826724227,-1.,3.43417156977749));
#41439=CARTESIAN_POINT('Ctrl Pts',(-1.52134826724227,1.,3.43417156977749));
#41440=CARTESIAN_POINT('Ctrl Pts',(-1.51969006980792,-1.,3.43076036253384));
#41441=CARTESIAN_POINT('Ctrl Pts',(-1.51969006980792,1.,3.43076036253384));
#41442=CARTESIAN_POINT('Ctrl Pts',(-1.51901585838879,-1.,3.42915787669388));
#41443=CARTESIAN_POINT('Ctrl Pts',(-1.51901585838879,1.,3.42915787669388));
#41444=CARTESIAN_POINT('Ctrl Pts',(-1.51888450659497,-1.,3.42860527148835));
#41445=CARTESIAN_POINT('Ctrl Pts',(-1.51888450659497,1.,3.42860527148835));
#41446=CARTESIAN_POINT('Ctrl Pts',(-1.51896318668306,-1.,3.42852521763648));
#41447=CARTESIAN_POINT('Ctrl Pts',(-1.51896318668306,1.,3.42852521763648));
#41448=CARTESIAN_POINT('Ctrl Pts',(-1.519044091397,-1.,3.42855728381368));
#41449=CARTESIAN_POINT('Ctrl Pts',(-1.519044091397,1.,3.42855728381368));
#41450=CARTESIAN_POINT('',(-1.83867539237861,1.,3.77614523045147));
#41451=CARTESIAN_POINT('Ctrl Pts',(-1.83867539237861,1.,3.77614523045147));
#41452=CARTESIAN_POINT('Ctrl Pts',(-1.83742834010821,1.,3.77518714458232));
#41453=CARTESIAN_POINT('Ctrl Pts',(-1.83493697935064,1.,3.77326886065484));
#41454=CARTESIAN_POINT('Ctrl Pts',(-1.83120816956515,1.,3.77038509819777));
#41455=CARTESIAN_POINT('Ctrl Pts',(-1.82625289221933,1.,3.76652740355856));
#41456=CARTESIAN_POINT('Ctrl Pts',(-1.82008629694924,1.,3.76168412709652));
#41457=CARTESIAN_POINT('Ctrl Pts',(-1.81394729834032,1.,3.75681965683995));
#41458=CARTESIAN_POINT('Ctrl Pts',(-1.80783603939662,1.,3.75193395888069));
#41459=CARTESIAN_POINT('Ctrl Pts',(-1.80175271485519,1.,3.74702700874954));
#41460=CARTESIAN_POINT('Ctrl Pts',(-1.79569757859041,1.,3.74209880351667));
#41461=CARTESIAN_POINT('Ctrl Pts',(-1.78967092823139,1.,3.73714934729962));
#41462=CARTESIAN_POINT('Ctrl Pts',(-1.78367308442682,1.,3.73217863095022));
#41463=CARTESIAN_POINT('Ctrl Pts',(-1.77770437039606,1.,3.72718661205504));
#41464=CARTESIAN_POINT('Ctrl Pts',(-1.77176509401846,1.,3.72217319911429));
#41465=CARTESIAN_POINT('Ctrl Pts',(-1.76585552124549,1.,3.71713822377675));
#41466=CARTESIAN_POINT('Ctrl Pts',(-1.75997588499021,1.,3.71208146346454));
#41467=CARTESIAN_POINT('Ctrl Pts',(-1.75412641804148,1.,3.70700269736876));
#41468=CARTESIAN_POINT('Ctrl Pts',(-1.74830738046092,1.,3.70190175673422));
#41469=CARTESIAN_POINT('Ctrl Pts',(-1.74251908492589,1.,3.6967785691046));
#41470=CARTESIAN_POINT('Ctrl Pts',(-1.73676193254493,1.,3.69163322647906));
#41471=CARTESIAN_POINT('Ctrl Pts',(-1.73103640956647,1.,3.68646597019188));
#41472=CARTESIAN_POINT('Ctrl Pts',(-1.72534302437003,1.,3.68127704936472));
#41473=CARTESIAN_POINT('Ctrl Pts',(-1.71968225581787,1.,3.67606660374665));
#41474=CARTESIAN_POINT('Ctrl Pts',(-1.71405450210392,1.,3.67083454901629));
#41475=CARTESIAN_POINT('Ctrl Pts',(-1.70846001610983,1.,3.6655804319893));
#41476=CARTESIAN_POINT('Ctrl Pts',(-1.70289888566904,1.,3.6603033877491));
#41477=CARTESIAN_POINT('Ctrl Pts',(-1.69737117722559,1.,3.65500246526798));
#41478=CARTESIAN_POINT('Ctrl Pts',(-1.691877054817,1.,3.64967689827393));
#41479=CARTESIAN_POINT('Ctrl Pts',(-1.68641690471455,1.,3.64432638915199));
#41480=CARTESIAN_POINT('Ctrl Pts',(-1.68099146651577,1.,3.63895140887443));
#41481=CARTESIAN_POINT('Ctrl Pts',(-1.67560193613145,1.,3.63355343201211));
#41482=CARTESIAN_POINT('Ctrl Pts',(-1.67024966008037,1.,3.62813422105257));
#41483=CARTESIAN_POINT('Ctrl Pts',(-1.66493585923853,1.,3.62269517989104));
#41484=CARTESIAN_POINT('Ctrl Pts',(-1.65966133399186,1.,3.61723666482457));
#41485=CARTESIAN_POINT('Ctrl Pts',(-1.65442619244327,1.,3.61175734965129));
#41486=CARTESIAN_POINT('Ctrl Pts',(-1.64922952425833,1.,3.60625346556992));
#41487=CARTESIAN_POINT('Ctrl Pts',(-1.6440700438558,1.,3.6007202851384));
#41488=CARTESIAN_POINT('Ctrl Pts',(-1.63894676675349,1.,3.59515368334887));
#41489=CARTESIAN_POINT('Ctrl Pts',(-1.63385971451259,1.,3.58955176627876));
#41490=CARTESIAN_POINT('Ctrl Pts',(-1.62881051550748,1.,3.5839162577435));
#41491=CARTESIAN_POINT('Ctrl Pts',(-1.62380329464851,1.,3.57825455954405));
#41492=CARTESIAN_POINT('Ctrl Pts',(-1.61884340915412,1.,3.57257679609826));
#41493=CARTESIAN_POINT('Ctrl Pts',(-1.61393581747522,1.,3.56689200468404));
#41494=CARTESIAN_POINT('Ctrl Pts',(-1.60908344685459,1.,3.56120432482986));
#41495=CARTESIAN_POINT('Ctrl Pts',(-1.60428584699848,1.,3.55550985096117));
#41496=CARTESIAN_POINT('Ctrl Pts',(-1.59953698113444,1.,3.54979148634426));
#41497=CARTESIAN_POINT('Ctrl Pts',(-1.5948276694975,1.,3.544024581823));
#41498=CARTESIAN_POINT('Ctrl Pts',(-1.59014958368725,1.,3.53818616861045));
#41499=CARTESIAN_POINT('Ctrl Pts',(-1.58549906268083,1.,3.53226378147068));
#41500=CARTESIAN_POINT('Ctrl Pts',(-1.58088027227856,1.,3.52626275334899));
#41501=CARTESIAN_POINT('Ctrl Pts',(-1.5763104998818,1.,3.52021847865961));
#41502=CARTESIAN_POINT('Ctrl Pts',(-1.57181569799774,1.,3.51418598431733));
#41503=CARTESIAN_POINT('Ctrl Pts',(-1.56742097575041,1.,3.50821771695427));
#41504=CARTESIAN_POINT('Ctrl Pts',(-1.56314187758689,1.,3.50234321621607));
#41505=CARTESIAN_POINT('Ctrl Pts',(-1.55897703097859,1.,3.49655185179623));
#41506=CARTESIAN_POINT('Ctrl Pts',(-1.5548959590107,1.,3.49076460877317));
#41507=CARTESIAN_POINT('Ctrl Pts',(-1.55084702970382,1.,3.48485155928414));
#41508=CARTESIAN_POINT('Ctrl Pts',(-1.54678009290207,1.,3.47868272898599));
#41509=CARTESIAN_POINT('Ctrl Pts',(-1.54266605398152,1.,3.47217189224576));
#41510=CARTESIAN_POINT('Ctrl Pts',(-1.53851507915533,1.,3.46531752207222));
#41511=CARTESIAN_POINT('Ctrl Pts',(-1.53440195378902,1.,3.45825932955273));
#41512=CARTESIAN_POINT('Ctrl Pts',(-1.530462444618,1.,3.45127136828667));
#41513=CARTESIAN_POINT('Ctrl Pts',(-1.52686242875717,1.,3.44469547527));
#41514=CARTESIAN_POINT('Ctrl Pts',(-1.52377348950429,1.,3.43888895974182));
#41515=CARTESIAN_POINT('Ctrl Pts',(-1.52134826724227,1.,3.43417156977749));
#41516=CARTESIAN_POINT('Ctrl Pts',(-1.5198144909343,1.,3.4310163189349));
#41517=CARTESIAN_POINT('Ctrl Pts',(-1.51914806898539,1.,3.42946838852728));
#41518=CARTESIAN_POINT('Ctrl Pts',(-1.51895133295017,1.,3.42884302333978));
#41519=CARTESIAN_POINT('Ctrl Pts',(-1.51893924967231,1.,3.42864616361967));
#41520=CARTESIAN_POINT('Ctrl Pts',(-1.51895082866166,1.,3.42859860294378));
#41521=CARTESIAN_POINT('',(-1.83867539237861,0.,3.77614523045147));
#41522=CARTESIAN_POINT('Ctrl Pts',(-1.88088939428811,-1.,3.24418789321065));
#41523=CARTESIAN_POINT('Ctrl Pts',(-1.88088939428811,1.,3.24418789321065));
#41524=CARTESIAN_POINT('Ctrl Pts',(-1.8809110068042,-1.,3.24410359189733));
#41525=CARTESIAN_POINT('Ctrl Pts',(-1.8809110068042,1.,3.24410359189733));
#41526=CARTESIAN_POINT('Ctrl Pts',(-1.8810220187274,-1.,3.24408699284449));
#41527=CARTESIAN_POINT('Ctrl Pts',(-1.8810220187274,1.,3.24408699284449));
#41528=CARTESIAN_POINT('Ctrl Pts',(-1.88139187908347,-1.,3.24451807186964));
#41529=CARTESIAN_POINT('Ctrl Pts',(-1.88139187908347,1.,3.24451807186964));
#41530=CARTESIAN_POINT('Ctrl Pts',(-1.88229202583187,-1.,3.24600543790876));
#41531=CARTESIAN_POINT('Ctrl Pts',(-1.88229202583187,1.,3.24600543790876));
#41532=CARTESIAN_POINT('Ctrl Pts',(-1.88407708646435,-1.,3.24935200512055));
#41533=CARTESIAN_POINT('Ctrl Pts',(-1.88407708646435,1.,3.24935200512055));
#41534=CARTESIAN_POINT('Ctrl Pts',(-1.88646802523372,-1.,3.25408686339298));
#41535=CARTESIAN_POINT('Ctrl Pts',(-1.88646802523372,1.,3.25408686339298));
#41536=CARTESIAN_POINT('Ctrl Pts',(-1.88934996203508,-1.,3.2599988519361));
#41537=CARTESIAN_POINT('Ctrl Pts',(-1.88934996203508,1.,3.2599988519361));
#41538=CARTESIAN_POINT('Ctrl Pts',(-1.89255393500769,-1.,3.2667765388833));
#41539=CARTESIAN_POINT('Ctrl Pts',(-1.89255393500769,1.,3.2667765388833));
#41540=CARTESIAN_POINT('Ctrl Pts',(-1.89589172903662,-1.,3.27407108932908));
#41541=CARTESIAN_POINT('Ctrl Pts',(-1.89589172903662,1.,3.27407108932908));
#41542=CARTESIAN_POINT('Ctrl Pts',(-1.89918429230425,-1.,3.28154737912287));
#41543=CARTESIAN_POINT('Ctrl Pts',(-1.89918429230425,1.,3.28154737912287));
#41544=CARTESIAN_POINT('Ctrl Pts',(-1.9022897124757,-1.,3.28893448600364));
#41545=CARTESIAN_POINT('Ctrl Pts',(-1.9022897124757,1.,3.28893448600364));
#41546=CARTESIAN_POINT('Ctrl Pts',(-1.9051389186417,-1.,3.29608978722258));
#41547=CARTESIAN_POINT('Ctrl Pts',(-1.9051389186417,1.,3.29608978722258));
#41548=CARTESIAN_POINT('Ctrl Pts',(-1.90773912171424,-1.,3.30300595568341));
#41549=CARTESIAN_POINT('Ctrl Pts',(-1.90773912171424,1.,3.30300595568341));
#41550=CARTESIAN_POINT('Ctrl Pts',(-1.91014297830502,-1.,3.30975721158694));
#41551=CARTESIAN_POINT('Ctrl Pts',(-1.91014297830502,1.,3.30975721158694));
#41552=CARTESIAN_POINT('Ctrl Pts',(-1.91242616234459,-1.,3.31646052426395));
#41553=CARTESIAN_POINT('Ctrl Pts',(-1.91242616234459,1.,3.31646052426395));
#41554=CARTESIAN_POINT('Ctrl Pts',(-1.91466343916612,-1.,3.32323403454507));
#41555=CARTESIAN_POINT('Ctrl Pts',(-1.91466343916612,1.,3.32323403454507));
#41556=CARTESIAN_POINT('Ctrl Pts',(-1.91690081930297,-1.,3.33014884257812));
#41557=CARTESIAN_POINT('Ctrl Pts',(-1.91690081930297,1.,3.33014884257812));
#41558=CARTESIAN_POINT('Ctrl Pts',(-1.91914609610173,-1.,3.33721230709948));
#41559=CARTESIAN_POINT('Ctrl Pts',(-1.91914609610173,1.,3.33721230709948));
#41560=CARTESIAN_POINT('Ctrl Pts',(-1.92138450828378,-1.,3.34439448941915));
#41561=CARTESIAN_POINT('Ctrl Pts',(-1.92138450828378,1.,3.34439448941915));
#41562=CARTESIAN_POINT('Ctrl Pts',(-1.92358838440518,-1.,3.35164424847206));
#41563=CARTESIAN_POINT('Ctrl Pts',(-1.92358838440518,1.,3.35164424847206));
#41564=CARTESIAN_POINT('Ctrl Pts',(-1.92572846125763,-1.,3.35890824422976));
#41565=CARTESIAN_POINT('Ctrl Pts',(-1.92572846125763,1.,3.35890824422976));
#41566=CARTESIAN_POINT('Ctrl Pts',(-1.92778626543803,-1.,3.36615168657597));
#41567=CARTESIAN_POINT('Ctrl Pts',(-1.92778626543803,1.,3.36615168657597));
#41568=CARTESIAN_POINT('Ctrl Pts',(-1.92975993109897,-1.,3.37336807068078));
#41569=CARTESIAN_POINT('Ctrl Pts',(-1.92975993109897,1.,3.37336807068078));
#41570=CARTESIAN_POINT('Ctrl Pts',(-1.93165739093292,-1.,3.38056768525577));
#41571=CARTESIAN_POINT('Ctrl Pts',(-1.93165739093292,1.,3.38056768525577));
#41572=CARTESIAN_POINT('Ctrl Pts',(-1.93349233176794,-1.,3.38777076883267));
#41573=CARTESIAN_POINT('Ctrl Pts',(-1.93349233176794,1.,3.38777076883267));
#41574=CARTESIAN_POINT('Ctrl Pts',(-1.93527929945982,-1.,3.39499923640789));
#41575=CARTESIAN_POINT('Ctrl Pts',(-1.93527929945982,1.,3.39499923640789));
#41576=CARTESIAN_POINT('Ctrl Pts',(-1.93702857723089,-1.,3.40226802104093));
#41577=CARTESIAN_POINT('Ctrl Pts',(-1.93702857723089,1.,3.40226802104093));
#41578=CARTESIAN_POINT('Ctrl Pts',(-1.93874306008132,-1.,3.40957978266622));
#41579=CARTESIAN_POINT('Ctrl Pts',(-1.93874306008132,1.,3.40957978266622));
#41580=CARTESIAN_POINT('Ctrl Pts',(-1.94042111965237,-1.,3.41692971994082));
#41581=CARTESIAN_POINT('Ctrl Pts',(-1.94042111965237,1.,3.41692971994082));
#41582=CARTESIAN_POINT('Ctrl Pts',(-1.94205835913692,-1.,3.42430850941497));
#41583=CARTESIAN_POINT('Ctrl Pts',(-1.94205835913692,1.,3.42430850941497));
#41584=CARTESIAN_POINT('Ctrl Pts',(-1.94364973660285,-1.,3.43170586602436));
#41585=CARTESIAN_POINT('Ctrl Pts',(-1.94364973660285,1.,3.43170586602436));
#41586=CARTESIAN_POINT('Ctrl Pts',(-1.94519168842883,-1.,3.43911410197693));
#41587=CARTESIAN_POINT('Ctrl Pts',(-1.94519168842883,1.,3.43911410197693));
#41588=CARTESIAN_POINT('Ctrl Pts',(-1.94668377715332,-1.,3.44653088665685));
#41589=CARTESIAN_POINT('Ctrl Pts',(-1.94668377715332,1.,3.44653088665685));
#41590=CARTESIAN_POINT('Ctrl Pts',(-1.94812754766524,-1.,3.45395731584051));
#41591=CARTESIAN_POINT('Ctrl Pts',(-1.94812754766524,1.,3.45395731584051));
#41592=CARTESIAN_POINT('Ctrl Pts',(-1.94952575850196,-1.,3.46139661060959));
#41593=CARTESIAN_POINT('Ctrl Pts',(-1.94952575850196,1.,3.46139661060959));
#41594=CARTESIAN_POINT('Ctrl Pts',(-1.95088147859876,-1.,3.4688525897419));
#41595=CARTESIAN_POINT('Ctrl Pts',(-1.95088147859876,1.,3.4688525897419));
#41596=CARTESIAN_POINT('Ctrl Pts',(-1.95219722189878,-1.,3.47632820495926));
#41597=CARTESIAN_POINT('Ctrl Pts',(-1.95219722189878,1.,3.47632820495926));
#41598=CARTESIAN_POINT('Ctrl Pts',(-1.95347412486316,-1.,3.48382414832648));
#41599=CARTESIAN_POINT('Ctrl Pts',(-1.95347412486316,1.,3.48382414832648));
#41600=CARTESIAN_POINT('Ctrl Pts',(-1.95471236969653,-1.,3.49133956289154));
#41601=CARTESIAN_POINT('Ctrl Pts',(-1.95471236969653,1.,3.49133956289154));
#41602=CARTESIAN_POINT('Ctrl Pts',(-1.9559115382367,-1.,3.49887263575602));
#41603=CARTESIAN_POINT('Ctrl Pts',(-1.9559115382367,1.,3.49887263575602));
#41604=CARTESIAN_POINT('Ctrl Pts',(-1.95707099606514,-1.,3.50642124159913));
#41605=CARTESIAN_POINT('Ctrl Pts',(-1.95707099606514,1.,3.50642124159913));
#41606=CARTESIAN_POINT('Ctrl Pts',(-1.95819025316768,-1.,3.51398354617772));
#41607=CARTESIAN_POINT('Ctrl Pts',(-1.95819025316768,1.,3.51398354617772));
#41608=CARTESIAN_POINT('Ctrl Pts',(-1.95926936324436,-1.,3.52155867431438));
#41609=CARTESIAN_POINT('Ctrl Pts',(-1.95926936324436,1.,3.52155867431438));
#41610=CARTESIAN_POINT('Ctrl Pts',(-1.96030879411534,-1.,3.52914648844289));
#41611=CARTESIAN_POINT('Ctrl Pts',(-1.96030879411534,1.,3.52914648844289));
#41612=CARTESIAN_POINT('Ctrl Pts',(-1.96130926212661,-1.,3.53674730625759));
#41613=CARTESIAN_POINT('Ctrl Pts',(-1.96130926212661,1.,3.53674730625759));
#41614=CARTESIAN_POINT('Ctrl Pts',(-1.96227157573058,-1.,3.54436163300425));
#41615=CARTESIAN_POINT('Ctrl Pts',(-1.96227157573058,1.,3.54436163300425));
#41616=CARTESIAN_POINT('Ctrl Pts',(-1.96319648628667,-1.,3.55198990600929));
#41617=CARTESIAN_POINT('Ctrl Pts',(-1.96319648628667,1.,3.55198990600929));
#41618=CARTESIAN_POINT('Ctrl Pts',(-1.96408450906868,-1.,3.55963218706201));
#41619=CARTESIAN_POINT('Ctrl Pts',(-1.96408450906868,1.,3.55963218706201));
#41620=CARTESIAN_POINT('Ctrl Pts',(-1.96493594634643,-1.,3.56728820357933));
#41621=CARTESIAN_POINT('Ctrl Pts',(-1.96493594634643,1.,3.56728820357933));
#41622=CARTESIAN_POINT('Ctrl Pts',(-1.96575096652857,-1.,3.57495748601088));
#41623=CARTESIAN_POINT('Ctrl Pts',(-1.96575096652857,1.,3.57495748601088));
#41624=CARTESIAN_POINT('Ctrl Pts',(-1.9665296668894,-1.,3.58263947663884));
#41625=CARTESIAN_POINT('Ctrl Pts',(-1.9665296668894,1.,3.58263947663884));
#41626=CARTESIAN_POINT('Ctrl Pts',(-1.96727213799507,-1.,3.5903336402273));
#41627=CARTESIAN_POINT('Ctrl Pts',(-1.96727213799507,1.,3.5903336402273));
#41628=CARTESIAN_POINT('Ctrl Pts',(-1.96797854118257,-1.,3.59803959819725));
#41629=CARTESIAN_POINT('Ctrl Pts',(-1.96797854118257,1.,3.59803959819725));
#41630=CARTESIAN_POINT('Ctrl Pts',(-1.96864911885775,-1.,3.60575714017676));
#41631=CARTESIAN_POINT('Ctrl Pts',(-1.96864911885775,1.,3.60575714017676));
#41632=CARTESIAN_POINT('Ctrl Pts',(-1.96928416040712,-1.,3.61348615496393));
#41633=CARTESIAN_POINT('Ctrl Pts',(-1.96928416040712,1.,3.61348615496393));
#41634=CARTESIAN_POINT('Ctrl Pts',(-1.96988398129888,-1.,3.62122658401722));
#41635=CARTESIAN_POINT('Ctrl Pts',(-1.96988398129888,1.,3.62122658401722));
#41636=CARTESIAN_POINT('Ctrl Pts',(-1.97044889850518,-1.,3.62897836973397));
#41637=CARTESIAN_POINT('Ctrl Pts',(-1.97044889850518,1.,3.62897836973397));
#41638=CARTESIAN_POINT('Ctrl Pts',(-1.97097920454698,-1.,3.63674139590853));
#41639=CARTESIAN_POINT('Ctrl Pts',(-1.97097920454698,1.,3.63674139590853));
#41640=CARTESIAN_POINT('Ctrl Pts',(-1.97147515441539,-1.,3.64451546724221));
#41641=CARTESIAN_POINT('Ctrl Pts',(-1.97147515441539,1.,3.64451546724221));
#41642=CARTESIAN_POINT('Ctrl Pts',(-1.97193697240645,-1.,3.65230034717364));
#41643=CARTESIAN_POINT('Ctrl Pts',(-1.97193697240645,1.,3.65230034717364));
#41644=CARTESIAN_POINT('Ctrl Pts',(-1.97236485439317,-1.,3.66009578166865));
#41645=CARTESIAN_POINT('Ctrl Pts',(-1.97236485439317,1.,3.66009578166865));
#41646=CARTESIAN_POINT('Ctrl Pts',(-1.9727589719863,-1.,3.66790152751984));
#41647=CARTESIAN_POINT('Ctrl Pts',(-1.9727589719863,1.,3.66790152751984));
#41648=CARTESIAN_POINT('Ctrl Pts',(-1.97311947678035,-1.,3.67571738106175));
#41649=CARTESIAN_POINT('Ctrl Pts',(-1.97311947678035,1.,3.67571738106175));
#41650=CARTESIAN_POINT('Ctrl Pts',(-1.97344650303631,-1.,3.68354319913416));
#41651=CARTESIAN_POINT('Ctrl Pts',(-1.97344650303631,1.,3.68354319913416));
#41652=CARTESIAN_POINT('Ctrl Pts',(-1.97374016224397,-1.,3.69137888597855));
#41653=CARTESIAN_POINT('Ctrl Pts',(-1.97374016224397,1.,3.69137888597855));
#41654=CARTESIAN_POINT('Ctrl Pts',(-1.97394846382289,-1.,3.69765528558292));
#41655=CARTESIAN_POINT('Ctrl Pts',(-1.97394846382289,1.,3.69765528558292));
#41656=CARTESIAN_POINT('Ctrl Pts',(-1.97408973726149,-1.,3.70236698911837));
#41657=CARTESIAN_POINT('Ctrl Pts',(-1.97408973726149,1.,3.70236698911837));
#41658=CARTESIAN_POINT('Ctrl Pts',(-1.974177276451,-1.,3.7055100813194));
#41659=CARTESIAN_POINT('Ctrl Pts',(-1.974177276451,1.,3.7055100813194));
#41660=CARTESIAN_POINT('Ctrl Pts',(-1.97421938526992,-1.,3.70708211654725));
#41661=CARTESIAN_POINT('Ctrl Pts',(-1.97421938526992,1.,3.70708211654725));
#41662=CARTESIAN_POINT('',(-1.88097764062542,1.,3.24413672884902));
#41663=CARTESIAN_POINT('Ctrl Pts',(-1.88097764062542,-1.,3.24413672884902));
#41664=CARTESIAN_POINT('Ctrl Pts',(-1.88097764062542,-0.666666666666667,
3.24413672884902));
#41665=CARTESIAN_POINT('Ctrl Pts',(-1.88097764062542,-0.333333333333333,
3.24413672884902));
#41666=CARTESIAN_POINT('Ctrl Pts',(-1.88097764062542,0.333333333333333,
3.24413672884902));
#41667=CARTESIAN_POINT('Ctrl Pts',(-1.88097764062542,0.666666666666667,
3.24413672884902));
#41668=CARTESIAN_POINT('Ctrl Pts',(-1.88097764062542,1.,3.24413672884902));
#41669=CARTESIAN_POINT('',(-1.97421938526992,1.,3.70708211654725));
#41670=CARTESIAN_POINT('',(-1.97421938526992,0.,3.70708211654725));
#41671=CARTESIAN_POINT('Ctrl Pts',(-1.88097764062542,1.,3.24413672884902));
#41672=CARTESIAN_POINT('Ctrl Pts',(-1.88102292397987,1.,3.24415531671311));
#41673=CARTESIAN_POINT('Ctrl Pts',(-1.88117508446657,1.,3.24428080352952));
#41674=CARTESIAN_POINT('Ctrl Pts',(-1.88156537699118,1.,3.24480754675942));
#41675=CARTESIAN_POINT('Ctrl Pts',(-1.88242596600422,1.,3.24625654410705));
#41676=CARTESIAN_POINT('Ctrl Pts',(-1.88407708646435,1.,3.24935200512055));
#41677=CARTESIAN_POINT('Ctrl Pts',(-1.88646802523372,1.,3.25408686339298));
#41678=CARTESIAN_POINT('Ctrl Pts',(-1.88934996203508,1.,3.2599988519361));
#41679=CARTESIAN_POINT('Ctrl Pts',(-1.89255393500769,1.,3.2667765388833));
#41680=CARTESIAN_POINT('Ctrl Pts',(-1.89589172903662,1.,3.27407108932908));
#41681=CARTESIAN_POINT('Ctrl Pts',(-1.89918429230425,1.,3.28154737912287));
#41682=CARTESIAN_POINT('Ctrl Pts',(-1.9022897124757,1.,3.28893448600364));
#41683=CARTESIAN_POINT('Ctrl Pts',(-1.9051389186417,1.,3.29608978722258));
#41684=CARTESIAN_POINT('Ctrl Pts',(-1.90773912171424,1.,3.30300595568341));
#41685=CARTESIAN_POINT('Ctrl Pts',(-1.91014297830502,1.,3.30975721158694));
#41686=CARTESIAN_POINT('Ctrl Pts',(-1.91242616234459,1.,3.31646052426395));
#41687=CARTESIAN_POINT('Ctrl Pts',(-1.91466343916612,1.,3.32323403454507));
#41688=CARTESIAN_POINT('Ctrl Pts',(-1.91690081930297,1.,3.33014884257812));
#41689=CARTESIAN_POINT('Ctrl Pts',(-1.91914609610173,1.,3.33721230709948));
#41690=CARTESIAN_POINT('Ctrl Pts',(-1.92138450828378,1.,3.34439448941915));
#41691=CARTESIAN_POINT('Ctrl Pts',(-1.92358838440518,1.,3.35164424847206));
#41692=CARTESIAN_POINT('Ctrl Pts',(-1.92572846125763,1.,3.35890824422976));
#41693=CARTESIAN_POINT('Ctrl Pts',(-1.92778626543803,1.,3.36615168657597));
#41694=CARTESIAN_POINT('Ctrl Pts',(-1.92975993109897,1.,3.37336807068078));
#41695=CARTESIAN_POINT('Ctrl Pts',(-1.93165739093292,1.,3.38056768525577));
#41696=CARTESIAN_POINT('Ctrl Pts',(-1.93349233176794,1.,3.38777076883267));
#41697=CARTESIAN_POINT('Ctrl Pts',(-1.93527929945982,1.,3.39499923640789));
#41698=CARTESIAN_POINT('Ctrl Pts',(-1.93702857723089,1.,3.40226802104093));
#41699=CARTESIAN_POINT('Ctrl Pts',(-1.93874306008132,1.,3.40957978266622));
#41700=CARTESIAN_POINT('Ctrl Pts',(-1.94042111965237,1.,3.41692971994082));
#41701=CARTESIAN_POINT('Ctrl Pts',(-1.94205835913692,1.,3.42430850941497));
#41702=CARTESIAN_POINT('Ctrl Pts',(-1.94364973660285,1.,3.43170586602436));
#41703=CARTESIAN_POINT('Ctrl Pts',(-1.94519168842883,1.,3.43911410197693));
#41704=CARTESIAN_POINT('Ctrl Pts',(-1.94668377715332,1.,3.44653088665685));
#41705=CARTESIAN_POINT('Ctrl Pts',(-1.94812754766524,1.,3.45395731584051));
#41706=CARTESIAN_POINT('Ctrl Pts',(-1.94952575850196,1.,3.46139661060959));
#41707=CARTESIAN_POINT('Ctrl Pts',(-1.95088147859876,1.,3.4688525897419));
#41708=CARTESIAN_POINT('Ctrl Pts',(-1.95219722189878,1.,3.47632820495926));
#41709=CARTESIAN_POINT('Ctrl Pts',(-1.95347412486316,1.,3.48382414832648));
#41710=CARTESIAN_POINT('Ctrl Pts',(-1.95471236969653,1.,3.49133956289154));
#41711=CARTESIAN_POINT('Ctrl Pts',(-1.9559115382367,1.,3.49887263575602));
#41712=CARTESIAN_POINT('Ctrl Pts',(-1.95707099606514,1.,3.50642124159913));
#41713=CARTESIAN_POINT('Ctrl Pts',(-1.95819025316768,1.,3.51398354617772));
#41714=CARTESIAN_POINT('Ctrl Pts',(-1.95926936324436,1.,3.52155867431438));
#41715=CARTESIAN_POINT('Ctrl Pts',(-1.96030879411534,1.,3.52914648844289));
#41716=CARTESIAN_POINT('Ctrl Pts',(-1.96130926212661,1.,3.53674730625759));
#41717=CARTESIAN_POINT('Ctrl Pts',(-1.96227157573058,1.,3.54436163300425));
#41718=CARTESIAN_POINT('Ctrl Pts',(-1.96319648628667,1.,3.55198990600929));
#41719=CARTESIAN_POINT('Ctrl Pts',(-1.96408450906868,1.,3.55963218706201));
#41720=CARTESIAN_POINT('Ctrl Pts',(-1.96493594634643,1.,3.56728820357933));
#41721=CARTESIAN_POINT('Ctrl Pts',(-1.96575096652857,1.,3.57495748601088));
#41722=CARTESIAN_POINT('Ctrl Pts',(-1.9665296668894,1.,3.58263947663884));
#41723=CARTESIAN_POINT('Ctrl Pts',(-1.96727213799507,1.,3.5903336402273));
#41724=CARTESIAN_POINT('Ctrl Pts',(-1.96797854118257,1.,3.59803959819725));
#41725=CARTESIAN_POINT('Ctrl Pts',(-1.96864911885775,1.,3.60575714017676));
#41726=CARTESIAN_POINT('Ctrl Pts',(-1.96928416040712,1.,3.61348615496393));
#41727=CARTESIAN_POINT('Ctrl Pts',(-1.96988398129888,1.,3.62122658401722));
#41728=CARTESIAN_POINT('Ctrl Pts',(-1.97044889850518,1.,3.62897836973397));
#41729=CARTESIAN_POINT('Ctrl Pts',(-1.97097920454698,1.,3.63674139590853));
#41730=CARTESIAN_POINT('Ctrl Pts',(-1.97147515441539,1.,3.64451546724221));
#41731=CARTESIAN_POINT('Ctrl Pts',(-1.97193697240645,1.,3.65230034717364));
#41732=CARTESIAN_POINT('Ctrl Pts',(-1.97236485439317,1.,3.66009578166865));
#41733=CARTESIAN_POINT('Ctrl Pts',(-1.9727589719863,1.,3.66790152751984));
#41734=CARTESIAN_POINT('Ctrl Pts',(-1.97311947678035,1.,3.67571738106175));
#41735=CARTESIAN_POINT('Ctrl Pts',(-1.97344650303631,1.,3.68354319913416));
#41736=CARTESIAN_POINT('Ctrl Pts',(-1.97374016224397,1.,3.69137888597855));
#41737=CARTESIAN_POINT('Ctrl Pts',(-1.97394846382289,1.,3.69765528558292));
#41738=CARTESIAN_POINT('Ctrl Pts',(-1.97408973726149,1.,3.70236698911837));
#41739=CARTESIAN_POINT('Ctrl Pts',(-1.974177276451,1.,3.7055100813194));
#41740=CARTESIAN_POINT('Ctrl Pts',(-1.97421938526992,1.,3.70708211654725));
#41741=CARTESIAN_POINT('Origin',(-1.97421938526992,0.,3.70708211654725));
#41742=CARTESIAN_POINT('',(-1.83867539237861,1.,3.77614523045147));
#41743=CARTESIAN_POINT('Origin',(0.,0.,0.));
#41744=CARTESIAN_POINT('',(-2.03660101169564,1.,3.14877060440425));
#41745=CARTESIAN_POINT('Origin',(0.,1.,0.));
#41746=CARTESIAN_POINT('Ctrl Pts',(-2.03660101169564,1.,3.14877060440425));
#41747=CARTESIAN_POINT('Ctrl Pts',(-2.03660101169564,0.666666666666667,
3.14877060440425));
#41748=CARTESIAN_POINT('Ctrl Pts',(-2.03660101169564,0.333333333333333,
3.14877060440425));
#41749=CARTESIAN_POINT('Ctrl Pts',(-2.03660101169564,-0.333333333333333,
3.14877060440425));
#41750=CARTESIAN_POINT('Ctrl Pts',(-2.03660101169564,-0.666666666666667,
3.14877060440425));
#41751=CARTESIAN_POINT('Ctrl Pts',(-2.03660101169564,-1.,3.14877060440425));
#41752=CARTESIAN_POINT('Ctrl Pts',(-2.40675750623143,-1.,3.44202241512147));
#41753=CARTESIAN_POINT('Ctrl Pts',(-2.40675750623143,1.,3.44202241512147));
#41754=CARTESIAN_POINT('Ctrl Pts',(-2.40537592959345,-1.,3.44127120683402));
#41755=CARTESIAN_POINT('Ctrl Pts',(-2.40537592959345,1.,3.44127120683402));
#41756=CARTESIAN_POINT('Ctrl Pts',(-2.40261515590099,-1.,3.43976627485223));
#41757=CARTESIAN_POINT('Ctrl Pts',(-2.40261515590099,1.,3.43976627485223));
#41758=CARTESIAN_POINT('Ctrl Pts',(-2.39848113411429,-1.,3.43750133066036));
#41759=CARTESIAN_POINT('Ctrl Pts',(-2.39848113411429,1.,3.43750133066036));
#41760=CARTESIAN_POINT('Ctrl Pts',(-2.39298338805823,-1.,3.43446630680436));
#41761=CARTESIAN_POINT('Ctrl Pts',(-2.39298338805823,1.,3.43446630680436));
#41762=CARTESIAN_POINT('Ctrl Pts',(-2.38613505844641,-1.,3.43064732714472));
#41763=CARTESIAN_POINT('Ctrl Pts',(-2.38613505844641,1.,3.43064732714472));
#41764=CARTESIAN_POINT('Ctrl Pts',(-2.37931067029517,-1.,3.42680309755241));
#41765=CARTESIAN_POINT('Ctrl Pts',(-2.37931067029517,1.,3.42680309755241));
#41766=CARTESIAN_POINT('Ctrl Pts',(-2.37251035954351,-1.,3.42293356216595));
#41767=CARTESIAN_POINT('Ctrl Pts',(-2.37251035954351,1.,3.42293356216595));
#41768=CARTESIAN_POINT('Ctrl Pts',(-2.36573431470314,-1.,3.41903866635384));
#41769=CARTESIAN_POINT('Ctrl Pts',(-2.36573431470314,1.,3.41903866635384));
#41770=CARTESIAN_POINT('Ctrl Pts',(-2.35898278606449,-1.,3.4151183675076));
#41771=CARTESIAN_POINT('Ctrl Pts',(-2.35898278606449,1.,3.4151183675076));
#41772=CARTESIAN_POINT('Ctrl Pts',(-2.35225606823649,-1.,3.41117262313464));
#41773=CARTESIAN_POINT('Ctrl Pts',(-2.35225606823649,1.,3.41117262313464));
#41774=CARTESIAN_POINT('Ctrl Pts',(-2.34555447648901,-1.,3.40720137403888));
#41775=CARTESIAN_POINT('Ctrl Pts',(-2.34555447648901,1.,3.40720137403888));
#41776=CARTESIAN_POINT('Ctrl Pts',(-2.33887832342715,-1.,3.40320452776646));
#41777=CARTESIAN_POINT('Ctrl Pts',(-2.33887832342715,1.,3.40320452776646));
#41778=CARTESIAN_POINT('Ctrl Pts',(-2.33222789882601,-1.,3.39918194578115));
#41779=CARTESIAN_POINT('Ctrl Pts',(-2.33222789882601,1.,3.39918194578115));
#41780=CARTESIAN_POINT('Ctrl Pts',(-2.32560343902683,-1.,3.39513342020045));
#41781=CARTESIAN_POINT('Ctrl Pts',(-2.32560343902683,1.,3.39513342020045));
#41782=CARTESIAN_POINT('Ctrl Pts',(-2.31900513925627,-1.,3.39105869475112));
#41783=CARTESIAN_POINT('Ctrl Pts',(-2.31900513925627,1.,3.39105869475112));
#41784=CARTESIAN_POINT('Ctrl Pts',(-2.31243319489505,-1.,3.38695751492659));
#41785=CARTESIAN_POINT('Ctrl Pts',(-2.31243319489505,1.,3.38695751492659));
#41786=CARTESIAN_POINT('Ctrl Pts',(-2.30588783640389,-1.,3.38282967336676));
#41787=CARTESIAN_POINT('Ctrl Pts',(-2.30588783640389,1.,3.38282967336676));
#41788=CARTESIAN_POINT('Ctrl Pts',(-2.29936936127588,-1.,3.37867504959382));
#41789=CARTESIAN_POINT('Ctrl Pts',(-2.29936936127588,1.,3.37867504959382));
#41790=CARTESIAN_POINT('Ctrl Pts',(-2.2928781800731,-1.,3.37449367172707));
#41791=CARTESIAN_POINT('Ctrl Pts',(-2.2928781800731,1.,3.37449367172707));
#41792=CARTESIAN_POINT('Ctrl Pts',(-2.28641481081045,-1.,3.37028570206357));
#41793=CARTESIAN_POINT('Ctrl Pts',(-2.28641481081045,1.,3.37028570206357));
#41794=CARTESIAN_POINT('Ctrl Pts',(-2.27997979457968,-1.,3.36605130712978));
#41795=CARTESIAN_POINT('Ctrl Pts',(-2.27997979457968,1.,3.36605130712978));
#41796=CARTESIAN_POINT('Ctrl Pts',(-2.27357362620902,-1.,3.36179055004369));
#41797=CARTESIAN_POINT('Ctrl Pts',(-2.27357362620902,1.,3.36179055004369));
#41798=CARTESIAN_POINT('Ctrl Pts',(-2.26719668579921,-1.,3.35750328523077));
#41799=CARTESIAN_POINT('Ctrl Pts',(-2.26719668579921,1.,3.35750328523077));
#41800=CARTESIAN_POINT('Ctrl Pts',(-2.26084915222484,-1.,3.35318902552676));
#41801=CARTESIAN_POINT('Ctrl Pts',(-2.26084915222484,1.,3.35318902552676));
#41802=CARTESIAN_POINT('Ctrl Pts',(-2.25453097693524,-1.,3.34884690292342));
#41803=CARTESIAN_POINT('Ctrl Pts',(-2.25453097693524,1.,3.34884690292342));
#41804=CARTESIAN_POINT('Ctrl Pts',(-2.24824207678288,-1.,3.34447596770768));
#41805=CARTESIAN_POINT('Ctrl Pts',(-2.24824207678288,1.,3.34447596770768));
#41806=CARTESIAN_POINT('Ctrl Pts',(-2.24198249391437,-1.,3.34007543738044));
#41807=CARTESIAN_POINT('Ctrl Pts',(-2.24198249391437,1.,3.34007543738044));
#41808=CARTESIAN_POINT('Ctrl Pts',(-2.2357525632881,-1.,3.33564495756478));
#41809=CARTESIAN_POINT('Ctrl Pts',(-2.2357525632881,1.,3.33564495756478));
#41810=CARTESIAN_POINT('Ctrl Pts',(-2.22955308907221,-1.,3.33118487773593));
#41811=CARTESIAN_POINT('Ctrl Pts',(-2.22955308907221,1.,3.33118487773593));
#41812=CARTESIAN_POINT('Ctrl Pts',(-2.22338548312758,-1.,3.32669646722871));
#41813=CARTESIAN_POINT('Ctrl Pts',(-2.22338548312758,1.,3.32669646722871));
#41814=CARTESIAN_POINT('Ctrl Pts',(-2.21725135110889,-1.,3.32218125618955));
#41815=CARTESIAN_POINT('Ctrl Pts',(-2.21725135110889,1.,3.32218125618955));
#41816=CARTESIAN_POINT('Ctrl Pts',(-2.21115211847872,-1.,3.31764044024231));
#41817=CARTESIAN_POINT('Ctrl Pts',(-2.21115211847872,1.,3.31764044024231));
#41818=CARTESIAN_POINT('Ctrl Pts',(-2.20508863150608,-1.,3.3130742460895));
#41819=CARTESIAN_POINT('Ctrl Pts',(-2.20508863150608,1.,3.3130742460895));
#41820=CARTESIAN_POINT('Ctrl Pts',(-2.19906078949924,-1.,3.30848134694596));
#41821=CARTESIAN_POINT('Ctrl Pts',(-2.19906078949924,1.,3.30848134694596));
#41822=CARTESIAN_POINT('Ctrl Pts',(-2.19306710376112,-1.,3.30385816281831));
#41823=CARTESIAN_POINT('Ctrl Pts',(-2.19306710376112,1.,3.30385816281831));
#41824=CARTESIAN_POINT('Ctrl Pts',(-2.18710556500325,-1.,3.29920022557635));
#41825=CARTESIAN_POINT('Ctrl Pts',(-2.18710556500325,1.,3.29920022557635));
#41826=CARTESIAN_POINT('Ctrl Pts',(-2.18117455557062,-1.,3.29450361500484));
#41827=CARTESIAN_POINT('Ctrl Pts',(-2.18117455557062,1.,3.29450361500484));
#41828=CARTESIAN_POINT('Ctrl Pts',(-2.17527380048422,-1.,3.28976645712566));
#41829=CARTESIAN_POINT('Ctrl Pts',(-2.17527380048422,1.,3.28976645712566));
#41830=CARTESIAN_POINT('Ctrl Pts',(-2.16940517773459,-1.,3.2849901997973));
#41831=CARTESIAN_POINT('Ctrl Pts',(-2.16940517773459,1.,3.2849901997973));
#41832=CARTESIAN_POINT('Ctrl Pts',(-2.16357391934434,-1.,3.28018150841414));
#41833=CARTESIAN_POINT('Ctrl Pts',(-2.16357391934434,1.,3.28018150841414));
#41834=CARTESIAN_POINT('Ctrl Pts',(-2.15778690038359,-1.,3.27534954469206));
#41835=CARTESIAN_POINT('Ctrl Pts',(-2.15778690038359,1.,3.27534954469206));
#41836=CARTESIAN_POINT('Ctrl Pts',(-2.15205043199818,-1.,3.27050245897244));
#41837=CARTESIAN_POINT('Ctrl Pts',(-2.15205043199818,1.,3.27050245897244));
#41838=CARTESIAN_POINT('Ctrl Pts',(-2.14636805295663,-1.,3.26564388189764));
#41839=CARTESIAN_POINT('Ctrl Pts',(-2.14636805295663,1.,3.26564388189764));
#41840=CARTESIAN_POINT('Ctrl Pts',(-2.14073870754257,-1.,3.26077002641868));
#41841=CARTESIAN_POINT('Ctrl Pts',(-2.14073870754257,1.,3.26077002641868));
#41842=CARTESIAN_POINT('Ctrl Pts',(-2.13515375878786,-1.,3.25586495065027));
#41843=CARTESIAN_POINT('Ctrl Pts',(-2.13515375878786,1.,3.25586495065027));
#41844=CARTESIAN_POINT('Ctrl Pts',(-2.1296002839681,-1.,3.25090574493994));
#41845=CARTESIAN_POINT('Ctrl Pts',(-2.1296002839681,1.,3.25090574493994));
#41846=CARTESIAN_POINT('Ctrl Pts',(-2.12406646410943,-1.,3.24587102613347));
#41847=CARTESIAN_POINT('Ctrl Pts',(-2.12406646410943,1.,3.24587102613347));
#41848=CARTESIAN_POINT('Ctrl Pts',(-2.11854673326972,-1.,3.24074905517282));
#41849=CARTESIAN_POINT('Ctrl Pts',(-2.11854673326972,1.,3.24074905517282));
#41850=CARTESIAN_POINT('Ctrl Pts',(-2.11304604021784,-1.,3.23554444767115));
#41851=CARTESIAN_POINT('Ctrl Pts',(-2.11304604021784,1.,3.23554444767115));
#41852=CARTESIAN_POINT('Ctrl Pts',(-2.1075869964248,-1.,3.23028945793334));
#41853=CARTESIAN_POINT('Ctrl Pts',(-2.1075869964248,1.,3.23028945793334));
#41854=CARTESIAN_POINT('Ctrl Pts',(-2.10220384298533,-1.,3.22503437553496));
#41855=CARTESIAN_POINT('Ctrl Pts',(-2.10220384298533,1.,3.22503437553496));
#41856=CARTESIAN_POINT('Ctrl Pts',(-2.09692958434933,-1.,3.21982707347067));
#41857=CARTESIAN_POINT('Ctrl Pts',(-2.09692958434933,1.,3.21982707347067));
#41858=CARTESIAN_POINT('Ctrl Pts',(-2.0917841946046,-1.,3.2146942960168));
#41859=CARTESIAN_POINT('Ctrl Pts',(-2.0917841946046,1.,3.2146942960168));
#41860=CARTESIAN_POINT('Ctrl Pts',(-2.08676465517435,-1.,3.20962575845433));
#41861=CARTESIAN_POINT('Ctrl Pts',(-2.08676465517435,1.,3.20962575845433));
#41862=CARTESIAN_POINT('Ctrl Pts',(-2.08182850370816,-1.,3.20454818630635));
#41863=CARTESIAN_POINT('Ctrl Pts',(-2.08182850370816,1.,3.20454818630635));
#41864=CARTESIAN_POINT('Ctrl Pts',(-2.0769044187063,-1.,3.19934132835879));
#41865=CARTESIAN_POINT('Ctrl Pts',(-2.0769044187063,1.,3.19934132835879));
#41866=CARTESIAN_POINT('Ctrl Pts',(-2.07192253497765,-1.,3.19388465568113));
#41867=CARTESIAN_POINT('Ctrl Pts',(-2.07192253497765,1.,3.19388465568113));
#41868=CARTESIAN_POINT('Ctrl Pts',(-2.06684062744065,-1.,3.18809755562297));
#41869=CARTESIAN_POINT('Ctrl Pts',(-2.06684062744065,1.,3.18809755562297));
#41870=CARTESIAN_POINT('Ctrl Pts',(-2.06166849827143,-1.,3.18197692964677));
#41871=CARTESIAN_POINT('Ctrl Pts',(-2.06166849827143,1.,3.18197692964677));
#41872=CARTESIAN_POINT('Ctrl Pts',(-2.05650186773279,-1.,3.17564906975592));
#41873=CARTESIAN_POINT('Ctrl Pts',(-2.05650186773279,1.,3.17564906975592));
#41874=CARTESIAN_POINT('Ctrl Pts',(-2.05151770247452,-1.,3.16936341689859));
#41875=CARTESIAN_POINT('Ctrl Pts',(-2.05151770247452,1.,3.16936341689859));
#41876=CARTESIAN_POINT('Ctrl Pts',(-2.0469333124766,-1.,3.16343165059235));
#41877=CARTESIAN_POINT('Ctrl Pts',(-2.0469333124766,1.,3.16343165059235));
#41878=CARTESIAN_POINT('Ctrl Pts',(-2.04297406404132,-1.,3.15817983946525));
#41879=CARTESIAN_POINT('Ctrl Pts',(-2.04297406404132,1.,3.15817983946525));
#41880=CARTESIAN_POINT('Ctrl Pts',(-2.03984073791432,-1.,3.1538999167466));
#41881=CARTESIAN_POINT('Ctrl Pts',(-2.03984073791432,1.,3.1538999167466));
#41882=CARTESIAN_POINT('Ctrl Pts',(-2.03766932526171,-1.,3.15079010635326));
#41883=CARTESIAN_POINT('Ctrl Pts',(-2.03766932526171,1.,3.15079010635326));
#41884=CARTESIAN_POINT('Ctrl Pts',(-2.03675273048882,-1.,3.14931281967585));
#41885=CARTESIAN_POINT('Ctrl Pts',(-2.03675273048882,1.,3.14931281967585));
#41886=CARTESIAN_POINT('Ctrl Pts',(-2.03653654935384,-1.,3.14878756590499));
#41887=CARTESIAN_POINT('Ctrl Pts',(-2.03653654935384,1.,3.14878756590499));
#41888=CARTESIAN_POINT('Ctrl Pts',(-2.036601737578,-1.,3.14869618937138));
#41889=CARTESIAN_POINT('Ctrl Pts',(-2.036601737578,1.,3.14869618937138));
#41890=CARTESIAN_POINT('Ctrl Pts',(-2.03668666247593,-1.,3.1487152044751));
#41891=CARTESIAN_POINT('Ctrl Pts',(-2.03668666247593,1.,3.1487152044751));
#41892=CARTESIAN_POINT('',(-2.40675750623143,1.,3.44202241512147));
#41893=CARTESIAN_POINT('Ctrl Pts',(-2.40675750623143,1.,3.44202241512147));
#41894=CARTESIAN_POINT('Ctrl Pts',(-2.40537592959345,1.,3.44127120683402));
#41895=CARTESIAN_POINT('Ctrl Pts',(-2.40261515590099,1.,3.43976627485223));
#41896=CARTESIAN_POINT('Ctrl Pts',(-2.39848113411429,1.,3.43750133066036));
#41897=CARTESIAN_POINT('Ctrl Pts',(-2.39298338805823,1.,3.43446630680436));
#41898=CARTESIAN_POINT('Ctrl Pts',(-2.38613505844641,1.,3.43064732714472));
#41899=CARTESIAN_POINT('Ctrl Pts',(-2.37931067029517,1.,3.42680309755241));
#41900=CARTESIAN_POINT('Ctrl Pts',(-2.37251035954351,1.,3.42293356216595));
#41901=CARTESIAN_POINT('Ctrl Pts',(-2.36573431470314,1.,3.41903866635384));
#41902=CARTESIAN_POINT('Ctrl Pts',(-2.35898278606449,1.,3.4151183675076));
#41903=CARTESIAN_POINT('Ctrl Pts',(-2.35225606823649,1.,3.41117262313464));
#41904=CARTESIAN_POINT('Ctrl Pts',(-2.34555447648901,1.,3.40720137403888));
#41905=CARTESIAN_POINT('Ctrl Pts',(-2.33887832342715,1.,3.40320452776646));
#41906=CARTESIAN_POINT('Ctrl Pts',(-2.33222789882601,1.,3.39918194578115));
#41907=CARTESIAN_POINT('Ctrl Pts',(-2.32560343902683,1.,3.39513342020045));
#41908=CARTESIAN_POINT('Ctrl Pts',(-2.31900513925627,1.,3.39105869475112));
#41909=CARTESIAN_POINT('Ctrl Pts',(-2.31243319489505,1.,3.38695751492659));
#41910=CARTESIAN_POINT('Ctrl Pts',(-2.30588783640389,1.,3.38282967336676));
#41911=CARTESIAN_POINT('Ctrl Pts',(-2.29936936127588,1.,3.37867504959382));
#41912=CARTESIAN_POINT('Ctrl Pts',(-2.2928781800731,1.,3.37449367172707));
#41913=CARTESIAN_POINT('Ctrl Pts',(-2.28641481081045,1.,3.37028570206357));
#41914=CARTESIAN_POINT('Ctrl Pts',(-2.27997979457968,1.,3.36605130712978));
#41915=CARTESIAN_POINT('Ctrl Pts',(-2.27357362620902,1.,3.36179055004369));
#41916=CARTESIAN_POINT('Ctrl Pts',(-2.26719668579921,1.,3.35750328523077));
#41917=CARTESIAN_POINT('Ctrl Pts',(-2.26084915222484,1.,3.35318902552676));
#41918=CARTESIAN_POINT('Ctrl Pts',(-2.25453097693524,1.,3.34884690292342));
#41919=CARTESIAN_POINT('Ctrl Pts',(-2.24824207678288,1.,3.34447596770768));
#41920=CARTESIAN_POINT('Ctrl Pts',(-2.24198249391437,1.,3.34007543738044));
#41921=CARTESIAN_POINT('Ctrl Pts',(-2.2357525632881,1.,3.33564495756478));
#41922=CARTESIAN_POINT('Ctrl Pts',(-2.22955308907221,1.,3.33118487773593));
#41923=CARTESIAN_POINT('Ctrl Pts',(-2.22338548312758,1.,3.32669646722871));
#41924=CARTESIAN_POINT('Ctrl Pts',(-2.21725135110889,1.,3.32218125618955));
#41925=CARTESIAN_POINT('Ctrl Pts',(-2.21115211847872,1.,3.31764044024231));
#41926=CARTESIAN_POINT('Ctrl Pts',(-2.20508863150608,1.,3.3130742460895));
#41927=CARTESIAN_POINT('Ctrl Pts',(-2.19906078949924,1.,3.30848134694596));
#41928=CARTESIAN_POINT('Ctrl Pts',(-2.19306710376112,1.,3.30385816281831));
#41929=CARTESIAN_POINT('Ctrl Pts',(-2.18710556500325,1.,3.29920022557635));
#41930=CARTESIAN_POINT('Ctrl Pts',(-2.18117455557062,1.,3.29450361500484));
#41931=CARTESIAN_POINT('Ctrl Pts',(-2.17527380048422,1.,3.28976645712566));
#41932=CARTESIAN_POINT('Ctrl Pts',(-2.16940517773459,1.,3.2849901997973));
#41933=CARTESIAN_POINT('Ctrl Pts',(-2.16357391934434,1.,3.28018150841414));
#41934=CARTESIAN_POINT('Ctrl Pts',(-2.15778690038359,1.,3.27534954469206));
#41935=CARTESIAN_POINT('Ctrl Pts',(-2.15205043199818,1.,3.27050245897244));
#41936=CARTESIAN_POINT('Ctrl Pts',(-2.14636805295663,1.,3.26564388189764));
#41937=CARTESIAN_POINT('Ctrl Pts',(-2.14073870754257,1.,3.26077002641868));
#41938=CARTESIAN_POINT('Ctrl Pts',(-2.13515375878786,1.,3.25586495065027));
#41939=CARTESIAN_POINT('Ctrl Pts',(-2.1296002839681,1.,3.25090574493994));
#41940=CARTESIAN_POINT('Ctrl Pts',(-2.12406646410943,1.,3.24587102613347));
#41941=CARTESIAN_POINT('Ctrl Pts',(-2.11854673326972,1.,3.24074905517282));
#41942=CARTESIAN_POINT('Ctrl Pts',(-2.11304604021784,1.,3.23554444767115));
#41943=CARTESIAN_POINT('Ctrl Pts',(-2.1075869964248,1.,3.23028945793334));
#41944=CARTESIAN_POINT('Ctrl Pts',(-2.10220384298533,1.,3.22503437553496));
#41945=CARTESIAN_POINT('Ctrl Pts',(-2.09692958434933,1.,3.21982707347067));
#41946=CARTESIAN_POINT('Ctrl Pts',(-2.0917841946046,1.,3.2146942960168));
#41947=CARTESIAN_POINT('Ctrl Pts',(-2.08676465517435,1.,3.20962575845433));
#41948=CARTESIAN_POINT('Ctrl Pts',(-2.08182850370816,1.,3.20454818630635));
#41949=CARTESIAN_POINT('Ctrl Pts',(-2.0769044187063,1.,3.19934132835879));
#41950=CARTESIAN_POINT('Ctrl Pts',(-2.07192253497765,1.,3.19388465568113));
#41951=CARTESIAN_POINT('Ctrl Pts',(-2.06684062744065,1.,3.18809755562297));
#41952=CARTESIAN_POINT('Ctrl Pts',(-2.06166849827143,1.,3.18197692964677));
#41953=CARTESIAN_POINT('Ctrl Pts',(-2.05650186773279,1.,3.17564906975592));
#41954=CARTESIAN_POINT('Ctrl Pts',(-2.05151770247452,1.,3.16936341689859));
#41955=CARTESIAN_POINT('Ctrl Pts',(-2.0469333124766,1.,3.16343165059235));
#41956=CARTESIAN_POINT('Ctrl Pts',(-2.04297406404132,1.,3.15817983946525));
#41957=CARTESIAN_POINT('Ctrl Pts',(-2.03984073791432,1.,3.1538999167466));
#41958=CARTESIAN_POINT('Ctrl Pts',(-2.03783225496023,1.,3.15102344775396));
#41959=CARTESIAN_POINT('Ctrl Pts',(-2.03693188810614,1.,3.14959882629936));
#41960=CARTESIAN_POINT('Ctrl Pts',(-2.03663974554941,1.,3.14901193669147));
#41961=CARTESIAN_POINT('Ctrl Pts',(-2.03659701539175,1.,3.1488193908823));
#41962=CARTESIAN_POINT('Ctrl Pts',(-2.03660101169564,1.,3.14877060440425));
#41963=CARTESIAN_POINT('',(-2.40675750623143,0.,3.44202241512147));
#41964=CARTESIAN_POINT('Ctrl Pts',(-2.36523532225181,-1.,2.91001063062876));
#41965=CARTESIAN_POINT('Ctrl Pts',(-2.36523532225181,1.,2.91001063062876));
#41966=CARTESIAN_POINT('Ctrl Pts',(-2.36524348105112,-1.,2.90992398626211));
#41967=CARTESIAN_POINT('Ctrl Pts',(-2.36524348105112,1.,2.90992398626211));
#41968=CARTESIAN_POINT('Ctrl Pts',(-2.36535052956938,-1.,2.90989022548032));
#41969=CARTESIAN_POINT('Ctrl Pts',(-2.36535052956938,1.,2.90989022548032));
#41970=CARTESIAN_POINT('Ctrl Pts',(-2.36578327194741,-1.,2.91025813830041));
#41971=CARTESIAN_POINT('Ctrl Pts',(-2.36578327194741,1.,2.91025813830041));
#41972=CARTESIAN_POINT('Ctrl Pts',(-2.36690501170627,-1.,2.9115863784204));
#41973=CARTESIAN_POINT('Ctrl Pts',(-2.36690501170627,1.,2.9115863784204));
#41974=CARTESIAN_POINT('Ctrl Pts',(-2.36919161373173,-1.,2.9146124988314));
#41975=CARTESIAN_POINT('Ctrl Pts',(-2.36919161373173,1.,2.9146124988314));
#41976=CARTESIAN_POINT('Ctrl Pts',(-2.37229381109821,-1.,2.91891503791411));
#41977=CARTESIAN_POINT('Ctrl Pts',(-2.37229381109821,1.,2.91891503791411));
#41978=CARTESIAN_POINT('Ctrl Pts',(-2.3760651052403,-1.,2.92430340582608));
#41979=CARTESIAN_POINT('Ctrl Pts',(-2.3760651052403,1.,2.92430340582608));
#41980=CARTESIAN_POINT('Ctrl Pts',(-2.38028989582073,-1.,2.93049643640206));
#41981=CARTESIAN_POINT('Ctrl Pts',(-2.38028989582073,1.,2.93049643640206));
#41982=CARTESIAN_POINT('Ctrl Pts',(-2.38472771516311,-1.,2.93717903280391));
#41983=CARTESIAN_POINT('Ctrl Pts',(-2.38472771516311,1.,2.93717903280391));
#41984=CARTESIAN_POINT('Ctrl Pts',(-2.38914929090759,-1.,2.94404820669076));
#41985=CARTESIAN_POINT('Ctrl Pts',(-2.38914929090759,1.,2.94404820669076));
#41986=CARTESIAN_POINT('Ctrl Pts',(-2.39337207631667,-1.,2.95085857128439));
#41987=CARTESIAN_POINT('Ctrl Pts',(-2.39337207631667,1.,2.95085857128439));
#41988=CARTESIAN_POINT('Ctrl Pts',(-2.39730553974517,-1.,2.95748006482942));
#41989=CARTESIAN_POINT('Ctrl Pts',(-2.39730553974517,1.,2.95748006482942));
#41990=CARTESIAN_POINT('Ctrl Pts',(-2.4009556571164,-1.,2.96390432240312));
#41991=CARTESIAN_POINT('Ctrl Pts',(-2.4009556571164,1.,2.96390432240312));
#41992=CARTESIAN_POINT('Ctrl Pts',(-2.40438604734919,-1.,2.9701964131236));
#41993=CARTESIAN_POINT('Ctrl Pts',(-2.40438604734919,1.,2.9701964131236));
#41994=CARTESIAN_POINT('Ctrl Pts',(-2.40768975073713,-1.,2.97646002822422));
#41995=CARTESIAN_POINT('Ctrl Pts',(-2.40768975073713,1.,2.97646002822422));
#41996=CARTESIAN_POINT('Ctrl Pts',(-2.41095909342571,-1.,2.98280015815107));
#41997=CARTESIAN_POINT('Ctrl Pts',(-2.41095909342571,1.,2.98280015815107));
#41998=CARTESIAN_POINT('Ctrl Pts',(-2.41425064199586,-1.,2.98927983005796));
#41999=CARTESIAN_POINT('Ctrl Pts',(-2.41425064199586,1.,2.98927983005796));
#42000=CARTESIAN_POINT('Ctrl Pts',(-2.41757324500514,-1.,2.99590509293503));
#42001=CARTESIAN_POINT('Ctrl Pts',(-2.41757324500514,1.,2.99590509293503));
#42002=CARTESIAN_POINT('Ctrl Pts',(-2.42090763946779,-1.,3.00264868585996));
#42003=CARTESIAN_POINT('Ctrl Pts',(-2.42090763946779,1.,3.00264868585996));
#42004=CARTESIAN_POINT('Ctrl Pts',(-2.42421849439613,-1.,3.00946442616658));
#42005=CARTESIAN_POINT('Ctrl Pts',(-2.42421849439613,1.,3.00946442616658));
#42006=CARTESIAN_POINT('Ctrl Pts',(-2.42746856264168,-1.,3.01630420830504));
#42007=CARTESIAN_POINT('Ctrl Pts',(-2.42746856264168,1.,3.01630420830504));
#42008=CARTESIAN_POINT('Ctrl Pts',(-2.43063415586637,-1.,3.02313656036004));
#42009=CARTESIAN_POINT('Ctrl Pts',(-2.43063415586637,1.,3.02313656036004));
#42010=CARTESIAN_POINT('Ctrl Pts',(-2.43371241361488,-1.,3.02995534946978));
#42011=CARTESIAN_POINT('Ctrl Pts',(-2.43371241361488,1.,3.02995534946978));
#42012=CARTESIAN_POINT('Ctrl Pts',(-2.43671278042414,-1.,3.03676949672821));
#42013=CARTESIAN_POINT('Ctrl Pts',(-2.43671278042414,1.,3.03676949672821));
#42014=CARTESIAN_POINT('Ctrl Pts',(-2.43965194061857,-1.,3.04359685040555));
#42015=CARTESIAN_POINT('Ctrl Pts',(-2.43965194061857,1.,3.04359685040555));
#42016=CARTESIAN_POINT('Ctrl Pts',(-2.44254768923105,-1.,3.05045678021504));
#42017=CARTESIAN_POINT('Ctrl Pts',(-2.44254768923105,1.,3.05045678021504));
#42018=CARTESIAN_POINT('Ctrl Pts',(-2.44541251892556,-1.,3.05736242671506));
#42019=CARTESIAN_POINT('Ctrl Pts',(-2.44541251892556,1.,3.05736242671506));
#42020=CARTESIAN_POINT('Ctrl Pts',(-2.44824970516544,-1.,3.06431596421405));
#42021=CARTESIAN_POINT('Ctrl Pts',(-2.44824970516544,1.,3.06431596421405));
#42022=CARTESIAN_POINT('Ctrl Pts',(-2.45105688854422,-1.,3.07131290521297));
#42023=CARTESIAN_POINT('Ctrl Pts',(-2.45105688854422,1.,3.07131290521297));
#42024=CARTESIAN_POINT('Ctrl Pts',(-2.4538282678779,-1.,3.07834472886139));
#42025=CARTESIAN_POINT('Ctrl Pts',(-2.4538282678779,1.,3.07834472886139));
#42026=CARTESIAN_POINT('Ctrl Pts',(-2.45655725437039,-1.,3.08540206545315));
#42027=CARTESIAN_POINT('Ctrl Pts',(-2.45655725437039,1.,3.08540206545315));
#42028=CARTESIAN_POINT('Ctrl Pts',(-2.4592391256388,-1.,3.09247787931887));
#42029=CARTESIAN_POINT('Ctrl Pts',(-2.4592391256388,1.,3.09247787931887));
#42030=CARTESIAN_POINT('Ctrl Pts',(-2.46187308501884,-1.,3.09956993697052));
#42031=CARTESIAN_POINT('Ctrl Pts',(-2.46187308501884,1.,3.09956993697052));
#42032=CARTESIAN_POINT('Ctrl Pts',(-2.46446082979646,-1.,3.1066790790198));
#42033=CARTESIAN_POINT('Ctrl Pts',(-2.46446082979646,1.,3.1066790790198));
#42034=CARTESIAN_POINT('Ctrl Pts',(-2.46700558843506,-1.,3.11380805536122));
#42035=CARTESIAN_POINT('Ctrl Pts',(-2.46700558843506,1.,3.11380805536122));
#42036=CARTESIAN_POINT('Ctrl Pts',(-2.46951098947469,-1.,3.12096015766983));
#42037=CARTESIAN_POINT('Ctrl Pts',(-2.46951098947469,1.,3.12096015766983));
#42038=CARTESIAN_POINT('Ctrl Pts',(-2.47197997765871,-1.,3.12813790805952));
#42039=CARTESIAN_POINT('Ctrl Pts',(-2.47197997765871,1.,3.12813790805952));
#42040=CARTESIAN_POINT('Ctrl Pts',(-2.47441378371932,-1.,3.13534181229295));
#42041=CARTESIAN_POINT('Ctrl Pts',(-2.47441378371932,1.,3.13534181229295));
#42042=CARTESIAN_POINT('Ctrl Pts',(-2.47681245356109,-1.,3.1425709954655));
#42043=CARTESIAN_POINT('Ctrl Pts',(-2.47681245356109,1.,3.1425709954655));
#42044=CARTESIAN_POINT('Ctrl Pts',(-2.47917529057029,-1.,3.14982373241352));
#42045=CARTESIAN_POINT('Ctrl Pts',(-2.47917529057029,1.,3.14982373241352));
#42046=CARTESIAN_POINT('Ctrl Pts',(-2.48150133566571,-1.,3.15709802322739));
#42047=CARTESIAN_POINT('Ctrl Pts',(-2.48150133566571,1.,3.15709802322739));
#42048=CARTESIAN_POINT('Ctrl Pts',(-2.48378981792725,-1.,3.16439213290161));
#42049=CARTESIAN_POINT('Ctrl Pts',(-2.48378981792725,1.,3.16439213290161));
#42050=CARTESIAN_POINT('Ctrl Pts',(-2.48604065348587,-1.,3.17170518863313));
#42051=CARTESIAN_POINT('Ctrl Pts',(-2.48604065348587,1.,3.17170518863313));
#42052=CARTESIAN_POINT('Ctrl Pts',(-2.48825428288201,-1.,3.17903698136622));
#42053=CARTESIAN_POINT('Ctrl Pts',(-2.48825428288201,1.,3.17903698136622));
#42054=CARTESIAN_POINT('Ctrl Pts',(-2.49043146334059,-1.,3.18638771282266));
#42055=CARTESIAN_POINT('Ctrl Pts',(-2.49043146334059,1.,3.18638771282266));
#42056=CARTESIAN_POINT('Ctrl Pts',(-2.49257307239848,-1.,3.19375775555798));
#42057=CARTESIAN_POINT('Ctrl Pts',(-2.49257307239848,1.,3.19375775555798));
#42058=CARTESIAN_POINT('Ctrl Pts',(-2.49467992057755,-1.,3.20114742397588));
#42059=CARTESIAN_POINT('Ctrl Pts',(-2.49467992057755,1.,3.20114742397588));
#42060=CARTESIAN_POINT('Ctrl Pts',(-2.4967525264737,-1.,3.20855669849836));
#42061=CARTESIAN_POINT('Ctrl Pts',(-2.4967525264737,1.,3.20855669849836));
#42062=CARTESIAN_POINT('Ctrl Pts',(-2.4987911459939,-1.,3.21598526261286));
#42063=CARTESIAN_POINT('Ctrl Pts',(-2.4987911459939,1.,3.21598526261286));
#42064=CARTESIAN_POINT('Ctrl Pts',(-2.50079587201957,-1.,3.22343262620503));
#42065=CARTESIAN_POINT('Ctrl Pts',(-2.50079587201957,1.,3.22343262620503));
#42066=CARTESIAN_POINT('Ctrl Pts',(-2.50276671338111,-1.,3.23089822320646));
#42067=CARTESIAN_POINT('Ctrl Pts',(-2.50276671338111,1.,3.23089822320646));
#42068=CARTESIAN_POINT('Ctrl Pts',(-2.5047036758003,-1.,3.23838151080319));
#42069=CARTESIAN_POINT('Ctrl Pts',(-2.5047036758003,1.,3.23838151080319));
#42070=CARTESIAN_POINT('Ctrl Pts',(-2.506606859405,-1.,3.24588208983849));
#42071=CARTESIAN_POINT('Ctrl Pts',(-2.506606859405,1.,3.24588208983849));
#42072=CARTESIAN_POINT('Ctrl Pts',(-2.50847647070723,-1.,3.25339971460982));
#42073=CARTESIAN_POINT('Ctrl Pts',(-2.50847647070723,1.,3.25339971460982));
#42074=CARTESIAN_POINT('Ctrl Pts',(-2.51031277813486,-1.,3.26093423001434));
#42075=CARTESIAN_POINT('Ctrl Pts',(-2.51031277813486,1.,3.26093423001434));
#42076=CARTESIAN_POINT('Ctrl Pts',(-2.51211608411423,-1.,3.26848552888115));
#42077=CARTESIAN_POINT('Ctrl Pts',(-2.51211608411423,1.,3.26848552888115));
#42078=CARTESIAN_POINT('Ctrl Pts',(-2.513886692704,-1.,3.27605350473142));
#42079=CARTESIAN_POINT('Ctrl Pts',(-2.513886692704,1.,3.27605350473142));
#42080=CARTESIAN_POINT('Ctrl Pts',(-2.51562487464514,-1.,3.28363799702982));
#42081=CARTESIAN_POINT('Ctrl Pts',(-2.51562487464514,1.,3.28363799702982));
#42082=CARTESIAN_POINT('Ctrl Pts',(-2.51733085123797,-1.,3.2912387729927));
#42083=CARTESIAN_POINT('Ctrl Pts',(-2.51733085123797,1.,3.2912387729927));
#42084=CARTESIAN_POINT('Ctrl Pts',(-2.51900480701069,-1.,3.29885556388352));
#42085=CARTESIAN_POINT('Ctrl Pts',(-2.51900480701069,1.,3.29885556388352));
#42086=CARTESIAN_POINT('Ctrl Pts',(-2.52064689568511,-1.,3.30648808815442));
#42087=CARTESIAN_POINT('Ctrl Pts',(-2.52064689568511,1.,3.30648808815442));
#42088=CARTESIAN_POINT('Ctrl Pts',(-2.52225724871313,-1.,3.31413607874645));
#42089=CARTESIAN_POINT('Ctrl Pts',(-2.52225724871313,1.,3.31413607874645));
#42090=CARTESIAN_POINT('Ctrl Pts',(-2.5238359839626,-1.,3.32179931078699));
#42091=CARTESIAN_POINT('Ctrl Pts',(-2.5238359839626,1.,3.32179931078699));
#42092=CARTESIAN_POINT('Ctrl Pts',(-2.52538321164634,-1.,3.32947762187533));
#42093=CARTESIAN_POINT('Ctrl Pts',(-2.52538321164634,1.,3.32947762187533));
#42094=CARTESIAN_POINT('Ctrl Pts',(-2.52689902690158,-1.,3.33717089999103));
#42095=CARTESIAN_POINT('Ctrl Pts',(-2.52689902690158,1.,3.33717089999103));
#42096=CARTESIAN_POINT('Ctrl Pts',(-2.52808660915689,-1.,3.34333744115511));
#42097=CARTESIAN_POINT('Ctrl Pts',(-2.52808660915689,1.,3.34333744115511));
#42098=CARTESIAN_POINT('Ctrl Pts',(-2.52896321610703,-1.,3.34796903576663));
#42099=CARTESIAN_POINT('Ctrl Pts',(-2.52896321610703,1.,3.34796903576663));
#42100=CARTESIAN_POINT('Ctrl Pts',(-2.5295413654909,-1.,3.35105973714071));
#42101=CARTESIAN_POINT('Ctrl Pts',(-2.5295413654909,1.,3.35105973714071));
#42102=CARTESIAN_POINT('Ctrl Pts',(-2.52982887637028,-1.,3.35260583073571));
#42103=CARTESIAN_POINT('Ctrl Pts',(-2.52982887637028,1.,3.35260583073571));
#42104=CARTESIAN_POINT('',(-2.36531447826073,1.,2.90994629141676));
#42105=CARTESIAN_POINT('Ctrl Pts',(-2.36531447826073,-1.,2.90994629141676));
#42106=CARTESIAN_POINT('Ctrl Pts',(-2.36531447826073,-0.666666666666667,
2.90994629141676));
#42107=CARTESIAN_POINT('Ctrl Pts',(-2.36531447826073,-0.333333333333333,
2.90994629141676));
#42108=CARTESIAN_POINT('Ctrl Pts',(-2.36531447826073,0.333333333333333,
2.90994629141676));
#42109=CARTESIAN_POINT('Ctrl Pts',(-2.36531447826073,0.666666666666667,
2.90994629141676));
#42110=CARTESIAN_POINT('Ctrl Pts',(-2.36531447826073,1.,2.90994629141676));
#42111=CARTESIAN_POINT('',(-2.52982887637028,1.,3.35260583073571));
#42112=CARTESIAN_POINT('',(-2.52982887637028,0.,3.35260583073571));
#42113=CARTESIAN_POINT('Ctrl Pts',(-2.36531447826073,1.,2.90994629141676));
#42114=CARTESIAN_POINT('Ctrl Pts',(-2.36536211188453,1.,2.90995756655606));
#42115=CARTESIAN_POINT('Ctrl Pts',(-2.36553202948613,1.,2.91005770527719));
#42116=CARTESIAN_POINT('Ctrl Pts',(-2.36599991765749,1.,2.91051690822156));
#42117=CARTESIAN_POINT('Ctrl Pts',(-2.36707658451664,1.,2.91181344022549));
#42118=CARTESIAN_POINT('Ctrl Pts',(-2.36919161373173,1.,2.9146124988314));
#42119=CARTESIAN_POINT('Ctrl Pts',(-2.37229381109821,1.,2.91891503791411));
#42120=CARTESIAN_POINT('Ctrl Pts',(-2.3760651052403,1.,2.92430340582608));
#42121=CARTESIAN_POINT('Ctrl Pts',(-2.38028989582073,1.,2.93049643640206));
#42122=CARTESIAN_POINT('Ctrl Pts',(-2.38472771516311,1.,2.93717903280391));
#42123=CARTESIAN_POINT('Ctrl Pts',(-2.38914929090759,1.,2.94404820669076));
#42124=CARTESIAN_POINT('Ctrl Pts',(-2.39337207631667,1.,2.95085857128439));
#42125=CARTESIAN_POINT('Ctrl Pts',(-2.39730553974517,1.,2.95748006482942));
#42126=CARTESIAN_POINT('Ctrl Pts',(-2.4009556571164,1.,2.96390432240312));
#42127=CARTESIAN_POINT('Ctrl Pts',(-2.40438604734919,1.,2.9701964131236));
#42128=CARTESIAN_POINT('Ctrl Pts',(-2.40768975073713,1.,2.97646002822422));
#42129=CARTESIAN_POINT('Ctrl Pts',(-2.41095909342571,1.,2.98280015815107));
#42130=CARTESIAN_POINT('Ctrl Pts',(-2.41425064199586,1.,2.98927983005796));
#42131=CARTESIAN_POINT('Ctrl Pts',(-2.41757324500514,1.,2.99590509293503));
#42132=CARTESIAN_POINT('Ctrl Pts',(-2.42090763946779,1.,3.00264868585996));
#42133=CARTESIAN_POINT('Ctrl Pts',(-2.42421849439613,1.,3.00946442616658));
#42134=CARTESIAN_POINT('Ctrl Pts',(-2.42746856264168,1.,3.01630420830504));
#42135=CARTESIAN_POINT('Ctrl Pts',(-2.43063415586637,1.,3.02313656036004));
#42136=CARTESIAN_POINT('Ctrl Pts',(-2.43371241361488,1.,3.02995534946978));
#42137=CARTESIAN_POINT('Ctrl Pts',(-2.43671278042414,1.,3.03676949672821));
#42138=CARTESIAN_POINT('Ctrl Pts',(-2.43965194061857,1.,3.04359685040555));
#42139=CARTESIAN_POINT('Ctrl Pts',(-2.44254768923105,1.,3.05045678021504));
#42140=CARTESIAN_POINT('Ctrl Pts',(-2.44541251892556,1.,3.05736242671506));
#42141=CARTESIAN_POINT('Ctrl Pts',(-2.44824970516544,1.,3.06431596421405));
#42142=CARTESIAN_POINT('Ctrl Pts',(-2.45105688854422,1.,3.07131290521297));
#42143=CARTESIAN_POINT('Ctrl Pts',(-2.4538282678779,1.,3.07834472886139));
#42144=CARTESIAN_POINT('Ctrl Pts',(-2.45655725437039,1.,3.08540206545315));
#42145=CARTESIAN_POINT('Ctrl Pts',(-2.4592391256388,1.,3.09247787931887));
#42146=CARTESIAN_POINT('Ctrl Pts',(-2.46187308501884,1.,3.09956993697052));
#42147=CARTESIAN_POINT('Ctrl Pts',(-2.46446082979646,1.,3.1066790790198));
#42148=CARTESIAN_POINT('Ctrl Pts',(-2.46700558843506,1.,3.11380805536122));
#42149=CARTESIAN_POINT('Ctrl Pts',(-2.46951098947469,1.,3.12096015766983));
#42150=CARTESIAN_POINT('Ctrl Pts',(-2.47197997765871,1.,3.12813790805952));
#42151=CARTESIAN_POINT('Ctrl Pts',(-2.47441378371932,1.,3.13534181229295));
#42152=CARTESIAN_POINT('Ctrl Pts',(-2.47681245356109,1.,3.1425709954655));
#42153=CARTESIAN_POINT('Ctrl Pts',(-2.47917529057029,1.,3.14982373241352));
#42154=CARTESIAN_POINT('Ctrl Pts',(-2.48150133566571,1.,3.15709802322739));
#42155=CARTESIAN_POINT('Ctrl Pts',(-2.48378981792725,1.,3.16439213290161));
#42156=CARTESIAN_POINT('Ctrl Pts',(-2.48604065348587,1.,3.17170518863313));
#42157=CARTESIAN_POINT('Ctrl Pts',(-2.48825428288201,1.,3.17903698136622));
#42158=CARTESIAN_POINT('Ctrl Pts',(-2.49043146334059,1.,3.18638771282266));
#42159=CARTESIAN_POINT('Ctrl Pts',(-2.49257307239848,1.,3.19375775555798));
#42160=CARTESIAN_POINT('Ctrl Pts',(-2.49467992057755,1.,3.20114742397588));
#42161=CARTESIAN_POINT('Ctrl Pts',(-2.4967525264737,1.,3.20855669849836));
#42162=CARTESIAN_POINT('Ctrl Pts',(-2.4987911459939,1.,3.21598526261286));
#42163=CARTESIAN_POINT('Ctrl Pts',(-2.50079587201957,1.,3.22343262620503));
#42164=CARTESIAN_POINT('Ctrl Pts',(-2.50276671338111,1.,3.23089822320646));
#42165=CARTESIAN_POINT('Ctrl Pts',(-2.5047036758003,1.,3.23838151080319));
#42166=CARTESIAN_POINT('Ctrl Pts',(-2.506606859405,1.,3.24588208983849));
#42167=CARTESIAN_POINT('Ctrl Pts',(-2.50847647070723,1.,3.25339971460982));
#42168=CARTESIAN_POINT('Ctrl Pts',(-2.51031277813486,1.,3.26093423001434));
#42169=CARTESIAN_POINT('Ctrl Pts',(-2.51211608411423,1.,3.26848552888115));
#42170=CARTESIAN_POINT('Ctrl Pts',(-2.513886692704,1.,3.27605350473142));
#42171=CARTESIAN_POINT('Ctrl Pts',(-2.51562487464514,1.,3.28363799702982));
#42172=CARTESIAN_POINT('Ctrl Pts',(-2.51733085123797,1.,3.2912387729927));
#42173=CARTESIAN_POINT('Ctrl Pts',(-2.51900480701069,1.,3.29885556388352));
#42174=CARTESIAN_POINT('Ctrl Pts',(-2.52064689568511,1.,3.30648808815442));
#42175=CARTESIAN_POINT('Ctrl Pts',(-2.52225724871313,1.,3.31413607874645));
#42176=CARTESIAN_POINT('Ctrl Pts',(-2.5238359839626,1.,3.32179931078699));
#42177=CARTESIAN_POINT('Ctrl Pts',(-2.52538321164634,1.,3.32947762187533));
#42178=CARTESIAN_POINT('Ctrl Pts',(-2.52689902690158,1.,3.33717089999103));
#42179=CARTESIAN_POINT('Ctrl Pts',(-2.52808660915689,1.,3.34333744115511));
#42180=CARTESIAN_POINT('Ctrl Pts',(-2.52896321610703,1.,3.34796903576663));
#42181=CARTESIAN_POINT('Ctrl Pts',(-2.5295413654909,1.,3.35105973714071));
#42182=CARTESIAN_POINT('Ctrl Pts',(-2.52982887637028,1.,3.35260583073571));
#42183=CARTESIAN_POINT('Origin',(-2.52982887637028,0.,3.35260583073571));
#42184=CARTESIAN_POINT('',(-2.40675750623143,1.,3.44202241512147));
#42185=CARTESIAN_POINT('Origin',(0.,0.,0.));
#42186=CARTESIAN_POINT('',(-2.50410331873042,1.,2.79140942341378));
#42187=CARTESIAN_POINT('Origin',(0.,1.,0.));
#42188=CARTESIAN_POINT('Ctrl Pts',(-2.50410331873042,1.,2.79140942341378));
#42189=CARTESIAN_POINT('Ctrl Pts',(-2.50410331873042,0.666666666666667,
2.79140942341378));
#42190=CARTESIAN_POINT('Ctrl Pts',(-2.50410331873043,0.333333333333333,
2.79140942341378));
#42191=CARTESIAN_POINT('Ctrl Pts',(-2.50410331873043,-0.333333333333333,
2.79140942341378));
#42192=CARTESIAN_POINT('Ctrl Pts',(-2.50410331873043,-0.666666666666667,
2.79140942341378));
#42193=CARTESIAN_POINT('Ctrl Pts',(-2.50410331873043,-1.,2.79140942341378));
#42194=CARTESIAN_POINT('Ctrl Pts',(-2.91557726271063,-1.,3.02314558451372));
#42195=CARTESIAN_POINT('Ctrl Pts',(-2.91557726271063,1.,3.02314558451372));
#42196=CARTESIAN_POINT('Ctrl Pts',(-2.91409518070707,-1.,3.02261975104912));
#42197=CARTESIAN_POINT('Ctrl Pts',(-2.91409518070707,1.,3.02261975104912));
#42198=CARTESIAN_POINT('Ctrl Pts',(-2.91113297349052,-1.,3.02156522743299));
#42199=CARTESIAN_POINT('Ctrl Pts',(-2.91113297349052,1.,3.02156522743299));
#42200=CARTESIAN_POINT('Ctrl Pts',(-2.90669553303902,-1.,3.01997487194926));
#42201=CARTESIAN_POINT('Ctrl Pts',(-2.90669553303902,1.,3.01997487194926));
#42202=CARTESIAN_POINT('Ctrl Pts',(-2.90079069102661,-1.,3.01783725123646));
#42203=CARTESIAN_POINT('Ctrl Pts',(-2.90079069102661,1.,3.01783725123646));
#42204=CARTESIAN_POINT('Ctrl Pts',(-2.8934292556764,-1.,3.01513660433291));
#42205=CARTESIAN_POINT('Ctrl Pts',(-2.8934292556764,1.,3.01513660433291));
#42206=CARTESIAN_POINT('Ctrl Pts',(-2.88608751706796,-1.,3.01240727309568));
#42207=CARTESIAN_POINT('Ctrl Pts',(-2.88608751706796,1.,3.01240727309568));
#42208=CARTESIAN_POINT('Ctrl Pts',(-2.87876560072799,-1.,3.0096491810855));
#42209=CARTESIAN_POINT('Ctrl Pts',(-2.87876560072799,1.,3.0096491810855));
#42210=CARTESIAN_POINT('Ctrl Pts',(-2.87146368430104,-1.,3.00686224485374));
#42211=CARTESIAN_POINT('Ctrl Pts',(-2.87146368430104,1.,3.00686224485374));
#42212=CARTESIAN_POINT('Ctrl Pts',(-2.86418200833065,-1.,3.00404638316245));
#42213=CARTESIAN_POINT('Ctrl Pts',(-2.86418200833065,1.,3.00404638316245));
#42214=CARTESIAN_POINT('Ctrl Pts',(-2.85692085715129,-1.,3.0012015079552));
#42215=CARTESIAN_POINT('Ctrl Pts',(-2.85692085715129,1.,3.0012015079552));
#42216=CARTESIAN_POINT('Ctrl Pts',(-2.84968053289104,-1.,2.99832751144566));
#42217=CARTESIAN_POINT('Ctrl Pts',(-2.84968053289104,1.,2.99832751144566));
#42218=CARTESIAN_POINT('Ctrl Pts',(-2.84246132984334,-1.,2.995424253416));
#42219=CARTESIAN_POINT('Ctrl Pts',(-2.84246132984334,1.,2.995424253416));
#42220=CARTESIAN_POINT('Ctrl Pts',(-2.83526351254383,-1.,2.99249155170479));
#42221=CARTESIAN_POINT('Ctrl Pts',(-2.83526351254383,1.,2.99249155170479));
#42222=CARTESIAN_POINT('Ctrl Pts',(-2.82808728190402,-1.,2.98952916401699));
#42223=CARTESIAN_POINT('Ctrl Pts',(-2.82808728190402,1.,2.98952916401699));
#42224=CARTESIAN_POINT('Ctrl Pts',(-2.82093279065704,-1.,2.98653680669434));
#42225=CARTESIAN_POINT('Ctrl Pts',(-2.82093279065704,1.,2.98653680669434));
#42226=CARTESIAN_POINT('Ctrl Pts',(-2.81380019196454,-1.,2.9835141977994));
#42227=CARTESIAN_POINT('Ctrl Pts',(-2.81380019196454,1.,2.9835141977994));
#42228=CARTESIAN_POINT('Ctrl Pts',(-2.80668968101162,-1.,2.98046109647299));
#42229=CARTESIAN_POINT('Ctrl Pts',(-2.80668968101162,1.,2.98046109647299));
#42230=CARTESIAN_POINT('Ctrl Pts',(-2.79960153278186,-1.,2.97737733718242));
#42231=CARTESIAN_POINT('Ctrl Pts',(-2.79960153278186,1.,2.97737733718242));
#42232=CARTESIAN_POINT('Ctrl Pts',(-2.79253615718147,-1.,2.97426288347475));
#42233=CARTESIAN_POINT('Ctrl Pts',(-2.79253615718147,1.,2.97426288347475));
#42234=CARTESIAN_POINT('Ctrl Pts',(-2.78549409123657,-1.,2.97111781461349));
#42235=CARTESIAN_POINT('Ctrl Pts',(-2.78549409123657,1.,2.97111781461349));
#42236=CARTESIAN_POINT('Ctrl Pts',(-2.77847589542767,-1.,2.9679422104295));
#42237=CARTESIAN_POINT('Ctrl Pts',(-2.77847589542767,1.,2.9679422104295));
#42238=CARTESIAN_POINT('Ctrl Pts',(-2.77148206836464,-1.,2.96473605585548));
#42239=CARTESIAN_POINT('Ctrl Pts',(-2.77148206836464,1.,2.96473605585548));
#42240=CARTESIAN_POINT('Ctrl Pts',(-2.76451296269571,-1.,2.96149914764832));
#42241=CARTESIAN_POINT('Ctrl Pts',(-2.76451296269571,1.,2.96149914764832));
#42242=CARTESIAN_POINT('Ctrl Pts',(-2.75756867888393,-1.,2.9582309766594));
#42243=CARTESIAN_POINT('Ctrl Pts',(-2.75756867888393,1.,2.9582309766594));
#42244=CARTESIAN_POINT('Ctrl Pts',(-2.75064903318996,-1.,2.95493069316211));
#42245=CARTESIAN_POINT('Ctrl Pts',(-2.75064903318996,1.,2.95493069316211));
#42246=CARTESIAN_POINT('Ctrl Pts',(-2.7437537949221,-1.,2.95159737214305));
#42247=CARTESIAN_POINT('Ctrl Pts',(-2.7437537949221,1.,2.95159737214305));
#42248=CARTESIAN_POINT('Ctrl Pts',(-2.73688288329825,-1.,2.94823023414381));
#42249=CARTESIAN_POINT('Ctrl Pts',(-2.73688288329825,1.,2.94823023414381));
#42250=CARTESIAN_POINT('Ctrl Pts',(-2.73003657371613,-1.,2.94482887675139));
#42251=CARTESIAN_POINT('Ctrl Pts',(-2.73003657371613,1.,2.94482887675139));
#42252=CARTESIAN_POINT('Ctrl Pts',(-2.72321571511322,-1.,2.94139351933882));
#42253=CARTESIAN_POINT('Ctrl Pts',(-2.72321571511322,1.,2.94139351933882));
#42254=CARTESIAN_POINT('Ctrl Pts',(-2.71642190053575,-1.,2.93792519474955));
#42255=CARTESIAN_POINT('Ctrl Pts',(-2.71642190053575,1.,2.93792519474955));
#42256=CARTESIAN_POINT('Ctrl Pts',(-2.70965695523776,-1.,2.93442516311168));
#42257=CARTESIAN_POINT('Ctrl Pts',(-2.70965695523776,1.,2.93442516311168));
#42258=CARTESIAN_POINT('Ctrl Pts',(-2.70292247416881,-1.,2.93089438233746));
#42259=CARTESIAN_POINT('Ctrl Pts',(-2.70292247416881,1.,2.93089438233746));
#42260=CARTESIAN_POINT('Ctrl Pts',(-2.69621932864302,-1.,2.92733294395268));
#42261=CARTESIAN_POINT('Ctrl Pts',(-2.69621932864302,1.,2.92733294395268));
#42262=CARTESIAN_POINT('Ctrl Pts',(-2.68954721165342,-1.,2.92373955325876));
#42263=CARTESIAN_POINT('Ctrl Pts',(-2.68954721165342,1.,2.92373955325876));
#42264=CARTESIAN_POINT('Ctrl Pts',(-2.68290409279689,-1.,2.92011090722152));
#42265=CARTESIAN_POINT('Ctrl Pts',(-2.68290409279689,1.,2.92011090722152));
#42266=CARTESIAN_POINT('Ctrl Pts',(-2.67628728855309,-1.,2.91644290704281));
#42267=CARTESIAN_POINT('Ctrl Pts',(-2.67628728855309,1.,2.91644290704281));
#42268=CARTESIAN_POINT('Ctrl Pts',(-2.66969458792627,-1.,2.91273193382876));
#42269=CARTESIAN_POINT('Ctrl Pts',(-2.66969458792627,1.,2.91273193382876));
#42270=CARTESIAN_POINT('Ctrl Pts',(-2.66312542616809,-1.,2.90897617968921));
#42271=CARTESIAN_POINT('Ctrl Pts',(-2.66312542616809,1.,2.90897617968921));
#42272=CARTESIAN_POINT('Ctrl Pts',(-2.65658188464287,-1.,2.90517678087467));
#42273=CARTESIAN_POINT('Ctrl Pts',(-2.65658188464287,1.,2.90517678087467));
#42274=CARTESIAN_POINT('Ctrl Pts',(-2.65007017365576,-1.,2.90133950224879));
#42275=CARTESIAN_POINT('Ctrl Pts',(-2.65007017365576,1.,2.90133950224879));
#42276=CARTESIAN_POINT('Ctrl Pts',(-2.64359851684146,-1.,2.89747231723361));
#42277=CARTESIAN_POINT('Ctrl Pts',(-2.64359851684146,1.,2.89747231723361));
#42278=CARTESIAN_POINT('Ctrl Pts',(-2.63717442263944,-1.,2.89358228854557));
#42279=CARTESIAN_POINT('Ctrl Pts',(-2.63717442263944,1.,2.89358228854557));
#42280=CARTESIAN_POINT('Ctrl Pts',(-2.63080195420771,-1.,2.88967244854243));
#42281=CARTESIAN_POINT('Ctrl Pts',(-2.63080195420771,1.,2.88967244854243));
#42282=CARTESIAN_POINT('Ctrl Pts',(-2.62447947640253,-1.,2.88573922195049));
#42283=CARTESIAN_POINT('Ctrl Pts',(-2.62447947640253,1.,2.88573922195049));
#42284=CARTESIAN_POINT('Ctrl Pts',(-2.61819596473087,-1.,2.88176821427502));
#42285=CARTESIAN_POINT('Ctrl Pts',(-2.61819596473087,1.,2.88176821427502));
#42286=CARTESIAN_POINT('Ctrl Pts',(-2.61193507170928,-1.,2.87773881947885));
#42287=CARTESIAN_POINT('Ctrl Pts',(-2.61193507170928,1.,2.87773881947885));
#42288=CARTESIAN_POINT('Ctrl Pts',(-2.6056817788128,-1.,2.87363176656475));
#42289=CARTESIAN_POINT('Ctrl Pts',(-2.6056817788128,1.,2.87363176656475));
#42290=CARTESIAN_POINT('Ctrl Pts',(-2.59942875223202,-1.,2.86943633170712));
#42291=CARTESIAN_POINT('Ctrl Pts',(-2.59942875223202,1.,2.86943633170712));
#42292=CARTESIAN_POINT('Ctrl Pts',(-2.59318160184921,-1.,2.86515629953528));
#42293=CARTESIAN_POINT('Ctrl Pts',(-2.59318160184921,1.,2.86515629953528));
#42294=CARTESIAN_POINT('Ctrl Pts',(-2.5869677064356,-1.,2.86081999003668));
#42295=CARTESIAN_POINT('Ctrl Pts',(-2.5869677064356,1.,2.86081999003668));
#42296=CARTESIAN_POINT('Ctrl Pts',(-2.58082875254407,-1.,2.85647171715147));
#42297=CARTESIAN_POINT('Ctrl Pts',(-2.58082875254407,1.,2.85647171715147));
#42298=CARTESIAN_POINT('Ctrl Pts',(-2.57480482727128,-1.,2.85215360144483));
#42299=CARTESIAN_POINT('Ctrl Pts',(-2.57480482727128,1.,2.85215360144483));
#42300=CARTESIAN_POINT('Ctrl Pts',(-2.56891984251743,-1.,2.84788893329091));
#42301=CARTESIAN_POINT('Ctrl Pts',(-2.56891984251743,1.,2.84788893329091));
#42302=CARTESIAN_POINT('Ctrl Pts',(-2.56316920798489,-1.,2.84366802680211));
#42303=CARTESIAN_POINT('Ctrl Pts',(-2.56316920798489,1.,2.84366802680211));
#42304=CARTESIAN_POINT('Ctrl Pts',(-2.55749952145165,-1.,2.83942515220699));
#42305=CARTESIAN_POINT('Ctrl Pts',(-2.55749952145165,1.,2.83942515220699));
#42306=CARTESIAN_POINT('Ctrl Pts',(-2.55182152806964,-1.,2.83505269592412));
#42307=CARTESIAN_POINT('Ctrl Pts',(-2.55182152806964,1.,2.83505269592412));
#42308=CARTESIAN_POINT('Ctrl Pts',(-2.54604736792542,-1.,2.83044254225794));
#42309=CARTESIAN_POINT('Ctrl Pts',(-2.54604736792542,1.,2.83044254225794));
#42310=CARTESIAN_POINT('Ctrl Pts',(-2.54012272520141,-1.,2.82552167649157));
#42311=CARTESIAN_POINT('Ctrl Pts',(-2.54012272520141,1.,2.82552167649157));
#42312=CARTESIAN_POINT('Ctrl Pts',(-2.53405679667463,-1.,2.82028550483744));
#42313=CARTESIAN_POINT('Ctrl Pts',(-2.53405679667463,1.,2.82028550483744));
#42314=CARTESIAN_POINT('Ctrl Pts',(-2.52796388055457,-1.,2.8148437904867));
#42315=CARTESIAN_POINT('Ctrl Pts',(-2.52796388055457,1.,2.8148437904867));
#42316=CARTESIAN_POINT('Ctrl Pts',(-2.52205778589922,-1.,2.80941521967234));
#42317=CARTESIAN_POINT('Ctrl Pts',(-2.52205778589922,1.,2.80941521967234));
#42318=CARTESIAN_POINT('Ctrl Pts',(-2.51660190466067,-1.,2.80427363984939));
#42319=CARTESIAN_POINT('Ctrl Pts',(-2.51660190466067,1.,2.80427363984939));
#42320=CARTESIAN_POINT('Ctrl Pts',(-2.51186983687947,-1.,2.79970585014308));
#42321=CARTESIAN_POINT('Ctrl Pts',(-2.51186983687947,1.,2.79970585014308));
#42322=CARTESIAN_POINT('Ctrl Pts',(-2.50810555977564,-1.,2.7959687805717));
#42323=CARTESIAN_POINT('Ctrl Pts',(-2.50810555977564,1.,2.7959687805717));
#42324=CARTESIAN_POINT('Ctrl Pts',(-2.50547439929077,-1.,2.79323694088143));
#42325=CARTESIAN_POINT('Ctrl Pts',(-2.50547439929077,1.,2.79323694088143));
#42326=CARTESIAN_POINT('Ctrl Pts',(-2.50433799076945,-1.,2.79192122906739));
#42327=CARTESIAN_POINT('Ctrl Pts',(-2.50433799076945,1.,2.79192122906739));
#42328=CARTESIAN_POINT('Ctrl Pts',(-2.50404230339032,-1.,2.79143626022225));
#42329=CARTESIAN_POINT('Ctrl Pts',(-2.50404230339032,1.,2.79143626022225));
#42330=CARTESIAN_POINT('Ctrl Pts',(-2.50409239460011,-1.,2.79133581100044));
#42331=CARTESIAN_POINT('Ctrl Pts',(-2.50409239460011,1.,2.79133581100044));
#42332=CARTESIAN_POINT('Ctrl Pts',(-2.50417924854921,-1.,2.79134130681569));
#42333=CARTESIAN_POINT('Ctrl Pts',(-2.50417924854921,1.,2.79134130681569));
#42334=CARTESIAN_POINT('',(-2.91557726271063,1.,3.02314558451372));
#42335=CARTESIAN_POINT('Ctrl Pts',(-2.91557726271063,1.,3.02314558451372));
#42336=CARTESIAN_POINT('Ctrl Pts',(-2.91409518070707,1.,3.02261975104912));
#42337=CARTESIAN_POINT('Ctrl Pts',(-2.91113297349052,1.,3.02156522743299));
#42338=CARTESIAN_POINT('Ctrl Pts',(-2.90669553303902,1.,3.01997487194926));
#42339=CARTESIAN_POINT('Ctrl Pts',(-2.90079069102661,1.,3.01783725123646));
#42340=CARTESIAN_POINT('Ctrl Pts',(-2.8934292556764,1.,3.01513660433291));
#42341=CARTESIAN_POINT('Ctrl Pts',(-2.88608751706796,1.,3.01240727309568));
#42342=CARTESIAN_POINT('Ctrl Pts',(-2.87876560072799,1.,3.0096491810855));
#42343=CARTESIAN_POINT('Ctrl Pts',(-2.87146368430104,1.,3.00686224485374));
#42344=CARTESIAN_POINT('Ctrl Pts',(-2.86418200833065,1.,3.00404638316245));
#42345=CARTESIAN_POINT('Ctrl Pts',(-2.85692085715129,1.,3.0012015079552));
#42346=CARTESIAN_POINT('Ctrl Pts',(-2.84968053289104,1.,2.99832751144566));
#42347=CARTESIAN_POINT('Ctrl Pts',(-2.84246132984334,1.,2.995424253416));
#42348=CARTESIAN_POINT('Ctrl Pts',(-2.83526351254383,1.,2.99249155170479));
#42349=CARTESIAN_POINT('Ctrl Pts',(-2.82808728190402,1.,2.98952916401699));
#42350=CARTESIAN_POINT('Ctrl Pts',(-2.82093279065704,1.,2.98653680669434));
#42351=CARTESIAN_POINT('Ctrl Pts',(-2.81380019196454,1.,2.9835141977994));
#42352=CARTESIAN_POINT('Ctrl Pts',(-2.80668968101162,1.,2.98046109647299));
#42353=CARTESIAN_POINT('Ctrl Pts',(-2.79960153278186,1.,2.97737733718242));
#42354=CARTESIAN_POINT('Ctrl Pts',(-2.79253615718147,1.,2.97426288347475));
#42355=CARTESIAN_POINT('Ctrl Pts',(-2.78549409123657,1.,2.97111781461349));
#42356=CARTESIAN_POINT('Ctrl Pts',(-2.77847589542767,1.,2.9679422104295));
#42357=CARTESIAN_POINT('Ctrl Pts',(-2.77148206836464,1.,2.96473605585548));
#42358=CARTESIAN_POINT('Ctrl Pts',(-2.76451296269571,1.,2.96149914764832));
#42359=CARTESIAN_POINT('Ctrl Pts',(-2.75756867888393,1.,2.9582309766594));
#42360=CARTESIAN_POINT('Ctrl Pts',(-2.75064903318996,1.,2.95493069316211));
#42361=CARTESIAN_POINT('Ctrl Pts',(-2.7437537949221,1.,2.95159737214305));
#42362=CARTESIAN_POINT('Ctrl Pts',(-2.73688288329825,1.,2.94823023414381));
#42363=CARTESIAN_POINT('Ctrl Pts',(-2.73003657371613,1.,2.94482887675139));
#42364=CARTESIAN_POINT('Ctrl Pts',(-2.72321571511322,1.,2.94139351933882));
#42365=CARTESIAN_POINT('Ctrl Pts',(-2.71642190053575,1.,2.93792519474955));
#42366=CARTESIAN_POINT('Ctrl Pts',(-2.70965695523776,1.,2.93442516311168));
#42367=CARTESIAN_POINT('Ctrl Pts',(-2.70292247416881,1.,2.93089438233746));
#42368=CARTESIAN_POINT('Ctrl Pts',(-2.69621932864302,1.,2.92733294395268));
#42369=CARTESIAN_POINT('Ctrl Pts',(-2.68954721165342,1.,2.92373955325876));
#42370=CARTESIAN_POINT('Ctrl Pts',(-2.68290409279689,1.,2.92011090722152));
#42371=CARTESIAN_POINT('Ctrl Pts',(-2.67628728855309,1.,2.91644290704281));
#42372=CARTESIAN_POINT('Ctrl Pts',(-2.66969458792627,1.,2.91273193382876));
#42373=CARTESIAN_POINT('Ctrl Pts',(-2.66312542616809,1.,2.90897617968921));
#42374=CARTESIAN_POINT('Ctrl Pts',(-2.65658188464287,1.,2.90517678087467));
#42375=CARTESIAN_POINT('Ctrl Pts',(-2.65007017365576,1.,2.90133950224879));
#42376=CARTESIAN_POINT('Ctrl Pts',(-2.64359851684146,1.,2.89747231723361));
#42377=CARTESIAN_POINT('Ctrl Pts',(-2.63717442263944,1.,2.89358228854557));
#42378=CARTESIAN_POINT('Ctrl Pts',(-2.63080195420771,1.,2.88967244854243));
#42379=CARTESIAN_POINT('Ctrl Pts',(-2.62447947640253,1.,2.88573922195049));
#42380=CARTESIAN_POINT('Ctrl Pts',(-2.61819596473087,1.,2.88176821427502));
#42381=CARTESIAN_POINT('Ctrl Pts',(-2.61193507170928,1.,2.87773881947885));
#42382=CARTESIAN_POINT('Ctrl Pts',(-2.6056817788128,1.,2.87363176656475));
#42383=CARTESIAN_POINT('Ctrl Pts',(-2.59942875223202,1.,2.86943633170712));
#42384=CARTESIAN_POINT('Ctrl Pts',(-2.59318160184921,1.,2.86515629953528));
#42385=CARTESIAN_POINT('Ctrl Pts',(-2.5869677064356,1.,2.86081999003668));
#42386=CARTESIAN_POINT('Ctrl Pts',(-2.58082875254407,1.,2.85647171715147));
#42387=CARTESIAN_POINT('Ctrl Pts',(-2.57480482727128,1.,2.85215360144483));
#42388=CARTESIAN_POINT('Ctrl Pts',(-2.56891984251743,1.,2.84788893329091));
#42389=CARTESIAN_POINT('Ctrl Pts',(-2.56316920798489,1.,2.84366802680211));
#42390=CARTESIAN_POINT('Ctrl Pts',(-2.55749952145165,1.,2.83942515220699));
#42391=CARTESIAN_POINT('Ctrl Pts',(-2.55182152806964,1.,2.83505269592412));
#42392=CARTESIAN_POINT('Ctrl Pts',(-2.54604736792542,1.,2.83044254225794));
#42393=CARTESIAN_POINT('Ctrl Pts',(-2.54012272520141,1.,2.82552167649157));
#42394=CARTESIAN_POINT('Ctrl Pts',(-2.53405679667463,1.,2.82028550483744));
#42395=CARTESIAN_POINT('Ctrl Pts',(-2.52796388055457,1.,2.8148437904867));
#42396=CARTESIAN_POINT('Ctrl Pts',(-2.52205778589922,1.,2.80941521967234));
#42397=CARTESIAN_POINT('Ctrl Pts',(-2.51660190466067,1.,2.80427363984939));
#42398=CARTESIAN_POINT('Ctrl Pts',(-2.51186983687947,1.,2.79970585014308));
#42399=CARTESIAN_POINT('Ctrl Pts',(-2.50810555977564,1.,2.7959687805717));
#42400=CARTESIAN_POINT('Ctrl Pts',(-2.50567182569153,1.,2.79344192164204));
#42401=CARTESIAN_POINT('Ctrl Pts',(-2.50455968395235,1.,2.79217568804874));
#42402=CARTESIAN_POINT('Ctrl Pts',(-2.50417932839343,1.,2.79164172519039));
#42403=CARTESIAN_POINT('Ctrl Pts',(-2.50410700351427,1.,2.79145823440899));
#42404=CARTESIAN_POINT('Ctrl Pts',(-2.50410331873043,1.,2.79140942341378));
#42405=CARTESIAN_POINT('',(-2.91557726271063,0.,3.02314558451372));
#42406=CARTESIAN_POINT('Ctrl Pts',(-2.79134130681569,-1.,2.50417924854921));
#42407=CARTESIAN_POINT('Ctrl Pts',(-2.79134130681569,1.,2.50417924854921));
#42408=CARTESIAN_POINT('Ctrl Pts',(-2.7913358110015,-1.,2.50409239460108));
#42409=CARTESIAN_POINT('Ctrl Pts',(-2.7913358110015,1.,2.50409239460108));
#42410=CARTESIAN_POINT('Ctrl Pts',(-2.79143626022503,-1.,2.50404230339286));
#42411=CARTESIAN_POINT('Ctrl Pts',(-2.79143626022503,1.,2.50404230339286));
#42412=CARTESIAN_POINT('Ctrl Pts',(-2.79192122907148,-1.,2.5043379907732));
#42413=CARTESIAN_POINT('Ctrl Pts',(-2.79192122907148,1.,2.5043379907732));
#42414=CARTESIAN_POINT('Ctrl Pts',(-2.7932369408851,-1.,2.50547439929414));
#42415=CARTESIAN_POINT('Ctrl Pts',(-2.7932369408851,1.,2.50547439929414));
#42416=CARTESIAN_POINT('Ctrl Pts',(-2.79596878057287,-1.,2.50810555977671));
#42417=CARTESIAN_POINT('Ctrl Pts',(-2.79596878057287,1.,2.50810555977671));
#42418=CARTESIAN_POINT('Ctrl Pts',(-2.79970585014168,-1.,2.51186983687818));
#42419=CARTESIAN_POINT('Ctrl Pts',(-2.79970585014168,1.,2.51186983687818));
#42420=CARTESIAN_POINT('Ctrl Pts',(-2.80427363984653,-1.,2.51660190465805));
#42421=CARTESIAN_POINT('Ctrl Pts',(-2.80427363984653,1.,2.51660190465805));
#42422=CARTESIAN_POINT('Ctrl Pts',(-2.80941521966941,-1.,2.52205778589653));
#42423=CARTESIAN_POINT('Ctrl Pts',(-2.80941521966941,1.,2.52205778589653));
#42424=CARTESIAN_POINT('Ctrl Pts',(-2.81484379048475,-1.,2.52796388055278));
#42425=CARTESIAN_POINT('Ctrl Pts',(-2.81484379048475,1.,2.52796388055278));
#42426=CARTESIAN_POINT('Ctrl Pts',(-2.82028550483689,-1.,2.53405679667412));
#42427=CARTESIAN_POINT('Ctrl Pts',(-2.82028550483689,1.,2.53405679667412));
#42428=CARTESIAN_POINT('Ctrl Pts',(-2.8255216764922,-1.,2.54012272520199));
#42429=CARTESIAN_POINT('Ctrl Pts',(-2.8255216764922,1.,2.54012272520199));
#42430=CARTESIAN_POINT('Ctrl Pts',(-2.83044254225917,-1.,2.54604736792655));
#42431=CARTESIAN_POINT('Ctrl Pts',(-2.83044254225917,1.,2.54604736792655));
#42432=CARTESIAN_POINT('Ctrl Pts',(-2.83505269592536,-1.,2.55182152807077));
#42433=CARTESIAN_POINT('Ctrl Pts',(-2.83505269592536,1.,2.55182152807077));
#42434=CARTESIAN_POINT('Ctrl Pts',(-2.83942515220782,-1.,2.55749952145241));
#42435=CARTESIAN_POINT('Ctrl Pts',(-2.83942515220782,1.,2.55749952145241));
#42436=CARTESIAN_POINT('Ctrl Pts',(-2.84366802680237,-1.,2.56316920798513));
#42437=CARTESIAN_POINT('Ctrl Pts',(-2.84366802680237,1.,2.56316920798513));
#42438=CARTESIAN_POINT('Ctrl Pts',(-2.84788893329067,-1.,2.56891984251721));
#42439=CARTESIAN_POINT('Ctrl Pts',(-2.84788893329067,1.,2.56891984251721));
#42440=CARTESIAN_POINT('Ctrl Pts',(-2.85215360144431,-1.,2.57480482727081));
#42441=CARTESIAN_POINT('Ctrl Pts',(-2.85215360144431,1.,2.57480482727081));
#42442=CARTESIAN_POINT('Ctrl Pts',(-2.85647171715092,-1.,2.58082875254357));
#42443=CARTESIAN_POINT('Ctrl Pts',(-2.85647171715092,1.,2.58082875254357));
#42444=CARTESIAN_POINT('Ctrl Pts',(-2.86081999003629,-1.,2.58696770643524));
#42445=CARTESIAN_POINT('Ctrl Pts',(-2.86081999003629,1.,2.58696770643524));
#42446=CARTESIAN_POINT('Ctrl Pts',(-2.86515629953513,-1.,2.59318160184908));
#42447=CARTESIAN_POINT('Ctrl Pts',(-2.86515629953513,1.,2.59318160184908));
#42448=CARTESIAN_POINT('Ctrl Pts',(-2.86943633170722,-1.,2.5994287522321));
#42449=CARTESIAN_POINT('Ctrl Pts',(-2.86943633170722,1.,2.5994287522321));
#42450=CARTESIAN_POINT('Ctrl Pts',(-2.87363176656501,-1.,2.60568177881303));
#42451=CARTESIAN_POINT('Ctrl Pts',(-2.87363176656501,1.,2.60568177881303));
#42452=CARTESIAN_POINT('Ctrl Pts',(-2.87773881947916,-1.,2.61193507170955));
#42453=CARTESIAN_POINT('Ctrl Pts',(-2.87773881947916,1.,2.61193507170955));
#42454=CARTESIAN_POINT('Ctrl Pts',(-2.88176821427525,-1.,2.61819596473108));
#42455=CARTESIAN_POINT('Ctrl Pts',(-2.88176821427525,1.,2.61819596473108));
#42456=CARTESIAN_POINT('Ctrl Pts',(-2.88573922195059,-1.,2.62447947640262));
#42457=CARTESIAN_POINT('Ctrl Pts',(-2.88573922195059,1.,2.62447947640262));
#42458=CARTESIAN_POINT('Ctrl Pts',(-2.88967244854239,-1.,2.63080195420767));
#42459=CARTESIAN_POINT('Ctrl Pts',(-2.88967244854239,1.,2.63080195420767));
#42460=CARTESIAN_POINT('Ctrl Pts',(-2.89358228854544,-1.,2.63717442263932));
#42461=CARTESIAN_POINT('Ctrl Pts',(-2.89358228854544,1.,2.63717442263932));
#42462=CARTESIAN_POINT('Ctrl Pts',(-2.89747231723345,-1.,2.64359851684131));
#42463=CARTESIAN_POINT('Ctrl Pts',(-2.89747231723345,1.,2.64359851684131));
#42464=CARTESIAN_POINT('Ctrl Pts',(-2.90133950224867,-1.,2.65007017365564));
#42465=CARTESIAN_POINT('Ctrl Pts',(-2.90133950224867,1.,2.65007017365564));
#42466=CARTESIAN_POINT('Ctrl Pts',(-2.90517678087461,-1.,2.65658188464282));
#42467=CARTESIAN_POINT('Ctrl Pts',(-2.90517678087461,1.,2.65658188464282));
#42468=CARTESIAN_POINT('Ctrl Pts',(-2.90897617968923,-1.,2.6631254261681));
#42469=CARTESIAN_POINT('Ctrl Pts',(-2.90897617968923,1.,2.6631254261681));
#42470=CARTESIAN_POINT('Ctrl Pts',(-2.91273193382882,-1.,2.66969458792631));
#42471=CARTESIAN_POINT('Ctrl Pts',(-2.91273193382882,1.,2.66969458792631));
#42472=CARTESIAN_POINT('Ctrl Pts',(-2.91644290704285,-1.,2.67628728855312));
#42473=CARTESIAN_POINT('Ctrl Pts',(-2.91644290704285,1.,2.67628728855312));
#42474=CARTESIAN_POINT('Ctrl Pts',(-2.92011090722152,-1.,2.68290409279688));
#42475=CARTESIAN_POINT('Ctrl Pts',(-2.92011090722152,1.,2.68290409279688));
#42476=CARTESIAN_POINT('Ctrl Pts',(-2.92373955325875,-1.,2.68954721165339));
#42477=CARTESIAN_POINT('Ctrl Pts',(-2.92373955325875,1.,2.68954721165339));
#42478=CARTESIAN_POINT('Ctrl Pts',(-2.92733294395267,-1.,2.69621932864301));
#42479=CARTESIAN_POINT('Ctrl Pts',(-2.92733294395267,1.,2.69621932864301));
#42480=CARTESIAN_POINT('Ctrl Pts',(-2.9308943823375,-1.,2.70292247416885));
#42481=CARTESIAN_POINT('Ctrl Pts',(-2.9308943823375,1.,2.70292247416885));
#42482=CARTESIAN_POINT('Ctrl Pts',(-2.93442516311179,-1.,2.70965695523787));
#42483=CARTESIAN_POINT('Ctrl Pts',(-2.93442516311179,1.,2.70965695523787));
#42484=CARTESIAN_POINT('Ctrl Pts',(-2.93792519474972,-1.,2.71642190053592));
#42485=CARTESIAN_POINT('Ctrl Pts',(-2.93792519474972,1.,2.71642190053592));
#42486=CARTESIAN_POINT('Ctrl Pts',(-2.94139351933897,-1.,2.72321571511337));
#42487=CARTESIAN_POINT('Ctrl Pts',(-2.94139351933897,1.,2.72321571511337));
#42488=CARTESIAN_POINT('Ctrl Pts',(-2.94482887675143,-1.,2.73003657371617));
#42489=CARTESIAN_POINT('Ctrl Pts',(-2.94482887675143,1.,2.73003657371617));
#42490=CARTESIAN_POINT('Ctrl Pts',(-2.94823023414364,-1.,2.73688288329808));
#42491=CARTESIAN_POINT('Ctrl Pts',(-2.94823023414364,1.,2.73688288329808));
#42492=CARTESIAN_POINT('Ctrl Pts',(-2.95159737214266,-1.,2.74375379492172));
#42493=CARTESIAN_POINT('Ctrl Pts',(-2.95159737214266,1.,2.74375379492172));
#42494=CARTESIAN_POINT('Ctrl Pts',(-2.95493069316161,-1.,2.75064903318947));
#42495=CARTESIAN_POINT('Ctrl Pts',(-2.95493069316161,1.,2.75064903318947));
#42496=CARTESIAN_POINT('Ctrl Pts',(-2.95823097665896,-1.,2.7575686788835));
#42497=CARTESIAN_POINT('Ctrl Pts',(-2.95823097665896,1.,2.7575686788835));
#42498=CARTESIAN_POINT('Ctrl Pts',(-2.96149914764818,-1.,2.76451296269557));
#42499=CARTESIAN_POINT('Ctrl Pts',(-2.96149914764818,1.,2.76451296269557));
#42500=CARTESIAN_POINT('Ctrl Pts',(-2.96473605585583,-1.,2.77148206836498));
#42501=CARTESIAN_POINT('Ctrl Pts',(-2.96473605585583,1.,2.77148206836498));
#42502=CARTESIAN_POINT('Ctrl Pts',(-2.96794221043036,-1.,2.7784758954285));
#42503=CARTESIAN_POINT('Ctrl Pts',(-2.96794221043036,1.,2.7784758954285));
#42504=CARTESIAN_POINT('Ctrl Pts',(-2.97111781461465,-1.,2.78549409123769));
#42505=CARTESIAN_POINT('Ctrl Pts',(-2.97111781461465,1.,2.78549409123769));
#42506=CARTESIAN_POINT('Ctrl Pts',(-2.9742628834758,-1.,2.79253615718248));
#42507=CARTESIAN_POINT('Ctrl Pts',(-2.9742628834758,1.,2.79253615718248));
#42508=CARTESIAN_POINT('Ctrl Pts',(-2.97737733718287,-1.,2.7996015327823));
#42509=CARTESIAN_POINT('Ctrl Pts',(-2.97737733718287,1.,2.7996015327823));
#42510=CARTESIAN_POINT('Ctrl Pts',(-2.98046109647241,-1.,2.80668968101106));
#42511=CARTESIAN_POINT('Ctrl Pts',(-2.98046109647241,1.,2.80668968101106));
#42512=CARTESIAN_POINT('Ctrl Pts',(-2.98351419779767,-1.,2.81380019196286));
#42513=CARTESIAN_POINT('Ctrl Pts',(-2.98351419779767,1.,2.81380019196286));
#42514=CARTESIAN_POINT('Ctrl Pts',(-2.9865368066918,-1.,2.82093279065457));
#42515=CARTESIAN_POINT('Ctrl Pts',(-2.9865368066918,1.,2.82093279065457));
#42516=CARTESIAN_POINT('Ctrl Pts',(-2.98952916401446,-1.,2.82808728190157));
#42517=CARTESIAN_POINT('Ctrl Pts',(-2.98952916401446,1.,2.82808728190157));
#42518=CARTESIAN_POINT('Ctrl Pts',(-2.9924915517034,-1.,2.83526351254248));
#42519=CARTESIAN_POINT('Ctrl Pts',(-2.9924915517034,1.,2.83526351254248));
#42520=CARTESIAN_POINT('Ctrl Pts',(-2.99542425341685,-1.,2.84246132984415));
#42521=CARTESIAN_POINT('Ctrl Pts',(-2.99542425341685,1.,2.84246132984415));
#42522=CARTESIAN_POINT('Ctrl Pts',(-2.99832751144925,-1.,2.84968053289451));
#42523=CARTESIAN_POINT('Ctrl Pts',(-2.99832751144925,1.,2.84968053289451));
#42524=CARTESIAN_POINT('Ctrl Pts',(-3.00120150796095,-1.,2.85692085715686));
#42525=CARTESIAN_POINT('Ctrl Pts',(-3.00120150796095,1.,2.85692085715686));
#42526=CARTESIAN_POINT('Ctrl Pts',(-3.00404638316867,-1.,2.86418200833667));
#42527=CARTESIAN_POINT('Ctrl Pts',(-3.00404638316867,1.,2.86418200833667));
#42528=CARTESIAN_POINT('Ctrl Pts',(-3.00686224485784,-1.,2.87146368430502));
#42529=CARTESIAN_POINT('Ctrl Pts',(-3.00686224485784,1.,2.87146368430502));
#42530=CARTESIAN_POINT('Ctrl Pts',(-3.00964918108476,-1.,2.87876560072727));
#42531=CARTESIAN_POINT('Ctrl Pts',(-3.00964918108476,1.,2.87876560072727));
#42532=CARTESIAN_POINT('Ctrl Pts',(-3.01240727308829,-1.,2.8860875170608));
#42533=CARTESIAN_POINT('Ctrl Pts',(-3.01240727308829,1.,2.8860875170608));
#42534=CARTESIAN_POINT('Ctrl Pts',(-3.01513660431928,-1.,2.89342925566321));
#42535=CARTESIAN_POINT('Ctrl Pts',(-3.01513660431928,1.,2.89342925566321));
#42536=CARTESIAN_POINT('Ctrl Pts',(-3.01783725121981,-1.,2.9007906910105));
#42537=CARTESIAN_POINT('Ctrl Pts',(-3.01783725121981,1.,2.9007906910105));
#42538=CARTESIAN_POINT('Ctrl Pts',(-3.01997487193503,-1.,2.90669553302526));
#42539=CARTESIAN_POINT('Ctrl Pts',(-3.01997487193503,1.,2.90669553302526));
#42540=CARTESIAN_POINT('Ctrl Pts',(-3.02156522742431,-1.,2.91113297348212));
#42541=CARTESIAN_POINT('Ctrl Pts',(-3.02156522742431,1.,2.91113297348212));
#42542=CARTESIAN_POINT('Ctrl Pts',(-3.02261975104593,-1.,2.91409518070399));
#42543=CARTESIAN_POINT('Ctrl Pts',(-3.02261975104593,1.,2.91409518070399));
#42544=CARTESIAN_POINT('Ctrl Pts',(-3.02314558451372,-1.,2.91557726271063));
#42545=CARTESIAN_POINT('Ctrl Pts',(-3.02314558451372,1.,2.91557726271063));
#42546=CARTESIAN_POINT('',(-2.79140942341258,1.,2.50410331873176));
#42547=CARTESIAN_POINT('Ctrl Pts',(-2.79140942341258,-1.,2.50410331873176));
#42548=CARTESIAN_POINT('Ctrl Pts',(-2.79140942341258,-0.666666666666667,
2.50410331873176));
#42549=CARTESIAN_POINT('Ctrl Pts',(-2.79140942341258,-0.333333333333333,
2.50410331873176));
#42550=CARTESIAN_POINT('Ctrl Pts',(-2.79140942341258,0.333333333333333,
2.50410331873176));
#42551=CARTESIAN_POINT('Ctrl Pts',(-2.79140942341258,0.666666666666667,
2.50410331873176));
#42552=CARTESIAN_POINT('Ctrl Pts',(-2.79140942341258,1.,2.50410331873176));
#42553=CARTESIAN_POINT('',(-3.02314558451372,1.,2.91557726271063));
#42554=CARTESIAN_POINT('',(-3.02314558451372,0.,2.91557726271063));
#42555=CARTESIAN_POINT('Ctrl Pts',(-2.79140942341258,1.,2.50410331873176));
#42556=CARTESIAN_POINT('Ctrl Pts',(-2.79145823440781,1.,2.50410700351493));
#42557=CARTESIAN_POINT('Ctrl Pts',(-2.79164172518905,1.,2.50417932839313));
#42558=CARTESIAN_POINT('Ctrl Pts',(-2.79217568804755,1.,2.50455968395146));
#42559=CARTESIAN_POINT('Ctrl Pts',(-2.79344192164147,1.,2.50567182569081));
#42560=CARTESIAN_POINT('Ctrl Pts',(-2.79596878057287,1.,2.50810555977671));
#42561=CARTESIAN_POINT('Ctrl Pts',(-2.79970585014168,1.,2.51186983687818));
#42562=CARTESIAN_POINT('Ctrl Pts',(-2.80427363984653,1.,2.51660190465805));
#42563=CARTESIAN_POINT('Ctrl Pts',(-2.80941521966941,1.,2.52205778589653));
#42564=CARTESIAN_POINT('Ctrl Pts',(-2.81484379048475,1.,2.52796388055278));
#42565=CARTESIAN_POINT('Ctrl Pts',(-2.82028550483689,1.,2.53405679667412));
#42566=CARTESIAN_POINT('Ctrl Pts',(-2.8255216764922,1.,2.54012272520199));
#42567=CARTESIAN_POINT('Ctrl Pts',(-2.83044254225917,1.,2.54604736792655));
#42568=CARTESIAN_POINT('Ctrl Pts',(-2.83505269592536,1.,2.55182152807077));
#42569=CARTESIAN_POINT('Ctrl Pts',(-2.83942515220782,1.,2.55749952145241));
#42570=CARTESIAN_POINT('Ctrl Pts',(-2.84366802680237,1.,2.56316920798513));
#42571=CARTESIAN_POINT('Ctrl Pts',(-2.84788893329067,1.,2.56891984251721));
#42572=CARTESIAN_POINT('Ctrl Pts',(-2.85215360144431,1.,2.57480482727081));
#42573=CARTESIAN_POINT('Ctrl Pts',(-2.85647171715092,1.,2.58082875254357));
#42574=CARTESIAN_POINT('Ctrl Pts',(-2.86081999003629,1.,2.58696770643524));
#42575=CARTESIAN_POINT('Ctrl Pts',(-2.86515629953513,1.,2.59318160184908));
#42576=CARTESIAN_POINT('Ctrl Pts',(-2.86943633170722,1.,2.5994287522321));
#42577=CARTESIAN_POINT('Ctrl Pts',(-2.87363176656501,1.,2.60568177881303));
#42578=CARTESIAN_POINT('Ctrl Pts',(-2.87773881947916,1.,2.61193507170955));
#42579=CARTESIAN_POINT('Ctrl Pts',(-2.88176821427525,1.,2.61819596473108));
#42580=CARTESIAN_POINT('Ctrl Pts',(-2.88573922195059,1.,2.62447947640262));
#42581=CARTESIAN_POINT('Ctrl Pts',(-2.88967244854239,1.,2.63080195420767));
#42582=CARTESIAN_POINT('Ctrl Pts',(-2.89358228854544,1.,2.63717442263932));
#42583=CARTESIAN_POINT('Ctrl Pts',(-2.89747231723345,1.,2.64359851684131));
#42584=CARTESIAN_POINT('Ctrl Pts',(-2.90133950224867,1.,2.65007017365564));
#42585=CARTESIAN_POINT('Ctrl Pts',(-2.90517678087461,1.,2.65658188464282));
#42586=CARTESIAN_POINT('Ctrl Pts',(-2.90897617968923,1.,2.6631254261681));
#42587=CARTESIAN_POINT('Ctrl Pts',(-2.91273193382882,1.,2.66969458792631));
#42588=CARTESIAN_POINT('Ctrl Pts',(-2.91644290704285,1.,2.67628728855312));
#42589=CARTESIAN_POINT('Ctrl Pts',(-2.92011090722152,1.,2.68290409279688));
#42590=CARTESIAN_POINT('Ctrl Pts',(-2.92373955325875,1.,2.68954721165339));
#42591=CARTESIAN_POINT('Ctrl Pts',(-2.92733294395267,1.,2.69621932864301));
#42592=CARTESIAN_POINT('Ctrl Pts',(-2.9308943823375,1.,2.70292247416885));
#42593=CARTESIAN_POINT('Ctrl Pts',(-2.93442516311179,1.,2.70965695523787));
#42594=CARTESIAN_POINT('Ctrl Pts',(-2.93792519474972,1.,2.71642190053592));
#42595=CARTESIAN_POINT('Ctrl Pts',(-2.94139351933897,1.,2.72321571511337));
#42596=CARTESIAN_POINT('Ctrl Pts',(-2.94482887675143,1.,2.73003657371617));
#42597=CARTESIAN_POINT('Ctrl Pts',(-2.94823023414364,1.,2.73688288329808));
#42598=CARTESIAN_POINT('Ctrl Pts',(-2.95159737214266,1.,2.74375379492172));
#42599=CARTESIAN_POINT('Ctrl Pts',(-2.95493069316161,1.,2.75064903318947));
#42600=CARTESIAN_POINT('Ctrl Pts',(-2.95823097665896,1.,2.7575686788835));
#42601=CARTESIAN_POINT('Ctrl Pts',(-2.96149914764818,1.,2.76451296269557));
#42602=CARTESIAN_POINT('Ctrl Pts',(-2.96473605585583,1.,2.77148206836498));
#42603=CARTESIAN_POINT('Ctrl Pts',(-2.96794221043036,1.,2.7784758954285));
#42604=CARTESIAN_POINT('Ctrl Pts',(-2.97111781461465,1.,2.78549409123769));
#42605=CARTESIAN_POINT('Ctrl Pts',(-2.9742628834758,1.,2.79253615718248));
#42606=CARTESIAN_POINT('Ctrl Pts',(-2.97737733718287,1.,2.7996015327823));
#42607=CARTESIAN_POINT('Ctrl Pts',(-2.98046109647241,1.,2.80668968101106));
#42608=CARTESIAN_POINT('Ctrl Pts',(-2.98351419779767,1.,2.81380019196286));
#42609=CARTESIAN_POINT('Ctrl Pts',(-2.9865368066918,1.,2.82093279065457));
#42610=CARTESIAN_POINT('Ctrl Pts',(-2.98952916401446,1.,2.82808728190157));
#42611=CARTESIAN_POINT('Ctrl Pts',(-2.9924915517034,1.,2.83526351254248));
#42612=CARTESIAN_POINT('Ctrl Pts',(-2.99542425341685,1.,2.84246132984415));
#42613=CARTESIAN_POINT('Ctrl Pts',(-2.99832751144925,1.,2.84968053289451));
#42614=CARTESIAN_POINT('Ctrl Pts',(-3.00120150796095,1.,2.85692085715686));
#42615=CARTESIAN_POINT('Ctrl Pts',(-3.00404638316867,1.,2.86418200833667));
#42616=CARTESIAN_POINT('Ctrl Pts',(-3.00686224485784,1.,2.87146368430502));
#42617=CARTESIAN_POINT('Ctrl Pts',(-3.00964918108476,1.,2.87876560072727));
#42618=CARTESIAN_POINT('Ctrl Pts',(-3.01240727308829,1.,2.8860875170608));
#42619=CARTESIAN_POINT('Ctrl Pts',(-3.01513660431928,1.,2.89342925566321));
#42620=CARTESIAN_POINT('Ctrl Pts',(-3.01783725121981,1.,2.9007906910105));
#42621=CARTESIAN_POINT('Ctrl Pts',(-3.01997487193503,1.,2.90669553302526));
#42622=CARTESIAN_POINT('Ctrl Pts',(-3.02156522742431,1.,2.91113297348212));
#42623=CARTESIAN_POINT('Ctrl Pts',(-3.02261975104593,1.,2.91409518070399));
#42624=CARTESIAN_POINT('Ctrl Pts',(-3.02314558451372,1.,2.91557726271063));
#42625=CARTESIAN_POINT('Origin',(-3.02314558451372,0.,2.91557726271063));
#42626=CARTESIAN_POINT('',(-2.91557726271063,1.,3.02314558451372));
#42627=CARTESIAN_POINT('Origin',(0.,0.,0.));
#42628=CARTESIAN_POINT('',(-2.90994629141562,1.,2.36531447826213));
#42629=CARTESIAN_POINT('Origin',(0.,1.,0.));
#42630=CARTESIAN_POINT('Ctrl Pts',(-2.90994629141562,1.,2.36531447826213));
#42631=CARTESIAN_POINT('Ctrl Pts',(-2.90994629141562,0.666666666666667,
2.36531447826213));
#42632=CARTESIAN_POINT('Ctrl Pts',(-2.90994629141562,0.333333333333333,
2.36531447826213));
#42633=CARTESIAN_POINT('Ctrl Pts',(-2.90994629141562,-0.333333333333333,
2.36531447826213));
#42634=CARTESIAN_POINT('Ctrl Pts',(-2.90994629141562,-0.666666666666667,
2.36531447826213));
#42635=CARTESIAN_POINT('Ctrl Pts',(-2.90994629141562,-1.,2.36531447826213));
#42636=CARTESIAN_POINT('Ctrl Pts',(-3.35260583073571,-1.,2.52982887637028));
#42637=CARTESIAN_POINT('Ctrl Pts',(-3.35260583073571,1.,2.52982887637028));
#42638=CARTESIAN_POINT('Ctrl Pts',(-3.35105973714426,-1.,2.52954136549357));
#42639=CARTESIAN_POINT('Ctrl Pts',(-3.35105973714426,1.,2.52954136549357));
#42640=CARTESIAN_POINT('Ctrl Pts',(-3.34796903577628,-1.,2.5289632161143));
#42641=CARTESIAN_POINT('Ctrl Pts',(-3.34796903577628,1.,2.5289632161143));
#42642=CARTESIAN_POINT('Ctrl Pts',(-3.34333744117093,-1.,2.52808660916879));
#42643=CARTESIAN_POINT('Ctrl Pts',(-3.34333744117093,1.,2.52808660916879));
#42644=CARTESIAN_POINT('Ctrl Pts',(-3.33717090000955,-1.,2.52689902691551));
#42645=CARTESIAN_POINT('Ctrl Pts',(-3.33717090000955,1.,2.52689902691551));
#42646=CARTESIAN_POINT('Ctrl Pts',(-3.32947762189049,-1.,2.52538321165774));
#42647=CARTESIAN_POINT('Ctrl Pts',(-3.32947762189049,1.,2.52538321165774));
#42648=CARTESIAN_POINT('Ctrl Pts',(-3.32179931079521,-1.,2.52383598396878));
#42649=CARTESIAN_POINT('Ctrl Pts',(-3.32179931079521,1.,2.52383598396878));
#42650=CARTESIAN_POINT('Ctrl Pts',(-3.31413607874727,-1.,2.52225724871375));
#42651=CARTESIAN_POINT('Ctrl Pts',(-3.31413607874727,1.,2.52225724871375));
#42652=CARTESIAN_POINT('Ctrl Pts',(-3.30648808814986,-1.,2.52064689568167));
#42653=CARTESIAN_POINT('Ctrl Pts',(-3.30648808814986,1.,2.52064689568167));
#42654=CARTESIAN_POINT('Ctrl Pts',(-3.29885556387661,-1.,2.51900480700548));
#42655=CARTESIAN_POINT('Ctrl Pts',(-3.29885556387661,1.,2.51900480700548));
#42656=CARTESIAN_POINT('Ctrl Pts',(-3.2912387729863,-1.,2.51733085123316));
#42657=CARTESIAN_POINT('Ctrl Pts',(-3.2912387729863,1.,2.51733085123316));
#42658=CARTESIAN_POINT('Ctrl Pts',(-3.28363799702583,-1.,2.51562487464215));
#42659=CARTESIAN_POINT('Ctrl Pts',(-3.28363799702583,1.,2.51562487464215));
#42660=CARTESIAN_POINT('Ctrl Pts',(-3.27605350473048,-1.,2.51388669270329));
#42661=CARTESIAN_POINT('Ctrl Pts',(-3.27605350473048,1.,2.51388669270329));
#42662=CARTESIAN_POINT('Ctrl Pts',(-3.26848552888271,-1.,2.51211608411539));
#42663=CARTESIAN_POINT('Ctrl Pts',(-3.26848552888271,1.,2.51211608411539));
#42664=CARTESIAN_POINT('Ctrl Pts',(-3.26093423001716,-1.,2.51031277813697));
#42665=CARTESIAN_POINT('Ctrl Pts',(-3.26093423001716,1.,2.51031277813697));
#42666=CARTESIAN_POINT('Ctrl Pts',(-3.25339971461265,-1.,2.50847647070936));
#42667=CARTESIAN_POINT('Ctrl Pts',(-3.25339971461265,1.,2.50847647070936));
#42668=CARTESIAN_POINT('Ctrl Pts',(-3.24588208984042,-1.,2.50660685940645));
#42669=CARTESIAN_POINT('Ctrl Pts',(-3.24588208984042,1.,2.50660685940645));
#42670=CARTESIAN_POINT('Ctrl Pts',(-3.23838151080383,-1.,2.50470367580078));
#42671=CARTESIAN_POINT('Ctrl Pts',(-3.23838151080383,1.,2.50470367580078));
#42672=CARTESIAN_POINT('Ctrl Pts',(-3.23089822320596,-1.,2.50276671338074));
#42673=CARTESIAN_POINT('Ctrl Pts',(-3.23089822320596,1.,2.50276671338074));
#42674=CARTESIAN_POINT('Ctrl Pts',(-3.22343262620387,-1.,2.5007958720187));
#42675=CARTESIAN_POINT('Ctrl Pts',(-3.22343262620387,1.,2.5007958720187));
#42676=CARTESIAN_POINT('Ctrl Pts',(-3.21598526261157,-1.,2.49879114599293));
#42677=CARTESIAN_POINT('Ctrl Pts',(-3.21598526261157,1.,2.49879114599293));
#42678=CARTESIAN_POINT('Ctrl Pts',(-3.2085566984974,-1.,2.49675252647298));
#42679=CARTESIAN_POINT('Ctrl Pts',(-3.2085566984974,1.,2.49675252647298));
#42680=CARTESIAN_POINT('Ctrl Pts',(-3.20114742397549,-1.,2.49467992057726));
#42681=CARTESIAN_POINT('Ctrl Pts',(-3.20114742397549,1.,2.49467992057726));
#42682=CARTESIAN_POINT('Ctrl Pts',(-3.19375775555814,-1.,2.4925730723986));
#42683=CARTESIAN_POINT('Ctrl Pts',(-3.19375775555814,1.,2.4925730723986));
#42684=CARTESIAN_POINT('Ctrl Pts',(-3.18638771282315,-1.,2.49043146334095));
#42685=CARTESIAN_POINT('Ctrl Pts',(-3.18638771282315,1.,2.49043146334095));
#42686=CARTESIAN_POINT('Ctrl Pts',(-3.17903698136679,-1.,2.48825428288243));
#42687=CARTESIAN_POINT('Ctrl Pts',(-3.17903698136679,1.,2.48825428288243));
#42688=CARTESIAN_POINT('Ctrl Pts',(-3.17170518863357,-1.,2.48604065348619));
#42689=CARTESIAN_POINT('Ctrl Pts',(-3.17170518863357,1.,2.48604065348619));
#42690=CARTESIAN_POINT('Ctrl Pts',(-3.16439213290181,-1.,2.48378981792739));
#42691=CARTESIAN_POINT('Ctrl Pts',(-3.16439213290181,1.,2.48378981792739));
#42692=CARTESIAN_POINT('Ctrl Pts',(-3.15709802322735,-1.,2.48150133566568));
#42693=CARTESIAN_POINT('Ctrl Pts',(-3.15709802322735,1.,2.48150133566568));
#42694=CARTESIAN_POINT('Ctrl Pts',(-3.14982373241335,-1.,2.47917529057016));
#42695=CARTESIAN_POINT('Ctrl Pts',(-3.14982373241335,1.,2.47917529057016));
#42696=CARTESIAN_POINT('Ctrl Pts',(-3.14257099546531,-1.,2.47681245356095));
#42697=CARTESIAN_POINT('Ctrl Pts',(-3.14257099546531,1.,2.47681245356095));
#42698=CARTESIAN_POINT('Ctrl Pts',(-3.13534181229282,-1.,2.47441378371923));
#42699=CARTESIAN_POINT('Ctrl Pts',(-3.13534181229282,1.,2.47441378371923));
#42700=CARTESIAN_POINT('Ctrl Pts',(-3.12813790805948,-1.,2.47197997765868));
#42701=CARTESIAN_POINT('Ctrl Pts',(-3.12813790805948,1.,2.47197997765868));
#42702=CARTESIAN_POINT('Ctrl Pts',(-3.12096015766984,-1.,2.4695109894747));
#42703=CARTESIAN_POINT('Ctrl Pts',(-3.12096015766984,1.,2.4695109894747));
#42704=CARTESIAN_POINT('Ctrl Pts',(-3.11380805536124,-1.,2.46700558843507));
#42705=CARTESIAN_POINT('Ctrl Pts',(-3.11380805536124,1.,2.46700558843507));
#42706=CARTESIAN_POINT('Ctrl Pts',(-3.10667907901981,-1.,2.46446082979645));
#42707=CARTESIAN_POINT('Ctrl Pts',(-3.10667907901981,1.,2.46446082979645));
#42708=CARTESIAN_POINT('Ctrl Pts',(-3.09956993697048,-1.,2.4618730850188));
#42709=CARTESIAN_POINT('Ctrl Pts',(-3.09956993697048,1.,2.4618730850188));
#42710=CARTESIAN_POINT('Ctrl Pts',(-3.09247787931881,-1.,2.45923912563875));
#42711=CARTESIAN_POINT('Ctrl Pts',(-3.09247787931881,1.,2.45923912563875));
#42712=CARTESIAN_POINT('Ctrl Pts',(-3.08540206545313,-1.,2.45655725437037));
#42713=CARTESIAN_POINT('Ctrl Pts',(-3.08540206545313,1.,2.45655725437037));
#42714=CARTESIAN_POINT('Ctrl Pts',(-3.07834472886145,-1.,2.45382826787795));
#42715=CARTESIAN_POINT('Ctrl Pts',(-3.07834472886145,1.,2.45382826787795));
#42716=CARTESIAN_POINT('Ctrl Pts',(-3.0713129052131,-1.,2.45105688854432));
#42717=CARTESIAN_POINT('Ctrl Pts',(-3.0713129052131,1.,2.45105688854432));
#42718=CARTESIAN_POINT('Ctrl Pts',(-3.06431596421422,-1.,2.44824970516558));
#42719=CARTESIAN_POINT('Ctrl Pts',(-3.06431596421422,1.,2.44824970516558));
#42720=CARTESIAN_POINT('Ctrl Pts',(-3.05736242671521,-1.,2.44541251892568));
#42721=CARTESIAN_POINT('Ctrl Pts',(-3.05736242671521,1.,2.44541251892568));
#42722=CARTESIAN_POINT('Ctrl Pts',(-3.05045678021509,-1.,2.44254768923109));
#42723=CARTESIAN_POINT('Ctrl Pts',(-3.05045678021509,1.,2.44254768923109));
#42724=CARTESIAN_POINT('Ctrl Pts',(-3.04359685040545,-1.,2.43965194061849));
#42725=CARTESIAN_POINT('Ctrl Pts',(-3.04359685040545,1.,2.43965194061849));
#42726=CARTESIAN_POINT('Ctrl Pts',(-3.03676949672797,-1.,2.43671278042394));
#42727=CARTESIAN_POINT('Ctrl Pts',(-3.03676949672797,1.,2.43671278042394));
#42728=CARTESIAN_POINT('Ctrl Pts',(-3.02995534946946,-1.,2.43371241361462));
#42729=CARTESIAN_POINT('Ctrl Pts',(-3.02995534946946,1.,2.43371241361462));
#42730=CARTESIAN_POINT('Ctrl Pts',(-3.02313656035977,-1.,2.43063415586615));
#42731=CARTESIAN_POINT('Ctrl Pts',(-3.02313656035977,1.,2.43063415586615));
#42732=CARTESIAN_POINT('Ctrl Pts',(-3.01630420830494,-1.,2.4274685626416));
#42733=CARTESIAN_POINT('Ctrl Pts',(-3.01630420830494,1.,2.4274685626416));
#42734=CARTESIAN_POINT('Ctrl Pts',(-3.00946442616674,-1.,2.42421849439625));
#42735=CARTESIAN_POINT('Ctrl Pts',(-3.00946442616674,1.,2.42421849439625));
#42736=CARTESIAN_POINT('Ctrl Pts',(-3.00264868586038,-1.,2.42090763946812));
#42737=CARTESIAN_POINT('Ctrl Pts',(-3.00264868586038,1.,2.42090763946812));
#42738=CARTESIAN_POINT('Ctrl Pts',(-2.99590509293561,-1.,2.4175732450056));
#42739=CARTESIAN_POINT('Ctrl Pts',(-2.99590509293561,1.,2.4175732450056));
#42740=CARTESIAN_POINT('Ctrl Pts',(-2.98927983005851,-1.,2.4142506419963));
#42741=CARTESIAN_POINT('Ctrl Pts',(-2.98927983005851,1.,2.4142506419963));
#42742=CARTESIAN_POINT('Ctrl Pts',(-2.98280015815132,-1.,2.41095909342591));
#42743=CARTESIAN_POINT('Ctrl Pts',(-2.98280015815132,1.,2.41095909342591));
#42744=CARTESIAN_POINT('Ctrl Pts',(-2.97646002822395,-1.,2.40768975073691));
#42745=CARTESIAN_POINT('Ctrl Pts',(-2.97646002822395,1.,2.40768975073691));
#42746=CARTESIAN_POINT('Ctrl Pts',(-2.97019641312272,-1.,2.40438604734848));
#42747=CARTESIAN_POINT('Ctrl Pts',(-2.97019641312272,1.,2.40438604734848));
#42748=CARTESIAN_POINT('Ctrl Pts',(-2.96390432240181,-1.,2.40095565711535));
#42749=CARTESIAN_POINT('Ctrl Pts',(-2.96390432240181,1.,2.40095565711535));
#42750=CARTESIAN_POINT('Ctrl Pts',(-2.95748006482811,-1.,2.39730553974412));
#42751=CARTESIAN_POINT('Ctrl Pts',(-2.95748006482811,1.,2.39730553974412));
#42752=CARTESIAN_POINT('Ctrl Pts',(-2.95085857128372,-1.,2.39337207631613));
#42753=CARTESIAN_POINT('Ctrl Pts',(-2.95085857128372,1.,2.39337207631613));
#42754=CARTESIAN_POINT('Ctrl Pts',(-2.94404820669135,-1.,2.38914929090806));
#42755=CARTESIAN_POINT('Ctrl Pts',(-2.94404820669135,1.,2.38914929090806));
#42756=CARTESIAN_POINT('Ctrl Pts',(-2.93717903280599,-1.,2.38472771516476));
#42757=CARTESIAN_POINT('Ctrl Pts',(-2.93717903280599,1.,2.38472771516476));
#42758=CARTESIAN_POINT('Ctrl Pts',(-2.93049643640517,-1.,2.3802898958232));
#42759=CARTESIAN_POINT('Ctrl Pts',(-2.93049643640517,1.,2.3802898958232));
#42760=CARTESIAN_POINT('Ctrl Pts',(-2.92430340582912,-1.,2.37606510524271));
#42761=CARTESIAN_POINT('Ctrl Pts',(-2.92430340582912,1.,2.37606510524271));
#42762=CARTESIAN_POINT('Ctrl Pts',(-2.9189150379156,-1.,2.37229381109939));
#42763=CARTESIAN_POINT('Ctrl Pts',(-2.9189150379156,1.,2.37229381109939));
#42764=CARTESIAN_POINT('Ctrl Pts',(-2.91461249883016,-1.,2.36919161373074));
#42765=CARTESIAN_POINT('Ctrl Pts',(-2.91461249883016,1.,2.36919161373074));
#42766=CARTESIAN_POINT('Ctrl Pts',(-2.9115863784165,-1.,2.36690501170317));
#42767=CARTESIAN_POINT('Ctrl Pts',(-2.9115863784165,1.,2.36690501170317));
#42768=CARTESIAN_POINT('Ctrl Pts',(-2.91025813829606,-1.,2.36578327194396));
#42769=CARTESIAN_POINT('Ctrl Pts',(-2.91025813829606,1.,2.36578327194396));
#42770=CARTESIAN_POINT('Ctrl Pts',(-2.90989022547738,-1.,2.36535052956704));
#42771=CARTESIAN_POINT('Ctrl Pts',(-2.90989022547738,1.,2.36535052956704));
#42772=CARTESIAN_POINT('Ctrl Pts',(-2.90992398626098,-1.,2.36524348105023));
#42773=CARTESIAN_POINT('Ctrl Pts',(-2.90992398626098,1.,2.36524348105023));
#42774=CARTESIAN_POINT('Ctrl Pts',(-2.91001063062876,-1.,2.36523532225181));
#42775=CARTESIAN_POINT('Ctrl Pts',(-2.91001063062876,1.,2.36523532225181));
#42776=CARTESIAN_POINT('',(-3.35260583073571,1.,2.52982887637028));
#42777=CARTESIAN_POINT('Ctrl Pts',(-3.35260583073571,1.,2.52982887637028));
#42778=CARTESIAN_POINT('Ctrl Pts',(-3.35105973714426,1.,2.52954136549357));
#42779=CARTESIAN_POINT('Ctrl Pts',(-3.34796903577628,1.,2.5289632161143));
#42780=CARTESIAN_POINT('Ctrl Pts',(-3.34333744117093,1.,2.52808660916879));
#42781=CARTESIAN_POINT('Ctrl Pts',(-3.33717090000955,1.,2.52689902691551));
#42782=CARTESIAN_POINT('Ctrl Pts',(-3.32947762189049,1.,2.52538321165774));
#42783=CARTESIAN_POINT('Ctrl Pts',(-3.32179931079521,1.,2.52383598396878));
#42784=CARTESIAN_POINT('Ctrl Pts',(-3.31413607874727,1.,2.52225724871375));
#42785=CARTESIAN_POINT('Ctrl Pts',(-3.30648808814986,1.,2.52064689568167));
#42786=CARTESIAN_POINT('Ctrl Pts',(-3.29885556387661,1.,2.51900480700548));
#42787=CARTESIAN_POINT('Ctrl Pts',(-3.2912387729863,1.,2.51733085123316));
#42788=CARTESIAN_POINT('Ctrl Pts',(-3.28363799702583,1.,2.51562487464215));
#42789=CARTESIAN_POINT('Ctrl Pts',(-3.27605350473048,1.,2.51388669270329));
#42790=CARTESIAN_POINT('Ctrl Pts',(-3.26848552888271,1.,2.51211608411539));
#42791=CARTESIAN_POINT('Ctrl Pts',(-3.26093423001716,1.,2.51031277813697));
#42792=CARTESIAN_POINT('Ctrl Pts',(-3.25339971461265,1.,2.50847647070936));
#42793=CARTESIAN_POINT('Ctrl Pts',(-3.24588208984042,1.,2.50660685940645));
#42794=CARTESIAN_POINT('Ctrl Pts',(-3.23838151080383,1.,2.50470367580078));
#42795=CARTESIAN_POINT('Ctrl Pts',(-3.23089822320596,1.,2.50276671338074));
#42796=CARTESIAN_POINT('Ctrl Pts',(-3.22343262620387,1.,2.5007958720187));
#42797=CARTESIAN_POINT('Ctrl Pts',(-3.21598526261157,1.,2.49879114599293));
#42798=CARTESIAN_POINT('Ctrl Pts',(-3.2085566984974,1.,2.49675252647298));
#42799=CARTESIAN_POINT('Ctrl Pts',(-3.20114742397549,1.,2.49467992057726));
#42800=CARTESIAN_POINT('Ctrl Pts',(-3.19375775555814,1.,2.4925730723986));
#42801=CARTESIAN_POINT('Ctrl Pts',(-3.18638771282315,1.,2.49043146334095));
#42802=CARTESIAN_POINT('Ctrl Pts',(-3.17903698136679,1.,2.48825428288243));
#42803=CARTESIAN_POINT('Ctrl Pts',(-3.17170518863357,1.,2.48604065348619));
#42804=CARTESIAN_POINT('Ctrl Pts',(-3.16439213290181,1.,2.48378981792739));
#42805=CARTESIAN_POINT('Ctrl Pts',(-3.15709802322735,1.,2.48150133566568));
#42806=CARTESIAN_POINT('Ctrl Pts',(-3.14982373241335,1.,2.47917529057016));
#42807=CARTESIAN_POINT('Ctrl Pts',(-3.14257099546531,1.,2.47681245356095));
#42808=CARTESIAN_POINT('Ctrl Pts',(-3.13534181229282,1.,2.47441378371923));
#42809=CARTESIAN_POINT('Ctrl Pts',(-3.12813790805948,1.,2.47197997765868));
#42810=CARTESIAN_POINT('Ctrl Pts',(-3.12096015766984,1.,2.4695109894747));
#42811=CARTESIAN_POINT('Ctrl Pts',(-3.11380805536124,1.,2.46700558843507));
#42812=CARTESIAN_POINT('Ctrl Pts',(-3.10667907901981,1.,2.46446082979645));
#42813=CARTESIAN_POINT('Ctrl Pts',(-3.09956993697048,1.,2.4618730850188));
#42814=CARTESIAN_POINT('Ctrl Pts',(-3.09247787931881,1.,2.45923912563875));
#42815=CARTESIAN_POINT('Ctrl Pts',(-3.08540206545313,1.,2.45655725437037));
#42816=CARTESIAN_POINT('Ctrl Pts',(-3.07834472886145,1.,2.45382826787795));
#42817=CARTESIAN_POINT('Ctrl Pts',(-3.0713129052131,1.,2.45105688854432));
#42818=CARTESIAN_POINT('Ctrl Pts',(-3.06431596421422,1.,2.44824970516558));
#42819=CARTESIAN_POINT('Ctrl Pts',(-3.05736242671521,1.,2.44541251892568));
#42820=CARTESIAN_POINT('Ctrl Pts',(-3.05045678021509,1.,2.44254768923109));
#42821=CARTESIAN_POINT('Ctrl Pts',(-3.04359685040545,1.,2.43965194061849));
#42822=CARTESIAN_POINT('Ctrl Pts',(-3.03676949672797,1.,2.43671278042394));
#42823=CARTESIAN_POINT('Ctrl Pts',(-3.02995534946946,1.,2.43371241361462));
#42824=CARTESIAN_POINT('Ctrl Pts',(-3.02313656035977,1.,2.43063415586615));
#42825=CARTESIAN_POINT('Ctrl Pts',(-3.01630420830494,1.,2.4274685626416));
#42826=CARTESIAN_POINT('Ctrl Pts',(-3.00946442616674,1.,2.42421849439625));
#42827=CARTESIAN_POINT('Ctrl Pts',(-3.00264868586038,1.,2.42090763946812));
#42828=CARTESIAN_POINT('Ctrl Pts',(-2.99590509293561,1.,2.4175732450056));
#42829=CARTESIAN_POINT('Ctrl Pts',(-2.98927983005851,1.,2.4142506419963));
#42830=CARTESIAN_POINT('Ctrl Pts',(-2.98280015815132,1.,2.41095909342591));
#42831=CARTESIAN_POINT('Ctrl Pts',(-2.97646002822395,1.,2.40768975073691));
#42832=CARTESIAN_POINT('Ctrl Pts',(-2.97019641312272,1.,2.40438604734848));
#42833=CARTESIAN_POINT('Ctrl Pts',(-2.96390432240181,1.,2.40095565711535));
#42834=CARTESIAN_POINT('Ctrl Pts',(-2.95748006482811,1.,2.39730553974412));
#42835=CARTESIAN_POINT('Ctrl Pts',(-2.95085857128372,1.,2.39337207631613));
#42836=CARTESIAN_POINT('Ctrl Pts',(-2.94404820669135,1.,2.38914929090806));
#42837=CARTESIAN_POINT('Ctrl Pts',(-2.93717903280599,1.,2.38472771516476));
#42838=CARTESIAN_POINT('Ctrl Pts',(-2.93049643640517,1.,2.3802898958232));
#42839=CARTESIAN_POINT('Ctrl Pts',(-2.92430340582912,1.,2.37606510524271));
#42840=CARTESIAN_POINT('Ctrl Pts',(-2.9189150379156,1.,2.37229381109939));
#42841=CARTESIAN_POINT('Ctrl Pts',(-2.91461249883016,1.,2.36919161373074));
#42842=CARTESIAN_POINT('Ctrl Pts',(-2.91181344022628,1.,2.36707658451709));
#42843=CARTESIAN_POINT('Ctrl Pts',(-2.91051690822262,1.,2.36599991765853));
#42844=CARTESIAN_POINT('Ctrl Pts',(-2.9100577052777,1.,2.36553202948741));
#42845=CARTESIAN_POINT('Ctrl Pts',(-2.90995756655559,1.,2.3653621118858));
#42846=CARTESIAN_POINT('Ctrl Pts',(-2.90994629141563,1.,2.36531447826213));
#42847=CARTESIAN_POINT('',(-3.35260583073571,0.,2.52982887637028));
#42848=CARTESIAN_POINT('Ctrl Pts',(-3.1487152044751,-1.,2.03668666247593));
#42849=CARTESIAN_POINT('Ctrl Pts',(-3.1487152044751,1.,2.03668666247593));
#42850=CARTESIAN_POINT('Ctrl Pts',(-3.14869618937258,-1.,2.03660173757879));
#42851=CARTESIAN_POINT('Ctrl Pts',(-3.14869618937258,1.,2.03660173757879));
#42852=CARTESIAN_POINT('Ctrl Pts',(-3.14878756590812,-1.,2.03653654935592));
#42853=CARTESIAN_POINT('Ctrl Pts',(-3.14878756590812,1.,2.03653654935592));
#42854=CARTESIAN_POINT('Ctrl Pts',(-3.14931281968048,-1.,2.03675273049189));
#42855=CARTESIAN_POINT('Ctrl Pts',(-3.14931281968048,1.,2.03675273049189));
#42856=CARTESIAN_POINT('Ctrl Pts',(-3.15079010635742,-1.,2.03766932526445));
#42857=CARTESIAN_POINT('Ctrl Pts',(-3.15079010635742,1.,2.03766932526445));
#42858=CARTESIAN_POINT('Ctrl Pts',(-3.15389991674792,-1.,2.03984073791519));
#42859=CARTESIAN_POINT('Ctrl Pts',(-3.15389991674792,1.,2.03984073791519));
#42860=CARTESIAN_POINT('Ctrl Pts',(-3.15817983946367,-1.,2.04297406404027));
#42861=CARTESIAN_POINT('Ctrl Pts',(-3.15817983946367,1.,2.04297406404027));
#42862=CARTESIAN_POINT('Ctrl Pts',(-3.16343165058912,-1.,2.04693331247446));
#42863=CARTESIAN_POINT('Ctrl Pts',(-3.16343165058912,1.,2.04693331247446));
#42864=CARTESIAN_POINT('Ctrl Pts',(-3.16936341689527,-1.,2.05151770247233));
#42865=CARTESIAN_POINT('Ctrl Pts',(-3.16936341689527,1.,2.05151770247233));
#42866=CARTESIAN_POINT('Ctrl Pts',(-3.17564906975371,-1.,2.05650186773132));
#42867=CARTESIAN_POINT('Ctrl Pts',(-3.17564906975371,1.,2.05650186773132));
#42868=CARTESIAN_POINT('Ctrl Pts',(-3.18197692964614,-1.,2.06166849827101));
#42869=CARTESIAN_POINT('Ctrl Pts',(-3.18197692964614,1.,2.06166849827101));
#42870=CARTESIAN_POINT('Ctrl Pts',(-3.18809755562368,-1.,2.06684062744112));
#42871=CARTESIAN_POINT('Ctrl Pts',(-3.18809755562368,1.,2.06684062744112));
#42872=CARTESIAN_POINT('Ctrl Pts',(-3.19388465568252,-1.,2.07192253497857));
#42873=CARTESIAN_POINT('Ctrl Pts',(-3.19388465568252,1.,2.07192253497857));
#42874=CARTESIAN_POINT('Ctrl Pts',(-3.19934132836019,-1.,2.07690441870722));
#42875=CARTESIAN_POINT('Ctrl Pts',(-3.19934132836019,1.,2.07690441870722));
#42876=CARTESIAN_POINT('Ctrl Pts',(-3.2045481863073,-1.,2.08182850370878));
#42877=CARTESIAN_POINT('Ctrl Pts',(-3.2045481863073,1.,2.08182850370878));
#42878=CARTESIAN_POINT('Ctrl Pts',(-3.20962575845463,-1.,2.08676465517455));
#42879=CARTESIAN_POINT('Ctrl Pts',(-3.20962575845463,1.,2.08676465517455));
#42880=CARTESIAN_POINT('Ctrl Pts',(-3.21469429601654,-1.,2.09178419460443));
#42881=CARTESIAN_POINT('Ctrl Pts',(-3.21469429601654,1.,2.09178419460443));
#42882=CARTESIAN_POINT('Ctrl Pts',(-3.21982707347009,-1.,2.09692958434895));
#42883=CARTESIAN_POINT('Ctrl Pts',(-3.21982707347009,1.,2.09692958434895));
#42884=CARTESIAN_POINT('Ctrl Pts',(-3.22503437553434,-1.,2.10220384298492));
#42885=CARTESIAN_POINT('Ctrl Pts',(-3.22503437553434,1.,2.10220384298492));
#42886=CARTESIAN_POINT('Ctrl Pts',(-3.23028945793289,-1.,2.10758699642451));
#42887=CARTESIAN_POINT('Ctrl Pts',(-3.23028945793289,1.,2.10758699642451));
#42888=CARTESIAN_POINT('Ctrl Pts',(-3.23554444767099,-1.,2.11304604021773));
#42889=CARTESIAN_POINT('Ctrl Pts',(-3.23554444767099,1.,2.11304604021773));
#42890=CARTESIAN_POINT('Ctrl Pts',(-3.24074905517293,-1.,2.11854673326979));
#42891=CARTESIAN_POINT('Ctrl Pts',(-3.24074905517293,1.,2.11854673326979));
#42892=CARTESIAN_POINT('Ctrl Pts',(-3.24587102613376,-1.,2.12406646410962));
#42893=CARTESIAN_POINT('Ctrl Pts',(-3.24587102613376,1.,2.12406646410962));
#42894=CARTESIAN_POINT('Ctrl Pts',(-3.25090574494028,-1.,2.12960028396832));
#42895=CARTESIAN_POINT('Ctrl Pts',(-3.25090574494028,1.,2.12960028396832));
#42896=CARTESIAN_POINT('Ctrl Pts',(-3.25586495065054,-1.,2.13515375878803));
#42897=CARTESIAN_POINT('Ctrl Pts',(-3.25586495065054,1.,2.13515375878803));
#42898=CARTESIAN_POINT('Ctrl Pts',(-3.26077002641879,-1.,2.14073870754264));
#42899=CARTESIAN_POINT('Ctrl Pts',(-3.26077002641879,1.,2.14073870754264));
#42900=CARTESIAN_POINT('Ctrl Pts',(-3.26564388189759,-1.,2.1463680529566));
#42901=CARTESIAN_POINT('Ctrl Pts',(-3.26564388189759,1.,2.1463680529566));
#42902=CARTESIAN_POINT('Ctrl Pts',(-3.27050245897228,-1.,2.15205043199808));
#42903=CARTESIAN_POINT('Ctrl Pts',(-3.27050245897228,1.,2.15205043199808));
#42904=CARTESIAN_POINT('Ctrl Pts',(-3.27534954469187,-1.,2.15778690038347));
#42905=CARTESIAN_POINT('Ctrl Pts',(-3.27534954469187,1.,2.15778690038347));
#42906=CARTESIAN_POINT('Ctrl Pts',(-3.280181508414,-1.,2.16357391934425));
#42907=CARTESIAN_POINT('Ctrl Pts',(-3.280181508414,1.,2.16357391934425));
#42908=CARTESIAN_POINT('Ctrl Pts',(-3.28499019979724,-1.,2.16940517773455));
#42909=CARTESIAN_POINT('Ctrl Pts',(-3.28499019979724,1.,2.16940517773455));
#42910=CARTESIAN_POINT('Ctrl Pts',(-3.28976645712568,-1.,2.17527380048423));
#42911=CARTESIAN_POINT('Ctrl Pts',(-3.28976645712568,1.,2.17527380048423));
#42912=CARTESIAN_POINT('Ctrl Pts',(-3.2945036150049,-1.,2.18117455557065));
#42913=CARTESIAN_POINT('Ctrl Pts',(-3.2945036150049,1.,2.18117455557065));
#42914=CARTESIAN_POINT('Ctrl Pts',(-3.29920022557639,-1.,2.18710556500327));
#42915=CARTESIAN_POINT('Ctrl Pts',(-3.29920022557639,1.,2.18710556500327));
#42916=CARTESIAN_POINT('Ctrl Pts',(-3.30385816281831,-1.,2.19306710376111));
#42917=CARTESIAN_POINT('Ctrl Pts',(-3.30385816281831,1.,2.19306710376111));
#42918=CARTESIAN_POINT('Ctrl Pts',(-3.30848134694595,-1.,2.19906078949923));
#42919=CARTESIAN_POINT('Ctrl Pts',(-3.30848134694595,1.,2.19906078949923));
#42920=CARTESIAN_POINT('Ctrl Pts',(-3.31307424608949,-1.,2.20508863150607));
#42921=CARTESIAN_POINT('Ctrl Pts',(-3.31307424608949,1.,2.20508863150607));
#42922=CARTESIAN_POINT('Ctrl Pts',(-3.31764044024235,-1.,2.21115211847875));
#42923=CARTESIAN_POINT('Ctrl Pts',(-3.31764044024235,1.,2.21115211847875));
#42924=CARTESIAN_POINT('Ctrl Pts',(-3.32218125618968,-1.,2.21725135110898));
#42925=CARTESIAN_POINT('Ctrl Pts',(-3.32218125618968,1.,2.21725135110898));
#42926=CARTESIAN_POINT('Ctrl Pts',(-3.3266964672289,-1.,2.22338548312772));
#42927=CARTESIAN_POINT('Ctrl Pts',(-3.3266964672289,1.,2.22338548312772));
#42928=CARTESIAN_POINT('Ctrl Pts',(-3.33118487773611,-1.,2.22955308907233));
#42929=CARTESIAN_POINT('Ctrl Pts',(-3.33118487773611,1.,2.22955308907233));
#42930=CARTESIAN_POINT('Ctrl Pts',(-3.33564495756482,-1.,2.23575256328812));
#42931=CARTESIAN_POINT('Ctrl Pts',(-3.33564495756482,1.,2.23575256328812));
#42932=CARTESIAN_POINT('Ctrl Pts',(-3.34007543738025,-1.,2.24198249391422));
#42933=CARTESIAN_POINT('Ctrl Pts',(-3.34007543738025,1.,2.24198249391422));
#42934=CARTESIAN_POINT('Ctrl Pts',(-3.34447596770723,-1.,2.24824207678256));
#42935=CARTESIAN_POINT('Ctrl Pts',(-3.34447596770723,1.,2.24824207678256));
#42936=CARTESIAN_POINT('Ctrl Pts',(-3.34884690292285,-1.,2.25453097693483));
#42937=CARTESIAN_POINT('Ctrl Pts',(-3.34884690292285,1.,2.25453097693483));
#42938=CARTESIAN_POINT('Ctrl Pts',(-3.35318902552626,-1.,2.26084915222449));
#42939=CARTESIAN_POINT('Ctrl Pts',(-3.35318902552626,1.,2.26084915222449));
#42940=CARTESIAN_POINT('Ctrl Pts',(-3.35750328523061,-1.,2.2671966857991));
#42941=CARTESIAN_POINT('Ctrl Pts',(-3.35750328523061,1.,2.2671966857991));
#42942=CARTESIAN_POINT('Ctrl Pts',(-3.36179055004409,-1.,2.2735736262093));
#42943=CARTESIAN_POINT('Ctrl Pts',(-3.36179055004409,1.,2.2735736262093));
#42944=CARTESIAN_POINT('Ctrl Pts',(-3.36605130713076,-1.,2.27997979458037));
#42945=CARTESIAN_POINT('Ctrl Pts',(-3.36605130713076,1.,2.27997979458037));
#42946=CARTESIAN_POINT('Ctrl Pts',(-3.37028570206488,-1.,2.28641481081137));
#42947=CARTESIAN_POINT('Ctrl Pts',(-3.37028570206488,1.,2.28641481081137));
#42948=CARTESIAN_POINT('Ctrl Pts',(-3.37449367172826,-1.,2.29287818007393));
#42949=CARTESIAN_POINT('Ctrl Pts',(-3.37449367172826,1.,2.29287818007393));
#42950=CARTESIAN_POINT('Ctrl Pts',(-3.37867504959433,-1.,2.29936936127624));
#42951=CARTESIAN_POINT('Ctrl Pts',(-3.37867504959433,1.,2.29936936127624));
#42952=CARTESIAN_POINT('Ctrl Pts',(-3.3828296733661,-1.,2.30588783640343));
#42953=CARTESIAN_POINT('Ctrl Pts',(-3.3828296733661,1.,2.30588783640343));
#42954=CARTESIAN_POINT('Ctrl Pts',(-3.38695751492462,-1.,2.31243319489367));
#42955=CARTESIAN_POINT('Ctrl Pts',(-3.38695751492462,1.,2.31243319489367));
#42956=CARTESIAN_POINT('Ctrl Pts',(-3.39105869474822,-1.,2.31900513925424));
#42957=CARTESIAN_POINT('Ctrl Pts',(-3.39105869474822,1.,2.31900513925424));
#42958=CARTESIAN_POINT('Ctrl Pts',(-3.39513342019756,-1.,2.3256034390248));
#42959=CARTESIAN_POINT('Ctrl Pts',(-3.39513342019756,1.,2.3256034390248));
#42960=CARTESIAN_POINT('Ctrl Pts',(-3.39918194577956,-1.,2.33222789882489));
#42961=CARTESIAN_POINT('Ctrl Pts',(-3.39918194577956,1.,2.33222789882489));
#42962=CARTESIAN_POINT('Ctrl Pts',(-3.40320452776743,-1.,2.33887832342782));
#42963=CARTESIAN_POINT('Ctrl Pts',(-3.40320452776743,1.,2.33887832342782));
#42964=CARTESIAN_POINT('Ctrl Pts',(-3.40720137404297,-1.,2.34555447649188));
#42965=CARTESIAN_POINT('Ctrl Pts',(-3.40720137404297,1.,2.34555447649188));
#42966=CARTESIAN_POINT('Ctrl Pts',(-3.41117262314119,-1.,2.35225606824109));
#42967=CARTESIAN_POINT('Ctrl Pts',(-3.41117262314119,1.,2.35225606824109));
#42968=CARTESIAN_POINT('Ctrl Pts',(-3.41511836751469,-1.,2.35898278606946));
#42969=CARTESIAN_POINT('Ctrl Pts',(-3.41511836751469,1.,2.35898278606946));
#42970=CARTESIAN_POINT('Ctrl Pts',(-3.41903866635852,-1.,2.36573431470642));
#42971=CARTESIAN_POINT('Ctrl Pts',(-3.41903866635852,1.,2.36573431470642));
#42972=CARTESIAN_POINT('Ctrl Pts',(-3.42293356216511,-1.,2.37251035954292));
#42973=CARTESIAN_POINT('Ctrl Pts',(-3.42293356216511,1.,2.37251035954292));
#42974=CARTESIAN_POINT('Ctrl Pts',(-3.42680309754399,-1.,2.37931067028926));
#42975=CARTESIAN_POINT('Ctrl Pts',(-3.42680309754399,1.,2.37931067028926));
#42976=CARTESIAN_POINT('Ctrl Pts',(-3.4306473271292,-1.,2.38613505843552));
#42977=CARTESIAN_POINT('Ctrl Pts',(-3.4306473271292,1.,2.38613505843552));
#42978=CARTESIAN_POINT('Ctrl Pts',(-3.4344663067854,-1.,2.39298338804493));
#42979=CARTESIAN_POINT('Ctrl Pts',(-3.4344663067854,1.,2.39298338804493));
#42980=CARTESIAN_POINT('Ctrl Pts',(-3.43750133064416,-1.,2.39848113410292));
#42981=CARTESIAN_POINT('Ctrl Pts',(-3.43750133064416,1.,2.39848113410292));
#42982=CARTESIAN_POINT('Ctrl Pts',(-3.43976627484234,-1.,2.40261515589405));
#42983=CARTESIAN_POINT('Ctrl Pts',(-3.43976627484234,1.,2.40261515589405));
#42984=CARTESIAN_POINT('Ctrl Pts',(-3.44127120683039,-1.,2.4053759295909));
#42985=CARTESIAN_POINT('Ctrl Pts',(-3.44127120683039,1.,2.4053759295909));
#42986=CARTESIAN_POINT('Ctrl Pts',(-3.44202241512147,-1.,2.40675750623143));
#42987=CARTESIAN_POINT('Ctrl Pts',(-3.44202241512147,1.,2.40675750623143));
#42988=CARTESIAN_POINT('',(-3.14877060440327,1.,2.03660101169715));
#42989=CARTESIAN_POINT('Ctrl Pts',(-3.14877060440327,-1.,2.03660101169715));
#42990=CARTESIAN_POINT('Ctrl Pts',(-3.14877060440327,-0.666666666666667,
2.03660101169715));
#42991=CARTESIAN_POINT('Ctrl Pts',(-3.14877060440327,-0.333333333333333,
2.03660101169715));
#42992=CARTESIAN_POINT('Ctrl Pts',(-3.14877060440327,0.333333333333333,
2.03660101169715));
#42993=CARTESIAN_POINT('Ctrl Pts',(-3.14877060440327,0.666666666666667,
2.03660101169715));
#42994=CARTESIAN_POINT('Ctrl Pts',(-3.14877060440327,1.,2.03660101169715));
#42995=CARTESIAN_POINT('',(-3.44202241512147,1.,2.40675750623143));
#42996=CARTESIAN_POINT('',(-3.44202241512147,0.,2.40675750623143));
#42997=CARTESIAN_POINT('Ctrl Pts',(-3.14877060440327,1.,2.03660101169715));
#42998=CARTESIAN_POINT('Ctrl Pts',(-3.14881939088124,1.,2.03659701539259));
#42999=CARTESIAN_POINT('Ctrl Pts',(-3.1490119366901,1.,2.03663974554932));
#43000=CARTESIAN_POINT('Ctrl Pts',(-3.14959882629805,1.,2.03693188810544));
#43001=CARTESIAN_POINT('Ctrl Pts',(-3.15102344775328,1.,2.03783225495961));
#43002=CARTESIAN_POINT('Ctrl Pts',(-3.15389991674792,1.,2.03984073791519));
#43003=CARTESIAN_POINT('Ctrl Pts',(-3.15817983946367,1.,2.04297406404027));
#43004=CARTESIAN_POINT('Ctrl Pts',(-3.16343165058912,1.,2.04693331247446));
#43005=CARTESIAN_POINT('Ctrl Pts',(-3.16936341689527,1.,2.05151770247233));
#43006=CARTESIAN_POINT('Ctrl Pts',(-3.17564906975371,1.,2.05650186773132));
#43007=CARTESIAN_POINT('Ctrl Pts',(-3.18197692964614,1.,2.06166849827101));
#43008=CARTESIAN_POINT('Ctrl Pts',(-3.18809755562368,1.,2.06684062744112));
#43009=CARTESIAN_POINT('Ctrl Pts',(-3.19388465568252,1.,2.07192253497857));
#43010=CARTESIAN_POINT('Ctrl Pts',(-3.19934132836019,1.,2.07690441870722));
#43011=CARTESIAN_POINT('Ctrl Pts',(-3.2045481863073,1.,2.08182850370878));
#43012=CARTESIAN_POINT('Ctrl Pts',(-3.20962575845463,1.,2.08676465517455));
#43013=CARTESIAN_POINT('Ctrl Pts',(-3.21469429601654,1.,2.09178419460443));
#43014=CARTESIAN_POINT('Ctrl Pts',(-3.21982707347009,1.,2.09692958434895));
#43015=CARTESIAN_POINT('Ctrl Pts',(-3.22503437553434,1.,2.10220384298492));
#43016=CARTESIAN_POINT('Ctrl Pts',(-3.23028945793289,1.,2.10758699642451));
#43017=CARTESIAN_POINT('Ctrl Pts',(-3.23554444767099,1.,2.11304604021773));
#43018=CARTESIAN_POINT('Ctrl Pts',(-3.24074905517293,1.,2.11854673326979));
#43019=CARTESIAN_POINT('Ctrl Pts',(-3.24587102613376,1.,2.12406646410962));
#43020=CARTESIAN_POINT('Ctrl Pts',(-3.25090574494028,1.,2.12960028396832));
#43021=CARTESIAN_POINT('Ctrl Pts',(-3.25586495065054,1.,2.13515375878803));
#43022=CARTESIAN_POINT('Ctrl Pts',(-3.26077002641879,1.,2.14073870754264));
#43023=CARTESIAN_POINT('Ctrl Pts',(-3.26564388189759,1.,2.1463680529566));
#43024=CARTESIAN_POINT('Ctrl Pts',(-3.27050245897228,1.,2.15205043199808));
#43025=CARTESIAN_POINT('Ctrl Pts',(-3.27534954469187,1.,2.15778690038347));
#43026=CARTESIAN_POINT('Ctrl Pts',(-3.280181508414,1.,2.16357391934425));
#43027=CARTESIAN_POINT('Ctrl Pts',(-3.28499019979724,1.,2.16940517773455));
#43028=CARTESIAN_POINT('Ctrl Pts',(-3.28976645712568,1.,2.17527380048423));
#43029=CARTESIAN_POINT('Ctrl Pts',(-3.2945036150049,1.,2.18117455557065));
#43030=CARTESIAN_POINT('Ctrl Pts',(-3.29920022557639,1.,2.18710556500327));
#43031=CARTESIAN_POINT('Ctrl Pts',(-3.30385816281831,1.,2.19306710376111));
#43032=CARTESIAN_POINT('Ctrl Pts',(-3.30848134694595,1.,2.19906078949923));
#43033=CARTESIAN_POINT('Ctrl Pts',(-3.31307424608949,1.,2.20508863150607));
#43034=CARTESIAN_POINT('Ctrl Pts',(-3.31764044024235,1.,2.21115211847875));
#43035=CARTESIAN_POINT('Ctrl Pts',(-3.32218125618968,1.,2.21725135110898));
#43036=CARTESIAN_POINT('Ctrl Pts',(-3.3266964672289,1.,2.22338548312772));
#43037=CARTESIAN_POINT('Ctrl Pts',(-3.33118487773611,1.,2.22955308907233));
#43038=CARTESIAN_POINT('Ctrl Pts',(-3.33564495756482,1.,2.23575256328812));
#43039=CARTESIAN_POINT('Ctrl Pts',(-3.34007543738025,1.,2.24198249391422));
#43040=CARTESIAN_POINT('Ctrl Pts',(-3.34447596770723,1.,2.24824207678256));
#43041=CARTESIAN_POINT('Ctrl Pts',(-3.34884690292285,1.,2.25453097693483));
#43042=CARTESIAN_POINT('Ctrl Pts',(-3.35318902552626,1.,2.26084915222449));
#43043=CARTESIAN_POINT('Ctrl Pts',(-3.35750328523061,1.,2.2671966857991));
#43044=CARTESIAN_POINT('Ctrl Pts',(-3.36179055004409,1.,2.2735736262093));
#43045=CARTESIAN_POINT('Ctrl Pts',(-3.36605130713076,1.,2.27997979458037));
#43046=CARTESIAN_POINT('Ctrl Pts',(-3.37028570206488,1.,2.28641481081137));
#43047=CARTESIAN_POINT('Ctrl Pts',(-3.37449367172826,1.,2.29287818007393));
#43048=CARTESIAN_POINT('Ctrl Pts',(-3.37867504959433,1.,2.29936936127624));
#43049=CARTESIAN_POINT('Ctrl Pts',(-3.3828296733661,1.,2.30588783640343));
#43050=CARTESIAN_POINT('Ctrl Pts',(-3.38695751492462,1.,2.31243319489367));
#43051=CARTESIAN_POINT('Ctrl Pts',(-3.39105869474822,1.,2.31900513925424));
#43052=CARTESIAN_POINT('Ctrl Pts',(-3.39513342019756,1.,2.3256034390248));
#43053=CARTESIAN_POINT('Ctrl Pts',(-3.39918194577956,1.,2.33222789882489));
#43054=CARTESIAN_POINT('Ctrl Pts',(-3.40320452776743,1.,2.33887832342782));
#43055=CARTESIAN_POINT('Ctrl Pts',(-3.40720137404297,1.,2.34555447649188));
#43056=CARTESIAN_POINT('Ctrl Pts',(-3.41117262314119,1.,2.35225606824109));
#43057=CARTESIAN_POINT('Ctrl Pts',(-3.41511836751469,1.,2.35898278606946));
#43058=CARTESIAN_POINT('Ctrl Pts',(-3.41903866635852,1.,2.36573431470642));
#43059=CARTESIAN_POINT('Ctrl Pts',(-3.42293356216511,1.,2.37251035954292));
#43060=CARTESIAN_POINT('Ctrl Pts',(-3.42680309754399,1.,2.37931067028926));
#43061=CARTESIAN_POINT('Ctrl Pts',(-3.4306473271292,1.,2.38613505843552));
#43062=CARTESIAN_POINT('Ctrl Pts',(-3.4344663067854,1.,2.39298338804493));
#43063=CARTESIAN_POINT('Ctrl Pts',(-3.43750133064416,1.,2.39848113410292));
#43064=CARTESIAN_POINT('Ctrl Pts',(-3.43976627484234,1.,2.40261515589405));
#43065=CARTESIAN_POINT('Ctrl Pts',(-3.44127120683039,1.,2.4053759295909));
#43066=CARTESIAN_POINT('Ctrl Pts',(-3.44202241512147,1.,2.40675750623143));
#43067=CARTESIAN_POINT('Origin',(-3.44202241512147,0.,2.40675750623143));
#43068=CARTESIAN_POINT('',(-3.35260583073571,1.,2.52982887637028));
#43069=CARTESIAN_POINT('Origin',(0.,0.,0.));
#43070=CARTESIAN_POINT('',(-3.24413672884812,1.,1.88097764062697));
#43071=CARTESIAN_POINT('Origin',(0.,1.,0.));
#43072=CARTESIAN_POINT('Ctrl Pts',(-3.24413672884812,1.,1.88097764062697));
#43073=CARTESIAN_POINT('Ctrl Pts',(-3.24413672884812,0.666666666666667,
1.88097764062697));
#43074=CARTESIAN_POINT('Ctrl Pts',(-3.24413672884812,0.333333333333333,
1.88097764062697));
#43075=CARTESIAN_POINT('Ctrl Pts',(-3.24413672884812,-0.333333333333333,
1.88097764062697));
#43076=CARTESIAN_POINT('Ctrl Pts',(-3.24413672884812,-0.666666666666667,
1.88097764062697));
#43077=CARTESIAN_POINT('Ctrl Pts',(-3.24413672884812,-1.,1.88097764062697));
#43078=CARTESIAN_POINT('Ctrl Pts',(-3.70708211654725,-1.,1.97421938526992));
#43079=CARTESIAN_POINT('Ctrl Pts',(-3.70708211654725,1.,1.97421938526992));
#43080=CARTESIAN_POINT('Ctrl Pts',(-3.70551008132332,-1.,1.97417727645308));
#43081=CARTESIAN_POINT('Ctrl Pts',(-3.70551008132332,1.,1.97417727645308));
#43082=CARTESIAN_POINT('Ctrl Pts',(-3.70236698912904,-1.,1.97408973726715));
#43083=CARTESIAN_POINT('Ctrl Pts',(-3.70236698912904,1.,1.97408973726715));
#43084=CARTESIAN_POINT('Ctrl Pts',(-3.6976552856004,-1.,1.97394846383216));
#43085=CARTESIAN_POINT('Ctrl Pts',(-3.6976552856004,1.,1.97394846383216));
#43086=CARTESIAN_POINT('Ctrl Pts',(-3.69137888599902,-1.,1.97374016225483));
#43087=CARTESIAN_POINT('Ctrl Pts',(-3.69137888599902,1.,1.97374016225483));
#43088=CARTESIAN_POINT('Ctrl Pts',(-3.68354319915092,-1.,1.97344650304519));
#43089=CARTESIAN_POINT('Ctrl Pts',(-3.68354319915092,1.,1.97344650304519));
#43090=CARTESIAN_POINT('Ctrl Pts',(-3.67571738107084,-1.,1.97311947678516));
#43091=CARTESIAN_POINT('Ctrl Pts',(-3.67571738107084,1.,1.97311947678516));
#43092=CARTESIAN_POINT('Ctrl Pts',(-3.66790152752075,-1.,1.97275897198678));
#43093=CARTESIAN_POINT('Ctrl Pts',(-3.66790152752075,1.,1.97275897198678));
#43094=CARTESIAN_POINT('Ctrl Pts',(-3.6600957816636,-1.,1.9723648543905));
#43095=CARTESIAN_POINT('Ctrl Pts',(-3.6600957816636,1.,1.9723648543905));
#43096=CARTESIAN_POINT('Ctrl Pts',(-3.652300347166,-1.,1.9719369724024));
#43097=CARTESIAN_POINT('Ctrl Pts',(-3.652300347166,1.,1.9719369724024));
#43098=CARTESIAN_POINT('Ctrl Pts',(-3.64451546723514,-1.,1.97147515441164));
#43099=CARTESIAN_POINT('Ctrl Pts',(-3.64451546723514,1.,1.97147515441164));
#43100=CARTESIAN_POINT('Ctrl Pts',(-3.63674139590412,-1.,1.97097920454464));
#43101=CARTESIAN_POINT('Ctrl Pts',(-3.63674139590412,1.,1.97097920454464));
#43102=CARTESIAN_POINT('Ctrl Pts',(-3.62897836973293,-1.,1.97044889850463));
#43103=CARTESIAN_POINT('Ctrl Pts',(-3.62897836973293,1.,1.97044889850463));
#43104=CARTESIAN_POINT('Ctrl Pts',(-3.62122658401893,-1.,1.96988398129978));
#43105=CARTESIAN_POINT('Ctrl Pts',(-3.62122658401893,1.,1.96988398129978));
#43106=CARTESIAN_POINT('Ctrl Pts',(-3.61348615496704,-1.,1.96928416040877));
#43107=CARTESIAN_POINT('Ctrl Pts',(-3.61348615496704,1.,1.96928416040877));
#43108=CARTESIAN_POINT('Ctrl Pts',(-3.60575714017989,-1.,1.9686491188594));
#43109=CARTESIAN_POINT('Ctrl Pts',(-3.60575714017989,1.,1.9686491188594));
#43110=CARTESIAN_POINT('Ctrl Pts',(-3.59803959819938,-1.,1.96797854118369));
#43111=CARTESIAN_POINT('Ctrl Pts',(-3.59803959819938,1.,1.96797854118369));
#43112=CARTESIAN_POINT('Ctrl Pts',(-3.59033364022801,-1.,1.96727213799544));
#43113=CARTESIAN_POINT('Ctrl Pts',(-3.59033364022801,1.,1.96727213799544));
#43114=CARTESIAN_POINT('Ctrl Pts',(-3.58263947663829,-1.,1.96652966688911));
#43115=CARTESIAN_POINT('Ctrl Pts',(-3.58263947663829,1.,1.96652966688911));
#43116=CARTESIAN_POINT('Ctrl Pts',(-3.57495748600959,-1.,1.96575096652789));
#43117=CARTESIAN_POINT('Ctrl Pts',(-3.57495748600959,1.,1.96575096652789));
#43118=CARTESIAN_POINT('Ctrl Pts',(-3.56728820357791,-1.,1.96493594634567));
#43119=CARTESIAN_POINT('Ctrl Pts',(-3.56728820357791,1.,1.96493594634567));
#43120=CARTESIAN_POINT('Ctrl Pts',(-3.55963218706096,-1.,1.96408450906812));
#43121=CARTESIAN_POINT('Ctrl Pts',(-3.55963218706096,1.,1.96408450906812));
#43122=CARTESIAN_POINT('Ctrl Pts',(-3.55198990600886,-1.,1.96319648628644));
#43123=CARTESIAN_POINT('Ctrl Pts',(-3.55198990600886,1.,1.96319648628644));
#43124=CARTESIAN_POINT('Ctrl Pts',(-3.54436163300443,-1.,1.96227157573067));
#43125=CARTESIAN_POINT('Ctrl Pts',(-3.54436163300443,1.,1.96227157573067));
#43126=CARTESIAN_POINT('Ctrl Pts',(-3.53674730625813,-1.,1.96130926212689));
#43127=CARTESIAN_POINT('Ctrl Pts',(-3.53674730625813,1.,1.96130926212689));
#43128=CARTESIAN_POINT('Ctrl Pts',(-3.52914648844351,-1.,1.96030879411566));
#43129=CARTESIAN_POINT('Ctrl Pts',(-3.52914648844351,1.,1.96030879411566));
#43130=CARTESIAN_POINT('Ctrl Pts',(-3.52155867431486,-1.,1.95926936324461));
#43131=CARTESIAN_POINT('Ctrl Pts',(-3.52155867431486,1.,1.95926936324461));
#43132=CARTESIAN_POINT('Ctrl Pts',(-3.51398354617794,-1.,1.95819025316779));
#43133=CARTESIAN_POINT('Ctrl Pts',(-3.51398354617794,1.,1.95819025316779));
#43134=CARTESIAN_POINT('Ctrl Pts',(-3.50642124159909,-1.,1.95707099606511));
#43135=CARTESIAN_POINT('Ctrl Pts',(-3.50642124159909,1.,1.95707099606511));
#43136=CARTESIAN_POINT('Ctrl Pts',(-3.49887263575583,-1.,1.95591153823661));
#43137=CARTESIAN_POINT('Ctrl Pts',(-3.49887263575583,1.,1.95591153823661));
#43138=CARTESIAN_POINT('Ctrl Pts',(-3.49133956289133,-1.,1.95471236969643));
#43139=CARTESIAN_POINT('Ctrl Pts',(-3.49133956289133,1.,1.95471236969643));
#43140=CARTESIAN_POINT('Ctrl Pts',(-3.48382414832634,-1.,1.95347412486308));
#43141=CARTESIAN_POINT('Ctrl Pts',(-3.48382414832634,1.,1.95347412486308));
#43142=CARTESIAN_POINT('Ctrl Pts',(-3.47632820495921,-1.,1.95219722189876));
#43143=CARTESIAN_POINT('Ctrl Pts',(-3.47632820495921,1.,1.95219722189876));
#43144=CARTESIAN_POINT('Ctrl Pts',(-3.46885258974191,-1.,1.95088147859876));
#43145=CARTESIAN_POINT('Ctrl Pts',(-3.46885258974191,1.,1.95088147859876));
#43146=CARTESIAN_POINT('Ctrl Pts',(-3.46139661060962,-1.,1.94952575850197));
#43147=CARTESIAN_POINT('Ctrl Pts',(-3.46139661060962,1.,1.94952575850197));
#43148=CARTESIAN_POINT('Ctrl Pts',(-3.45395731584051,-1.,1.94812754766524));
#43149=CARTESIAN_POINT('Ctrl Pts',(-3.45395731584051,1.,1.94812754766524));
#43150=CARTESIAN_POINT('Ctrl Pts',(-3.44653088665681,-1.,1.94668377715329));
#43151=CARTESIAN_POINT('Ctrl Pts',(-3.44653088665681,1.,1.94668377715329));
#43152=CARTESIAN_POINT('Ctrl Pts',(-3.43911410197687,-1.,1.94519168842879));
#43153=CARTESIAN_POINT('Ctrl Pts',(-3.43911410197687,1.,1.94519168842879));
#43154=CARTESIAN_POINT('Ctrl Pts',(-3.43170586602434,-1.,1.94364973660284));
#43155=CARTESIAN_POINT('Ctrl Pts',(-3.43170586602434,1.,1.94364973660284));
#43156=CARTESIAN_POINT('Ctrl Pts',(-3.42430850941503,-1.,1.94205835913696));
#43157=CARTESIAN_POINT('Ctrl Pts',(-3.42430850941503,1.,1.94205835913696));
#43158=CARTESIAN_POINT('Ctrl Pts',(-3.41692971994096,-1.,1.94042111965246));
#43159=CARTESIAN_POINT('Ctrl Pts',(-3.41692971994096,1.,1.94042111965246));
#43160=CARTESIAN_POINT('Ctrl Pts',(-3.40957978266642,-1.,1.93874306008143));
#43161=CARTESIAN_POINT('Ctrl Pts',(-3.40957978266642,1.,1.93874306008143));
#43162=CARTESIAN_POINT('Ctrl Pts',(-3.40226802104109,-1.,1.93702857723098));
#43163=CARTESIAN_POINT('Ctrl Pts',(-3.40226802104109,1.,1.93702857723098));
#43164=CARTESIAN_POINT('Ctrl Pts',(-3.39499923640795,-1.,1.93527929945985));
#43165=CARTESIAN_POINT('Ctrl Pts',(-3.39499923640795,1.,1.93527929945985));
#43166=CARTESIAN_POINT('Ctrl Pts',(-3.38777076883256,-1.,1.93349233176788));
#43167=CARTESIAN_POINT('Ctrl Pts',(-3.38777076883256,1.,1.93349233176788));
#43168=CARTESIAN_POINT('Ctrl Pts',(-3.3805676852555,-1.,1.93165739093276));
#43169=CARTESIAN_POINT('Ctrl Pts',(-3.3805676852555,1.,1.93165739093276));
#43170=CARTESIAN_POINT('Ctrl Pts',(-3.37336807068043,-1.,1.92975993109877));
#43171=CARTESIAN_POINT('Ctrl Pts',(-3.37336807068043,1.,1.92975993109877));
#43172=CARTESIAN_POINT('Ctrl Pts',(-3.36615168657567,-1.,1.92778626543786));
#43173=CARTESIAN_POINT('Ctrl Pts',(-3.36615168657567,1.,1.92778626543786));
#43174=CARTESIAN_POINT('Ctrl Pts',(-3.35890824422965,-1.,1.92572846125756));
#43175=CARTESIAN_POINT('Ctrl Pts',(-3.35890824422965,1.,1.92572846125756));
#43176=CARTESIAN_POINT('Ctrl Pts',(-3.35164424847223,-1.,1.92358838440528));
#43177=CARTESIAN_POINT('Ctrl Pts',(-3.35164424847223,1.,1.92358838440528));
#43178=CARTESIAN_POINT('Ctrl Pts',(-3.34439448941961,-1.,1.92138450828404));
#43179=CARTESIAN_POINT('Ctrl Pts',(-3.34439448941961,1.,1.92138450828404));
#43180=CARTESIAN_POINT('Ctrl Pts',(-3.33721230710012,-1.,1.9191460961021));
#43181=CARTESIAN_POINT('Ctrl Pts',(-3.33721230710012,1.,1.9191460961021));
#43182=CARTESIAN_POINT('Ctrl Pts',(-3.33014884257873,-1.,1.91690081930331));
#43183=CARTESIAN_POINT('Ctrl Pts',(-3.33014884257873,1.,1.91690081930331));
#43184=CARTESIAN_POINT('Ctrl Pts',(-3.32323403454535,-1.,1.91466343916628));
#43185=CARTESIAN_POINT('Ctrl Pts',(-3.32323403454535,1.,1.91466343916628));
#43186=CARTESIAN_POINT('Ctrl Pts',(-3.31646052426364,-1.,1.91242616234442));
#43187=CARTESIAN_POINT('Ctrl Pts',(-3.31646052426364,1.,1.91242616234442));
#43188=CARTESIAN_POINT('Ctrl Pts',(-3.30975721158596,-1.,1.91014297830446));
#43189=CARTESIAN_POINT('Ctrl Pts',(-3.30975721158596,1.,1.91014297830446));
#43190=CARTESIAN_POINT('Ctrl Pts',(-3.30300595568195,-1.,1.90773912171341));
#43191=CARTESIAN_POINT('Ctrl Pts',(-3.30300595568195,1.,1.90773912171341));
#43192=CARTESIAN_POINT('Ctrl Pts',(-3.29608978722113,-1.,1.90513891864087));
#43193=CARTESIAN_POINT('Ctrl Pts',(-3.29608978722113,1.,1.90513891864087));
#43194=CARTESIAN_POINT('Ctrl Pts',(-3.2889344860029,-1.,1.90228971247527));
#43195=CARTESIAN_POINT('Ctrl Pts',(-3.2889344860029,1.,1.90228971247527));
#43196=CARTESIAN_POINT('Ctrl Pts',(-3.28154737912352,-1.,1.89918429230462));
#43197=CARTESIAN_POINT('Ctrl Pts',(-3.28154737912352,1.,1.89918429230462));
#43198=CARTESIAN_POINT('Ctrl Pts',(-3.27407108933139,-1.,1.89589172903793));
#43199=CARTESIAN_POINT('Ctrl Pts',(-3.27407108933139,1.,1.89589172903793));
#43200=CARTESIAN_POINT('Ctrl Pts',(-3.26677653888676,-1.,1.89255393500965));
#43201=CARTESIAN_POINT('Ctrl Pts',(-3.26677653888676,1.,1.89255393500965));
#43202=CARTESIAN_POINT('Ctrl Pts',(-3.25999885193947,-1.,1.88934996203698));
#43203=CARTESIAN_POINT('Ctrl Pts',(-3.25999885193947,1.,1.88934996203698));
#43204=CARTESIAN_POINT('Ctrl Pts',(-3.25408686339463,-1.,1.88646802523466));
#43205=CARTESIAN_POINT('Ctrl Pts',(-3.25408686339463,1.,1.88646802523466));
#43206=CARTESIAN_POINT('Ctrl Pts',(-3.24935200511918,-1.,1.88407708646357));
#43207=CARTESIAN_POINT('Ctrl Pts',(-3.24935200511918,1.,1.88407708646357));
#43208=CARTESIAN_POINT('Ctrl Pts',(-3.24600543790443,-1.,1.88229202582941));
#43209=CARTESIAN_POINT('Ctrl Pts',(-3.24600543790443,1.,1.88229202582941));
#43210=CARTESIAN_POINT('Ctrl Pts',(-3.24451807186481,-1.,1.88139187908074));
#43211=CARTESIAN_POINT('Ctrl Pts',(-3.24451807186481,1.,1.88139187908074));
#43212=CARTESIAN_POINT('Ctrl Pts',(-3.24408699284121,-1.,1.88102201872555));
#43213=CARTESIAN_POINT('Ctrl Pts',(-3.24408699284121,1.,1.88102201872555));
#43214=CARTESIAN_POINT('Ctrl Pts',(-3.24410359189609,-1.,1.88091100680349));
#43215=CARTESIAN_POINT('Ctrl Pts',(-3.24410359189609,1.,1.88091100680349));
#43216=CARTESIAN_POINT('Ctrl Pts',(-3.24418789321065,-1.,1.8808893942881));
#43217=CARTESIAN_POINT('Ctrl Pts',(-3.24418789321065,1.,1.8808893942881));
#43218=CARTESIAN_POINT('',(-3.70708211654725,1.,1.97421938526992));
#43219=CARTESIAN_POINT('Ctrl Pts',(-3.70708211654725,1.,1.97421938526992));
#43220=CARTESIAN_POINT('Ctrl Pts',(-3.70551008132332,1.,1.97417727645308));
#43221=CARTESIAN_POINT('Ctrl Pts',(-3.70236698912904,1.,1.97408973726715));
#43222=CARTESIAN_POINT('Ctrl Pts',(-3.6976552856004,1.,1.97394846383216));
#43223=CARTESIAN_POINT('Ctrl Pts',(-3.69137888599902,1.,1.97374016225483));
#43224=CARTESIAN_POINT('Ctrl Pts',(-3.68354319915092,1.,1.97344650304519));
#43225=CARTESIAN_POINT('Ctrl Pts',(-3.67571738107084,1.,1.97311947678516));
#43226=CARTESIAN_POINT('Ctrl Pts',(-3.66790152752075,1.,1.97275897198678));
#43227=CARTESIAN_POINT('Ctrl Pts',(-3.6600957816636,1.,1.9723648543905));
#43228=CARTESIAN_POINT('Ctrl Pts',(-3.652300347166,1.,1.9719369724024));
#43229=CARTESIAN_POINT('Ctrl Pts',(-3.64451546723514,1.,1.97147515441164));
#43230=CARTESIAN_POINT('Ctrl Pts',(-3.63674139590412,1.,1.97097920454464));
#43231=CARTESIAN_POINT('Ctrl Pts',(-3.62897836973293,1.,1.97044889850463));
#43232=CARTESIAN_POINT('Ctrl Pts',(-3.62122658401893,1.,1.96988398129978));
#43233=CARTESIAN_POINT('Ctrl Pts',(-3.61348615496704,1.,1.96928416040877));
#43234=CARTESIAN_POINT('Ctrl Pts',(-3.60575714017989,1.,1.9686491188594));
#43235=CARTESIAN_POINT('Ctrl Pts',(-3.59803959819938,1.,1.96797854118369));
#43236=CARTESIAN_POINT('Ctrl Pts',(-3.59033364022801,1.,1.96727213799544));
#43237=CARTESIAN_POINT('Ctrl Pts',(-3.58263947663829,1.,1.96652966688911));
#43238=CARTESIAN_POINT('Ctrl Pts',(-3.57495748600959,1.,1.96575096652789));
#43239=CARTESIAN_POINT('Ctrl Pts',(-3.56728820357791,1.,1.96493594634567));
#43240=CARTESIAN_POINT('Ctrl Pts',(-3.55963218706096,1.,1.96408450906812));
#43241=CARTESIAN_POINT('Ctrl Pts',(-3.55198990600886,1.,1.96319648628644));
#43242=CARTESIAN_POINT('Ctrl Pts',(-3.54436163300443,1.,1.96227157573067));
#43243=CARTESIAN_POINT('Ctrl Pts',(-3.53674730625813,1.,1.96130926212689));
#43244=CARTESIAN_POINT('Ctrl Pts',(-3.52914648844351,1.,1.96030879411566));
#43245=CARTESIAN_POINT('Ctrl Pts',(-3.52155867431486,1.,1.95926936324461));
#43246=CARTESIAN_POINT('Ctrl Pts',(-3.51398354617794,1.,1.95819025316779));
#43247=CARTESIAN_POINT('Ctrl Pts',(-3.50642124159909,1.,1.95707099606511));
#43248=CARTESIAN_POINT('Ctrl Pts',(-3.49887263575583,1.,1.95591153823661));
#43249=CARTESIAN_POINT('Ctrl Pts',(-3.49133956289133,1.,1.95471236969643));
#43250=CARTESIAN_POINT('Ctrl Pts',(-3.48382414832634,1.,1.95347412486308));
#43251=CARTESIAN_POINT('Ctrl Pts',(-3.47632820495921,1.,1.95219722189876));
#43252=CARTESIAN_POINT('Ctrl Pts',(-3.46885258974191,1.,1.95088147859876));
#43253=CARTESIAN_POINT('Ctrl Pts',(-3.46139661060962,1.,1.94952575850197));
#43254=CARTESIAN_POINT('Ctrl Pts',(-3.45395731584051,1.,1.94812754766524));
#43255=CARTESIAN_POINT('Ctrl Pts',(-3.44653088665681,1.,1.94668377715329));
#43256=CARTESIAN_POINT('Ctrl Pts',(-3.43911410197687,1.,1.94519168842879));
#43257=CARTESIAN_POINT('Ctrl Pts',(-3.43170586602434,1.,1.94364973660284));
#43258=CARTESIAN_POINT('Ctrl Pts',(-3.42430850941503,1.,1.94205835913696));
#43259=CARTESIAN_POINT('Ctrl Pts',(-3.41692971994096,1.,1.94042111965246));
#43260=CARTESIAN_POINT('Ctrl Pts',(-3.40957978266642,1.,1.93874306008143));
#43261=CARTESIAN_POINT('Ctrl Pts',(-3.40226802104109,1.,1.93702857723098));
#43262=CARTESIAN_POINT('Ctrl Pts',(-3.39499923640795,1.,1.93527929945985));
#43263=CARTESIAN_POINT('Ctrl Pts',(-3.38777076883256,1.,1.93349233176788));
#43264=CARTESIAN_POINT('Ctrl Pts',(-3.3805676852555,1.,1.93165739093276));
#43265=CARTESIAN_POINT('Ctrl Pts',(-3.37336807068043,1.,1.92975993109877));
#43266=CARTESIAN_POINT('Ctrl Pts',(-3.36615168657567,1.,1.92778626543786));
#43267=CARTESIAN_POINT('Ctrl Pts',(-3.35890824422965,1.,1.92572846125756));
#43268=CARTESIAN_POINT('Ctrl Pts',(-3.35164424847223,1.,1.92358838440528));
#43269=CARTESIAN_POINT('Ctrl Pts',(-3.34439448941961,1.,1.92138450828404));
#43270=CARTESIAN_POINT('Ctrl Pts',(-3.33721230710012,1.,1.9191460961021));
#43271=CARTESIAN_POINT('Ctrl Pts',(-3.33014884257873,1.,1.91690081930331));
#43272=CARTESIAN_POINT('Ctrl Pts',(-3.32323403454535,1.,1.91466343916628));
#43273=CARTESIAN_POINT('Ctrl Pts',(-3.31646052426364,1.,1.91242616234442));
#43274=CARTESIAN_POINT('Ctrl Pts',(-3.30975721158596,1.,1.91014297830446));
#43275=CARTESIAN_POINT('Ctrl Pts',(-3.30300595568195,1.,1.90773912171341));
#43276=CARTESIAN_POINT('Ctrl Pts',(-3.29608978722113,1.,1.90513891864087));
#43277=CARTESIAN_POINT('Ctrl Pts',(-3.2889344860029,1.,1.90228971247527));
#43278=CARTESIAN_POINT('Ctrl Pts',(-3.28154737912352,1.,1.89918429230462));
#43279=CARTESIAN_POINT('Ctrl Pts',(-3.27407108933139,1.,1.89589172903793));
#43280=CARTESIAN_POINT('Ctrl Pts',(-3.26677653888676,1.,1.89255393500965));
#43281=CARTESIAN_POINT('Ctrl Pts',(-3.25999885193947,1.,1.88934996203698));
#43282=CARTESIAN_POINT('Ctrl Pts',(-3.25408686339463,1.,1.88646802523466));
#43283=CARTESIAN_POINT('Ctrl Pts',(-3.24935200511918,1.,1.88407708646357));
#43284=CARTESIAN_POINT('Ctrl Pts',(-3.2462565441079,1.,1.88242596600454));
#43285=CARTESIAN_POINT('Ctrl Pts',(-3.24480754676064,1.,1.88156537699203));
#43286=CARTESIAN_POINT('Ctrl Pts',(-3.24428080353022,1.,1.88117508446775));
#43287=CARTESIAN_POINT('Ctrl Pts',(-3.24415531671284,1.,1.8810229239812));
#43288=CARTESIAN_POINT('Ctrl Pts',(-3.24413672884812,1.,1.88097764062697));
#43289=CARTESIAN_POINT('',(-3.70708211654725,0.,1.97421938526992));
#43290=CARTESIAN_POINT('Ctrl Pts',(-3.42855728381368,-1.,1.519044091397));
#43291=CARTESIAN_POINT('Ctrl Pts',(-3.42855728381368,1.,1.519044091397));
#43292=CARTESIAN_POINT('Ctrl Pts',(-3.42852521763778,-1.,1.51896318668366));
#43293=CARTESIAN_POINT('Ctrl Pts',(-3.42852521763778,1.,1.51896318668366));
#43294=CARTESIAN_POINT('Ctrl Pts',(-3.42860527149177,-1.,1.51888450659652));
#43295=CARTESIAN_POINT('Ctrl Pts',(-3.42860527149177,1.,1.51888450659652));
#43296=CARTESIAN_POINT('Ctrl Pts',(-3.42915787669893,-1.,1.51901585839109));
#43297=CARTESIAN_POINT('Ctrl Pts',(-3.42915787669893,1.,1.51901585839109));
#43298=CARTESIAN_POINT('Ctrl Pts',(-3.43076036253837,-1.,1.51969006980999));
#43299=CARTESIAN_POINT('Ctrl Pts',(-3.43076036253837,1.,1.51969006980999));
#43300=CARTESIAN_POINT('Ctrl Pts',(-3.43417156977893,-1.,1.52134826724292));
#43301=CARTESIAN_POINT('Ctrl Pts',(-3.43417156977893,1.,1.52134826724292));
#43302=CARTESIAN_POINT('Ctrl Pts',(-3.4388889597401,-1.,1.5237734895035));
#43303=CARTESIAN_POINT('Ctrl Pts',(-3.4388889597401,1.,1.5237734895035));
#43304=CARTESIAN_POINT('Ctrl Pts',(-3.44469547526647,-1.,1.52686242875556));
#43305=CARTESIAN_POINT('Ctrl Pts',(-3.44469547526647,1.,1.52686242875556));
#43306=CARTESIAN_POINT('Ctrl Pts',(-3.45127136828305,-1.,1.53046244461635));
#43307=CARTESIAN_POINT('Ctrl Pts',(-3.45127136828305,1.,1.53046244461635));
#43308=CARTESIAN_POINT('Ctrl Pts',(-3.45825932955032,-1.,1.53440195378792));
#43309=CARTESIAN_POINT('Ctrl Pts',(-3.45825932955032,1.,1.53440195378792));
#43310=CARTESIAN_POINT('Ctrl Pts',(-3.46531752207153,-1.,1.53851507915502));
#43311=CARTESIAN_POINT('Ctrl Pts',(-3.46531752207153,1.,1.53851507915502));
#43312=CARTESIAN_POINT('Ctrl Pts',(-3.47217189224653,-1.,1.54266605398187));
#43313=CARTESIAN_POINT('Ctrl Pts',(-3.47217189224653,1.,1.54266605398187));
#43314=CARTESIAN_POINT('Ctrl Pts',(-3.47868272898751,-1.,1.54678009290276));
#43315=CARTESIAN_POINT('Ctrl Pts',(-3.47868272898751,1.,1.54678009290276));
#43316=CARTESIAN_POINT('Ctrl Pts',(-3.48485155928567,-1.,1.55084702970452));
#43317=CARTESIAN_POINT('Ctrl Pts',(-3.48485155928567,1.,1.55084702970452));
#43318=CARTESIAN_POINT('Ctrl Pts',(-3.4907646087742,-1.,1.55489595901116));
#43319=CARTESIAN_POINT('Ctrl Pts',(-3.4907646087742,1.,1.55489595901116));
#43320=CARTESIAN_POINT('Ctrl Pts',(-3.49655185179655,-1.,1.55897703097874));
#43321=CARTESIAN_POINT('Ctrl Pts',(-3.49655185179655,1.,1.55897703097874));
#43322=CARTESIAN_POINT('Ctrl Pts',(-3.50234321621578,-1.,1.56314187758675));
#43323=CARTESIAN_POINT('Ctrl Pts',(-3.50234321621578,1.,1.56314187758675));
#43324=CARTESIAN_POINT('Ctrl Pts',(-3.50821771695363,-1.,1.56742097575012));
#43325=CARTESIAN_POINT('Ctrl Pts',(-3.50821771695363,1.,1.56742097575012));
#43326=CARTESIAN_POINT('Ctrl Pts',(-3.51418598431665,-1.,1.57181569799743));
#43327=CARTESIAN_POINT('Ctrl Pts',(-3.51418598431665,1.,1.57181569799743));
#43328=CARTESIAN_POINT('Ctrl Pts',(-3.52021847865912,-1.,1.57631049988158));
#43329=CARTESIAN_POINT('Ctrl Pts',(-3.52021847865912,1.,1.57631049988158));
#43330=CARTESIAN_POINT('Ctrl Pts',(-3.52626275334881,-1.,1.58088027227848));
#43331=CARTESIAN_POINT('Ctrl Pts',(-3.52626275334881,1.,1.58088027227848));
#43332=CARTESIAN_POINT('Ctrl Pts',(-3.5322637814708,-1.,1.58549906268088));
#43333=CARTESIAN_POINT('Ctrl Pts',(-3.5322637814708,1.,1.58549906268088));
#43334=CARTESIAN_POINT('Ctrl Pts',(-3.53818616861077,-1.,1.59014958368739));
#43335=CARTESIAN_POINT('Ctrl Pts',(-3.53818616861077,1.,1.59014958368739));
#43336=CARTESIAN_POINT('Ctrl Pts',(-3.54402458182337,-1.,1.59482766949766));
#43337=CARTESIAN_POINT('Ctrl Pts',(-3.54402458182337,1.,1.59482766949766));
#43338=CARTESIAN_POINT('Ctrl Pts',(-3.54979148634454,-1.,1.59953698113457));
#43339=CARTESIAN_POINT('Ctrl Pts',(-3.54979148634454,1.,1.59953698113457));
#43340=CARTESIAN_POINT('Ctrl Pts',(-3.55550985096129,-1.,1.60428584699853));
#43341=CARTESIAN_POINT('Ctrl Pts',(-3.55550985096129,1.,1.60428584699853));
#43342=CARTESIAN_POINT('Ctrl Pts',(-3.5612043248298,-1.,1.60908344685457));
#43343=CARTESIAN_POINT('Ctrl Pts',(-3.5612043248298,1.,1.60908344685457));
#43344=CARTESIAN_POINT('Ctrl Pts',(-3.56689200468387,-1.,1.61393581747514));
#43345=CARTESIAN_POINT('Ctrl Pts',(-3.56689200468387,1.,1.61393581747514));
#43346=CARTESIAN_POINT('Ctrl Pts',(-3.57257679609806,-1.,1.61884340915404));
#43347=CARTESIAN_POINT('Ctrl Pts',(-3.57257679609806,1.,1.61884340915404));
#43348=CARTESIAN_POINT('Ctrl Pts',(-3.5782545595439,-1.,1.62380329464844));
#43349=CARTESIAN_POINT('Ctrl Pts',(-3.5782545595439,1.,1.62380329464844));
#43350=CARTESIAN_POINT('Ctrl Pts',(-3.58391625774343,-1.,1.62881051550745));
#43351=CARTESIAN_POINT('Ctrl Pts',(-3.58391625774343,1.,1.62881051550745));
#43352=CARTESIAN_POINT('Ctrl Pts',(-3.58955176627879,-1.,1.6338597145126));
#43353=CARTESIAN_POINT('Ctrl Pts',(-3.58955176627879,1.,1.6338597145126));
#43354=CARTESIAN_POINT('Ctrl Pts',(-3.59515368334893,-1.,1.63894676675352));
#43355=CARTESIAN_POINT('Ctrl Pts',(-3.59515368334893,1.,1.63894676675352));
#43356=CARTESIAN_POINT('Ctrl Pts',(-3.60072028513845,-1.,1.64407004385582));
#43357=CARTESIAN_POINT('Ctrl Pts',(-3.60072028513845,1.,1.64407004385582));
#43358=CARTESIAN_POINT('Ctrl Pts',(-3.60625346556992,-1.,1.64922952425832));
#43359=CARTESIAN_POINT('Ctrl Pts',(-3.60625346556992,1.,1.64922952425832));
#43360=CARTESIAN_POINT('Ctrl Pts',(-3.61175734965127,-1.,1.65442619244325));
#43361=CARTESIAN_POINT('Ctrl Pts',(-3.61175734965127,1.,1.65442619244325));
#43362=CARTESIAN_POINT('Ctrl Pts',(-3.61723666482456,-1.,1.65966133399186));
#43363=CARTESIAN_POINT('Ctrl Pts',(-3.61723666482456,1.,1.65966133399186));
#43364=CARTESIAN_POINT('Ctrl Pts',(-3.62269517989109,-1.,1.66493585923855));
#43365=CARTESIAN_POINT('Ctrl Pts',(-3.62269517989109,1.,1.66493585923855));
#43366=CARTESIAN_POINT('Ctrl Pts',(-3.62813422105271,-1.,1.67024966008045));
#43367=CARTESIAN_POINT('Ctrl Pts',(-3.62813422105271,1.,1.67024966008045));
#43368=CARTESIAN_POINT('Ctrl Pts',(-3.63355343201232,-1.,1.67560193613156));
#43369=CARTESIAN_POINT('Ctrl Pts',(-3.63355343201232,1.,1.67560193613156));
#43370=CARTESIAN_POINT('Ctrl Pts',(-3.63895140887462,-1.,1.68099146651586));
#43371=CARTESIAN_POINT('Ctrl Pts',(-3.63895140887462,1.,1.68099146651586));
#43372=CARTESIAN_POINT('Ctrl Pts',(-3.64432638915203,-1.,1.68641690471457));
#43373=CARTESIAN_POINT('Ctrl Pts',(-3.64432638915203,1.,1.68641690471457));
#43374=CARTESIAN_POINT('Ctrl Pts',(-3.64967689827371,-1.,1.69187705481689));
#43375=CARTESIAN_POINT('Ctrl Pts',(-3.64967689827371,1.,1.69187705481689));
#43376=CARTESIAN_POINT('Ctrl Pts',(-3.65500246526749,-1.,1.69737117722534));
#43377=CARTESIAN_POINT('Ctrl Pts',(-3.65500246526749,1.,1.69737117722534));
#43378=CARTESIAN_POINT('Ctrl Pts',(-3.66030338774847,-1.,1.70289888566873));
#43379=CARTESIAN_POINT('Ctrl Pts',(-3.66030338774847,1.,1.70289888566873));
#43380=CARTESIAN_POINT('Ctrl Pts',(-3.66558043198876,-1.,1.70846001610956));
#43381=CARTESIAN_POINT('Ctrl Pts',(-3.66558043198876,1.,1.70846001610956));
#43382=CARTESIAN_POINT('Ctrl Pts',(-3.67083454901611,-1.,1.71405450210383));
#43383=CARTESIAN_POINT('Ctrl Pts',(-3.67083454901611,1.,1.71405450210383));
#43384=CARTESIAN_POINT('Ctrl Pts',(-3.67606660374709,-1.,1.71968225581808));
#43385=CARTESIAN_POINT('Ctrl Pts',(-3.67606660374709,1.,1.71968225581808));
#43386=CARTESIAN_POINT('Ctrl Pts',(-3.68127704936579,-1.,1.72534302437056));
#43387=CARTESIAN_POINT('Ctrl Pts',(-3.68127704936579,1.,1.72534302437056));
#43388=CARTESIAN_POINT('Ctrl Pts',(-3.68646597019332,-1.,1.73103640956717));
#43389=CARTESIAN_POINT('Ctrl Pts',(-3.68646597019332,1.,1.73103640956717));
#43390=CARTESIAN_POINT('Ctrl Pts',(-3.69163322648036,-1.,1.73676193254557));
#43391=CARTESIAN_POINT('Ctrl Pts',(-3.69163322648036,1.,1.73676193254557));
#43392=CARTESIAN_POINT('Ctrl Pts',(-3.69677856910517,-1.,1.74251908492617));
#43393=CARTESIAN_POINT('Ctrl Pts',(-3.69677856910517,1.,1.74251908492617));
#43394=CARTESIAN_POINT('Ctrl Pts',(-3.7019017567335,-1.,1.74830738046057));
#43395=CARTESIAN_POINT('Ctrl Pts',(-3.7019017567335,1.,1.74830738046057));
#43396=CARTESIAN_POINT('Ctrl Pts',(-3.70700269736659,-1.,1.75412641804042));
#43397=CARTESIAN_POINT('Ctrl Pts',(-3.70700269736659,1.,1.75412641804042));
#43398=CARTESIAN_POINT('Ctrl Pts',(-3.71208146346136,-1.,1.75997588498865));
#43399=CARTESIAN_POINT('Ctrl Pts',(-3.71208146346136,1.,1.75997588498865));
#43400=CARTESIAN_POINT('Ctrl Pts',(-3.71713822377359,-1.,1.76585552124394));
#43401=CARTESIAN_POINT('Ctrl Pts',(-3.71713822377359,1.,1.76585552124394));
#43402=CARTESIAN_POINT('Ctrl Pts',(-3.72217319911254,-1.,1.77176509401761));
#43403=CARTESIAN_POINT('Ctrl Pts',(-3.72217319911254,1.,1.77176509401761));
#43404=CARTESIAN_POINT('Ctrl Pts',(-3.72718661205609,-1.,1.77770437039658));
#43405=CARTESIAN_POINT('Ctrl Pts',(-3.72718661205609,1.,1.77770437039658));
#43406=CARTESIAN_POINT('Ctrl Pts',(-3.7321786309547,-1.,1.78367308442901));
#43407=CARTESIAN_POINT('Ctrl Pts',(-3.7321786309547,1.,1.78367308442901));
#43408=CARTESIAN_POINT('Ctrl Pts',(-3.73714934730681,-1.,1.78967092823491));
#43409=CARTESIAN_POINT('Ctrl Pts',(-3.73714934730681,1.,1.78967092823491));
#43410=CARTESIAN_POINT('Ctrl Pts',(-3.74209880352445,-1.,1.79569757859422));
#43411=CARTESIAN_POINT('Ctrl Pts',(-3.74209880352445,1.,1.79569757859422));
#43412=CARTESIAN_POINT('Ctrl Pts',(-3.74702700875467,-1.,1.8017527148577));
#43413=CARTESIAN_POINT('Ctrl Pts',(-3.74702700875467,1.,1.8017527148577));
#43414=CARTESIAN_POINT('Ctrl Pts',(-3.75193395887977,-1.,1.80783603939617));
#43415=CARTESIAN_POINT('Ctrl Pts',(-3.75193395887977,1.,1.80783603939617));
#43416=CARTESIAN_POINT('Ctrl Pts',(-3.75681965683071,-1.,1.8139472983358));
#43417=CARTESIAN_POINT('Ctrl Pts',(-3.75681965683071,1.,1.8139472983358));
#43418=CARTESIAN_POINT('Ctrl Pts',(-3.76168412707948,-1.,1.82008629694091));
#43419=CARTESIAN_POINT('Ctrl Pts',(-3.76168412707948,1.,1.82008629694091));
#43420=CARTESIAN_POINT('Ctrl Pts',(-3.76652740353775,-1.,1.82625289220915));
#43421=CARTESIAN_POINT('Ctrl Pts',(-3.76652740353775,1.,1.82625289220915));
#43422=CARTESIAN_POINT('Ctrl Pts',(-3.77038509817999,-1.,1.83120816955645));
#43423=CARTESIAN_POINT('Ctrl Pts',(-3.77038509817999,1.,1.83120816955645));
#43424=CARTESIAN_POINT('Ctrl Pts',(-3.77326886064398,-1.,1.83493697934534));
#43425=CARTESIAN_POINT('Ctrl Pts',(-3.77326886064398,1.,1.83493697934534));
#43426=CARTESIAN_POINT('Ctrl Pts',(-3.77518714457833,-1.,1.83742834010626));
#43427=CARTESIAN_POINT('Ctrl Pts',(-3.77518714457833,1.,1.83742834010626));
#43428=CARTESIAN_POINT('Ctrl Pts',(-3.77614523045147,-1.,1.8386753923786));
#43429=CARTESIAN_POINT('Ctrl Pts',(-3.77614523045147,1.,1.8386753923786));
#43430=CARTESIAN_POINT('',(-3.42859860294306,1.,1.5189508286633));
#43431=CARTESIAN_POINT('Ctrl Pts',(-3.42859860294306,-1.,1.5189508286633));
#43432=CARTESIAN_POINT('Ctrl Pts',(-3.42859860294306,-0.666666666666667,
1.5189508286633));
#43433=CARTESIAN_POINT('Ctrl Pts',(-3.42859860294306,-0.333333333333333,
1.5189508286633));
#43434=CARTESIAN_POINT('Ctrl Pts',(-3.42859860294306,0.333333333333333,
1.5189508286633));
#43435=CARTESIAN_POINT('Ctrl Pts',(-3.42859860294306,0.666666666666667,
1.5189508286633));
#43436=CARTESIAN_POINT('Ctrl Pts',(-3.42859860294306,1.,1.5189508286633));
#43437=CARTESIAN_POINT('',(-3.77614523045147,1.,1.8386753923786));
#43438=CARTESIAN_POINT('',(-3.77614523045147,0.,1.8386753923786));
#43439=CARTESIAN_POINT('Ctrl Pts',(-3.42859860294306,1.,1.5189508286633));
#43440=CARTESIAN_POINT('Ctrl Pts',(-3.42864616361875,1.,1.51893924967331));
#43441=CARTESIAN_POINT('Ctrl Pts',(-3.42884302333841,1.,1.5189513329503));
#43442=CARTESIAN_POINT('Ctrl Pts',(-3.42946838852587,1.,1.51914806898491));
#43443=CARTESIAN_POINT('Ctrl Pts',(-3.43101631893414,1.,1.5198144909338));
#43444=CARTESIAN_POINT('Ctrl Pts',(-3.43417156977893,1.,1.52134826724292));
#43445=CARTESIAN_POINT('Ctrl Pts',(-3.4388889597401,1.,1.5237734895035));
#43446=CARTESIAN_POINT('Ctrl Pts',(-3.44469547526647,1.,1.52686242875556));
#43447=CARTESIAN_POINT('Ctrl Pts',(-3.45127136828305,1.,1.53046244461635));
#43448=CARTESIAN_POINT('Ctrl Pts',(-3.45825932955032,1.,1.53440195378792));
#43449=CARTESIAN_POINT('Ctrl Pts',(-3.46531752207153,1.,1.53851507915502));
#43450=CARTESIAN_POINT('Ctrl Pts',(-3.47217189224653,1.,1.54266605398187));
#43451=CARTESIAN_POINT('Ctrl Pts',(-3.47868272898751,1.,1.54678009290276));
#43452=CARTESIAN_POINT('Ctrl Pts',(-3.48485155928567,1.,1.55084702970452));
#43453=CARTESIAN_POINT('Ctrl Pts',(-3.4907646087742,1.,1.55489595901116));
#43454=CARTESIAN_POINT('Ctrl Pts',(-3.49655185179655,1.,1.55897703097874));
#43455=CARTESIAN_POINT('Ctrl Pts',(-3.50234321621578,1.,1.56314187758675));
#43456=CARTESIAN_POINT('Ctrl Pts',(-3.50821771695363,1.,1.56742097575012));
#43457=CARTESIAN_POINT('Ctrl Pts',(-3.51418598431665,1.,1.57181569799743));
#43458=CARTESIAN_POINT('Ctrl Pts',(-3.52021847865912,1.,1.57631049988158));
#43459=CARTESIAN_POINT('Ctrl Pts',(-3.52626275334881,1.,1.58088027227848));
#43460=CARTESIAN_POINT('Ctrl Pts',(-3.5322637814708,1.,1.58549906268088));
#43461=CARTESIAN_POINT('Ctrl Pts',(-3.53818616861077,1.,1.59014958368739));
#43462=CARTESIAN_POINT('Ctrl Pts',(-3.54402458182337,1.,1.59482766949766));
#43463=CARTESIAN_POINT('Ctrl Pts',(-3.54979148634454,1.,1.59953698113457));
#43464=CARTESIAN_POINT('Ctrl Pts',(-3.55550985096129,1.,1.60428584699853));
#43465=CARTESIAN_POINT('Ctrl Pts',(-3.5612043248298,1.,1.60908344685457));
#43466=CARTESIAN_POINT('Ctrl Pts',(-3.56689200468387,1.,1.61393581747514));
#43467=CARTESIAN_POINT('Ctrl Pts',(-3.57257679609806,1.,1.61884340915404));
#43468=CARTESIAN_POINT('Ctrl Pts',(-3.5782545595439,1.,1.62380329464844));
#43469=CARTESIAN_POINT('Ctrl Pts',(-3.58391625774343,1.,1.62881051550745));
#43470=CARTESIAN_POINT('Ctrl Pts',(-3.58955176627879,1.,1.6338597145126));
#43471=CARTESIAN_POINT('Ctrl Pts',(-3.59515368334893,1.,1.63894676675352));
#43472=CARTESIAN_POINT('Ctrl Pts',(-3.60072028513845,1.,1.64407004385582));
#43473=CARTESIAN_POINT('Ctrl Pts',(-3.60625346556992,1.,1.64922952425832));
#43474=CARTESIAN_POINT('Ctrl Pts',(-3.61175734965127,1.,1.65442619244325));
#43475=CARTESIAN_POINT('Ctrl Pts',(-3.61723666482456,1.,1.65966133399186));
#43476=CARTESIAN_POINT('Ctrl Pts',(-3.62269517989109,1.,1.66493585923855));
#43477=CARTESIAN_POINT('Ctrl Pts',(-3.62813422105271,1.,1.67024966008045));
#43478=CARTESIAN_POINT('Ctrl Pts',(-3.63355343201232,1.,1.67560193613156));
#43479=CARTESIAN_POINT('Ctrl Pts',(-3.63895140887462,1.,1.68099146651586));
#43480=CARTESIAN_POINT('Ctrl Pts',(-3.64432638915203,1.,1.68641690471457));
#43481=CARTESIAN_POINT('Ctrl Pts',(-3.64967689827371,1.,1.69187705481689));
#43482=CARTESIAN_POINT('Ctrl Pts',(-3.65500246526749,1.,1.69737117722534));
#43483=CARTESIAN_POINT('Ctrl Pts',(-3.66030338774847,1.,1.70289888566873));
#43484=CARTESIAN_POINT('Ctrl Pts',(-3.66558043198876,1.,1.70846001610956));
#43485=CARTESIAN_POINT('Ctrl Pts',(-3.67083454901611,1.,1.71405450210383));
#43486=CARTESIAN_POINT('Ctrl Pts',(-3.67606660374709,1.,1.71968225581808));
#43487=CARTESIAN_POINT('Ctrl Pts',(-3.68127704936579,1.,1.72534302437056));
#43488=CARTESIAN_POINT('Ctrl Pts',(-3.68646597019332,1.,1.73103640956717));
#43489=CARTESIAN_POINT('Ctrl Pts',(-3.69163322648036,1.,1.73676193254557));
#43490=CARTESIAN_POINT('Ctrl Pts',(-3.69677856910517,1.,1.74251908492617));
#43491=CARTESIAN_POINT('Ctrl Pts',(-3.7019017567335,1.,1.74830738046057));
#43492=CARTESIAN_POINT('Ctrl Pts',(-3.70700269736659,1.,1.75412641804042));
#43493=CARTESIAN_POINT('Ctrl Pts',(-3.71208146346136,1.,1.75997588498865));
#43494=CARTESIAN_POINT('Ctrl Pts',(-3.71713822377359,1.,1.76585552124394));
#43495=CARTESIAN_POINT('Ctrl Pts',(-3.72217319911254,1.,1.77176509401761));
#43496=CARTESIAN_POINT('Ctrl Pts',(-3.72718661205609,1.,1.77770437039658));
#43497=CARTESIAN_POINT('Ctrl Pts',(-3.7321786309547,1.,1.78367308442901));
#43498=CARTESIAN_POINT('Ctrl Pts',(-3.73714934730681,1.,1.78967092823491));
#43499=CARTESIAN_POINT('Ctrl Pts',(-3.74209880352445,1.,1.79569757859422));
#43500=CARTESIAN_POINT('Ctrl Pts',(-3.74702700875467,1.,1.8017527148577));
#43501=CARTESIAN_POINT('Ctrl Pts',(-3.75193395887977,1.,1.80783603939617));
#43502=CARTESIAN_POINT('Ctrl Pts',(-3.75681965683071,1.,1.8139472983358));
#43503=CARTESIAN_POINT('Ctrl Pts',(-3.76168412707948,1.,1.82008629694091));
#43504=CARTESIAN_POINT('Ctrl Pts',(-3.76652740353775,1.,1.82625289220915));
#43505=CARTESIAN_POINT('Ctrl Pts',(-3.77038509817999,1.,1.83120816955645));
#43506=CARTESIAN_POINT('Ctrl Pts',(-3.77326886064398,1.,1.83493697934534));
#43507=CARTESIAN_POINT('Ctrl Pts',(-3.77518714457833,1.,1.83742834010626));
#43508=CARTESIAN_POINT('Ctrl Pts',(-3.77614523045147,1.,1.8386753923786));
#43509=CARTESIAN_POINT('Origin',(-3.77614523045147,0.,1.8386753923786));
#43510=CARTESIAN_POINT('',(-3.70708211654725,1.,1.97421938526992));
#43511=CARTESIAN_POINT('Origin',(0.,0.,0.));
#43512=CARTESIAN_POINT('',(-3.49844575334386,1.,1.35032489087269));
#43513=CARTESIAN_POINT('Origin',(0.,1.,0.));
#43514=CARTESIAN_POINT('Ctrl Pts',(-3.49844575334386,1.,1.35032489087269));
#43515=CARTESIAN_POINT('Ctrl Pts',(-3.49844575334386,0.666666666666667,
1.35032489087269));
#43516=CARTESIAN_POINT('Ctrl Pts',(-3.49844575334386,0.333333333333333,
1.35032489087269));
#43517=CARTESIAN_POINT('Ctrl Pts',(-3.49844575334386,-0.333333333333333,
1.35032489087269));
#43518=CARTESIAN_POINT('Ctrl Pts',(-3.49844575334386,-0.666666666666667,
1.35032489087269));
#43519=CARTESIAN_POINT('Ctrl Pts',(-3.49844575334386,-1.,1.35032489087269));
#43520=CARTESIAN_POINT('Ctrl Pts',(-3.97027773754922,-1.,1.36999806084572));
#43521=CARTESIAN_POINT('Ctrl Pts',(-3.97027773754922,1.,1.36999806084572));
#43522=CARTESIAN_POINT('Ctrl Pts',(-3.9687184694173,-1.,1.37020239094758));
#43523=CARTESIAN_POINT('Ctrl Pts',(-3.9687184694173,1.,1.37020239094758));
#43524=CARTESIAN_POINT('Ctrl Pts',(-3.96560037975788,-1.,1.37060761746027));
#43525=CARTESIAN_POINT('Ctrl Pts',(-3.96560037975788,1.,1.37060761746027));
#43526=CARTESIAN_POINT('Ctrl Pts',(-3.96092458508407,-1.,1.37120515615663));
#43527=CARTESIAN_POINT('Ctrl Pts',(-3.96092458508407,1.,1.37120515615663));
#43528=CARTESIAN_POINT('Ctrl Pts',(-3.95469287283105,-1.,1.37198126433139));
#43529=CARTESIAN_POINT('Ctrl Pts',(-3.95469287283105,1.,1.37198126433139));
#43530=CARTESIAN_POINT('Ctrl Pts',(-3.94690771786926,-1.,1.37291699203423));
#43531=CARTESIAN_POINT('Ctrl Pts',(-3.94690771786926,1.,1.37291699203423));
#43532=CARTESIAN_POINT('Ctrl Pts',(-3.93912709041791,-1.,1.37381821967499));
#43533=CARTESIAN_POINT('Ctrl Pts',(-3.93912709041791,1.,1.37381821967499));
#43534=CARTESIAN_POINT('Ctrl Pts',(-3.93135106761941,-1.,1.37468482215784));
#43535=CARTESIAN_POINT('Ctrl Pts',(-3.93135106761941,1.,1.37468482215784));
#43536=CARTESIAN_POINT('Ctrl Pts',(-3.92357976987132,-1.,1.37551664448057));
#43537=CARTESIAN_POINT('Ctrl Pts',(-3.92357976987132,1.,1.37551664448057));
#43538=CARTESIAN_POINT('Ctrl Pts',(-3.91581337461825,-1.,1.37631350505516));
#43539=CARTESIAN_POINT('Ctrl Pts',(-3.91581337461825,1.,1.37631350505516));
#43540=CARTESIAN_POINT('Ctrl Pts',(-3.90805209522729,-1.,1.3770751963376));
#43541=CARTESIAN_POINT('Ctrl Pts',(-3.90805209522729,1.,1.3770751963376));
#43542=CARTESIAN_POINT('Ctrl Pts',(-3.90029615196255,-1.,1.3778014851263));
#43543=CARTESIAN_POINT('Ctrl Pts',(-3.90029615196255,1.,1.3778014851263));
#43544=CARTESIAN_POINT('Ctrl Pts',(-3.89254574338385,-1.,1.37849211287981));
#43545=CARTESIAN_POINT('Ctrl Pts',(-3.89254574338385,1.,1.37849211287981));
#43546=CARTESIAN_POINT('Ctrl Pts',(-3.88480102249461,-1.,1.37914679719446));
#43547=CARTESIAN_POINT('Ctrl Pts',(-3.88480102249461,1.,1.37914679719446));
#43548=CARTESIAN_POINT('Ctrl Pts',(-3.87706205830865,-1.,1.37976523097187));
#43549=CARTESIAN_POINT('Ctrl Pts',(-3.87706205830865,1.,1.37976523097187));
#43550=CARTESIAN_POINT('Ctrl Pts',(-3.86932885813403,-1.,1.38034709213129));
#43551=CARTESIAN_POINT('Ctrl Pts',(-3.86932885813403,1.,1.38034709213129));
#43552=CARTESIAN_POINT('Ctrl Pts',(-3.86160143044187,-1.,1.38089205993067));
#43553=CARTESIAN_POINT('Ctrl Pts',(-3.86160143044187,1.,1.38089205993067));
#43554=CARTESIAN_POINT('Ctrl Pts',(-3.85387983979557,-1.,1.38139983115075));
#43555=CARTESIAN_POINT('Ctrl Pts',(-3.85387983979557,1.,1.38139983115075));
#43556=CARTESIAN_POINT('Ctrl Pts',(-3.84616425605705,-1.,1.38187013346089));
#43557=CARTESIAN_POINT('Ctrl Pts',(-3.84616425605705,1.,1.38187013346089));
#43558=CARTESIAN_POINT('Ctrl Pts',(-3.83845502790609,-1.,1.38230274828774));
#43559=CARTESIAN_POINT('Ctrl Pts',(-3.83845502790609,1.,1.38230274828774));
#43560=CARTESIAN_POINT('Ctrl Pts',(-3.83075266982138,-1.,1.38269750245086));
#43561=CARTESIAN_POINT('Ctrl Pts',(-3.83075266982138,1.,1.38269750245086));
#43562=CARTESIAN_POINT('Ctrl Pts',(-3.82305771743715,-1.,1.38305421262724));
#43563=CARTESIAN_POINT('Ctrl Pts',(-3.82305771743715,1.,1.38305421262724));
#43564=CARTESIAN_POINT('Ctrl Pts',(-3.81537060817765,-1.,1.38337263902766));
#43565=CARTESIAN_POINT('Ctrl Pts',(-3.81537060817765,1.,1.38337263902766));
#43566=CARTESIAN_POINT('Ctrl Pts',(-3.80769156398429,-1.,1.38365244046226));
#43567=CARTESIAN_POINT('Ctrl Pts',(-3.80769156398429,1.,1.38365244046226));
#43568=CARTESIAN_POINT('Ctrl Pts',(-3.80002044322169,-1.,1.38389311766701));
#43569=CARTESIAN_POINT('Ctrl Pts',(-3.80002044322169,1.,1.38389311766701));
#43570=CARTESIAN_POINT('Ctrl Pts',(-3.79235669640907,-1.,1.38409399694588));
#43571=CARTESIAN_POINT('Ctrl Pts',(-3.79235669640907,1.,1.38409399694588));
#43572=CARTESIAN_POINT('Ctrl Pts',(-3.78469969805134,-1.,1.38425435883773));
#43573=CARTESIAN_POINT('Ctrl Pts',(-3.78469969805134,1.,1.38425435883773));
#43574=CARTESIAN_POINT('Ctrl Pts',(-3.77704902230441,-1.,1.38437354551435));
#43575=CARTESIAN_POINT('Ctrl Pts',(-3.77704902230441,1.,1.38437354551435));
#43576=CARTESIAN_POINT('Ctrl Pts',(-3.76940473185775,-1.,1.38445107339517));
#43577=CARTESIAN_POINT('Ctrl Pts',(-3.76940473185775,1.,1.38445107339517));
#43578=CARTESIAN_POINT('Ctrl Pts',(-3.76176768271347,-1.,1.38448675253343));
#43579=CARTESIAN_POINT('Ctrl Pts',(-3.76176768271347,1.,1.38448675253343));
#43580=CARTESIAN_POINT('Ctrl Pts',(-3.75413976318727,-1.,1.38448077997155));
#43581=CARTESIAN_POINT('Ctrl Pts',(-3.75413976318727,1.,1.38448077997155));
#43582=CARTESIAN_POINT('Ctrl Pts',(-3.7465231716786,-1.,1.38443344984389));
#43583=CARTESIAN_POINT('Ctrl Pts',(-3.7465231716786,1.,1.38443344984389));
#43584=CARTESIAN_POINT('Ctrl Pts',(-3.73891976418099,-1.,1.38434489156456));
#43585=CARTESIAN_POINT('Ctrl Pts',(-3.73891976418099,1.,1.38434489156456));
#43586=CARTESIAN_POINT('Ctrl Pts',(-3.73133035859283,-1.,1.38421479111531));
#43587=CARTESIAN_POINT('Ctrl Pts',(-3.73133035859283,1.,1.38421479111531));
#43588=CARTESIAN_POINT('Ctrl Pts',(-3.72375409358805,-1.,1.3840421342895));
#43589=CARTESIAN_POINT('Ctrl Pts',(-3.72375409358805,1.,1.3840421342895));
#43590=CARTESIAN_POINT('Ctrl Pts',(-3.7161876605181,-1.,1.38382489984585));
#43591=CARTESIAN_POINT('Ctrl Pts',(-3.7161876605181,1.,1.38382489984585));
#43592=CARTESIAN_POINT('Ctrl Pts',(-3.70862680753343,-1.,1.38356065402122));
#43593=CARTESIAN_POINT('Ctrl Pts',(-3.70862680753343,1.,1.38356065402122));
#43594=CARTESIAN_POINT('Ctrl Pts',(-3.70106792167894,-1.,1.38324717612862));
#43595=CARTESIAN_POINT('Ctrl Pts',(-3.70106792167894,1.,1.38324717612862));
#43596=CARTESIAN_POINT('Ctrl Pts',(-3.69350967899523,-1.,1.38288311171649));
#43597=CARTESIAN_POINT('Ctrl Pts',(-3.69350967899523,1.,1.38288311171649));
#43598=CARTESIAN_POINT('Ctrl Pts',(-3.68595444983844,-1.,1.38246852827185));
#43599=CARTESIAN_POINT('Ctrl Pts',(-3.68595444983844,1.,1.38246852827185));
#43600=CARTESIAN_POINT('Ctrl Pts',(-3.6784103848243,-1.,1.38200574290626));
#43601=CARTESIAN_POINT('Ctrl Pts',(-3.6784103848243,1.,1.38200574290626));
#43602=CARTESIAN_POINT('Ctrl Pts',(-3.67088843112282,-1.,1.38149812653876));
#43603=CARTESIAN_POINT('Ctrl Pts',(-3.67088843112282,1.,1.38149812653876));
#43604=CARTESIAN_POINT('Ctrl Pts',(-3.66339848520874,-1.,1.38094856333558));
#43605=CARTESIAN_POINT('Ctrl Pts',(-3.66339848520874,1.,1.38094856333558));
#43606=CARTESIAN_POINT('Ctrl Pts',(-3.65594554404396,-1.,1.38035791051215));
#43607=CARTESIAN_POINT('Ctrl Pts',(-3.65594554404396,1.,1.38035791051215));
#43608=CARTESIAN_POINT('Ctrl Pts',(-3.64852652756444,-1.,1.37972372481598));
#43609=CARTESIAN_POINT('Ctrl Pts',(-3.64852652756444,1.,1.37972372481598));
#43610=CARTESIAN_POINT('Ctrl Pts',(-3.64112507791112,-1.,1.37903818567347));
#43611=CARTESIAN_POINT('Ctrl Pts',(-3.64112507791112,1.,1.37903818567347));
#43612=CARTESIAN_POINT('Ctrl Pts',(-3.63371727442448,-1.,1.37829035457324));
#43613=CARTESIAN_POINT('Ctrl Pts',(-3.63371727442448,1.,1.37829035457324));
#43614=CARTESIAN_POINT('Ctrl Pts',(-3.62628098665112,-1.,1.37746987919868));
#43615=CARTESIAN_POINT('Ctrl Pts',(-3.62628098665112,1.,1.37746987919868));
#43616=CARTESIAN_POINT('Ctrl Pts',(-3.61880481160408,-1.,1.37657053403102));
#43617=CARTESIAN_POINT('Ctrl Pts',(-3.61880481160408,1.,1.37657053403102));
#43618=CARTESIAN_POINT('Ctrl Pts',(-3.61129546591082,-1.,1.37559314436641));
#43619=CARTESIAN_POINT('Ctrl Pts',(-3.61129546591082,1.,1.37559314436641));
#43620=CARTESIAN_POINT('Ctrl Pts',(-3.60379020124038,-1.,1.37455051379642));
#43621=CARTESIAN_POINT('Ctrl Pts',(-3.60379020124038,1.,1.37455051379642));
#43622=CARTESIAN_POINT('Ctrl Pts',(-3.59634627869117,-1.,1.37346320103184));
#43623=CARTESIAN_POINT('Ctrl Pts',(-3.59634627869117,1.,1.37346320103184));
#43624=CARTESIAN_POINT('Ctrl Pts',(-3.5890185384643,-1.,1.37235053661));
#43625=CARTESIAN_POINT('Ctrl Pts',(-3.5890185384643,1.,1.37235053661));
#43626=CARTESIAN_POINT('Ctrl Pts',(-3.58183885982745,-1.,1.37122241663073));
#43627=CARTESIAN_POINT('Ctrl Pts',(-3.58183885982745,1.,1.37122241663073));
#43628=CARTESIAN_POINT('Ctrl Pts',(-3.57479875549453,-1.,1.37007229485646));
#43629=CARTESIAN_POINT('Ctrl Pts',(-3.57479875549453,1.,1.37007229485646));
#43630=CARTESIAN_POINT('Ctrl Pts',(-3.56782080304554,-1.,1.36886584973349));
#43631=CARTESIAN_POINT('Ctrl Pts',(-3.56782080304554,1.,1.36886584973349));
#43632=CARTESIAN_POINT('Ctrl Pts',(-3.56077662028492,-1.,1.36754771771174));
#43633=CARTESIAN_POINT('Ctrl Pts',(-3.56077662028492,1.,1.36754771771174));
#43634=CARTESIAN_POINT('Ctrl Pts',(-3.55353883995793,-1.,1.36606145456711));
#43635=CARTESIAN_POINT('Ctrl Pts',(-3.55353883995793,1.,1.36606145456711));
#43636=CARTESIAN_POINT('Ctrl Pts',(-3.54602591832893,-1.,1.36436666257567));
#43637=CARTESIAN_POINT('Ctrl Pts',(-3.54602591832893,1.,1.36436666257567));
#43638=CARTESIAN_POINT('Ctrl Pts',(-3.53824396425032,-1.,1.36245507339334));
#43639=CARTESIAN_POINT('Ctrl Pts',(-3.53824396425032,1.,1.36245507339334));
#43640=CARTESIAN_POINT('Ctrl Pts',(-3.53034464961849,-1.,1.36037259643827));
#43641=CARTESIAN_POINT('Ctrl Pts',(-3.53034464961849,1.,1.36037259643827));
#43642=CARTESIAN_POINT('Ctrl Pts',(-3.52261776117121,-1.,1.35821701528975));
#43643=CARTESIAN_POINT('Ctrl Pts',(-3.52261776117121,1.,1.35821701528975));
#43644=CARTESIAN_POINT('Ctrl Pts',(-3.51542230699919,-1.,1.35611275237288));
#43645=CARTESIAN_POINT('Ctrl Pts',(-3.51542230699919,1.,1.35611275237288));
#43646=CARTESIAN_POINT('Ctrl Pts',(-3.50913227060177,-1.,1.35419113576022));
#43647=CARTESIAN_POINT('Ctrl Pts',(-3.50913227060177,1.,1.35419113576022));
#43648=CARTESIAN_POINT('Ctrl Pts',(-3.50408168106113,-1.,1.3525703284343));
#43649=CARTESIAN_POINT('Ctrl Pts',(-3.50408168106113,1.,1.3525703284343));
#43650=CARTESIAN_POINT('Ctrl Pts',(-3.50049707063673,-1.,1.35133076331065));
#43651=CARTESIAN_POINT('Ctrl Pts',(-3.50049707063673,1.,1.35133076331065));
#43652=CARTESIAN_POINT('Ctrl Pts',(-3.49888720256612,-1.,1.35067437417289));
#43653=CARTESIAN_POINT('Ctrl Pts',(-3.49888720256612,1.,1.35067437417289));
#43654=CARTESIAN_POINT('Ctrl Pts',(-3.49840357193384,-1.,1.35037650302887));
#43655=CARTESIAN_POINT('Ctrl Pts',(-3.49840357193384,1.,1.35037650302887));
#43656=CARTESIAN_POINT('Ctrl Pts',(-3.49840260053616,-1.,1.35026426118351));
#43657=CARTESIAN_POINT('Ctrl Pts',(-3.49840260053616,1.,1.35026426118351));
#43658=CARTESIAN_POINT('Ctrl Pts',(-3.49848248301936,-1.,1.35022972712301));
#43659=CARTESIAN_POINT('Ctrl Pts',(-3.49848248301936,1.,1.35022972712301));
#43660=CARTESIAN_POINT('',(-3.97027773754922,1.,1.36999806084572));
#43661=CARTESIAN_POINT('Ctrl Pts',(-3.97027773754922,1.,1.36999806084572));
#43662=CARTESIAN_POINT('Ctrl Pts',(-3.9687184694173,1.,1.37020239094758));
#43663=CARTESIAN_POINT('Ctrl Pts',(-3.96560037975788,1.,1.37060761746027));
#43664=CARTESIAN_POINT('Ctrl Pts',(-3.96092458508407,1.,1.37120515615663));
#43665=CARTESIAN_POINT('Ctrl Pts',(-3.95469287283105,1.,1.37198126433139));
#43666=CARTESIAN_POINT('Ctrl Pts',(-3.94690771786926,1.,1.37291699203423));
#43667=CARTESIAN_POINT('Ctrl Pts',(-3.93912709041791,1.,1.37381821967499));
#43668=CARTESIAN_POINT('Ctrl Pts',(-3.93135106761941,1.,1.37468482215784));
#43669=CARTESIAN_POINT('Ctrl Pts',(-3.92357976987132,1.,1.37551664448057));
#43670=CARTESIAN_POINT('Ctrl Pts',(-3.91581337461825,1.,1.37631350505516));
#43671=CARTESIAN_POINT('Ctrl Pts',(-3.90805209522729,1.,1.3770751963376));
#43672=CARTESIAN_POINT('Ctrl Pts',(-3.90029615196255,1.,1.3778014851263));
#43673=CARTESIAN_POINT('Ctrl Pts',(-3.89254574338385,1.,1.37849211287981));
#43674=CARTESIAN_POINT('Ctrl Pts',(-3.88480102249461,1.,1.37914679719446));
#43675=CARTESIAN_POINT('Ctrl Pts',(-3.87706205830865,1.,1.37976523097187));
#43676=CARTESIAN_POINT('Ctrl Pts',(-3.86932885813403,1.,1.38034709213129));
#43677=CARTESIAN_POINT('Ctrl Pts',(-3.86160143044187,1.,1.38089205993067));
#43678=CARTESIAN_POINT('Ctrl Pts',(-3.85387983979557,1.,1.38139983115075));
#43679=CARTESIAN_POINT('Ctrl Pts',(-3.84616425605705,1.,1.38187013346089));
#43680=CARTESIAN_POINT('Ctrl Pts',(-3.83845502790609,1.,1.38230274828774));
#43681=CARTESIAN_POINT('Ctrl Pts',(-3.83075266982138,1.,1.38269750245086));
#43682=CARTESIAN_POINT('Ctrl Pts',(-3.82305771743715,1.,1.38305421262724));
#43683=CARTESIAN_POINT('Ctrl Pts',(-3.81537060817765,1.,1.38337263902766));
#43684=CARTESIAN_POINT('Ctrl Pts',(-3.80769156398429,1.,1.38365244046226));
#43685=CARTESIAN_POINT('Ctrl Pts',(-3.80002044322169,1.,1.38389311766701));
#43686=CARTESIAN_POINT('Ctrl Pts',(-3.79235669640907,1.,1.38409399694588));
#43687=CARTESIAN_POINT('Ctrl Pts',(-3.78469969805134,1.,1.38425435883773));
#43688=CARTESIAN_POINT('Ctrl Pts',(-3.77704902230441,1.,1.38437354551435));
#43689=CARTESIAN_POINT('Ctrl Pts',(-3.76940473185775,1.,1.38445107339517));
#43690=CARTESIAN_POINT('Ctrl Pts',(-3.76176768271347,1.,1.38448675253343));
#43691=CARTESIAN_POINT('Ctrl Pts',(-3.75413976318727,1.,1.38448077997155));
#43692=CARTESIAN_POINT('Ctrl Pts',(-3.7465231716786,1.,1.38443344984389));
#43693=CARTESIAN_POINT('Ctrl Pts',(-3.73891976418099,1.,1.38434489156456));
#43694=CARTESIAN_POINT('Ctrl Pts',(-3.73133035859283,1.,1.38421479111531));
#43695=CARTESIAN_POINT('Ctrl Pts',(-3.72375409358805,1.,1.3840421342895));
#43696=CARTESIAN_POINT('Ctrl Pts',(-3.7161876605181,1.,1.38382489984585));
#43697=CARTESIAN_POINT('Ctrl Pts',(-3.70862680753343,1.,1.38356065402122));
#43698=CARTESIAN_POINT('Ctrl Pts',(-3.70106792167894,1.,1.38324717612862));
#43699=CARTESIAN_POINT('Ctrl Pts',(-3.69350967899523,1.,1.38288311171649));
#43700=CARTESIAN_POINT('Ctrl Pts',(-3.68595444983844,1.,1.38246852827185));
#43701=CARTESIAN_POINT('Ctrl Pts',(-3.6784103848243,1.,1.38200574290626));
#43702=CARTESIAN_POINT('Ctrl Pts',(-3.67088843112282,1.,1.38149812653876));
#43703=CARTESIAN_POINT('Ctrl Pts',(-3.66339848520874,1.,1.38094856333558));
#43704=CARTESIAN_POINT('Ctrl Pts',(-3.65594554404396,1.,1.38035791051215));
#43705=CARTESIAN_POINT('Ctrl Pts',(-3.64852652756444,1.,1.37972372481598));
#43706=CARTESIAN_POINT('Ctrl Pts',(-3.64112507791112,1.,1.37903818567347));
#43707=CARTESIAN_POINT('Ctrl Pts',(-3.63371727442448,1.,1.37829035457324));
#43708=CARTESIAN_POINT('Ctrl Pts',(-3.62628098665112,1.,1.37746987919868));
#43709=CARTESIAN_POINT('Ctrl Pts',(-3.61880481160408,1.,1.37657053403102));
#43710=CARTESIAN_POINT('Ctrl Pts',(-3.61129546591082,1.,1.37559314436641));
#43711=CARTESIAN_POINT('Ctrl Pts',(-3.60379020124038,1.,1.37455051379642));
#43712=CARTESIAN_POINT('Ctrl Pts',(-3.59634627869117,1.,1.37346320103184));
#43713=CARTESIAN_POINT('Ctrl Pts',(-3.5890185384643,1.,1.37235053661));
#43714=CARTESIAN_POINT('Ctrl Pts',(-3.58183885982745,1.,1.37122241663073));
#43715=CARTESIAN_POINT('Ctrl Pts',(-3.57479875549453,1.,1.37007229485646));
#43716=CARTESIAN_POINT('Ctrl Pts',(-3.56782080304554,1.,1.36886584973349));
#43717=CARTESIAN_POINT('Ctrl Pts',(-3.56077662028492,1.,1.36754771771174));
#43718=CARTESIAN_POINT('Ctrl Pts',(-3.55353883995793,1.,1.36606145456711));
#43719=CARTESIAN_POINT('Ctrl Pts',(-3.54602591832893,1.,1.36436666257567));
#43720=CARTESIAN_POINT('Ctrl Pts',(-3.53824396425032,1.,1.36245507339334));
#43721=CARTESIAN_POINT('Ctrl Pts',(-3.53034464961849,1.,1.36037259643827));
#43722=CARTESIAN_POINT('Ctrl Pts',(-3.52261776117121,1.,1.35821701528975));
#43723=CARTESIAN_POINT('Ctrl Pts',(-3.51542230699919,1.,1.35611275237288));
#43724=CARTESIAN_POINT('Ctrl Pts',(-3.50913227060177,1.,1.35419113576022));
#43725=CARTESIAN_POINT('Ctrl Pts',(-3.50408168106113,1.,1.3525703284343));
#43726=CARTESIAN_POINT('Ctrl Pts',(-3.5007660381658,1.,1.35142377279535));
#43727=CARTESIAN_POINT('Ctrl Pts',(-3.49920025459856,1.,1.35080045218652));
#43728=CARTESIAN_POINT('Ctrl Pts',(-3.49861894124915,1.,1.35049736560633));
#43729=CARTESIAN_POINT('Ctrl Pts',(-3.49847119623841,1.,1.35036670893102));
#43730=CARTESIAN_POINT('Ctrl Pts',(-3.49844575334386,1.,1.35032489087269));
#43731=CARTESIAN_POINT('',(-3.97027773754922,0.,1.36999806084572));
#43732=CARTESIAN_POINT('Ctrl Pts',(-3.62397690409552,-1.,0.96399761336957));
#43733=CARTESIAN_POINT('Ctrl Pts',(-3.62397690409552,1.,0.96399761336957));
#43734=CARTESIAN_POINT('Ctrl Pts',(-3.62393257642191,-1.,0.963922720982576));
#43735=CARTESIAN_POINT('Ctrl Pts',(-3.62393257642191,1.,0.963922720982576));
#43736=CARTESIAN_POINT('Ctrl Pts',(-3.62399933640277,-1.,0.963832486396055));
#43737=CARTESIAN_POINT('Ctrl Pts',(-3.62399933640277,1.,0.963832486396055));
#43738=CARTESIAN_POINT('Ctrl Pts',(-3.62456568607055,-1.,0.963875774532102));
#43739=CARTESIAN_POINT('Ctrl Pts',(-3.62456568607055,1.,0.963875774532102));
#43740=CARTESIAN_POINT('Ctrl Pts',(-3.62625391255277,-1.,0.964291001274618));
#43741=CARTESIAN_POINT('Ctrl Pts',(-3.62625391255277,1.,0.964291001274618));
#43742=CARTESIAN_POINT('Ctrl Pts',(-3.62988252139998,-1.,0.965395153165716));
#43743=CARTESIAN_POINT('Ctrl Pts',(-3.62988252139998,1.,0.965395153165716));
#43744=CARTESIAN_POINT('Ctrl Pts',(-3.6349212208096,-1.,0.967052554540877));
#43745=CARTESIAN_POINT('Ctrl Pts',(-3.6349212208096,1.,0.967052554540877));
#43746=CARTESIAN_POINT('Ctrl Pts',(-3.64113946505393,-1.,0.969195124674829));
#43747=CARTESIAN_POINT('Ctrl Pts',(-3.64113946505393,1.,0.969195124674829));
#43748=CARTESIAN_POINT('Ctrl Pts',(-3.64819756447072,-1.,0.971722122060277));
#43749=CARTESIAN_POINT('Ctrl Pts',(-3.64819756447072,1.,0.971722122060277));
#43750=CARTESIAN_POINT('Ctrl Pts',(-3.6557157673487,-1.,0.974519971354138));
#43751=CARTESIAN_POINT('Ctrl Pts',(-3.6557157673487,1.,0.974519971354138));
#43752=CARTESIAN_POINT('Ctrl Pts',(-3.66333049637403,-1.,0.977478312751416));
#43753=CARTESIAN_POINT('Ctrl Pts',(-3.66333049637403,1.,0.977478312751416));
#43754=CARTESIAN_POINT('Ctrl Pts',(-3.67074983340444,-1.,0.980505922458494));
#43755=CARTESIAN_POINT('Ctrl Pts',(-3.67074983340444,1.,0.980505922458494));
#43756=CARTESIAN_POINT('Ctrl Pts',(-3.67782408841876,-1.,0.983550791470864));
#43757=CARTESIAN_POINT('Ctrl Pts',(-3.67782408841876,1.,0.983550791470864));
#43758=CARTESIAN_POINT('Ctrl Pts',(-3.6845531792623,-1.,0.986602639864285));
#43759=CARTESIAN_POINT('Ctrl Pts',(-3.6845531792623,1.,0.986602639864285));
#43760=CARTESIAN_POINT('Ctrl Pts',(-3.69102682138955,-1.,0.989676715398858));
#43761=CARTESIAN_POINT('Ctrl Pts',(-3.69102682138955,1.,0.989676715398858));
#43762=CARTESIAN_POINT('Ctrl Pts',(-3.69738123415696,-1.,0.992802218332103));
#43763=CARTESIAN_POINT('Ctrl Pts',(-3.69738123415696,1.,0.992802218332103));
#43764=CARTESIAN_POINT('Ctrl Pts',(-3.70375282282107,-1.,0.996009819772431));
#43765=CARTESIAN_POINT('Ctrl Pts',(-3.70375282282107,1.,0.996009819772431));
#43766=CARTESIAN_POINT('Ctrl Pts',(-3.7102243971387,-1.,0.999317260756344));
#43767=CARTESIAN_POINT('Ctrl Pts',(-3.7102243971387,1.,0.999317260756344));
#43768=CARTESIAN_POINT('Ctrl Pts',(-3.71680667125047,-1.,1.00272423396802));
#43769=CARTESIAN_POINT('Ctrl Pts',(-3.71680667125047,1.,1.00272423396802));
#43770=CARTESIAN_POINT('Ctrl Pts',(-3.72346803750544,-1.,1.00622000735696));
#43771=CARTESIAN_POINT('Ctrl Pts',(-3.72346803750544,1.,1.00622000735696));
#43772=CARTESIAN_POINT('Ctrl Pts',(-3.73015276704407,-1.,1.00978798539491));
#43773=CARTESIAN_POINT('Ctrl Pts',(-3.73015276704407,1.,1.00978798539491));
#43774=CARTESIAN_POINT('Ctrl Pts',(-3.73680245055747,-1.,1.01341114319906));
#43775=CARTESIAN_POINT('Ctrl Pts',(-3.73680245055747,1.,1.01341114319906));
#43776=CARTESIAN_POINT('Ctrl Pts',(-3.74337942504993,-1.,1.01707794311088));
#43777=CARTESIAN_POINT('Ctrl Pts',(-3.74337942504993,1.,1.01707794311088));
#43778=CARTESIAN_POINT('Ctrl Pts',(-3.74987777155873,-1.,1.02078510487439));
#43779=CARTESIAN_POINT('Ctrl Pts',(-3.74987777155873,1.,1.02078510487439));
#43780=CARTESIAN_POINT('Ctrl Pts',(-3.75631037456224,-1.,1.02453429444668));
#43781=CARTESIAN_POINT('Ctrl Pts',(-3.75631037456224,1.,1.02453429444668));
#43782=CARTESIAN_POINT('Ctrl Pts',(-3.76270122291245,-1.,1.02833014458184));
#43783=CARTESIAN_POINT('Ctrl Pts',(-3.76270122291245,1.,1.02833014458184));
#43784=CARTESIAN_POINT('Ctrl Pts',(-3.76907609832516,-1.,1.03217786604919));
#43785=CARTESIAN_POINT('Ctrl Pts',(-3.76907609832516,1.,1.03217786604919));
#43786=CARTESIAN_POINT('Ctrl Pts',(-3.77545283140427,-1.,1.03608074678008));
#43787=CARTESIAN_POINT('Ctrl Pts',(-3.77545283140427,1.,1.03608074678008));
#43788=CARTESIAN_POINT('Ctrl Pts',(-3.7818353500817,-1.,1.04003862055798));
#43789=CARTESIAN_POINT('Ctrl Pts',(-3.7818353500817,1.,1.04003862055798));
#43790=CARTESIAN_POINT('Ctrl Pts',(-3.78821910787179,-1.,1.04404924374422));
#43791=CARTESIAN_POINT('Ctrl Pts',(-3.78821910787179,1.,1.04404924374422));
#43792=CARTESIAN_POINT('Ctrl Pts',(-3.79459440308786,-1.,1.04810913267639));
#43793=CARTESIAN_POINT('Ctrl Pts',(-3.79459440308786,1.,1.04810913267639));
#43794=CARTESIAN_POINT('Ctrl Pts',(-3.80095039790681,-1.,1.05221457990016));
#43795=CARTESIAN_POINT('Ctrl Pts',(-3.80095039790681,1.,1.05221457990016));
#43796=CARTESIAN_POINT('Ctrl Pts',(-3.80727913637791,-1.,1.05636266918644));
#43797=CARTESIAN_POINT('Ctrl Pts',(-3.80727913637791,1.,1.05636266918644));
#43798=CARTESIAN_POINT('Ctrl Pts',(-3.8135786611749,-1.,1.06055206187299));
#43799=CARTESIAN_POINT('Ctrl Pts',(-3.8135786611749,1.,1.06055206187299));
#43800=CARTESIAN_POINT('Ctrl Pts',(-3.81985083953012,-1.,1.0647824403893));
#43801=CARTESIAN_POINT('Ctrl Pts',(-3.81985083953012,1.,1.0647824403893));
#43802=CARTESIAN_POINT('Ctrl Pts',(-3.82609989967276,-1.,1.06905413180359));
#43803=CARTESIAN_POINT('Ctrl Pts',(-3.82609989967276,1.,1.06905413180359));
#43804=CARTESIAN_POINT('Ctrl Pts',(-3.83233071195144,-1.,1.07336766633459));
#43805=CARTESIAN_POINT('Ctrl Pts',(-3.83233071195144,1.,1.07336766633459));
#43806=CARTESIAN_POINT('Ctrl Pts',(-3.83854714117491,-1.,1.07772335353858));
#43807=CARTESIAN_POINT('Ctrl Pts',(-3.83854714117491,1.,1.07772335353858));
#43808=CARTESIAN_POINT('Ctrl Pts',(-3.8447504803063,-1.,1.08212087917991));
#43809=CARTESIAN_POINT('Ctrl Pts',(-3.8447504803063,1.,1.08212087917991));
#43810=CARTESIAN_POINT('Ctrl Pts',(-3.85094025222713,-1.,1.08655950846384));
#43811=CARTESIAN_POINT('Ctrl Pts',(-3.85094025222713,1.,1.08655950846384));
#43812=CARTESIAN_POINT('Ctrl Pts',(-3.85711487933931,-1.,1.09103825516294));
#43813=CARTESIAN_POINT('Ctrl Pts',(-3.85711487933931,1.,1.09103825516294));
#43814=CARTESIAN_POINT('Ctrl Pts',(-3.86327241021247,-1.,1.09555606505013));
#43815=CARTESIAN_POINT('Ctrl Pts',(-3.86327241021247,1.,1.09555606505013));
#43816=CARTESIAN_POINT('Ctrl Pts',(-3.86941120134849,-1.,1.10011198761195));
#43817=CARTESIAN_POINT('Ctrl Pts',(-3.86941120134849,1.,1.10011198761195));
#43818=CARTESIAN_POINT('Ctrl Pts',(-3.87553067187514,-1.,1.10470536603287));
#43819=CARTESIAN_POINT('Ctrl Pts',(-3.87553067187514,1.,1.10470536603287));
#43820=CARTESIAN_POINT('Ctrl Pts',(-3.88163105531724,-1.,1.10933577224008));
#43821=CARTESIAN_POINT('Ctrl Pts',(-3.88163105531724,1.,1.10933577224008));
#43822=CARTESIAN_POINT('Ctrl Pts',(-3.88771308285171,-1.,1.11400292434429));
#43823=CARTESIAN_POINT('Ctrl Pts',(-3.88771308285171,1.,1.11400292434429));
#43824=CARTESIAN_POINT('Ctrl Pts',(-3.89377768340344,-1.,1.11870660794603));
#43825=CARTESIAN_POINT('Ctrl Pts',(-3.89377768340344,1.,1.11870660794603));
#43826=CARTESIAN_POINT('Ctrl Pts',(-3.89982569750025,-1.,1.12344660099043));
#43827=CARTESIAN_POINT('Ctrl Pts',(-3.89982569750025,1.,1.12344660099043));
#43828=CARTESIAN_POINT('Ctrl Pts',(-3.90585753318737,-1.,1.12822258281553));
#43829=CARTESIAN_POINT('Ctrl Pts',(-3.90585753318737,1.,1.12822258281553));
#43830=CARTESIAN_POINT('Ctrl Pts',(-3.91187321145649,-1.,1.13303414693896));
#43831=CARTESIAN_POINT('Ctrl Pts',(-3.91187321145649,1.,1.13303414693896));
#43832=CARTESIAN_POINT('Ctrl Pts',(-3.91787251936827,-1.,1.13788084225554));
#43833=CARTESIAN_POINT('Ctrl Pts',(-3.91787251936827,1.,1.13788084225554));
#43834=CARTESIAN_POINT('Ctrl Pts',(-3.92385513133997,-1.,1.14276220561593));
#43835=CARTESIAN_POINT('Ctrl Pts',(-3.92385513133997,1.,1.14276220561593));
#43836=CARTESIAN_POINT('Ctrl Pts',(-3.92982073294257,-1.,1.14767779451123));
#43837=CARTESIAN_POINT('Ctrl Pts',(-3.92982073294257,1.,1.14767779451123));
#43838=CARTESIAN_POINT('Ctrl Pts',(-3.9357691705628,-1.,1.1526272271632));
#43839=CARTESIAN_POINT('Ctrl Pts',(-3.9357691705628,1.,1.1526272271632));
#43840=CARTESIAN_POINT('Ctrl Pts',(-3.94170046685203,-1.,1.15761018340956));
#43841=CARTESIAN_POINT('Ctrl Pts',(-3.94170046685203,1.,1.15761018340956));
#43842=CARTESIAN_POINT('Ctrl Pts',(-3.94761474780583,-1.,1.16262637999157));
#43843=CARTESIAN_POINT('Ctrl Pts',(-3.94761474780583,1.,1.16262637999157));
#43844=CARTESIAN_POINT('Ctrl Pts',(-3.95351219509876,-1.,1.16767555244438));
#43845=CARTESIAN_POINT('Ctrl Pts',(-3.95351219509876,1.,1.16767555244438));
#43846=CARTESIAN_POINT('Ctrl Pts',(-3.95939299213276,-1.,1.17275743590361));
#43847=CARTESIAN_POINT('Ctrl Pts',(-3.95939299213276,1.,1.17275743590361));
#43848=CARTESIAN_POINT('Ctrl Pts',(-3.96525726358159,-1.,1.17787174135592));
#43849=CARTESIAN_POINT('Ctrl Pts',(-3.96525726358159,1.,1.17787174135592));
#43850=CARTESIAN_POINT('Ctrl Pts',(-3.97110505165415,-1.,1.18301815039831));
#43851=CARTESIAN_POINT('Ctrl Pts',(-3.97110505165415,1.,1.18301815039831));
#43852=CARTESIAN_POINT('Ctrl Pts',(-3.97693634767754,-1.,1.18819633715539));
#43853=CARTESIAN_POINT('Ctrl Pts',(-3.97693634767754,1.,1.18819633715539));
#43854=CARTESIAN_POINT('Ctrl Pts',(-3.98275111052561,-1.,1.19340598349475));
#43855=CARTESIAN_POINT('Ctrl Pts',(-3.98275111052561,1.,1.19340598349475));
#43856=CARTESIAN_POINT('Ctrl Pts',(-3.98854928957189,-1.,1.19864679609566));
#43857=CARTESIAN_POINT('Ctrl Pts',(-3.98854928957189,1.,1.19864679609566));
#43858=CARTESIAN_POINT('Ctrl Pts',(-3.99433084799666,-1.,1.20391852375139));
#43859=CARTESIAN_POINT('Ctrl Pts',(-3.99433084799666,1.,1.20391852375139));
#43860=CARTESIAN_POINT('Ctrl Pts',(-4.00009577950721,-1.,1.20922097029551));
#43861=CARTESIAN_POINT('Ctrl Pts',(-4.00009577950721,1.,1.20922097029551));
#43862=CARTESIAN_POINT('Ctrl Pts',(-4.00584409522722,-1.,1.21455398918133));
#43863=CARTESIAN_POINT('Ctrl Pts',(-4.00584409522722,1.,1.21455398918133));
#43864=CARTESIAN_POINT('Ctrl Pts',(-4.01042947140789,-1.,1.21884478244403));
#43865=CARTESIAN_POINT('Ctrl Pts',(-4.01042947140789,1.,1.21884478244403));
#43866=CARTESIAN_POINT('Ctrl Pts',(-4.01386104433519,-1.,1.22207656455845));
#43867=CARTESIAN_POINT('Ctrl Pts',(-4.01386104433519,1.,1.22207656455845));
#43868=CARTESIAN_POINT('Ctrl Pts',(-4.01614544569895,-1.,1.22423716681317));
#43869=CARTESIAN_POINT('Ctrl Pts',(-4.01614544569895,1.,1.22423716681317));
#43870=CARTESIAN_POINT('Ctrl Pts',(-4.01728681790024,-1.,1.22531898815164));
#43871=CARTESIAN_POINT('Ctrl Pts',(-4.01728681790024,1.,1.22531898815164));
#43872=CARTESIAN_POINT('',(-3.62400312501199,1.,0.963899035118986));
#43873=CARTESIAN_POINT('Ctrl Pts',(-3.62400312501199,-1.,0.963899035118986));
#43874=CARTESIAN_POINT('Ctrl Pts',(-3.62400312501199,-0.666666666666667,
0.963899035118986));
#43875=CARTESIAN_POINT('Ctrl Pts',(-3.62400312501199,-0.333333333333333,
0.963899035118986));
#43876=CARTESIAN_POINT('Ctrl Pts',(-3.62400312501199,0.333333333333333,
0.963899035118986));
#43877=CARTESIAN_POINT('Ctrl Pts',(-3.62400312501199,0.666666666666667,
0.963899035118985));
#43878=CARTESIAN_POINT('Ctrl Pts',(-3.62400312501199,1.,0.963899035118985));
#43879=CARTESIAN_POINT('',(-4.01728681790024,1.,1.22531898815164));
#43880=CARTESIAN_POINT('',(-4.01728681790024,0.,1.22531898815164));
#43881=CARTESIAN_POINT('Ctrl Pts',(-3.62400312501199,1.,0.963899035118985));
#43882=CARTESIAN_POINT('Ctrl Pts',(-3.62404828878374,1.,0.963880158556713));
#43883=CARTESIAN_POINT('Ctrl Pts',(-3.62424461507455,1.,0.963861297423579));
#43884=CARTESIAN_POINT('Ctrl Pts',(-3.62489305727516,1.,0.963957782642589));
#43885=CARTESIAN_POINT('Ctrl Pts',(-3.62652618145252,1.,0.964373850166081));
#43886=CARTESIAN_POINT('Ctrl Pts',(-3.62988252139998,1.,0.965395153165716));
#43887=CARTESIAN_POINT('Ctrl Pts',(-3.6349212208096,1.,0.967052554540877));
#43888=CARTESIAN_POINT('Ctrl Pts',(-3.64113946505393,1.,0.969195124674829));
#43889=CARTESIAN_POINT('Ctrl Pts',(-3.64819756447072,1.,0.971722122060277));
#43890=CARTESIAN_POINT('Ctrl Pts',(-3.6557157673487,1.,0.974519971354138));
#43891=CARTESIAN_POINT('Ctrl Pts',(-3.66333049637403,1.,0.977478312751416));
#43892=CARTESIAN_POINT('Ctrl Pts',(-3.67074983340444,1.,0.980505922458494));
#43893=CARTESIAN_POINT('Ctrl Pts',(-3.67782408841876,1.,0.983550791470864));
#43894=CARTESIAN_POINT('Ctrl Pts',(-3.6845531792623,1.,0.986602639864285));
#43895=CARTESIAN_POINT('Ctrl Pts',(-3.69102682138955,1.,0.989676715398858));
#43896=CARTESIAN_POINT('Ctrl Pts',(-3.69738123415696,1.,0.992802218332103));
#43897=CARTESIAN_POINT('Ctrl Pts',(-3.70375282282107,1.,0.996009819772431));
#43898=CARTESIAN_POINT('Ctrl Pts',(-3.7102243971387,1.,0.999317260756344));
#43899=CARTESIAN_POINT('Ctrl Pts',(-3.71680667125047,1.,1.00272423396802));
#43900=CARTESIAN_POINT('Ctrl Pts',(-3.72346803750544,1.,1.00622000735696));
#43901=CARTESIAN_POINT('Ctrl Pts',(-3.73015276704407,1.,1.00978798539491));
#43902=CARTESIAN_POINT('Ctrl Pts',(-3.73680245055747,1.,1.01341114319906));
#43903=CARTESIAN_POINT('Ctrl Pts',(-3.74337942504993,1.,1.01707794311088));
#43904=CARTESIAN_POINT('Ctrl Pts',(-3.74987777155873,1.,1.02078510487439));
#43905=CARTESIAN_POINT('Ctrl Pts',(-3.75631037456224,1.,1.02453429444668));
#43906=CARTESIAN_POINT('Ctrl Pts',(-3.76270122291245,1.,1.02833014458184));
#43907=CARTESIAN_POINT('Ctrl Pts',(-3.76907609832516,1.,1.03217786604919));
#43908=CARTESIAN_POINT('Ctrl Pts',(-3.77545283140427,1.,1.03608074678008));
#43909=CARTESIAN_POINT('Ctrl Pts',(-3.7818353500817,1.,1.04003862055798));
#43910=CARTESIAN_POINT('Ctrl Pts',(-3.78821910787179,1.,1.04404924374422));
#43911=CARTESIAN_POINT('Ctrl Pts',(-3.79459440308786,1.,1.04810913267639));
#43912=CARTESIAN_POINT('Ctrl Pts',(-3.80095039790681,1.,1.05221457990016));
#43913=CARTESIAN_POINT('Ctrl Pts',(-3.80727913637791,1.,1.05636266918644));
#43914=CARTESIAN_POINT('Ctrl Pts',(-3.8135786611749,1.,1.06055206187299));
#43915=CARTESIAN_POINT('Ctrl Pts',(-3.81985083953012,1.,1.0647824403893));
#43916=CARTESIAN_POINT('Ctrl Pts',(-3.82609989967276,1.,1.06905413180359));
#43917=CARTESIAN_POINT('Ctrl Pts',(-3.83233071195144,1.,1.07336766633459));
#43918=CARTESIAN_POINT('Ctrl Pts',(-3.83854714117491,1.,1.07772335353858));
#43919=CARTESIAN_POINT('Ctrl Pts',(-3.8447504803063,1.,1.08212087917991));
#43920=CARTESIAN_POINT('Ctrl Pts',(-3.85094025222713,1.,1.08655950846384));
#43921=CARTESIAN_POINT('Ctrl Pts',(-3.85711487933931,1.,1.09103825516294));
#43922=CARTESIAN_POINT('Ctrl Pts',(-3.86327241021247,1.,1.09555606505013));
#43923=CARTESIAN_POINT('Ctrl Pts',(-3.86941120134849,1.,1.10011198761195));
#43924=CARTESIAN_POINT('Ctrl Pts',(-3.87553067187514,1.,1.10470536603287));
#43925=CARTESIAN_POINT('Ctrl Pts',(-3.88163105531724,1.,1.10933577224008));
#43926=CARTESIAN_POINT('Ctrl Pts',(-3.88771308285171,1.,1.11400292434429));
#43927=CARTESIAN_POINT('Ctrl Pts',(-3.89377768340344,1.,1.11870660794603));
#43928=CARTESIAN_POINT('Ctrl Pts',(-3.89982569750025,1.,1.12344660099043));
#43929=CARTESIAN_POINT('Ctrl Pts',(-3.90585753318737,1.,1.12822258281553));
#43930=CARTESIAN_POINT('Ctrl Pts',(-3.91187321145649,1.,1.13303414693896));
#43931=CARTESIAN_POINT('Ctrl Pts',(-3.91787251936827,1.,1.13788084225554));
#43932=CARTESIAN_POINT('Ctrl Pts',(-3.92385513133997,1.,1.14276220561593));
#43933=CARTESIAN_POINT('Ctrl Pts',(-3.92982073294257,1.,1.14767779451123));
#43934=CARTESIAN_POINT('Ctrl Pts',(-3.9357691705628,1.,1.1526272271632));
#43935=CARTESIAN_POINT('Ctrl Pts',(-3.94170046685203,1.,1.15761018340956));
#43936=CARTESIAN_POINT('Ctrl Pts',(-3.94761474780583,1.,1.16262637999157));
#43937=CARTESIAN_POINT('Ctrl Pts',(-3.95351219509876,1.,1.16767555244438));
#43938=CARTESIAN_POINT('Ctrl Pts',(-3.95939299213276,1.,1.17275743590361));
#43939=CARTESIAN_POINT('Ctrl Pts',(-3.96525726358159,1.,1.17787174135592));
#43940=CARTESIAN_POINT('Ctrl Pts',(-3.97110505165415,1.,1.18301815039831));
#43941=CARTESIAN_POINT('Ctrl Pts',(-3.97693634767754,1.,1.18819633715539));
#43942=CARTESIAN_POINT('Ctrl Pts',(-3.98275111052561,1.,1.19340598349475));
#43943=CARTESIAN_POINT('Ctrl Pts',(-3.98854928957189,1.,1.19864679609566));
#43944=CARTESIAN_POINT('Ctrl Pts',(-3.99433084799666,1.,1.20391852375139));
#43945=CARTESIAN_POINT('Ctrl Pts',(-4.00009577950721,1.,1.20922097029551));
#43946=CARTESIAN_POINT('Ctrl Pts',(-4.00584409522722,1.,1.21455398918133));
#43947=CARTESIAN_POINT('Ctrl Pts',(-4.01042947140789,1.,1.21884478244403));
#43948=CARTESIAN_POINT('Ctrl Pts',(-4.01386104433519,1.,1.22207656455845));
#43949=CARTESIAN_POINT('Ctrl Pts',(-4.01614544569895,1.,1.22423716681317));
#43950=CARTESIAN_POINT('Ctrl Pts',(-4.01728681790024,1.,1.22531898815164));
#43951=CARTESIAN_POINT('Origin',(-4.01728681790024,0.,1.22531898815164));
#43952=CARTESIAN_POINT('',(-3.97027773754922,1.,1.36999806084572));
#43953=CARTESIAN_POINT('Origin',(0.,0.,0.));
#43954=CARTESIAN_POINT('',(-3.66661143271648,1.,0.786422660833743));
#43955=CARTESIAN_POINT('Origin',(0.,1.,0.));
#43956=CARTESIAN_POINT('Ctrl Pts',(-3.66661143271648,1.,0.786422660833743));
#43957=CARTESIAN_POINT('Ctrl Pts',(-3.66661143271648,0.666666666666667,
0.786422660833743));
#43958=CARTESIAN_POINT('Ctrl Pts',(-3.66661143271648,0.333333333333333,
0.786422660833743));
#43959=CARTESIAN_POINT('Ctrl Pts',(-3.66661143271648,-0.333333333333333,
0.786422660833743));
#43960=CARTESIAN_POINT('Ctrl Pts',(-3.66661143271648,-0.666666666666667,
0.786422660833743));
#43961=CARTESIAN_POINT('Ctrl Pts',(-3.66661143271648,-1.,0.786422660833743));
#43962=CARTESIAN_POINT('Ctrl Pts',(-4.13571194405636,-1.,0.732042837400619));
#43963=CARTESIAN_POINT('Ctrl Pts',(-4.13571194405636,1.,0.732042837400619));
#43964=CARTESIAN_POINT('Ctrl Pts',(-4.13420383737278,-1.,0.732488575135926));
#43965=CARTESIAN_POINT('Ctrl Pts',(-4.13420383737278,1.,0.732488575135926));
#43966=CARTESIAN_POINT('Ctrl Pts',(-4.13118752796397,-1.,0.733376589325634));
#43967=CARTESIAN_POINT('Ctrl Pts',(-4.13118752796397,1.,0.733376589325634));
#43968=CARTESIAN_POINT('Ctrl Pts',(-4.12666277572794,-1.,0.734698226767512));
#43969=CARTESIAN_POINT('Ctrl Pts',(-4.12666277572794,1.,0.734698226767512));
#43970=CARTESIAN_POINT('Ctrl Pts',(-4.12062919626082,-1.,0.736439634335347));
#43971=CARTESIAN_POINT('Ctrl Pts',(-4.12062919626082,1.,0.736439634335347));
#43972=CARTESIAN_POINT('Ctrl Pts',(-4.11308626953795,-1.,0.738581708229118));
#43973=CARTESIAN_POINT('Ctrl Pts',(-4.11308626953795,1.,0.738581708229118));
#43974=CARTESIAN_POINT('Ctrl Pts',(-4.1055424175856,-1.,0.740688998555151));
#43975=CARTESIAN_POINT('Ctrl Pts',(-4.1055424175856,1.,0.740688998555151));
#43976=CARTESIAN_POINT('Ctrl Pts',(-4.09799769702712,-1.,0.742761369690017));
#43977=CARTESIAN_POINT('Ctrl Pts',(-4.09799769702712,1.,0.742761369690017));
#43978=CARTESIAN_POINT('Ctrl Pts',(-4.09045220253011,-1.,0.744798649705514));
#43979=CARTESIAN_POINT('Ctrl Pts',(-4.09045220253011,1.,0.744798649705514));
#43980=CARTESIAN_POINT('Ctrl Pts',(-4.08290608094789,-1.,0.746800631490821));
#43981=CARTESIAN_POINT('Ctrl Pts',(-4.08290608094789,1.,0.746800631490821));
#43982=CARTESIAN_POINT('Ctrl Pts',(-4.07535951055363,-1.,0.748767076679177));
#43983=CARTESIAN_POINT('Ctrl Pts',(-4.07535951055363,1.,0.748767076679177));
#43984=CARTESIAN_POINT('Ctrl Pts',(-4.06781267241886,-1.,0.750697720483175));
#43985=CARTESIAN_POINT('Ctrl Pts',(-4.06781267241886,1.,0.750697720483175));
#43986=CARTESIAN_POINT('Ctrl Pts',(-4.06026572221399,-1.,0.752592276482869));
#43987=CARTESIAN_POINT('Ctrl Pts',(-4.06026572221399,1.,0.752592276482869));
#43988=CARTESIAN_POINT('Ctrl Pts',(-4.05271876688106,-1.,0.754450441816411));
#43989=CARTESIAN_POINT('Ctrl Pts',(-4.05271876688106,1.,0.754450441816411));
#43990=CARTESIAN_POINT('Ctrl Pts',(-4.04517182654344,-1.,0.756271902370186));
#43991=CARTESIAN_POINT('Ctrl Pts',(-4.04517182654344,1.,0.756271902370186));
#43992=CARTESIAN_POINT('Ctrl Pts',(-4.03762485803468,-1.,0.758056338885553));
#43993=CARTESIAN_POINT('Ctrl Pts',(-4.03762485803468,1.,0.758056338885553));
#43994=CARTESIAN_POINT('Ctrl Pts',(-4.0300778195465,-1.,0.759803433244166));
#43995=CARTESIAN_POINT('Ctrl Pts',(-4.0300778195465,1.,0.759803433244166));
#43996=CARTESIAN_POINT('Ctrl Pts',(-4.02253072741347,-1.,0.761512875859941));
#43997=CARTESIAN_POINT('Ctrl Pts',(-4.02253072741347,1.,0.761512875859941));
#43998=CARTESIAN_POINT('Ctrl Pts',(-4.01498370680434,-1.,0.763184371182826));
#43999=CARTESIAN_POINT('Ctrl Pts',(-4.01498370680434,1.,0.763184371182826));
#44000=CARTESIAN_POINT('Ctrl Pts',(-4.00743706791366,-1.,0.764817648784946));
#44001=CARTESIAN_POINT('Ctrl Pts',(-4.00743706791366,1.,0.764817648784946));
#44002=CARTESIAN_POINT('Ctrl Pts',(-3.99989129179464,-1.,0.766412457135785));
#44003=CARTESIAN_POINT('Ctrl Pts',(-3.99989129179464,1.,0.766412457135785));
#44004=CARTESIAN_POINT('Ctrl Pts',(-3.99234687880892,-1.,0.767968531377708));
#44005=CARTESIAN_POINT('Ctrl Pts',(-3.99234687880892,1.,0.767968531377708));
#44006=CARTESIAN_POINT('Ctrl Pts',(-3.98480422348403,-1.,0.769485566245459));
#44007=CARTESIAN_POINT('Ctrl Pts',(-3.98480422348403,1.,0.769485566245459));
#44008=CARTESIAN_POINT('Ctrl Pts',(-3.97726349165507,-1.,0.770963190030503));
#44009=CARTESIAN_POINT('Ctrl Pts',(-3.97726349165507,1.,0.770963190030503));
#44010=CARTESIAN_POINT('Ctrl Pts',(-3.96972446532832,-1.,0.772400931772238));
#44011=CARTESIAN_POINT('Ctrl Pts',(-3.96972446532832,1.,0.772400931772238));
#44012=CARTESIAN_POINT('Ctrl Pts',(-3.96218649639876,-1.,0.773798212026682));
#44013=CARTESIAN_POINT('Ctrl Pts',(-3.96218649639876,1.,0.773798212026682));
#44014=CARTESIAN_POINT('Ctrl Pts',(-3.95464885452364,-1.,0.775154418039441));
#44015=CARTESIAN_POINT('Ctrl Pts',(-3.95464885452364,1.,0.775154418039441));
#44016=CARTESIAN_POINT('Ctrl Pts',(-3.94711101619471,-1.,0.77646896669796));
#44017=CARTESIAN_POINT('Ctrl Pts',(-3.94711101619471,1.,0.77646896669796));
#44018=CARTESIAN_POINT('Ctrl Pts',(-3.93957296768098,-1.,0.777741370568549));
#44019=CARTESIAN_POINT('Ctrl Pts',(-3.93957296768098,1.,0.777741370568549));
#44020=CARTESIAN_POINT('Ctrl Pts',(-3.93203552473153,-1.,0.778971308134786));
#44021=CARTESIAN_POINT('Ctrl Pts',(-3.93203552473153,1.,0.778971308134786));
#44022=CARTESIAN_POINT('Ctrl Pts',(-3.92450058323799,-1.,0.780158678615506));
#44023=CARTESIAN_POINT('Ctrl Pts',(-3.92450058323799,1.,0.780158678615506));
#44024=CARTESIAN_POINT('Ctrl Pts',(-3.9169703605466,-1.,0.781303428618343));
#44025=CARTESIAN_POINT('Ctrl Pts',(-3.9169703605466,1.,0.781303428618343));
#44026=CARTESIAN_POINT('Ctrl Pts',(-3.90944671004536,-1.,0.782405395622758));
#44027=CARTESIAN_POINT('Ctrl Pts',(-3.90944671004536,1.,0.782405395622758));
#44028=CARTESIAN_POINT('Ctrl Pts',(-3.90193039043971,-1.,0.783464141529082));
#44029=CARTESIAN_POINT('Ctrl Pts',(-3.90193039043971,1.,0.783464141529082));
#44030=CARTESIAN_POINT('Ctrl Pts',(-3.89442039235105,-1.,0.784478799358335));
#44031=CARTESIAN_POINT('Ctrl Pts',(-3.89442039235105,1.,0.784478799358335));
#44032=CARTESIAN_POINT('Ctrl Pts',(-3.88691313167399,-1.,0.785447890340723));
#44033=CARTESIAN_POINT('Ctrl Pts',(-3.88691313167399,1.,0.785447890340723));
#44034=CARTESIAN_POINT('Ctrl Pts',(-3.87940402818186,-1.,0.786369675812592));
#44035=CARTESIAN_POINT('Ctrl Pts',(-3.87940402818186,1.,0.786369675812592));
#44036=CARTESIAN_POINT('Ctrl Pts',(-3.87188916600905,-1.,0.78724252761798));
#44037=CARTESIAN_POINT('Ctrl Pts',(-3.87188916600905,1.,0.78724252761798));
#44038=CARTESIAN_POINT('Ctrl Pts',(-3.86436702561342,-1.,0.788065315093771));
#44039=CARTESIAN_POINT('Ctrl Pts',(-3.86436702561342,1.,0.788065315093771));
#44040=CARTESIAN_POINT('Ctrl Pts',(-3.85683995872536,-1.,0.788837734090688));
#44041=CARTESIAN_POINT('Ctrl Pts',(-3.85683995872536,1.,0.788837734090688));
#44042=CARTESIAN_POINT('Ctrl Pts',(-3.8493163780891,-1.,0.789560798155618));
#44043=CARTESIAN_POINT('Ctrl Pts',(-3.8493163780891,1.,0.789560798155618));
#44044=CARTESIAN_POINT('Ctrl Pts',(-3.84180762342476,-1.,0.790236124191289));
#44045=CARTESIAN_POINT('Ctrl Pts',(-3.84180762342476,1.,0.790236124191289));
#44046=CARTESIAN_POINT('Ctrl Pts',(-3.83432392054804,-1.,0.79086501270534));
#44047=CARTESIAN_POINT('Ctrl Pts',(-3.83432392054804,1.,0.79086501270534));
#44048=CARTESIAN_POINT('Ctrl Pts',(-3.82687033899799,-1.,0.791447528662381));
#44049=CARTESIAN_POINT('Ctrl Pts',(-3.82687033899799,1.,0.791447528662381));
#44050=CARTESIAN_POINT('Ctrl Pts',(-3.81944345442237,-1.,0.791981740718606));
#44051=CARTESIAN_POINT('Ctrl Pts',(-3.81944345442237,1.,0.791981740718606));
#44052=CARTESIAN_POINT('Ctrl Pts',(-3.81202588694726,-1.,0.792462483517568));
#44053=CARTESIAN_POINT('Ctrl Pts',(-3.81202588694726,1.,0.792462483517568));
#44054=CARTESIAN_POINT('Ctrl Pts',(-3.80459229925598,-1.,0.792882695234693));
#44055=CARTESIAN_POINT('Ctrl Pts',(-3.80459229925598,1.,0.792882695234693));
#44056=CARTESIAN_POINT('Ctrl Pts',(-3.79711921389862,-1.,0.7932356129732));
#44057=CARTESIAN_POINT('Ctrl Pts',(-3.79711921389862,1.,0.7932356129732));
#44058=CARTESIAN_POINT('Ctrl Pts',(-3.78959439439222,-1.,0.793516871680966));
#44059=CARTESIAN_POINT('Ctrl Pts',(-3.78959439439222,1.,0.793516871680966));
#44060=CARTESIAN_POINT('Ctrl Pts',(-3.78202460377617,-1.,0.793726235781339));
#44061=CARTESIAN_POINT('Ctrl Pts',(-3.78202460377617,1.,0.793726235781339));
#44062=CARTESIAN_POINT('Ctrl Pts',(-3.77444863801264,-1.,0.793870523787515));
#44063=CARTESIAN_POINT('Ctrl Pts',(-3.77444863801264,1.,0.793870523787515));
#44064=CARTESIAN_POINT('Ctrl Pts',(-3.76692626931184,-1.,0.793961083689141));
#44065=CARTESIAN_POINT('Ctrl Pts',(-3.76692626931184,1.,0.793961083689141));
#44066=CARTESIAN_POINT('Ctrl Pts',(-3.75951468666325,-1.,0.794008429135047));
#44067=CARTESIAN_POINT('Ctrl Pts',(-3.75951468666325,1.,0.794008429135047));
#44068=CARTESIAN_POINT('Ctrl Pts',(-3.75224692493895,-1.,0.79401734737144));
#44069=CARTESIAN_POINT('Ctrl Pts',(-3.75224692493895,1.,0.79401734737144));
#44070=CARTESIAN_POINT('Ctrl Pts',(-3.74511357728827,-1.,0.79398270045988));
#44071=CARTESIAN_POINT('Ctrl Pts',(-3.74511357728827,1.,0.79398270045988));
#44072=CARTESIAN_POINT('Ctrl Pts',(-3.73803280541576,-1.,0.79388270093679));
#44073=CARTESIAN_POINT('Ctrl Pts',(-3.73803280541576,1.,0.79388270093679));
#44074=CARTESIAN_POINT('Ctrl Pts',(-3.7308691469564,-1.,0.793682750269347));
#44075=CARTESIAN_POINT('Ctrl Pts',(-3.7308691469564,1.,0.793682750269347));
#44076=CARTESIAN_POINT('Ctrl Pts',(-3.7234879729357,-1.,0.79334702378387));
#44077=CARTESIAN_POINT('Ctrl Pts',(-3.7234879729357,1.,0.79334702378387));
#44078=CARTESIAN_POINT('Ctrl Pts',(-3.7158024239604,-1.,0.792848377370115));
#44079=CARTESIAN_POINT('Ctrl Pts',(-3.7158024239604,1.,0.792848377370115));
#44080=CARTESIAN_POINT('Ctrl Pts',(-3.70781724021879,-1.,0.792177688845967));
#44081=CARTESIAN_POINT('Ctrl Pts',(-3.70781724021879,1.,0.792177688845967));
#44082=CARTESIAN_POINT('Ctrl Pts',(-3.69968940808982,-1.,0.791356575696509));
#44083=CARTESIAN_POINT('Ctrl Pts',(-3.69968940808982,1.,0.791356575696509));
#44084=CARTESIAN_POINT('Ctrl Pts',(-3.69172044327754,-1.,0.79043628498958));
#44085=CARTESIAN_POINT('Ctrl Pts',(-3.69172044327754,1.,0.79043628498958));
#44086=CARTESIAN_POINT('Ctrl Pts',(-3.68428439784285,-1.,0.789483546065158));
#44087=CARTESIAN_POINT('Ctrl Pts',(-3.68428439784285,1.,0.789483546065158));
#44088=CARTESIAN_POINT('Ctrl Pts',(-3.67777119516438,-1.,0.788569566220662));
#44089=CARTESIAN_POINT('Ctrl Pts',(-3.67777119516438,1.,0.788569566220662));
#44090=CARTESIAN_POINT('Ctrl Pts',(-3.672529236635,-1.,0.787758799995426));
#44091=CARTESIAN_POINT('Ctrl Pts',(-3.672529236635,1.,0.787758799995426));
#44092=CARTESIAN_POINT('Ctrl Pts',(-3.66879484800625,-1.,0.787095252589507));
#44093=CARTESIAN_POINT('Ctrl Pts',(-3.66879484800625,1.,0.787095252589507));
#44094=CARTESIAN_POINT('Ctrl Pts',(-3.66710211819938,-1.,0.786698783541657));
#44095=CARTESIAN_POINT('Ctrl Pts',(-3.66710211819938,1.,0.786698783541657));
#44096=CARTESIAN_POINT('Ctrl Pts',(-3.66657784454965,-1.,0.786480236184947));
#44097=CARTESIAN_POINT('Ctrl Pts',(-3.66657784454965,1.,0.786480236184947));
#44098=CARTESIAN_POINT('Ctrl Pts',(-3.66655932661846,-1.,0.786369528183039));
#44099=CARTESIAN_POINT('Ctrl Pts',(-3.66655932661846,1.,0.786369528183039));
#44100=CARTESIAN_POINT('Ctrl Pts',(-3.66663282329846,-1.,0.786322922920599));
#44101=CARTESIAN_POINT('Ctrl Pts',(-3.66663282329846,1.,0.786322922920599));
#44102=CARTESIAN_POINT('',(-4.13571194405636,1.,0.732042837400619));
#44103=CARTESIAN_POINT('Ctrl Pts',(-4.13571194405636,1.,0.732042837400619));
#44104=CARTESIAN_POINT('Ctrl Pts',(-4.13420383737278,1.,0.732488575135926));
#44105=CARTESIAN_POINT('Ctrl Pts',(-4.13118752796397,1.,0.733376589325634));
#44106=CARTESIAN_POINT('Ctrl Pts',(-4.12666277572794,1.,0.734698226767512));
#44107=CARTESIAN_POINT('Ctrl Pts',(-4.12062919626082,1.,0.736439634335347));
#44108=CARTESIAN_POINT('Ctrl Pts',(-4.11308626953795,1.,0.738581708229118));
#44109=CARTESIAN_POINT('Ctrl Pts',(-4.1055424175856,1.,0.740688998555151));
#44110=CARTESIAN_POINT('Ctrl Pts',(-4.09799769702712,1.,0.742761369690017));
#44111=CARTESIAN_POINT('Ctrl Pts',(-4.09045220253011,1.,0.744798649705514));
#44112=CARTESIAN_POINT('Ctrl Pts',(-4.08290608094789,1.,0.746800631490821));
#44113=CARTESIAN_POINT('Ctrl Pts',(-4.07535951055363,1.,0.748767076679177));
#44114=CARTESIAN_POINT('Ctrl Pts',(-4.06781267241886,1.,0.750697720483175));
#44115=CARTESIAN_POINT('Ctrl Pts',(-4.06026572221399,1.,0.752592276482869));
#44116=CARTESIAN_POINT('Ctrl Pts',(-4.05271876688106,1.,0.754450441816411));
#44117=CARTESIAN_POINT('Ctrl Pts',(-4.04517182654344,1.,0.756271902370186));
#44118=CARTESIAN_POINT('Ctrl Pts',(-4.03762485803468,1.,0.758056338885553));
#44119=CARTESIAN_POINT('Ctrl Pts',(-4.0300778195465,1.,0.759803433244166));
#44120=CARTESIAN_POINT('Ctrl Pts',(-4.02253072741347,1.,0.761512875859941));
#44121=CARTESIAN_POINT('Ctrl Pts',(-4.01498370680434,1.,0.763184371182826));
#44122=CARTESIAN_POINT('Ctrl Pts',(-4.00743706791366,1.,0.764817648784946));
#44123=CARTESIAN_POINT('Ctrl Pts',(-3.99989129179464,1.,0.766412457135785));
#44124=CARTESIAN_POINT('Ctrl Pts',(-3.99234687880892,1.,0.767968531377708));
#44125=CARTESIAN_POINT('Ctrl Pts',(-3.98480422348403,1.,0.769485566245459));
#44126=CARTESIAN_POINT('Ctrl Pts',(-3.97726349165507,1.,0.770963190030503));
#44127=CARTESIAN_POINT('Ctrl Pts',(-3.96972446532832,1.,0.772400931772238));
#44128=CARTESIAN_POINT('Ctrl Pts',(-3.96218649639876,1.,0.773798212026682));
#44129=CARTESIAN_POINT('Ctrl Pts',(-3.95464885452364,1.,0.775154418039441));
#44130=CARTESIAN_POINT('Ctrl Pts',(-3.94711101619471,1.,0.77646896669796));
#44131=CARTESIAN_POINT('Ctrl Pts',(-3.93957296768098,1.,0.777741370568549));
#44132=CARTESIAN_POINT('Ctrl Pts',(-3.93203552473153,1.,0.778971308134786));
#44133=CARTESIAN_POINT('Ctrl Pts',(-3.92450058323799,1.,0.780158678615506));
#44134=CARTESIAN_POINT('Ctrl Pts',(-3.9169703605466,1.,0.781303428618343));
#44135=CARTESIAN_POINT('Ctrl Pts',(-3.90944671004536,1.,0.782405395622758));
#44136=CARTESIAN_POINT('Ctrl Pts',(-3.90193039043971,1.,0.783464141529082));
#44137=CARTESIAN_POINT('Ctrl Pts',(-3.89442039235105,1.,0.784478799358335));
#44138=CARTESIAN_POINT('Ctrl Pts',(-3.88691313167399,1.,0.785447890340723));
#44139=CARTESIAN_POINT('Ctrl Pts',(-3.87940402818186,1.,0.786369675812592));
#44140=CARTESIAN_POINT('Ctrl Pts',(-3.87188916600905,1.,0.78724252761798));
#44141=CARTESIAN_POINT('Ctrl Pts',(-3.86436702561342,1.,0.788065315093771));
#44142=CARTESIAN_POINT('Ctrl Pts',(-3.85683995872536,1.,0.788837734090688));
#44143=CARTESIAN_POINT('Ctrl Pts',(-3.8493163780891,1.,0.789560798155618));
#44144=CARTESIAN_POINT('Ctrl Pts',(-3.84180762342476,1.,0.790236124191289));
#44145=CARTESIAN_POINT('Ctrl Pts',(-3.83432392054804,1.,0.79086501270534));
#44146=CARTESIAN_POINT('Ctrl Pts',(-3.82687033899799,1.,0.791447528662381));
#44147=CARTESIAN_POINT('Ctrl Pts',(-3.81944345442237,1.,0.791981740718606));
#44148=CARTESIAN_POINT('Ctrl Pts',(-3.81202588694726,1.,0.792462483517568));
#44149=CARTESIAN_POINT('Ctrl Pts',(-3.80459229925598,1.,0.792882695234693));
#44150=CARTESIAN_POINT('Ctrl Pts',(-3.79711921389862,1.,0.7932356129732));
#44151=CARTESIAN_POINT('Ctrl Pts',(-3.78959439439222,1.,0.793516871680966));
#44152=CARTESIAN_POINT('Ctrl Pts',(-3.78202460377617,1.,0.793726235781339));
#44153=CARTESIAN_POINT('Ctrl Pts',(-3.77444863801264,1.,0.793870523787515));
#44154=CARTESIAN_POINT('Ctrl Pts',(-3.76692626931184,1.,0.793961083689141));
#44155=CARTESIAN_POINT('Ctrl Pts',(-3.75951468666325,1.,0.794008429135047));
#44156=CARTESIAN_POINT('Ctrl Pts',(-3.75224692493895,1.,0.79401734737144));
#44157=CARTESIAN_POINT('Ctrl Pts',(-3.74511357728827,1.,0.79398270045988));
#44158=CARTESIAN_POINT('Ctrl Pts',(-3.73803280541576,1.,0.79388270093679));
#44159=CARTESIAN_POINT('Ctrl Pts',(-3.7308691469564,1.,0.793682750269347));
#44160=CARTESIAN_POINT('Ctrl Pts',(-3.7234879729357,1.,0.79334702378387));
#44161=CARTESIAN_POINT('Ctrl Pts',(-3.7158024239604,1.,0.792848377370115));
#44162=CARTESIAN_POINT('Ctrl Pts',(-3.70781724021879,1.,0.792177688845967));
#44163=CARTESIAN_POINT('Ctrl Pts',(-3.69968940808982,1.,0.791356575696509));
#44164=CARTESIAN_POINT('Ctrl Pts',(-3.69172044327754,1.,0.79043628498958));
#44165=CARTESIAN_POINT('Ctrl Pts',(-3.68428439784285,1.,0.789483546065158));
#44166=CARTESIAN_POINT('Ctrl Pts',(-3.67777119516438,1.,0.788569566220662));
#44167=CARTESIAN_POINT('Ctrl Pts',(-3.672529236635,1.,0.787758799995426));
#44168=CARTESIAN_POINT('Ctrl Pts',(-3.66907505398769,1.,0.787145041181588));
#44169=CARTESIAN_POINT('Ctrl Pts',(-3.66743103898844,1.,0.786774337198499));
#44170=CARTESIAN_POINT('Ctrl Pts',(-3.66680946938396,1.,0.786565919559889));
#44171=CARTESIAN_POINT('Ctrl Pts',(-3.66664310415236,1.,0.786459983896781));
#44172=CARTESIAN_POINT('Ctrl Pts',(-3.66661143271648,1.,0.786422660833743));
#44173=CARTESIAN_POINT('',(-4.13571194405636,0.,0.732042837400619));
#44174=CARTESIAN_POINT('Ctrl Pts',(-3.73016218570874,-1.,0.385214314776329));
#44175=CARTESIAN_POINT('Ctrl Pts',(-3.73016218570874,1.,0.385214314776329));
#44176=CARTESIAN_POINT('Ctrl Pts',(-3.73010668803185,-1.,0.385147278814804));
#44177=CARTESIAN_POINT('Ctrl Pts',(-3.73010668803185,1.,0.385147278814804));
#44178=CARTESIAN_POINT('Ctrl Pts',(-3.73015851028729,-1.,0.385047711603887));
#44179=CARTESIAN_POINT('Ctrl Pts',(-3.73015851028729,1.,0.385047711603887));
#44180=CARTESIAN_POINT('Ctrl Pts',(-3.73072465900727,-1.,0.385001870183841));
#44181=CARTESIAN_POINT('Ctrl Pts',(-3.73072465900727,1.,0.385001870183841));
#44182=CARTESIAN_POINT('Ctrl Pts',(-3.73245705639337,-1.,0.385147887989514));
#44183=CARTESIAN_POINT('Ctrl Pts',(-3.73245705639337,1.,0.385147887989514));
#44184=CARTESIAN_POINT('Ctrl Pts',(-3.73621371845475,-1.,0.385670806454744));
#44185=CARTESIAN_POINT('Ctrl Pts',(-3.73621371845475,1.,0.385670806454744));
#44186=CARTESIAN_POINT('Ctrl Pts',(-3.74144965781088,-1.,0.386519576222035));
#44187=CARTESIAN_POINT('Ctrl Pts',(-3.74144965781088,1.,0.386519576222035));
#44188=CARTESIAN_POINT('Ctrl Pts',(-3.74792651696269,-1.,0.387663020050396));
#44189=CARTESIAN_POINT('Ctrl Pts',(-3.74792651696269,1.,0.387663020050396));
#44190=CARTESIAN_POINT('Ctrl Pts',(-3.75529302894757,-1.,0.389054775898251));
#44191=CARTESIAN_POINT('Ctrl Pts',(-3.75529302894757,1.,0.389054775898251));
#44192=CARTESIAN_POINT('Ctrl Pts',(-3.76315635032993,-1.,0.390642072979259));
#44193=CARTESIAN_POINT('Ctrl Pts',(-3.76315635032993,1.,0.390642072979259));
#44194=CARTESIAN_POINT('Ctrl Pts',(-3.77114011595892,-1.,0.392372786223346));
#44195=CARTESIAN_POINT('Ctrl Pts',(-3.77114011595892,1.,0.392372786223346));
#44196=CARTESIAN_POINT('Ctrl Pts',(-3.77894173114368,-1.,0.394202481011595));
#44197=CARTESIAN_POINT('Ctrl Pts',(-3.77894173114368,1.,0.394202481011595));
#44198=CARTESIAN_POINT('Ctrl Pts',(-3.78640521279479,-1.,0.396103205335028));
#44199=CARTESIAN_POINT('Ctrl Pts',(-3.78640521279479,1.,0.396103205335028));
#44200=CARTESIAN_POINT('Ctrl Pts',(-3.79352887163457,-1.,0.398064818684158));
#44201=CARTESIAN_POINT('Ctrl Pts',(-3.79352887163457,1.,0.398064818684158));
#44202=CARTESIAN_POINT('Ctrl Pts',(-3.80040370384659,-1.,0.400088346504726));
#44203=CARTESIAN_POINT('Ctrl Pts',(-3.80040370384659,1.,0.400088346504726));
#44204=CARTESIAN_POINT('Ctrl Pts',(-3.80716881962763,-1.,0.402181320148474));
#44205=CARTESIAN_POINT('Ctrl Pts',(-3.80716881962763,1.,0.402181320148474));
#44206=CARTESIAN_POINT('Ctrl Pts',(-3.81396374287762,-1.,0.404352694628236));
#44207=CARTESIAN_POINT('Ctrl Pts',(-3.81396374287762,1.,0.404352694628236));
#44208=CARTESIAN_POINT('Ctrl Pts',(-3.82087303913741,-1.,0.406607038258906));
#44209=CARTESIAN_POINT('Ctrl Pts',(-3.82087303913741,1.,0.406607038258906));
#44210=CARTESIAN_POINT('Ctrl Pts',(-3.82790724256397,-1.,0.408942371447377));
#44211=CARTESIAN_POINT('Ctrl Pts',(-3.82790724256397,1.,0.408942371447377));
#44212=CARTESIAN_POINT('Ctrl Pts',(-3.83503345578645,-1.,0.411353038798459));
#44213=CARTESIAN_POINT('Ctrl Pts',(-3.83503345578645,1.,0.411353038798459));
#44214=CARTESIAN_POINT('Ctrl Pts',(-3.84219403994742,-1.,0.413831367016726));
#44215=CARTESIAN_POINT('Ctrl Pts',(-3.84219403994742,1.,0.413831367016726));
#44216=CARTESIAN_POINT('Ctrl Pts',(-3.8493286415751,-1.,0.41636967805292));
#44217=CARTESIAN_POINT('Ctrl Pts',(-3.8493286415751,1.,0.41636967805292));
#44218=CARTESIAN_POINT('Ctrl Pts',(-3.85639825648031,-1.,0.418962468086809));
#44219=CARTESIAN_POINT('Ctrl Pts',(-3.85639825648031,1.,0.418962468086809));
#44220=CARTESIAN_POINT('Ctrl Pts',(-3.86339652542749,-1.,0.421607423177575));
#44221=CARTESIAN_POINT('Ctrl Pts',(-3.86339652542749,1.,0.421607423177575));
#44222=CARTESIAN_POINT('Ctrl Pts',(-3.87033643487882,-1.,0.424304173195142));
#44223=CARTESIAN_POINT('Ctrl Pts',(-3.87033643487882,1.,0.424304173195142));
#44224=CARTESIAN_POINT('Ctrl Pts',(-3.87724240306609,-1.,0.427053541173469));
#44225=CARTESIAN_POINT('Ctrl Pts',(-3.87724240306609,1.,0.427053541173469));
#44226=CARTESIAN_POINT('Ctrl Pts',(-3.88414070943334,-1.,0.429856640579733));
#44227=CARTESIAN_POINT('Ctrl Pts',(-3.88414070943334,1.,0.429856640579733));
#44228=CARTESIAN_POINT('Ctrl Pts',(-3.89104947940592,-1.,0.432713929544439));
#44229=CARTESIAN_POINT('Ctrl Pts',(-3.89104947940592,1.,0.432713929544439));
#44230=CARTESIAN_POINT('Ctrl Pts',(-3.8979725665544,-1.,0.435624629433505));
#44231=CARTESIAN_POINT('Ctrl Pts',(-3.8979725665544,1.,0.435624629433505));
#44232=CARTESIAN_POINT('Ctrl Pts',(-3.90490512938546,-1.,0.438587235458233));
#44233=CARTESIAN_POINT('Ctrl Pts',(-3.90490512938546,1.,0.438587235458233));
#44234=CARTESIAN_POINT('Ctrl Pts',(-3.91183704069146,-1.,0.441599824524047));
#44235=CARTESIAN_POINT('Ctrl Pts',(-3.91183704069146,1.,0.441599824524047));
#44236=CARTESIAN_POINT('Ctrl Pts',(-3.91875701610721,-1.,0.444660430230592));
#44237=CARTESIAN_POINT('Ctrl Pts',(-3.91875701610721,1.,0.444660430230592));
#44238=CARTESIAN_POINT('Ctrl Pts',(-3.92565674143424,-1.,0.447767416837296));
#44239=CARTESIAN_POINT('Ctrl Pts',(-3.92565674143424,1.,0.447767416837296));
#44240=CARTESIAN_POINT('Ctrl Pts',(-3.93253407403128,-1.,0.450919768356347));
#44241=CARTESIAN_POINT('Ctrl Pts',(-3.93253407403128,1.,0.450919768356347));
#44242=CARTESIAN_POINT('Ctrl Pts',(-3.93939080846298,-1.,0.454116879027576));
#44243=CARTESIAN_POINT('Ctrl Pts',(-3.93939080846298,1.,0.454116879027576));
#44244=CARTESIAN_POINT('Ctrl Pts',(-3.94623117206675,-1.,0.457358410451674));
#44245=CARTESIAN_POINT('Ctrl Pts',(-3.94623117206675,1.,0.457358410451674));
#44246=CARTESIAN_POINT('Ctrl Pts',(-3.95306005817363,-1.,0.460644124429119));
#44247=CARTESIAN_POINT('Ctrl Pts',(-3.95306005817363,1.,0.460644124429119));
#44248=CARTESIAN_POINT('Ctrl Pts',(-3.95988133243543,-1.,0.463973722115744));
#44249=CARTESIAN_POINT('Ctrl Pts',(-3.95988133243543,1.,0.463973722115744));
#44250=CARTESIAN_POINT('Ctrl Pts',(-3.96669622273946,-1.,0.467346690880671));
#44251=CARTESIAN_POINT('Ctrl Pts',(-3.96669622273946,1.,0.467346690880671));
#44252=CARTESIAN_POINT('Ctrl Pts',(-3.97350414289415,-1.,0.470762379613477));
#44253=CARTESIAN_POINT('Ctrl Pts',(-3.97350414289415,1.,0.470762379613477));
#44254=CARTESIAN_POINT('Ctrl Pts',(-3.9803033804443,-1.,0.474220061019542));
#44255=CARTESIAN_POINT('Ctrl Pts',(-3.9803033804443,1.,0.474220061019542));
#44256=CARTESIAN_POINT('Ctrl Pts',(-3.98709184306743,-1.,0.477718999122033));
#44257=CARTESIAN_POINT('Ctrl Pts',(-3.98709184306743,1.,0.477718999122033));
#44258=CARTESIAN_POINT('Ctrl Pts',(-3.99386775880655,-1.,0.481258512209638));
#44259=CARTESIAN_POINT('Ctrl Pts',(-3.99386775880655,1.,0.481258512209638));
#44260=CARTESIAN_POINT('Ctrl Pts',(-4.00063045119234,-1.,0.484838042421754));
#44261=CARTESIAN_POINT('Ctrl Pts',(-4.00063045119234,1.,0.484838042421754));
#44262=CARTESIAN_POINT('Ctrl Pts',(-4.0073800839092,-1.,0.48845713042453));
#44263=CARTESIAN_POINT('Ctrl Pts',(-4.0073800839092,1.,0.48845713042453));
#44264=CARTESIAN_POINT('Ctrl Pts',(-4.01411733503486,-1.,0.49211538341793));
#44265=CARTESIAN_POINT('Ctrl Pts',(-4.01411733503486,1.,0.49211538341793));
#44266=CARTESIAN_POINT('Ctrl Pts',(-4.02084308851813,-1.,0.495812444326223));
#44267=CARTESIAN_POINT('Ctrl Pts',(-4.02084308851813,1.,0.495812444326223));
#44268=CARTESIAN_POINT('Ctrl Pts',(-4.0275581398015,-1.,0.499547962340889));
#44269=CARTESIAN_POINT('Ctrl Pts',(-4.0275581398015,1.,0.499547962340889));
#44270=CARTESIAN_POINT('Ctrl Pts',(-4.0342628417439,-1.,0.503321556915513));
#44271=CARTESIAN_POINT('Ctrl Pts',(-4.0342628417439,1.,0.503321556915513));
#44272=CARTESIAN_POINT('Ctrl Pts',(-4.04095715149074,-1.,0.507132823288361));
#44273=CARTESIAN_POINT('Ctrl Pts',(-4.04095715149074,1.,0.507132823288361));
#44274=CARTESIAN_POINT('Ctrl Pts',(-4.04764078815591,-1.,0.510981349219173));
#44275=CARTESIAN_POINT('Ctrl Pts',(-4.04764078815591,1.,0.510981349219173));
#44276=CARTESIAN_POINT('Ctrl Pts',(-4.05431335771261,-1.,0.514866728193104));
#44277=CARTESIAN_POINT('Ctrl Pts',(-4.05431335771261,1.,0.514866728193104));
#44278=CARTESIAN_POINT('Ctrl Pts',(-4.06097448037934,-1.,0.518788572336809));
#44279=CARTESIAN_POINT('Ctrl Pts',(-4.06097448037934,1.,0.518788572336809));
#44280=CARTESIAN_POINT('Ctrl Pts',(-4.06762394471075,-1.,0.522746528602767));
#44281=CARTESIAN_POINT('Ctrl Pts',(-4.06762394471075,1.,0.522746528602767));
#44282=CARTESIAN_POINT('Ctrl Pts',(-4.07426172299496,-1.,0.526740277226999));
#44283=CARTESIAN_POINT('Ctrl Pts',(-4.07426172299496,1.,0.526740277226999));
#44284=CARTESIAN_POINT('Ctrl Pts',(-4.08088789536488,-1.,0.530769518728075));
#44285=CARTESIAN_POINT('Ctrl Pts',(-4.08088789536488,1.,0.530769518728075));
#44286=CARTESIAN_POINT('Ctrl Pts',(-4.08750259988693,-1.,0.534833963476999));
#44287=CARTESIAN_POINT('Ctrl Pts',(-4.08750259988693,1.,0.534833963476999));
#44288=CARTESIAN_POINT('Ctrl Pts',(-4.09410597627116,-1.,0.53893332117992));
#44289=CARTESIAN_POINT('Ctrl Pts',(-4.09410597627116,1.,0.53893332117992));
#44290=CARTESIAN_POINT('Ctrl Pts',(-4.10069810244473,-1.,0.543067286878457));
#44291=CARTESIAN_POINT('Ctrl Pts',(-4.10069810244473,1.,0.543067286878457));
#44292=CARTESIAN_POINT('Ctrl Pts',(-4.1072789702877,-1.,0.547235539486759));
#44293=CARTESIAN_POINT('Ctrl Pts',(-4.1072789702877,1.,0.547235539486759));
#44294=CARTESIAN_POINT('Ctrl Pts',(-4.11384852025578,-1.,0.551437758498246));
#44295=CARTESIAN_POINT('Ctrl Pts',(-4.11384852025578,1.,0.551437758498246));
#44296=CARTESIAN_POINT('Ctrl Pts',(-4.1204066619623,-1.,0.555673636130778));
#44297=CARTESIAN_POINT('Ctrl Pts',(-4.1204066619623,1.,0.555673636130778));
#44298=CARTESIAN_POINT('Ctrl Pts',(-4.12695329951859,-1.,0.559942890594628));
#44299=CARTESIAN_POINT('Ctrl Pts',(-4.12695329951859,1.,0.559942890594628));
#44300=CARTESIAN_POINT('Ctrl Pts',(-4.13348835726086,-1.,0.564245279535705));
#44301=CARTESIAN_POINT('Ctrl Pts',(-4.13348835726086,1.,0.564245279535705));
#44302=CARTESIAN_POINT('Ctrl Pts',(-4.14001179828669,-1.,0.568580610187116));
#44303=CARTESIAN_POINT('Ctrl Pts',(-4.14001179828669,1.,0.568580610187116));
#44304=CARTESIAN_POINT('Ctrl Pts',(-4.14652361065787,-1.,0.572948736066276));
#44305=CARTESIAN_POINT('Ctrl Pts',(-4.14652361065787,1.,0.572948736066276));
#44306=CARTESIAN_POINT('Ctrl Pts',(-4.1517237611974,-1.,0.576469391673916));
#44307=CARTESIAN_POINT('Ctrl Pts',(-4.1517237611974,1.,0.576469391673916));
#44308=CARTESIAN_POINT('Ctrl Pts',(-4.15561864787379,-1.,0.579124568912543));
#44309=CARTESIAN_POINT('Ctrl Pts',(-4.15561864787379,1.,0.579124568912543));
#44310=CARTESIAN_POINT('Ctrl Pts',(-4.15821291712391,-1.,0.580901211462913));
#44311=CARTESIAN_POINT('Ctrl Pts',(-4.15821291712391,1.,0.580901211462913));
#44312=CARTESIAN_POINT('Ctrl Pts',(-4.15950947128175,-1.,0.581791163835814));
#44313=CARTESIAN_POINT('Ctrl Pts',(-4.15950947128175,1.,0.581791163835814));
#44314=CARTESIAN_POINT('',(-3.73017266276632,1.,0.385112848332549));
#44315=CARTESIAN_POINT('Ctrl Pts',(-3.73017266276632,-1.,0.385112848332549));
#44316=CARTESIAN_POINT('Ctrl Pts',(-3.73017266276632,-0.666666666666667,
0.385112848332549));
#44317=CARTESIAN_POINT('Ctrl Pts',(-3.73017266276632,-0.333333333333333,
0.385112848332549));
#44318=CARTESIAN_POINT('Ctrl Pts',(-3.73017266276632,0.333333333333333,
0.385112848332549));
#44319=CARTESIAN_POINT('Ctrl Pts',(-3.73017266276632,0.666666666666667,
0.385112848332549));
#44320=CARTESIAN_POINT('Ctrl Pts',(-3.73017266276632,1.,0.385112848332549));
#44321=CARTESIAN_POINT('',(-4.15950947128175,1.,0.581791163835814));
#44322=CARTESIAN_POINT('',(-4.15950947128175,0.,0.581791163835814));
#44323=CARTESIAN_POINT('Ctrl Pts',(-3.73017266276632,1.,0.385112848332549));
#44324=CARTESIAN_POINT('Ctrl Pts',(-3.73021431755218,1.,0.385087139001609));
#44325=CARTESIAN_POINT('Ctrl Pts',(-3.73040527620929,1.,0.385037797882046));
#44326=CARTESIAN_POINT('Ctrl Pts',(-3.73106082862399,1.,0.385031656499141));
#44327=CARTESIAN_POINT('Ctrl Pts',(-3.73273893363318,1.,0.385187124633964));
#44328=CARTESIAN_POINT('Ctrl Pts',(-3.73621371845475,1.,0.385670806454744));
#44329=CARTESIAN_POINT('Ctrl Pts',(-3.74144965781088,1.,0.386519576222035));
#44330=CARTESIAN_POINT('Ctrl Pts',(-3.74792651696269,1.,0.387663020050396));
#44331=CARTESIAN_POINT('Ctrl Pts',(-3.75529302894757,1.,0.389054775898251));
#44332=CARTESIAN_POINT('Ctrl Pts',(-3.76315635032993,1.,0.390642072979259));
#44333=CARTESIAN_POINT('Ctrl Pts',(-3.77114011595892,1.,0.392372786223346));
#44334=CARTESIAN_POINT('Ctrl Pts',(-3.77894173114368,1.,0.394202481011595));
#44335=CARTESIAN_POINT('Ctrl Pts',(-3.78640521279479,1.,0.396103205335028));
#44336=CARTESIAN_POINT('Ctrl Pts',(-3.79352887163457,1.,0.398064818684158));
#44337=CARTESIAN_POINT('Ctrl Pts',(-3.80040370384659,1.,0.400088346504726));
#44338=CARTESIAN_POINT('Ctrl Pts',(-3.80716881962763,1.,0.402181320148474));
#44339=CARTESIAN_POINT('Ctrl Pts',(-3.81396374287762,1.,0.404352694628236));
#44340=CARTESIAN_POINT('Ctrl Pts',(-3.82087303913741,1.,0.406607038258906));
#44341=CARTESIAN_POINT('Ctrl Pts',(-3.82790724256397,1.,0.408942371447377));
#44342=CARTESIAN_POINT('Ctrl Pts',(-3.83503345578645,1.,0.411353038798459));
#44343=CARTESIAN_POINT('Ctrl Pts',(-3.84219403994742,1.,0.413831367016726));
#44344=CARTESIAN_POINT('Ctrl Pts',(-3.8493286415751,1.,0.41636967805292));
#44345=CARTESIAN_POINT('Ctrl Pts',(-3.85639825648031,1.,0.418962468086809));
#44346=CARTESIAN_POINT('Ctrl Pts',(-3.86339652542749,1.,0.421607423177575));
#44347=CARTESIAN_POINT('Ctrl Pts',(-3.87033643487882,1.,0.424304173195142));
#44348=CARTESIAN_POINT('Ctrl Pts',(-3.87724240306609,1.,0.427053541173469));
#44349=CARTESIAN_POINT('Ctrl Pts',(-3.88414070943334,1.,0.429856640579733));
#44350=CARTESIAN_POINT('Ctrl Pts',(-3.89104947940592,1.,0.432713929544439));
#44351=CARTESIAN_POINT('Ctrl Pts',(-3.8979725665544,1.,0.435624629433505));
#44352=CARTESIAN_POINT('Ctrl Pts',(-3.90490512938546,1.,0.438587235458233));
#44353=CARTESIAN_POINT('Ctrl Pts',(-3.91183704069146,1.,0.441599824524047));
#44354=CARTESIAN_POINT('Ctrl Pts',(-3.91875701610721,1.,0.444660430230592));
#44355=CARTESIAN_POINT('Ctrl Pts',(-3.92565674143424,1.,0.447767416837296));
#44356=CARTESIAN_POINT('Ctrl Pts',(-3.93253407403128,1.,0.450919768356347));
#44357=CARTESIAN_POINT('Ctrl Pts',(-3.93939080846298,1.,0.454116879027576));
#44358=CARTESIAN_POINT('Ctrl Pts',(-3.94623117206675,1.,0.457358410451674));
#44359=CARTESIAN_POINT('Ctrl Pts',(-3.95306005817363,1.,0.460644124429119));
#44360=CARTESIAN_POINT('Ctrl Pts',(-3.95988133243543,1.,0.463973722115744));
#44361=CARTESIAN_POINT('Ctrl Pts',(-3.96669622273946,1.,0.467346690880671));
#44362=CARTESIAN_POINT('Ctrl Pts',(-3.97350414289415,1.,0.470762379613477));
#44363=CARTESIAN_POINT('Ctrl Pts',(-3.9803033804443,1.,0.474220061019542));
#44364=CARTESIAN_POINT('Ctrl Pts',(-3.98709184306743,1.,0.477718999122033));
#44365=CARTESIAN_POINT('Ctrl Pts',(-3.99386775880655,1.,0.481258512209638));
#44366=CARTESIAN_POINT('Ctrl Pts',(-4.00063045119234,1.,0.484838042421754));
#44367=CARTESIAN_POINT('Ctrl Pts',(-4.0073800839092,1.,0.48845713042453));
#44368=CARTESIAN_POINT('Ctrl Pts',(-4.01411733503486,1.,0.49211538341793));
#44369=CARTESIAN_POINT('Ctrl Pts',(-4.02084308851813,1.,0.495812444326223));
#44370=CARTESIAN_POINT('Ctrl Pts',(-4.0275581398015,1.,0.499547962340889));
#44371=CARTESIAN_POINT('Ctrl Pts',(-4.0342628417439,1.,0.503321556915513));
#44372=CARTESIAN_POINT('Ctrl Pts',(-4.04095715149074,1.,0.507132823288361));
#44373=CARTESIAN_POINT('Ctrl Pts',(-4.04764078815591,1.,0.510981349219173));
#44374=CARTESIAN_POINT('Ctrl Pts',(-4.05431335771261,1.,0.514866728193104));
#44375=CARTESIAN_POINT('Ctrl Pts',(-4.06097448037934,1.,0.518788572336809));
#44376=CARTESIAN_POINT('Ctrl Pts',(-4.06762394471075,1.,0.522746528602767));
#44377=CARTESIAN_POINT('Ctrl Pts',(-4.07426172299496,1.,0.526740277226999));
#44378=CARTESIAN_POINT('Ctrl Pts',(-4.08088789536488,1.,0.530769518728075));
#44379=CARTESIAN_POINT('Ctrl Pts',(-4.08750259988693,1.,0.534833963476999));
#44380=CARTESIAN_POINT('Ctrl Pts',(-4.09410597627116,1.,0.53893332117992));
#44381=CARTESIAN_POINT('Ctrl Pts',(-4.10069810244473,1.,0.543067286878457));
#44382=CARTESIAN_POINT('Ctrl Pts',(-4.1072789702877,1.,0.547235539486759));
#44383=CARTESIAN_POINT('Ctrl Pts',(-4.11384852025578,1.,0.551437758498246));
#44384=CARTESIAN_POINT('Ctrl Pts',(-4.1204066619623,1.,0.555673636130778));
#44385=CARTESIAN_POINT('Ctrl Pts',(-4.12695329951859,1.,0.559942890594628));
#44386=CARTESIAN_POINT('Ctrl Pts',(-4.13348835726086,1.,0.564245279535705));
#44387=CARTESIAN_POINT('Ctrl Pts',(-4.14001179828669,1.,0.568580610187116));
#44388=CARTESIAN_POINT('Ctrl Pts',(-4.14652361065787,1.,0.572948736066276));
#44389=CARTESIAN_POINT('Ctrl Pts',(-4.1517237611974,1.,0.576469391673916));
#44390=CARTESIAN_POINT('Ctrl Pts',(-4.15561864787379,1.,0.579124568912543));
#44391=CARTESIAN_POINT('Ctrl Pts',(-4.15821291712391,1.,0.580901211462913));
#44392=CARTESIAN_POINT('Ctrl Pts',(-4.15950947128175,1.,0.581791163835814));
#44393=CARTESIAN_POINT('Origin',(-4.15950947128175,0.,0.581791163835814));
#44394=CARTESIAN_POINT('',(-4.13571194405636,1.,0.732042837400619));
#44395=CARTESIAN_POINT('Origin',(0.,0.,0.));
#44396=CARTESIAN_POINT('',(-3.74449296982994,1.,0.203156094897896));
#44397=CARTESIAN_POINT('Origin',(0.,1.,0.));
#44398=CARTESIAN_POINT('Ctrl Pts',(-3.74449296982994,1.,0.203156094897896));
#44399=CARTESIAN_POINT('Ctrl Pts',(-3.74449296982994,0.666666666666667,
0.203156094897896));
#44400=CARTESIAN_POINT('Ctrl Pts',(-3.74449296982994,0.333333333333333,
0.203156094897896));
#44401=CARTESIAN_POINT('Ctrl Pts',(-3.74449296982994,-0.333333333333333,
0.203156094897896));
#44402=CARTESIAN_POINT('Ctrl Pts',(-3.74449296982994,-0.666666666666667,
0.203156094897896));
#44403=CARTESIAN_POINT('Ctrl Pts',(-3.74449296982994,-1.,0.203156094897896));
#44404=CARTESIAN_POINT('Ctrl Pts',(-4.19931119685982,-1.,0.0760622897878236));
#44405=CARTESIAN_POINT('Ctrl Pts',(-4.19931119685982,1.,0.0760622897878236));
#44406=CARTESIAN_POINT('Ctrl Pts',(-4.19789138621624,-1.,0.0767384596142195));
#44407=CARTESIAN_POINT('Ctrl Pts',(-4.19789138621624,1.,0.0767384596142195));
#44408=CARTESIAN_POINT('Ctrl Pts',(-4.19505112860624,-1.,0.0780873956244402));
#44409=CARTESIAN_POINT('Ctrl Pts',(-4.19505112860624,1.,0.0780873956244402));
#44410=CARTESIAN_POINT('Ctrl Pts',(-4.19078883322483,-1.,0.0801005887117603));
#44411=CARTESIAN_POINT('Ctrl Pts',(-4.19078883322483,1.,0.0801005887117603));
#44412=CARTESIAN_POINT('Ctrl Pts',(-4.1851019532944,-1.,0.082764416438951));
#44413=CARTESIAN_POINT('Ctrl Pts',(-4.1851019532944,1.,0.082764416438951));
#44414=CARTESIAN_POINT('Ctrl Pts',(-4.17798698669991,-1.,0.0860600915552515));
#44415=CARTESIAN_POINT('Ctrl Pts',(-4.17798698669991,1.,0.0860600915552515));
#44416=CARTESIAN_POINT('Ctrl Pts',(-4.17086566491823,-1.,0.0893215560850327));
#44417=CARTESIAN_POINT('Ctrl Pts',(-4.17086566491823,1.,0.0893215560850327));
#44418=CARTESIAN_POINT('Ctrl Pts',(-4.16373802265942,-1.,0.092548667216769));
#44419=CARTESIAN_POINT('Ctrl Pts',(-4.16373802265942,1.,0.092548667216769));
#44420=CARTESIAN_POINT('Ctrl Pts',(-4.15660412653006,-1.,0.0957412403297067));
#44421=CARTESIAN_POINT('Ctrl Pts',(-4.15660412653006,1.,0.0957412403297067));
#44422=CARTESIAN_POINT('Ctrl Pts',(-4.1494640891762,-1.,0.0988990478899811));
#44423=CARTESIAN_POINT('Ctrl Pts',(-4.1494640891762,1.,0.0988990478899811));
#44424=CARTESIAN_POINT('Ctrl Pts',(-4.14231804938737,-1.,0.102021826577454));
#44425=CARTESIAN_POINT('Ctrl Pts',(-4.14231804938737,1.,0.102021826577454));
#44426=CARTESIAN_POINT('Ctrl Pts',(-4.13516614458396,-1.,0.105109286538864));
#44427=CARTESIAN_POINT('Ctrl Pts',(-4.13516614458396,1.,0.105109286538864));
#44428=CARTESIAN_POINT('Ctrl Pts',(-4.12800848371386,-1.,0.10816112052835));
#44429=CARTESIAN_POINT('Ctrl Pts',(-4.12800848371386,1.,0.10816112052835));
#44430=CARTESIAN_POINT('Ctrl Pts',(-4.12084512502444,-1.,0.111177012683377));
#44431=CARTESIAN_POINT('Ctrl Pts',(-4.12084512502444,1.,0.111177012683377));
#44432=CARTESIAN_POINT('Ctrl Pts',(-4.11367603925313,-1.,0.114156649609601));
#44433=CARTESIAN_POINT('Ctrl Pts',(-4.11367603925313,1.,0.114156649609601));
#44434=CARTESIAN_POINT('Ctrl Pts',(-4.10650113382187,-1.,0.117099722731704));
#44435=CARTESIAN_POINT('Ctrl Pts',(-4.10650113382187,1.,0.117099722731704));
#44436=CARTESIAN_POINT('Ctrl Pts',(-4.09932031767243,-1.,0.120005924388162));
#44437=CARTESIAN_POINT('Ctrl Pts',(-4.09932031767243,1.,0.120005924388162));
#44438=CARTESIAN_POINT('Ctrl Pts',(-4.09213355850836,-1.,0.122874946249119));
#44439=CARTESIAN_POINT('Ctrl Pts',(-4.09213355850836,1.,0.122874946249119));
#44440=CARTESIAN_POINT('Ctrl Pts',(-4.08494093372315,-1.,0.125706476822529));
#44441=CARTESIAN_POINT('Ctrl Pts',(-4.08494093372315,1.,0.125706476822529));
#44442=CARTESIAN_POINT('Ctrl Pts',(-4.07774270738809,-1.,0.128500200484814));
#44443=CARTESIAN_POINT('Ctrl Pts',(-4.07774270738809,1.,0.128500200484814));
#44444=CARTESIAN_POINT('Ctrl Pts',(-4.07053931528579,-1.,0.131255793548914));
#44445=CARTESIAN_POINT('Ctrl Pts',(-4.07053931528579,1.,0.131255793548914));
#44446=CARTESIAN_POINT('Ctrl Pts',(-4.06333121018476,-1.,0.133972916144225));
#44447=CARTESIAN_POINT('Ctrl Pts',(-4.06333121018476,1.,0.133972916144225));
#44448=CARTESIAN_POINT('Ctrl Pts',(-4.05611873400122,-1.,0.136651205046111));
#44449=CARTESIAN_POINT('Ctrl Pts',(-4.05611873400122,1.,0.136651205046111));
#44450=CARTESIAN_POINT('Ctrl Pts',(-4.04890199238056,-1.,0.139290267180059));
#44451=CARTESIAN_POINT('Ctrl Pts',(-4.04890199238056,1.,0.139290267180059));
#44452=CARTESIAN_POINT('Ctrl Pts',(-4.04168069633842,-1.,0.141889671485508));
#44453=CARTESIAN_POINT('Ctrl Pts',(-4.04168069633842,1.,0.141889671485508));
#44454=CARTESIAN_POINT('Ctrl Pts',(-4.03445411510403,-1.,0.144448947038352));
#44455=CARTESIAN_POINT('Ctrl Pts',(-4.03445411510403,1.,0.144448947038352));
#44456=CARTESIAN_POINT('Ctrl Pts',(-4.02722143147048,-1.,0.146967602878998));
#44457=CARTESIAN_POINT('Ctrl Pts',(-4.02722143147048,1.,0.146967602878998));
#44458=CARTESIAN_POINT('Ctrl Pts',(-4.01998203715588,-1.,0.149445144968707));
#44459=CARTESIAN_POINT('Ctrl Pts',(-4.01998203715588,1.,0.149445144968707));
#44460=CARTESIAN_POINT('Ctrl Pts',(-4.01273584234684,-1.,0.151881094022909));
#44461=CARTESIAN_POINT('Ctrl Pts',(-4.01273584234684,1.,0.151881094022909));
#44462=CARTESIAN_POINT('Ctrl Pts',(-4.00548360245297,-1.,0.15427500487231));
#44463=CARTESIAN_POINT('Ctrl Pts',(-4.00548360245297,1.,0.15427500487231));
#44464=CARTESIAN_POINT('Ctrl Pts',(-3.99822717425869,-1.,0.156626481393735));
#44465=CARTESIAN_POINT('Ctrl Pts',(-3.99822717425869,1.,0.156626481393735));
#44466=CARTESIAN_POINT('Ctrl Pts',(-3.99096873945862,-1.,0.158935123982796));
#44467=CARTESIAN_POINT('Ctrl Pts',(-3.99096873945862,1.,0.158935123982796));
#44468=CARTESIAN_POINT('Ctrl Pts',(-3.98371010319866,-1.,0.161200482186087));
#44469=CARTESIAN_POINT('Ctrl Pts',(-3.98371010319866,1.,0.161200482186087));
#44470=CARTESIAN_POINT('Ctrl Pts',(-3.97645194630944,-1.,0.163422004609999));
#44471=CARTESIAN_POINT('Ctrl Pts',(-3.97645194630944,1.,0.163422004609999));
#44472=CARTESIAN_POINT('Ctrl Pts',(-3.9691931362141,-1.,0.165598992851097));
#44473=CARTESIAN_POINT('Ctrl Pts',(-3.9691931362141,1.,0.165598992851097));
#44474=CARTESIAN_POINT('Ctrl Pts',(-3.96192990160296,-1.,0.167730547023312));
#44475=CARTESIAN_POINT('Ctrl Pts',(-3.96192990160296,1.,0.167730547023312));
#44476=CARTESIAN_POINT('Ctrl Pts',(-3.95465744665263,-1.,0.16981566637413));
#44477=CARTESIAN_POINT('Ctrl Pts',(-3.95465744665263,1.,0.16981566637413));
#44478=CARTESIAN_POINT('Ctrl Pts',(-3.94737164900861,-1.,0.171853355369233));
#44479=CARTESIAN_POINT('Ctrl Pts',(-3.94737164900861,1.,0.171853355369233));
#44480=CARTESIAN_POINT('Ctrl Pts',(-3.94007083096214,-1.,0.173842734974607));
#44481=CARTESIAN_POINT('Ctrl Pts',(-3.94007083096214,1.,0.173842734974607));
#44482=CARTESIAN_POINT('Ctrl Pts',(-3.93275726771049,-1.,0.175783136893872));
#44483=CARTESIAN_POINT('Ctrl Pts',(-3.93275726771049,1.,0.175783136893872));
#44484=CARTESIAN_POINT('Ctrl Pts',(-3.92543942697672,-1.,0.177674246152328));
#44485=CARTESIAN_POINT('Ctrl Pts',(-3.92543942697672,1.,0.177674246152328));
#44486=CARTESIAN_POINT('Ctrl Pts',(-3.91812876180948,-1.,0.179515885822894));
#44487=CARTESIAN_POINT('Ctrl Pts',(-3.91812876180948,1.,0.179515885822894));
#44488=CARTESIAN_POINT('Ctrl Pts',(-3.91083557557193,-1.,0.181307740731796));
#44489=CARTESIAN_POINT('Ctrl Pts',(-3.91083557557193,1.,0.181307740731796));
#44490=CARTESIAN_POINT('Ctrl Pts',(-3.90356488555138,-1.,0.183049081993193));
#44491=CARTESIAN_POINT('Ctrl Pts',(-3.90356488555138,1.,0.183049081993193));
#44492=CARTESIAN_POINT('Ctrl Pts',(-3.89631300742633,-1.,0.184738537728035));
#44493=CARTESIAN_POINT('Ctrl Pts',(-3.89631300742633,1.,0.184738537728035));
#44494=CARTESIAN_POINT('Ctrl Pts',(-3.88906196725817,-1.,0.186373724985263));
#44495=CARTESIAN_POINT('Ctrl Pts',(-3.88906196725817,1.,0.186373724985263));
#44496=CARTESIAN_POINT('Ctrl Pts',(-3.88178563496187,-1.,0.187951632512663));
#44497=CARTESIAN_POINT('Ctrl Pts',(-3.88178563496187,1.,0.187951632512663));
#44498=CARTESIAN_POINT('Ctrl Pts',(-3.87445976418377,-1.,0.189469253358254));
#44499=CARTESIAN_POINT('Ctrl Pts',(-3.87445976418377,1.,0.189469253358254));
#44500=CARTESIAN_POINT('Ctrl Pts',(-3.8670715862477,-1.,0.190924190418613));
#44501=CARTESIAN_POINT('Ctrl Pts',(-3.8670715862477,1.,0.190924190418613));
#44502=CARTESIAN_POINT('Ctrl Pts',(-3.85962774407652,-1.,0.192315153044979));
#44503=CARTESIAN_POINT('Ctrl Pts',(-3.85962774407652,1.,0.192315153044979));
#44504=CARTESIAN_POINT('Ctrl Pts',(-3.85216762264019,-1.,0.193642806777747));
#44505=CARTESIAN_POINT('Ctrl Pts',(-3.85216762264019,1.,0.193642806777747));
#44506=CARTESIAN_POINT('Ctrl Pts',(-3.84475203347052,-1.,0.194909009460254));
#44507=CARTESIAN_POINT('Ctrl Pts',(-3.84475203347052,1.,0.194909009460254));
#44508=CARTESIAN_POINT('Ctrl Pts',(-3.83743910616265,-1.,0.196115198971889));
#44509=CARTESIAN_POINT('Ctrl Pts',(-3.83743910616265,1.,0.196115198971889));
#44510=CARTESIAN_POINT('Ctrl Pts',(-3.83026221776488,-1.,0.197260935827375));
#44511=CARTESIAN_POINT('Ctrl Pts',(-3.83026221776488,1.,0.197260935827375));
#44512=CARTESIAN_POINT('Ctrl Pts',(-3.82321127348981,-1.,0.19834261690047));
#44513=CARTESIAN_POINT('Ctrl Pts',(-3.82321127348981,1.,0.19834261690047));
#44514=CARTESIAN_POINT('Ctrl Pts',(-3.81620203429702,-1.,0.199351525297396));
#44515=CARTESIAN_POINT('Ctrl Pts',(-3.81620203429702,1.,0.199351525297396));
#44516=CARTESIAN_POINT('Ctrl Pts',(-3.80909529318501,-1.,0.20027467943329));
#44517=CARTESIAN_POINT('Ctrl Pts',(-3.80909529318501,1.,0.20027467943329));
#44518=CARTESIAN_POINT('Ctrl Pts',(-3.80175247447171,-1.,0.201097756307252));
#44519=CARTESIAN_POINT('Ctrl Pts',(-3.80175247447171,1.,0.201097756307252));
#44520=CARTESIAN_POINT('Ctrl Pts',(-3.79408354187274,-1.,0.201807533800799));
#44521=CARTESIAN_POINT('Ctrl Pts',(-3.79408354187274,1.,0.201807533800799));
#44522=CARTESIAN_POINT('Ctrl Pts',(-3.78609175019317,-1.,0.202394260512193));
#44523=CARTESIAN_POINT('Ctrl Pts',(-3.78609175019317,1.,0.202394260512193));
#44524=CARTESIAN_POINT('Ctrl Pts',(-3.77793553476879,-1.,0.202854729699196));
#44525=CARTESIAN_POINT('Ctrl Pts',(-3.77793553476879,1.,0.202854729699196));
#44526=CARTESIAN_POINT('Ctrl Pts',(-3.76992071595267,-1.,0.203192390045337));
#44527=CARTESIAN_POINT('Ctrl Pts',(-3.76992071595267,1.,0.203192390045337));
#44528=CARTESIAN_POINT('Ctrl Pts',(-3.76242717937273,-1.,0.203414634707646));
#44529=CARTESIAN_POINT('Ctrl Pts',(-3.76242717937273,1.,0.203414634707646));
#44530=CARTESIAN_POINT('Ctrl Pts',(-3.75585118707924,-1.,0.203530796848403));
#44531=CARTESIAN_POINT('Ctrl Pts',(-3.75585118707924,1.,0.203530796848403));
#44532=CARTESIAN_POINT('Ctrl Pts',(-3.75054693397716,-1.,0.203550035479097));
#44533=CARTESIAN_POINT('Ctrl Pts',(-3.75054693397716,1.,0.203550035479097));
#44534=CARTESIAN_POINT('Ctrl Pts',(-3.74675472018582,-1.,0.203478844530229));
#44535=CARTESIAN_POINT('Ctrl Pts',(-3.74675472018582,1.,0.203478844530229));
#44536=CARTESIAN_POINT('Ctrl Pts',(-3.7450208092684,-1.,0.203352057956055));
#44537=CARTESIAN_POINT('Ctrl Pts',(-3.7450208092684,1.,0.203352057956055));
#44538=CARTESIAN_POINT('Ctrl Pts',(-3.74446880195845,-1.,0.203218215747894));
#44539=CARTESIAN_POINT('Ctrl Pts',(-3.74446880195845,1.,0.203218215747894));
#44540=CARTESIAN_POINT('Ctrl Pts',(-3.74443319346666,-1.,0.20311176758786));
#44541=CARTESIAN_POINT('Ctrl Pts',(-3.74443319346666,1.,0.20311176758786));
#44542=CARTESIAN_POINT('Ctrl Pts',(-3.74449849461127,-1.,0.203054238699719));
#44543=CARTESIAN_POINT('Ctrl Pts',(-3.74449849461127,1.,0.203054238699719));
#44544=CARTESIAN_POINT('',(-4.19931119685982,1.,0.0760622897878236));
#44545=CARTESIAN_POINT('Ctrl Pts',(-4.19931119685982,1.,0.0760622897878236));
#44546=CARTESIAN_POINT('Ctrl Pts',(-4.19789138621624,1.,0.0767384596142195));
#44547=CARTESIAN_POINT('Ctrl Pts',(-4.19505112860624,1.,0.0780873956244402));
#44548=CARTESIAN_POINT('Ctrl Pts',(-4.19078883322483,1.,0.0801005887117603));
#44549=CARTESIAN_POINT('Ctrl Pts',(-4.1851019532944,1.,0.082764416438951));
#44550=CARTESIAN_POINT('Ctrl Pts',(-4.17798698669991,1.,0.0860600915552515));
#44551=CARTESIAN_POINT('Ctrl Pts',(-4.17086566491823,1.,0.0893215560850327));
#44552=CARTESIAN_POINT('Ctrl Pts',(-4.16373802265942,1.,0.092548667216769));
#44553=CARTESIAN_POINT('Ctrl Pts',(-4.15660412653006,1.,0.0957412403297067));
#44554=CARTESIAN_POINT('Ctrl Pts',(-4.1494640891762,1.,0.0988990478899811));
#44555=CARTESIAN_POINT('Ctrl Pts',(-4.14231804938737,1.,0.102021826577454));
#44556=CARTESIAN_POINT('Ctrl Pts',(-4.13516614458396,1.,0.105109286538864));
#44557=CARTESIAN_POINT('Ctrl Pts',(-4.12800848371386,1.,0.10816112052835));
#44558=CARTESIAN_POINT('Ctrl Pts',(-4.12084512502444,1.,0.111177012683377));
#44559=CARTESIAN_POINT('Ctrl Pts',(-4.11367603925313,1.,0.114156649609601));
#44560=CARTESIAN_POINT('Ctrl Pts',(-4.10650113382187,1.,0.117099722731704));
#44561=CARTESIAN_POINT('Ctrl Pts',(-4.09932031767243,1.,0.120005924388162));
#44562=CARTESIAN_POINT('Ctrl Pts',(-4.09213355850836,1.,0.122874946249119));
#44563=CARTESIAN_POINT('Ctrl Pts',(-4.08494093372315,1.,0.125706476822529));
#44564=CARTESIAN_POINT('Ctrl Pts',(-4.07774270738809,1.,0.128500200484814));
#44565=CARTESIAN_POINT('Ctrl Pts',(-4.07053931528579,1.,0.131255793548914));
#44566=CARTESIAN_POINT('Ctrl Pts',(-4.06333121018476,1.,0.133972916144225));
#44567=CARTESIAN_POINT('Ctrl Pts',(-4.05611873400122,1.,0.136651205046111));
#44568=CARTESIAN_POINT('Ctrl Pts',(-4.04890199238056,1.,0.139290267180059));
#44569=CARTESIAN_POINT('Ctrl Pts',(-4.04168069633842,1.,0.141889671485508));
#44570=CARTESIAN_POINT('Ctrl Pts',(-4.03445411510403,1.,0.144448947038352));
#44571=CARTESIAN_POINT('Ctrl Pts',(-4.02722143147048,1.,0.146967602878998));
#44572=CARTESIAN_POINT('Ctrl Pts',(-4.01998203715588,1.,0.149445144968707));
#44573=CARTESIAN_POINT('Ctrl Pts',(-4.01273584234684,1.,0.151881094022909));
#44574=CARTESIAN_POINT('Ctrl Pts',(-4.00548360245297,1.,0.15427500487231));
#44575=CARTESIAN_POINT('Ctrl Pts',(-3.99822717425869,1.,0.156626481393735));
#44576=CARTESIAN_POINT('Ctrl Pts',(-3.99096873945862,1.,0.158935123982796));
#44577=CARTESIAN_POINT('Ctrl Pts',(-3.98371010319866,1.,0.161200482186087));
#44578=CARTESIAN_POINT('Ctrl Pts',(-3.97645194630944,1.,0.163422004609999));
#44579=CARTESIAN_POINT('Ctrl Pts',(-3.9691931362141,1.,0.165598992851097));
#44580=CARTESIAN_POINT('Ctrl Pts',(-3.96192990160296,1.,0.167730547023312));
#44581=CARTESIAN_POINT('Ctrl Pts',(-3.95465744665263,1.,0.16981566637413));
#44582=CARTESIAN_POINT('Ctrl Pts',(-3.94737164900861,1.,0.171853355369233));
#44583=CARTESIAN_POINT('Ctrl Pts',(-3.94007083096214,1.,0.173842734974607));
#44584=CARTESIAN_POINT('Ctrl Pts',(-3.93275726771049,1.,0.175783136893872));
#44585=CARTESIAN_POINT('Ctrl Pts',(-3.92543942697672,1.,0.177674246152328));
#44586=CARTESIAN_POINT('Ctrl Pts',(-3.91812876180948,1.,0.179515885822894));
#44587=CARTESIAN_POINT('Ctrl Pts',(-3.91083557557193,1.,0.181307740731796));
#44588=CARTESIAN_POINT('Ctrl Pts',(-3.90356488555138,1.,0.183049081993193));
#44589=CARTESIAN_POINT('Ctrl Pts',(-3.89631300742633,1.,0.184738537728035));
#44590=CARTESIAN_POINT('Ctrl Pts',(-3.88906196725817,1.,0.186373724985263));
#44591=CARTESIAN_POINT('Ctrl Pts',(-3.88178563496187,1.,0.187951632512663));
#44592=CARTESIAN_POINT('Ctrl Pts',(-3.87445976418377,1.,0.189469253358254));
#44593=CARTESIAN_POINT('Ctrl Pts',(-3.8670715862477,1.,0.190924190418613));
#44594=CARTESIAN_POINT('Ctrl Pts',(-3.85962774407652,1.,0.192315153044979));
#44595=CARTESIAN_POINT('Ctrl Pts',(-3.85216762264019,1.,0.193642806777747));
#44596=CARTESIAN_POINT('Ctrl Pts',(-3.84475203347052,1.,0.194909009460254));
#44597=CARTESIAN_POINT('Ctrl Pts',(-3.83743910616265,1.,0.196115198971889));
#44598=CARTESIAN_POINT('Ctrl Pts',(-3.83026221776488,1.,0.197260935827375));
#44599=CARTESIAN_POINT('Ctrl Pts',(-3.82321127348981,1.,0.19834261690047));
#44600=CARTESIAN_POINT('Ctrl Pts',(-3.81620203429702,1.,0.199351525297396));
#44601=CARTESIAN_POINT('Ctrl Pts',(-3.80909529318501,1.,0.20027467943329));
#44602=CARTESIAN_POINT('Ctrl Pts',(-3.80175247447171,1.,0.201097756307252));
#44603=CARTESIAN_POINT('Ctrl Pts',(-3.79408354187274,1.,0.201807533800799));
#44604=CARTESIAN_POINT('Ctrl Pts',(-3.78609175019317,1.,0.202394260512193));
#44605=CARTESIAN_POINT('Ctrl Pts',(-3.77793553476879,1.,0.202854729699196));
#44606=CARTESIAN_POINT('Ctrl Pts',(-3.76992071595267,1.,0.203192390045337));
#44607=CARTESIAN_POINT('Ctrl Pts',(-3.76242717937273,1.,0.203414634707646));
#44608=CARTESIAN_POINT('Ctrl Pts',(-3.75585118707924,1.,0.203530796848403));
#44609=CARTESIAN_POINT('Ctrl Pts',(-3.75054693397716,1.,0.203550035479097));
#44610=CARTESIAN_POINT('Ctrl Pts',(-3.74703926501843,1.,0.203484186269314));
#44611=CARTESIAN_POINT('Ctrl Pts',(-3.74535749969262,1.,0.203375226874331));
#44612=CARTESIAN_POINT('Ctrl Pts',(-3.74471097893961,1.,0.203266610111264));
#44613=CARTESIAN_POINT('Ctrl Pts',(-3.74453008995129,1.,0.203188003947965));
#44614=CARTESIAN_POINT('Ctrl Pts',(-3.74449296982994,1.,0.203156094897896));
#44615=CARTESIAN_POINT('',(-4.19931119685982,0.,0.0760622897878236));
#44616=CARTESIAN_POINT('Ctrl Pts',(-3.74449849461127,-1.,-0.20305423869972));
#44617=CARTESIAN_POINT('Ctrl Pts',(-3.74449849461127,1.,-0.20305423869972));
#44618=CARTESIAN_POINT('Ctrl Pts',(-3.7444331934681,-1.,-0.203111767587923));
#44619=CARTESIAN_POINT('Ctrl Pts',(-3.7444331934681,1.,-0.203111767587923));
#44620=CARTESIAN_POINT('Ctrl Pts',(-3.7444688019622,-1.,-0.203218215748059));
#44621=CARTESIAN_POINT('Ctrl Pts',(-3.7444688019622,1.,-0.203218215748059));
#44622=CARTESIAN_POINT('Ctrl Pts',(-3.74502080927395,-1.,-0.203352057956297));
#44623=CARTESIAN_POINT('Ctrl Pts',(-3.74502080927395,1.,-0.203352057956297));
#44624=CARTESIAN_POINT('Ctrl Pts',(-3.7467547201908,-1.,-0.203478844530447));
#44625=CARTESIAN_POINT('Ctrl Pts',(-3.7467547201908,1.,-0.203478844530447));
#44626=CARTESIAN_POINT('Ctrl Pts',(-3.75054693397875,-1.,-0.203550035479166));
#44627=CARTESIAN_POINT('Ctrl Pts',(-3.75054693397875,1.,-0.203550035479166));
#44628=CARTESIAN_POINT('Ctrl Pts',(-3.75585118707734,-1.,-0.203530796848322));
#44629=CARTESIAN_POINT('Ctrl Pts',(-3.75585118707734,1.,-0.203530796848322));
#44630=CARTESIAN_POINT('Ctrl Pts',(-3.76242717936885,-1.,-0.203414634707478));
#44631=CARTESIAN_POINT('Ctrl Pts',(-3.76242717936885,1.,-0.203414634707478));
#44632=CARTESIAN_POINT('Ctrl Pts',(-3.7699207159487,-1.,-0.203192390045164));
#44633=CARTESIAN_POINT('Ctrl Pts',(-3.7699207159487,1.,-0.203192390045164));
#44634=CARTESIAN_POINT('Ctrl Pts',(-3.77793553476614,-1.,-0.202854729699081));
#44635=CARTESIAN_POINT('Ctrl Pts',(-3.77793553476614,1.,-0.202854729699081));
#44636=CARTESIAN_POINT('Ctrl Pts',(-3.78609175019242,-1.,-0.20239426051216));
#44637=CARTESIAN_POINT('Ctrl Pts',(-3.78609175019242,1.,-0.20239426051216));
#44638=CARTESIAN_POINT('Ctrl Pts',(-3.7940835418736,-1.,-0.201807533800837));
#44639=CARTESIAN_POINT('Ctrl Pts',(-3.7940835418736,1.,-0.201807533800837));
#44640=CARTESIAN_POINT('Ctrl Pts',(-3.80175247447337,-1.,-0.201097756307326));
#44641=CARTESIAN_POINT('Ctrl Pts',(-3.80175247447337,1.,-0.201097756307326));
#44642=CARTESIAN_POINT('Ctrl Pts',(-3.80909529318669,-1.,-0.200274679433364));
#44643=CARTESIAN_POINT('Ctrl Pts',(-3.80909529318669,1.,-0.200274679433364));
#44644=CARTESIAN_POINT('Ctrl Pts',(-3.81620203429815,-1.,-0.199351525297447));
#44645=CARTESIAN_POINT('Ctrl Pts',(-3.81620203429815,1.,-0.199351525297447));
#44646=CARTESIAN_POINT('Ctrl Pts',(-3.82321127349016,-1.,-0.198342616900486));
#44647=CARTESIAN_POINT('Ctrl Pts',(-3.82321127349016,1.,-0.198342616900486));
#44648=CARTESIAN_POINT('Ctrl Pts',(-3.83026221776456,-1.,-0.197260935827361));
#44649=CARTESIAN_POINT('Ctrl Pts',(-3.83026221776456,1.,-0.197260935827361));
#44650=CARTESIAN_POINT('Ctrl Pts',(-3.83743910616195,-1.,-0.196115198971859));
#44651=CARTESIAN_POINT('Ctrl Pts',(-3.83743910616195,1.,-0.196115198971859));
#44652=CARTESIAN_POINT('Ctrl Pts',(-3.84475203346977,-1.,-0.194909009460221));
#44653=CARTESIAN_POINT('Ctrl Pts',(-3.84475203346977,1.,-0.194909009460221));
#44654=CARTESIAN_POINT('Ctrl Pts',(-3.85216762263966,-1.,-0.193642806777723));
#44655=CARTESIAN_POINT('Ctrl Pts',(-3.85216762263966,1.,-0.193642806777723));
#44656=CARTESIAN_POINT('Ctrl Pts',(-3.85962774407633,-1.,-0.192315153044971));
#44657=CARTESIAN_POINT('Ctrl Pts',(-3.85962774407633,1.,-0.192315153044971));
#44658=CARTESIAN_POINT('Ctrl Pts',(-3.86707158624783,-1.,-0.19092419041862));
#44659=CARTESIAN_POINT('Ctrl Pts',(-3.86707158624783,1.,-0.19092419041862));
#44660=CARTESIAN_POINT('Ctrl Pts',(-3.87445976418412,-1.,-0.189469253358272));
#44661=CARTESIAN_POINT('Ctrl Pts',(-3.87445976418412,1.,-0.189469253358272));
#44662=CARTESIAN_POINT('Ctrl Pts',(-3.88178563496228,-1.,-0.187951632512685));
#44663=CARTESIAN_POINT('Ctrl Pts',(-3.88178563496228,1.,-0.187951632512685));
#44664=CARTESIAN_POINT('Ctrl Pts',(-3.88906196725848,-1.,-0.18637372498528));
#44665=CARTESIAN_POINT('Ctrl Pts',(-3.88906196725848,1.,-0.18637372498528));
#44666=CARTESIAN_POINT('Ctrl Pts',(-3.89631300742646,-1.,-0.184738537728043));
#44667=CARTESIAN_POINT('Ctrl Pts',(-3.89631300742646,1.,-0.184738537728043));
#44668=CARTESIAN_POINT('Ctrl Pts',(-3.90356488555132,-1.,-0.183049081993191));
#44669=CARTESIAN_POINT('Ctrl Pts',(-3.90356488555132,1.,-0.183049081993191));
#44670=CARTESIAN_POINT('Ctrl Pts',(-3.91083557557175,-1.,-0.181307740731786));
#44671=CARTESIAN_POINT('Ctrl Pts',(-3.91083557557175,1.,-0.181307740731786));
#44672=CARTESIAN_POINT('Ctrl Pts',(-3.91812876180926,-1.,-0.179515885822882));
#44673=CARTESIAN_POINT('Ctrl Pts',(-3.91812876180926,1.,-0.179515885822882));
#44674=CARTESIAN_POINT('Ctrl Pts',(-3.92543942697655,-1.,-0.177674246152317));
#44675=CARTESIAN_POINT('Ctrl Pts',(-3.92543942697655,1.,-0.177674246152317));
#44676=CARTESIAN_POINT('Ctrl Pts',(-3.93275726771042,-1.,-0.175783136893868));
#44677=CARTESIAN_POINT('Ctrl Pts',(-3.93275726771042,1.,-0.175783136893868));
#44678=CARTESIAN_POINT('Ctrl Pts',(-3.94007083096217,-1.,-0.17384273497461));
#44679=CARTESIAN_POINT('Ctrl Pts',(-3.94007083096217,1.,-0.17384273497461));
#44680=CARTESIAN_POINT('Ctrl Pts',(-3.94737164900868,-1.,-0.17185335536924));
#44681=CARTESIAN_POINT('Ctrl Pts',(-3.94737164900868,1.,-0.17185335536924));
#44682=CARTESIAN_POINT('Ctrl Pts',(-3.95465744665268,-1.,-0.169815666374139));
#44683=CARTESIAN_POINT('Ctrl Pts',(-3.95465744665268,1.,-0.169815666374139));
#44684=CARTESIAN_POINT('Ctrl Pts',(-3.96192990160296,-1.,-0.167730547023319));
#44685=CARTESIAN_POINT('Ctrl Pts',(-3.96192990160296,1.,-0.167730547023319));
#44686=CARTESIAN_POINT('Ctrl Pts',(-3.96919313621407,-1.,-0.165598992851102));
#44687=CARTESIAN_POINT('Ctrl Pts',(-3.96919313621407,1.,-0.165598992851102));
#44688=CARTESIAN_POINT('Ctrl Pts',(-3.97645194630943,-1.,-0.163422004609999));
#44689=CARTESIAN_POINT('Ctrl Pts',(-3.97645194630943,1.,-0.163422004609999));
#44690=CARTESIAN_POINT('Ctrl Pts',(-3.98371010319872,-1.,-0.161200482186085));
#44691=CARTESIAN_POINT('Ctrl Pts',(-3.98371010319872,1.,-0.161200482186085));
#44692=CARTESIAN_POINT('Ctrl Pts',(-3.99096873945878,-1.,-0.158935123982793));
#44693=CARTESIAN_POINT('Ctrl Pts',(-3.99096873945878,1.,-0.158935123982793));
#44694=CARTESIAN_POINT('Ctrl Pts',(-3.99822717425893,-1.,-0.156626481393734));
#44695=CARTESIAN_POINT('Ctrl Pts',(-3.99822717425893,1.,-0.156626481393734));
#44696=CARTESIAN_POINT('Ctrl Pts',(-4.00548360245319,-1.,-0.154275004872311));
#44697=CARTESIAN_POINT('Ctrl Pts',(-4.00548360245319,1.,-0.154275004872311));
#44698=CARTESIAN_POINT('Ctrl Pts',(-4.01273584234689,-1.,-0.151881094022911));
#44699=CARTESIAN_POINT('Ctrl Pts',(-4.01273584234689,1.,-0.151881094022911));
#44700=CARTESIAN_POINT('Ctrl Pts',(-4.01998203715564,-1.,-0.149445144968707));
#44701=CARTESIAN_POINT('Ctrl Pts',(-4.01998203715564,1.,-0.149445144968707));
#44702=CARTESIAN_POINT('Ctrl Pts',(-4.02722143146994,-1.,-0.146967602878994));
#44703=CARTESIAN_POINT('Ctrl Pts',(-4.02722143146994,1.,-0.146967602878994));
#44704=CARTESIAN_POINT('Ctrl Pts',(-4.03445411510333,-1.,-0.144448947038345));
#44705=CARTESIAN_POINT('Ctrl Pts',(-4.03445411510333,1.,-0.144448947038345));
#44706=CARTESIAN_POINT('Ctrl Pts',(-4.04168069633781,-1.,-0.1418896714855));
#44707=CARTESIAN_POINT('Ctrl Pts',(-4.04168069633781,1.,-0.1418896714855));
#44708=CARTESIAN_POINT('Ctrl Pts',(-4.04890199238036,-1.,-0.139290267180057));
#44709=CARTESIAN_POINT('Ctrl Pts',(-4.04890199238036,1.,-0.139290267180057));
#44710=CARTESIAN_POINT('Ctrl Pts',(-4.05611873400172,-1.,-0.136651205046119));
#44711=CARTESIAN_POINT('Ctrl Pts',(-4.05611873400172,1.,-0.136651205046119));
#44712=CARTESIAN_POINT('Ctrl Pts',(-4.06333121018596,-1.,-0.133972916144245));
#44713=CARTESIAN_POINT('Ctrl Pts',(-4.06333121018596,1.,-0.133972916144245));
#44714=CARTESIAN_POINT('Ctrl Pts',(-4.0705393152874,-1.,-0.13125579354894));
#44715=CARTESIAN_POINT('Ctrl Pts',(-4.0705393152874,1.,-0.13125579354894));
#44716=CARTESIAN_POINT('Ctrl Pts',(-4.07774270738954,-1.,-0.128500200484838));
#44717=CARTESIAN_POINT('Ctrl Pts',(-4.07774270738954,1.,-0.128500200484838));
#44718=CARTESIAN_POINT('Ctrl Pts',(-4.08494093372377,-1.,-0.12570647682254));
#44719=CARTESIAN_POINT('Ctrl Pts',(-4.08494093372377,1.,-0.12570647682254));
#44720=CARTESIAN_POINT('Ctrl Pts',(-4.09213355850756,-1.,-0.122874946249107));
#44721=CARTESIAN_POINT('Ctrl Pts',(-4.09213355850756,1.,-0.122874946249107));
#44722=CARTESIAN_POINT('Ctrl Pts',(-4.09932031767002,-1.,-0.120005924388124));
#44723=CARTESIAN_POINT('Ctrl Pts',(-4.09932031767002,1.,-0.120005924388124));
#44724=CARTESIAN_POINT('Ctrl Pts',(-4.10650113381833,-1.,-0.117099722731648));
#44725=CARTESIAN_POINT('Ctrl Pts',(-4.10650113381833,1.,-0.117099722731648));
#44726=CARTESIAN_POINT('Ctrl Pts',(-4.11367603924961,-1.,-0.114156649609546));
#44727=CARTESIAN_POINT('Ctrl Pts',(-4.11367603924961,1.,-0.114156649609546));
#44728=CARTESIAN_POINT('Ctrl Pts',(-4.1208451250225,-1.,-0.111177012683347));
#44729=CARTESIAN_POINT('Ctrl Pts',(-4.1208451250225,1.,-0.111177012683347));
#44730=CARTESIAN_POINT('Ctrl Pts',(-4.12800848371504,-1.,-0.108161120528369));
#44731=CARTESIAN_POINT('Ctrl Pts',(-4.12800848371504,1.,-0.108161120528369));
#44732=CARTESIAN_POINT('Ctrl Pts',(-4.13516614458895,-1.,-0.105109286538945));
#44733=CARTESIAN_POINT('Ctrl Pts',(-4.13516614458895,1.,-0.105109286538945));
#44734=CARTESIAN_POINT('Ctrl Pts',(-4.14231804939538,-1.,-0.102021826577584));
#44735=CARTESIAN_POINT('Ctrl Pts',(-4.14231804939538,1.,-0.102021826577584));
#44736=CARTESIAN_POINT('Ctrl Pts',(-4.14946408918485,-1.,-0.0988990478901226));
#44737=CARTESIAN_POINT('Ctrl Pts',(-4.14946408918485,1.,-0.0988990478901226));
#44738=CARTESIAN_POINT('Ctrl Pts',(-4.15660412653577,-1.,-0.0957412403298007));
#44739=CARTESIAN_POINT('Ctrl Pts',(-4.15660412653577,1.,-0.0957412403298007));
#44740=CARTESIAN_POINT('Ctrl Pts',(-4.16373802265839,-1.,-0.0925486672167531));
#44741=CARTESIAN_POINT('Ctrl Pts',(-4.16373802265839,1.,-0.0925486672167531));
#44742=CARTESIAN_POINT('Ctrl Pts',(-4.17086566490794,-1.,-0.0893215560848649));
#44743=CARTESIAN_POINT('Ctrl Pts',(-4.17086566490794,1.,-0.0893215560848649));
#44744=CARTESIAN_POINT('Ctrl Pts',(-4.17798698668094,-1.,-0.0860600915549397));
#44745=CARTESIAN_POINT('Ctrl Pts',(-4.17798698668094,1.,-0.0860600915549397));
#44746=CARTESIAN_POINT('Ctrl Pts',(-4.18510195327123,-1.,-0.0827644164385679));
#44747=CARTESIAN_POINT('Ctrl Pts',(-4.18510195327123,1.,-0.0827644164385679));
#44748=CARTESIAN_POINT('Ctrl Pts',(-4.19078883320504,-1.,-0.080100588711432));
#44749=CARTESIAN_POINT('Ctrl Pts',(-4.19078883320504,1.,-0.080100588711432));
#44750=CARTESIAN_POINT('Ctrl Pts',(-4.19505112859416,-1.,-0.0780873956242397));
#44751=CARTESIAN_POINT('Ctrl Pts',(-4.19505112859416,1.,-0.0780873956242397));
#44752=CARTESIAN_POINT('Ctrl Pts',(-4.1978913862118,-1.,-0.0767384596141464));
#44753=CARTESIAN_POINT('Ctrl Pts',(-4.1978913862118,1.,-0.0767384596141464));
#44754=CARTESIAN_POINT('Ctrl Pts',(-4.19931119685982,-1.,-0.0760622897878246));
#44755=CARTESIAN_POINT('Ctrl Pts',(-4.19931119685982,1.,-0.0760622897878246));
#44756=CARTESIAN_POINT('',(-3.74449296983004,1.,-0.2031560948961));
#44757=CARTESIAN_POINT('Ctrl Pts',(-3.74449296983004,-1.,-0.203156094896101));
#44758=CARTESIAN_POINT('Ctrl Pts',(-3.74449296983004,-0.666666666666667,
-0.203156094896101));
#44759=CARTESIAN_POINT('Ctrl Pts',(-3.74449296983004,-0.333333333333333,
-0.203156094896101));
#44760=CARTESIAN_POINT('Ctrl Pts',(-3.74449296983004,0.333333333333333,
-0.203156094896101));
#44761=CARTESIAN_POINT('Ctrl Pts',(-3.74449296983004,0.666666666666667,
-0.203156094896101));
#44762=CARTESIAN_POINT('Ctrl Pts',(-3.74449296983004,1.,-0.203156094896101));
#44763=CARTESIAN_POINT('',(-4.19931119685982,1.,-0.0760622897878246));
#44764=CARTESIAN_POINT('',(-4.19931119685982,0.,-0.0760622897878246));
#44765=CARTESIAN_POINT('Ctrl Pts',(-3.74449296983004,1.,-0.203156094896101));
#44766=CARTESIAN_POINT('Ctrl Pts',(-3.74453008995092,1.,-0.203188003946657));
#44767=CARTESIAN_POINT('Ctrl Pts',(-3.74471097893844,1.,-0.203266610110531));
#44768=CARTESIAN_POINT('Ctrl Pts',(-3.74535749969115,1.,-0.203375226874121));
#44769=CARTESIAN_POINT('Ctrl Pts',(-3.74703926501752,1.,-0.203484186269415));
#44770=CARTESIAN_POINT('Ctrl Pts',(-3.75054693397875,1.,-0.203550035479166));
#44771=CARTESIAN_POINT('Ctrl Pts',(-3.75585118707734,1.,-0.203530796848322));
#44772=CARTESIAN_POINT('Ctrl Pts',(-3.76242717936885,1.,-0.203414634707478));
#44773=CARTESIAN_POINT('Ctrl Pts',(-3.7699207159487,1.,-0.203192390045164));
#44774=CARTESIAN_POINT('Ctrl Pts',(-3.77793553476614,1.,-0.202854729699081));
#44775=CARTESIAN_POINT('Ctrl Pts',(-3.78609175019242,1.,-0.20239426051216));
#44776=CARTESIAN_POINT('Ctrl Pts',(-3.7940835418736,1.,-0.201807533800837));
#44777=CARTESIAN_POINT('Ctrl Pts',(-3.80175247447337,1.,-0.201097756307326));
#44778=CARTESIAN_POINT('Ctrl Pts',(-3.80909529318669,1.,-0.200274679433364));
#44779=CARTESIAN_POINT('Ctrl Pts',(-3.81620203429815,1.,-0.199351525297447));
#44780=CARTESIAN_POINT('Ctrl Pts',(-3.82321127349016,1.,-0.198342616900486));
#44781=CARTESIAN_POINT('Ctrl Pts',(-3.83026221776456,1.,-0.197260935827361));
#44782=CARTESIAN_POINT('Ctrl Pts',(-3.83743910616195,1.,-0.196115198971859));
#44783=CARTESIAN_POINT('Ctrl Pts',(-3.84475203346977,1.,-0.194909009460221));
#44784=CARTESIAN_POINT('Ctrl Pts',(-3.85216762263966,1.,-0.193642806777723));
#44785=CARTESIAN_POINT('Ctrl Pts',(-3.85962774407633,1.,-0.192315153044971));
#44786=CARTESIAN_POINT('Ctrl Pts',(-3.86707158624783,1.,-0.19092419041862));
#44787=CARTESIAN_POINT('Ctrl Pts',(-3.87445976418412,1.,-0.189469253358272));
#44788=CARTESIAN_POINT('Ctrl Pts',(-3.88178563496228,1.,-0.187951632512685));
#44789=CARTESIAN_POINT('Ctrl Pts',(-3.88906196725848,1.,-0.18637372498528));
#44790=CARTESIAN_POINT('Ctrl Pts',(-3.89631300742646,1.,-0.184738537728043));
#44791=CARTESIAN_POINT('Ctrl Pts',(-3.90356488555132,1.,-0.183049081993191));
#44792=CARTESIAN_POINT('Ctrl Pts',(-3.91083557557175,1.,-0.181307740731786));
#44793=CARTESIAN_POINT('Ctrl Pts',(-3.91812876180926,1.,-0.179515885822882));
#44794=CARTESIAN_POINT('Ctrl Pts',(-3.92543942697655,1.,-0.177674246152317));
#44795=CARTESIAN_POINT('Ctrl Pts',(-3.93275726771042,1.,-0.175783136893868));
#44796=CARTESIAN_POINT('Ctrl Pts',(-3.94007083096217,1.,-0.17384273497461));
#44797=CARTESIAN_POINT('Ctrl Pts',(-3.94737164900868,1.,-0.17185335536924));
#44798=CARTESIAN_POINT('Ctrl Pts',(-3.95465744665268,1.,-0.169815666374139));
#44799=CARTESIAN_POINT('Ctrl Pts',(-3.96192990160296,1.,-0.167730547023319));
#44800=CARTESIAN_POINT('Ctrl Pts',(-3.96919313621407,1.,-0.165598992851102));
#44801=CARTESIAN_POINT('Ctrl Pts',(-3.97645194630943,1.,-0.163422004609999));
#44802=CARTESIAN_POINT('Ctrl Pts',(-3.98371010319872,1.,-0.161200482186085));
#44803=CARTESIAN_POINT('Ctrl Pts',(-3.99096873945878,1.,-0.158935123982793));
#44804=CARTESIAN_POINT('Ctrl Pts',(-3.99822717425893,1.,-0.156626481393734));
#44805=CARTESIAN_POINT('Ctrl Pts',(-4.00548360245319,1.,-0.154275004872311));
#44806=CARTESIAN_POINT('Ctrl Pts',(-4.01273584234689,1.,-0.151881094022911));
#44807=CARTESIAN_POINT('Ctrl Pts',(-4.01998203715564,1.,-0.149445144968707));
#44808=CARTESIAN_POINT('Ctrl Pts',(-4.02722143146994,1.,-0.146967602878994));
#44809=CARTESIAN_POINT('Ctrl Pts',(-4.03445411510333,1.,-0.144448947038345));
#44810=CARTESIAN_POINT('Ctrl Pts',(-4.04168069633781,1.,-0.1418896714855));
#44811=CARTESIAN_POINT('Ctrl Pts',(-4.04890199238036,1.,-0.139290267180057));
#44812=CARTESIAN_POINT('Ctrl Pts',(-4.05611873400172,1.,-0.136651205046119));
#44813=CARTESIAN_POINT('Ctrl Pts',(-4.06333121018596,1.,-0.133972916144245));
#44814=CARTESIAN_POINT('Ctrl Pts',(-4.0705393152874,1.,-0.13125579354894));
#44815=CARTESIAN_POINT('Ctrl Pts',(-4.07774270738954,1.,-0.128500200484838));
#44816=CARTESIAN_POINT('Ctrl Pts',(-4.08494093372377,1.,-0.12570647682254));
#44817=CARTESIAN_POINT('Ctrl Pts',(-4.09213355850756,1.,-0.122874946249107));
#44818=CARTESIAN_POINT('Ctrl Pts',(-4.09932031767002,1.,-0.120005924388124));
#44819=CARTESIAN_POINT('Ctrl Pts',(-4.10650113381833,1.,-0.117099722731648));
#44820=CARTESIAN_POINT('Ctrl Pts',(-4.11367603924961,1.,-0.114156649609546));
#44821=CARTESIAN_POINT('Ctrl Pts',(-4.1208451250225,1.,-0.111177012683347));
#44822=CARTESIAN_POINT('Ctrl Pts',(-4.12800848371504,1.,-0.108161120528369));
#44823=CARTESIAN_POINT('Ctrl Pts',(-4.13516614458895,1.,-0.105109286538945));
#44824=CARTESIAN_POINT('Ctrl Pts',(-4.14231804939538,1.,-0.102021826577584));
#44825=CARTESIAN_POINT('Ctrl Pts',(-4.14946408918485,1.,-0.0988990478901226));
#44826=CARTESIAN_POINT('Ctrl Pts',(-4.15660412653577,1.,-0.0957412403298007));
#44827=CARTESIAN_POINT('Ctrl Pts',(-4.16373802265839,1.,-0.0925486672167531));
#44828=CARTESIAN_POINT('Ctrl Pts',(-4.17086566490794,1.,-0.0893215560848649));
#44829=CARTESIAN_POINT('Ctrl Pts',(-4.17798698668094,1.,-0.0860600915549397));
#44830=CARTESIAN_POINT('Ctrl Pts',(-4.18510195327123,1.,-0.0827644164385679));
#44831=CARTESIAN_POINT('Ctrl Pts',(-4.19078883320504,1.,-0.080100588711432));
#44832=CARTESIAN_POINT('Ctrl Pts',(-4.19505112859416,1.,-0.0780873956242397));
#44833=CARTESIAN_POINT('Ctrl Pts',(-4.1978913862118,1.,-0.0767384596141464));
#44834=CARTESIAN_POINT('Ctrl Pts',(-4.19931119685982,1.,-0.0760622897878246));
#44835=CARTESIAN_POINT('Origin',(-4.19931119685982,0.,-0.0760622897878246));
#44836=CARTESIAN_POINT('',(-4.19931119685982,1.,0.0760622897878236));
#44837=CARTESIAN_POINT('Origin',(0.,0.,0.));
#44838=CARTESIAN_POINT('',(-3.73017266276651,1.,-0.385112848330761));
#44839=CARTESIAN_POINT('Origin',(0.,1.,0.));
#44840=CARTESIAN_POINT('Ctrl Pts',(-3.73017266276651,1.,-0.385112848330762));
#44841=CARTESIAN_POINT('Ctrl Pts',(-3.73017266276651,0.666666666666667,
-0.385112848330762));
#44842=CARTESIAN_POINT('Ctrl Pts',(-3.73017266276651,0.333333333333333,
-0.385112848330762));
#44843=CARTESIAN_POINT('Ctrl Pts',(-3.73017266276651,-0.333333333333333,
-0.385112848330762));
#44844=CARTESIAN_POINT('Ctrl Pts',(-3.73017266276651,-0.666666666666667,
-0.385112848330762));
#44845=CARTESIAN_POINT('Ctrl Pts',(-3.73017266276651,-1.,-0.385112848330762));
#44846=CARTESIAN_POINT('Ctrl Pts',(-4.15950947128175,-1.,-0.581791163835815));
#44847=CARTESIAN_POINT('Ctrl Pts',(-4.15950947128175,1.,-0.581791163835815));
#44848=CARTESIAN_POINT('Ctrl Pts',(-4.1582129171283,-1.,-0.580901211463535));
#44849=CARTESIAN_POINT('Ctrl Pts',(-4.1582129171283,1.,-0.580901211463535));
#44850=CARTESIAN_POINT('Ctrl Pts',(-4.15561864788576,-1.,-0.579124568914235));
#44851=CARTESIAN_POINT('Ctrl Pts',(-4.15561864788576,1.,-0.579124568914235));
#44852=CARTESIAN_POINT('Ctrl Pts',(-4.151723761217,-1.,-0.576469391676688));
#44853=CARTESIAN_POINT('Ctrl Pts',(-4.151723761217,1.,-0.576469391676688));
#44854=CARTESIAN_POINT('Ctrl Pts',(-4.14652361068081,-1.,-0.572948736069522));
#44855=CARTESIAN_POINT('Ctrl Pts',(-4.14652361068081,1.,-0.572948736069522));
#44856=CARTESIAN_POINT('Ctrl Pts',(-4.14001179830547,-1.,-0.568580610189774));
#44857=CARTESIAN_POINT('Ctrl Pts',(-4.14001179830547,1.,-0.568580610189774));
#44858=CARTESIAN_POINT('Ctrl Pts',(-4.13348835727104,-1.,-0.564245279537148));
#44859=CARTESIAN_POINT('Ctrl Pts',(-4.13348835727104,1.,-0.564245279537148));
#44860=CARTESIAN_POINT('Ctrl Pts',(-4.12695329951961,-1.,-0.559942890594773));
#44861=CARTESIAN_POINT('Ctrl Pts',(-4.12695329951961,1.,-0.559942890594773));
#44862=CARTESIAN_POINT('Ctrl Pts',(-4.12040666195664,-1.,-0.555673636129977));
#44863=CARTESIAN_POINT('Ctrl Pts',(-4.12040666195664,1.,-0.555673636129977));
#44864=CARTESIAN_POINT('Ctrl Pts',(-4.11384852024721,-1.,-0.551437758497032));
#44865=CARTESIAN_POINT('Ctrl Pts',(-4.11384852024721,1.,-0.551437758497032));
#44866=CARTESIAN_POINT('Ctrl Pts',(-4.10727897027977,-1.,-0.547235539485637));
#44867=CARTESIAN_POINT('Ctrl Pts',(-4.10727897027977,1.,-0.547235539485637));
#44868=CARTESIAN_POINT('Ctrl Pts',(-4.10069810243979,-1.,-0.543067286877757));
#44869=CARTESIAN_POINT('Ctrl Pts',(-4.10069810243979,1.,-0.543067286877757));
#44870=CARTESIAN_POINT('Ctrl Pts',(-4.09410597627,-1.,-0.538933321179756));
#44871=CARTESIAN_POINT('Ctrl Pts',(-4.09410597627,1.,-0.538933321179756));
#44872=CARTESIAN_POINT('Ctrl Pts',(-4.08750259988885,-1.,-0.534833963477273));
#44873=CARTESIAN_POINT('Ctrl Pts',(-4.08750259988885,1.,-0.534833963477273));
#44874=CARTESIAN_POINT('Ctrl Pts',(-4.08088789536836,-1.,-0.530769518728571));
#44875=CARTESIAN_POINT('Ctrl Pts',(-4.08088789536836,1.,-0.530769518728571));
#44876=CARTESIAN_POINT('Ctrl Pts',(-4.07426172299847,-1.,-0.526740277227498));
#44877=CARTESIAN_POINT('Ctrl Pts',(-4.07426172299847,1.,-0.526740277227498));
#44878=CARTESIAN_POINT('Ctrl Pts',(-4.06762394471314,-1.,-0.522746528603107));
#44879=CARTESIAN_POINT('Ctrl Pts',(-4.06762394471314,1.,-0.522746528603107));
#44880=CARTESIAN_POINT('Ctrl Pts',(-4.06097448038013,-1.,-0.518788572336923));
#44881=CARTESIAN_POINT('Ctrl Pts',(-4.06097448038013,1.,-0.518788572336923));
#44882=CARTESIAN_POINT('Ctrl Pts',(-4.05431335771199,-1.,-0.514866728193017));
#44883=CARTESIAN_POINT('Ctrl Pts',(-4.05431335771199,1.,-0.514866728193017));
#44884=CARTESIAN_POINT('Ctrl Pts',(-4.04764078815447,-1.,-0.51098134921897));
#44885=CARTESIAN_POINT('Ctrl Pts',(-4.04764078815447,1.,-0.51098134921897));
#44886=CARTESIAN_POINT('Ctrl Pts',(-4.04095715148915,-1.,-0.507132823288136));
#44887=CARTESIAN_POINT('Ctrl Pts',(-4.04095715148915,1.,-0.507132823288136));
#44888=CARTESIAN_POINT('Ctrl Pts',(-4.03426284174272,-1.,-0.503321556915346));
#44889=CARTESIAN_POINT('Ctrl Pts',(-4.03426284174272,1.,-0.503321556915346));
#44890=CARTESIAN_POINT('Ctrl Pts',(-4.02755813980101,-1.,-0.499547962340821));
#44891=CARTESIAN_POINT('Ctrl Pts',(-4.02755813980101,1.,-0.499547962340821));
#44892=CARTESIAN_POINT('Ctrl Pts',(-4.02084308851832,-1.,-0.495812444326251));
#44893=CARTESIAN_POINT('Ctrl Pts',(-4.02084308851832,1.,-0.495812444326251));
#44894=CARTESIAN_POINT('Ctrl Pts',(-4.01411733503546,-1.,-0.492115383418018));
#44895=CARTESIAN_POINT('Ctrl Pts',(-4.01411733503546,1.,-0.492115383418018));
#44896=CARTESIAN_POINT('Ctrl Pts',(-4.0073800839099,-1.,-0.488457130424633));
#44897=CARTESIAN_POINT('Ctrl Pts',(-4.0073800839099,1.,-0.488457130424633));
#44898=CARTESIAN_POINT('Ctrl Pts',(-4.00063045119288,-1.,-0.484838042421835));
#44899=CARTESIAN_POINT('Ctrl Pts',(-4.00063045119288,1.,-0.484838042421835));
#44900=CARTESIAN_POINT('Ctrl Pts',(-3.99386775880679,-1.,-0.481258512209675));
#44901=CARTESIAN_POINT('Ctrl Pts',(-3.99386775880679,1.,-0.481258512209675));
#44902=CARTESIAN_POINT('Ctrl Pts',(-3.98709184306738,-1.,-0.477718999122027));
#44903=CARTESIAN_POINT('Ctrl Pts',(-3.98709184306738,1.,-0.477718999122027));
#44904=CARTESIAN_POINT('Ctrl Pts',(-3.98030338044409,-1.,-0.47422006101951));
#44905=CARTESIAN_POINT('Ctrl Pts',(-3.98030338044409,1.,-0.47422006101951));
#44906=CARTESIAN_POINT('Ctrl Pts',(-3.97350414289392,-1.,-0.470762379613439));
#44907=CARTESIAN_POINT('Ctrl Pts',(-3.97350414289392,1.,-0.470762379613439));
#44908=CARTESIAN_POINT('Ctrl Pts',(-3.9666962227393,-1.,-0.467346690880643));
#44909=CARTESIAN_POINT('Ctrl Pts',(-3.9666962227393,1.,-0.467346690880643));
#44910=CARTESIAN_POINT('Ctrl Pts',(-3.95988133243538,-1.,-0.463973722115733));
#44911=CARTESIAN_POINT('Ctrl Pts',(-3.95988133243538,1.,-0.463973722115733));
#44912=CARTESIAN_POINT('Ctrl Pts',(-3.95306005817364,-1.,-0.460644124429121));
#44913=CARTESIAN_POINT('Ctrl Pts',(-3.95306005817364,1.,-0.460644124429121));
#44914=CARTESIAN_POINT('Ctrl Pts',(-3.94623117206678,-1.,-0.457358410451683));
#44915=CARTESIAN_POINT('Ctrl Pts',(-3.94623117206678,1.,-0.457358410451683));
#44916=CARTESIAN_POINT('Ctrl Pts',(-3.93939080846298,-1.,-0.454116879027584));
#44917=CARTESIAN_POINT('Ctrl Pts',(-3.93939080846298,1.,-0.454116879027584));
#44918=CARTESIAN_POINT('Ctrl Pts',(-3.93253407403123,-1.,-0.450919768356348));
#44919=CARTESIAN_POINT('Ctrl Pts',(-3.93253407403123,1.,-0.450919768356348));
#44920=CARTESIAN_POINT('Ctrl Pts',(-3.92565674143416,-1.,-0.447767416837292));
#44921=CARTESIAN_POINT('Ctrl Pts',(-3.92565674143416,1.,-0.447767416837292));
#44922=CARTESIAN_POINT('Ctrl Pts',(-3.91875701610719,-1.,-0.444660430230591));
#44923=CARTESIAN_POINT('Ctrl Pts',(-3.91875701610719,1.,-0.444660430230591));
#44924=CARTESIAN_POINT('Ctrl Pts',(-3.91183704069153,-1.,-0.441599824524054));
#44925=CARTESIAN_POINT('Ctrl Pts',(-3.91183704069153,1.,-0.441599824524054));
#44926=CARTESIAN_POINT('Ctrl Pts',(-3.90490512938563,-1.,-0.438587235458249));
#44927=CARTESIAN_POINT('Ctrl Pts',(-3.90490512938563,1.,-0.438587235458249));
#44928=CARTESIAN_POINT('Ctrl Pts',(-3.89797256655462,-1.,-0.435624629433527));
#44929=CARTESIAN_POINT('Ctrl Pts',(-3.89797256655462,1.,-0.435624629433527));
#44930=CARTESIAN_POINT('Ctrl Pts',(-3.89104947940611,-1.,-0.432713929544458));
#44931=CARTESIAN_POINT('Ctrl Pts',(-3.89104947940611,1.,-0.432713929544458));
#44932=CARTESIAN_POINT('Ctrl Pts',(-3.88414070943341,-1.,-0.429856640579741));
#44933=CARTESIAN_POINT('Ctrl Pts',(-3.88414070943341,1.,-0.429856640579741));
#44934=CARTESIAN_POINT('Ctrl Pts',(-3.87724240306597,-1.,-0.427053541173457));
#44935=CARTESIAN_POINT('Ctrl Pts',(-3.87724240306597,1.,-0.427053541173457));
#44936=CARTESIAN_POINT('Ctrl Pts',(-3.87033643487851,-1.,-0.424304173195111));
#44937=CARTESIAN_POINT('Ctrl Pts',(-3.87033643487851,1.,-0.424304173195111));
#44938=CARTESIAN_POINT('Ctrl Pts',(-3.86339652542709,-1.,-0.421607423177534));
#44939=CARTESIAN_POINT('Ctrl Pts',(-3.86339652542709,1.,-0.421607423177534));
#44940=CARTESIAN_POINT('Ctrl Pts',(-3.85639825647996,-1.,-0.418962468086773));
#44941=CARTESIAN_POINT('Ctrl Pts',(-3.85639825647996,1.,-0.418962468086773));
#44942=CARTESIAN_POINT('Ctrl Pts',(-3.84932864157497,-1.,-0.416369678052907));
#44943=CARTESIAN_POINT('Ctrl Pts',(-3.84932864157497,1.,-0.416369678052907));
#44944=CARTESIAN_POINT('Ctrl Pts',(-3.84219403994762,-1.,-0.413831367016748));
#44945=CARTESIAN_POINT('Ctrl Pts',(-3.84219403994762,1.,-0.413831367016748));
#44946=CARTESIAN_POINT('Ctrl Pts',(-3.83503345578698,-1.,-0.411353038798518));
#44947=CARTESIAN_POINT('Ctrl Pts',(-3.83503345578698,1.,-0.411353038798518));
#44948=CARTESIAN_POINT('Ctrl Pts',(-3.82790724256471,-1.,-0.40894237144746));
#44949=CARTESIAN_POINT('Ctrl Pts',(-3.82790724256471,1.,-0.40894237144746));
#44950=CARTESIAN_POINT('Ctrl Pts',(-3.8208730391381,-1.,-0.406607038258985));
#44951=CARTESIAN_POINT('Ctrl Pts',(-3.8208730391381,1.,-0.406607038258985));
#44952=CARTESIAN_POINT('Ctrl Pts',(-3.81396374287793,-1.,-0.404352694628273));
#44953=CARTESIAN_POINT('Ctrl Pts',(-3.81396374287793,1.,-0.404352694628273));
#44954=CARTESIAN_POINT('Ctrl Pts',(-3.80716881962728,-1.,-0.402181320148436));
#44955=CARTESIAN_POINT('Ctrl Pts',(-3.80716881962728,1.,-0.402181320148436));
#44956=CARTESIAN_POINT('Ctrl Pts',(-3.80040370384546,-1.,-0.4000883465046));
#44957=CARTESIAN_POINT('Ctrl Pts',(-3.80040370384546,1.,-0.4000883465046));
#44958=CARTESIAN_POINT('Ctrl Pts',(-3.7935288716329,-1.,-0.398064818683969));
#44959=CARTESIAN_POINT('Ctrl Pts',(-3.7935288716329,1.,-0.398064818683969));
#44960=CARTESIAN_POINT('Ctrl Pts',(-3.78640521279313,-1.,-0.396103205334841));
#44961=CARTESIAN_POINT('Ctrl Pts',(-3.78640521279313,1.,-0.396103205334841));
#44962=CARTESIAN_POINT('Ctrl Pts',(-3.77894173114283,-1.,-0.394202481011499));
#44963=CARTESIAN_POINT('Ctrl Pts',(-3.77894173114283,1.,-0.394202481011499));
#44964=CARTESIAN_POINT('Ctrl Pts',(-3.77114011595967,-1.,-0.392372786223432));
#44965=CARTESIAN_POINT('Ctrl Pts',(-3.77114011595967,1.,-0.392372786223432));
#44966=CARTESIAN_POINT('Ctrl Pts',(-3.76315635033257,-1.,-0.39064207297956));
#44967=CARTESIAN_POINT('Ctrl Pts',(-3.76315635033257,1.,-0.39064207297956));
#44968=CARTESIAN_POINT('Ctrl Pts',(-3.75529302895152,-1.,-0.389054775898702));
#44969=CARTESIAN_POINT('Ctrl Pts',(-3.75529302895152,1.,-0.389054775898702));
#44970=CARTESIAN_POINT('Ctrl Pts',(-3.74792651696654,-1.,-0.387663020050836));
#44971=CARTESIAN_POINT('Ctrl Pts',(-3.74792651696654,1.,-0.387663020050836));
#44972=CARTESIAN_POINT('Ctrl Pts',(-3.74144965781276,-1.,-0.386519576222251));
#44973=CARTESIAN_POINT('Ctrl Pts',(-3.74144965781276,1.,-0.386519576222251));
#44974=CARTESIAN_POINT('Ctrl Pts',(-3.73621371845318,-1.,-0.385670806454566));
#44975=CARTESIAN_POINT('Ctrl Pts',(-3.73621371845318,1.,-0.385670806454566));
#44976=CARTESIAN_POINT('Ctrl Pts',(-3.73245705638843,-1.,-0.385147887988951));
#44977=CARTESIAN_POINT('Ctrl Pts',(-3.73245705638843,1.,-0.385147887988951));
#44978=CARTESIAN_POINT('Ctrl Pts',(-3.73072465900175,-1.,-0.385001870183213));
#44979=CARTESIAN_POINT('Ctrl Pts',(-3.73072465900175,1.,-0.385001870183213));
#44980=CARTESIAN_POINT('Ctrl Pts',(-3.73015851028356,-1.,-0.385047711603462));
#44981=CARTESIAN_POINT('Ctrl Pts',(-3.73015851028356,1.,-0.385047711603462));
#44982=CARTESIAN_POINT('Ctrl Pts',(-3.73010668803042,-1.,-0.385147278814642));
#44983=CARTESIAN_POINT('Ctrl Pts',(-3.73010668803042,1.,-0.385147278814642));
#44984=CARTESIAN_POINT('Ctrl Pts',(-3.73016218570874,-1.,-0.38521431477633));
#44985=CARTESIAN_POINT('Ctrl Pts',(-3.73016218570874,1.,-0.38521431477633));
#44986=CARTESIAN_POINT('',(-4.15950947128175,1.,-0.581791163835815));
#44987=CARTESIAN_POINT('Ctrl Pts',(-4.15950947128175,1.,-0.581791163835815));
#44988=CARTESIAN_POINT('Ctrl Pts',(-4.1582129171283,1.,-0.580901211463535));
#44989=CARTESIAN_POINT('Ctrl Pts',(-4.15561864788576,1.,-0.579124568914235));
#44990=CARTESIAN_POINT('Ctrl Pts',(-4.151723761217,1.,-0.576469391676688));
#44991=CARTESIAN_POINT('Ctrl Pts',(-4.14652361068081,1.,-0.572948736069522));
#44992=CARTESIAN_POINT('Ctrl Pts',(-4.14001179830547,1.,-0.568580610189774));
#44993=CARTESIAN_POINT('Ctrl Pts',(-4.13348835727104,1.,-0.564245279537148));
#44994=CARTESIAN_POINT('Ctrl Pts',(-4.12695329951961,1.,-0.559942890594773));
#44995=CARTESIAN_POINT('Ctrl Pts',(-4.12040666195664,1.,-0.555673636129977));
#44996=CARTESIAN_POINT('Ctrl Pts',(-4.11384852024721,1.,-0.551437758497032));
#44997=CARTESIAN_POINT('Ctrl Pts',(-4.10727897027977,1.,-0.547235539485637));
#44998=CARTESIAN_POINT('Ctrl Pts',(-4.10069810243979,1.,-0.543067286877757));
#44999=CARTESIAN_POINT('Ctrl Pts',(-4.09410597627,1.,-0.538933321179756));
#45000=CARTESIAN_POINT('Ctrl Pts',(-4.08750259988885,1.,-0.534833963477273));
#45001=CARTESIAN_POINT('Ctrl Pts',(-4.08088789536836,1.,-0.530769518728571));
#45002=CARTESIAN_POINT('Ctrl Pts',(-4.07426172299847,1.,-0.526740277227498));
#45003=CARTESIAN_POINT('Ctrl Pts',(-4.06762394471314,1.,-0.522746528603107));
#45004=CARTESIAN_POINT('Ctrl Pts',(-4.06097448038013,1.,-0.518788572336923));
#45005=CARTESIAN_POINT('Ctrl Pts',(-4.05431335771199,1.,-0.514866728193017));
#45006=CARTESIAN_POINT('Ctrl Pts',(-4.04764078815447,1.,-0.51098134921897));
#45007=CARTESIAN_POINT('Ctrl Pts',(-4.04095715148915,1.,-0.507132823288136));
#45008=CARTESIAN_POINT('Ctrl Pts',(-4.03426284174272,1.,-0.503321556915346));
#45009=CARTESIAN_POINT('Ctrl Pts',(-4.02755813980101,1.,-0.499547962340821));
#45010=CARTESIAN_POINT('Ctrl Pts',(-4.02084308851832,1.,-0.495812444326251));
#45011=CARTESIAN_POINT('Ctrl Pts',(-4.01411733503546,1.,-0.492115383418018));
#45012=CARTESIAN_POINT('Ctrl Pts',(-4.0073800839099,1.,-0.488457130424633));
#45013=CARTESIAN_POINT('Ctrl Pts',(-4.00063045119288,1.,-0.484838042421835));
#45014=CARTESIAN_POINT('Ctrl Pts',(-3.99386775880679,1.,-0.481258512209675));
#45015=CARTESIAN_POINT('Ctrl Pts',(-3.98709184306738,1.,-0.477718999122027));
#45016=CARTESIAN_POINT('Ctrl Pts',(-3.98030338044409,1.,-0.47422006101951));
#45017=CARTESIAN_POINT('Ctrl Pts',(-3.97350414289392,1.,-0.470762379613439));
#45018=CARTESIAN_POINT('Ctrl Pts',(-3.9666962227393,1.,-0.467346690880643));
#45019=CARTESIAN_POINT('Ctrl Pts',(-3.95988133243538,1.,-0.463973722115733));
#45020=CARTESIAN_POINT('Ctrl Pts',(-3.95306005817364,1.,-0.460644124429121));
#45021=CARTESIAN_POINT('Ctrl Pts',(-3.94623117206678,1.,-0.457358410451683));
#45022=CARTESIAN_POINT('Ctrl Pts',(-3.93939080846298,1.,-0.454116879027584));
#45023=CARTESIAN_POINT('Ctrl Pts',(-3.93253407403123,1.,-0.450919768356348));
#45024=CARTESIAN_POINT('Ctrl Pts',(-3.92565674143416,1.,-0.447767416837292));
#45025=CARTESIAN_POINT('Ctrl Pts',(-3.91875701610719,1.,-0.444660430230591));
#45026=CARTESIAN_POINT('Ctrl Pts',(-3.91183704069153,1.,-0.441599824524054));
#45027=CARTESIAN_POINT('Ctrl Pts',(-3.90490512938563,1.,-0.438587235458249));
#45028=CARTESIAN_POINT('Ctrl Pts',(-3.89797256655462,1.,-0.435624629433527));
#45029=CARTESIAN_POINT('Ctrl Pts',(-3.89104947940611,1.,-0.432713929544458));
#45030=CARTESIAN_POINT('Ctrl Pts',(-3.88414070943341,1.,-0.429856640579741));
#45031=CARTESIAN_POINT('Ctrl Pts',(-3.87724240306597,1.,-0.427053541173457));
#45032=CARTESIAN_POINT('Ctrl Pts',(-3.87033643487851,1.,-0.424304173195111));
#45033=CARTESIAN_POINT('Ctrl Pts',(-3.86339652542709,1.,-0.421607423177534));
#45034=CARTESIAN_POINT('Ctrl Pts',(-3.85639825647996,1.,-0.418962468086773));
#45035=CARTESIAN_POINT('Ctrl Pts',(-3.84932864157497,1.,-0.416369678052907));
#45036=CARTESIAN_POINT('Ctrl Pts',(-3.84219403994762,1.,-0.413831367016748));
#45037=CARTESIAN_POINT('Ctrl Pts',(-3.83503345578698,1.,-0.411353038798518));
#45038=CARTESIAN_POINT('Ctrl Pts',(-3.82790724256471,1.,-0.40894237144746));
#45039=CARTESIAN_POINT('Ctrl Pts',(-3.8208730391381,1.,-0.406607038258985));
#45040=CARTESIAN_POINT('Ctrl Pts',(-3.81396374287793,1.,-0.404352694628273));
#45041=CARTESIAN_POINT('Ctrl Pts',(-3.80716881962728,1.,-0.402181320148436));
#45042=CARTESIAN_POINT('Ctrl Pts',(-3.80040370384546,1.,-0.4000883465046));
#45043=CARTESIAN_POINT('Ctrl Pts',(-3.7935288716329,1.,-0.398064818683969));
#45044=CARTESIAN_POINT('Ctrl Pts',(-3.78640521279313,1.,-0.396103205334841));
#45045=CARTESIAN_POINT('Ctrl Pts',(-3.77894173114283,1.,-0.394202481011499));
#45046=CARTESIAN_POINT('Ctrl Pts',(-3.77114011595967,1.,-0.392372786223432));
#45047=CARTESIAN_POINT('Ctrl Pts',(-3.76315635033257,1.,-0.39064207297956));
#45048=CARTESIAN_POINT('Ctrl Pts',(-3.75529302895152,1.,-0.389054775898702));
#45049=CARTESIAN_POINT('Ctrl Pts',(-3.74792651696654,1.,-0.387663020050836));
#45050=CARTESIAN_POINT('Ctrl Pts',(-3.74144965781276,1.,-0.386519576222251));
#45051=CARTESIAN_POINT('Ctrl Pts',(-3.73621371845318,1.,-0.385670806454566));
#45052=CARTESIAN_POINT('Ctrl Pts',(-3.73273893363406,1.,-0.385187124634206));
#45053=CARTESIAN_POINT('Ctrl Pts',(-3.73106082862548,1.,-0.385031656499164));
#45054=CARTESIAN_POINT('Ctrl Pts',(-3.73040527621055,1.,-0.385037797881504));
#45055=CARTESIAN_POINT('Ctrl Pts',(-3.73021431755274,1.,-0.385087139000374));
#45056=CARTESIAN_POINT('Ctrl Pts',(-3.73017266276651,1.,-0.385112848330762));
#45057=CARTESIAN_POINT('',(-4.15950947128175,0.,-0.581791163835815));
#45058=CARTESIAN_POINT('Ctrl Pts',(-3.66663282329846,-1.,-0.7863229229206));
#45059=CARTESIAN_POINT('Ctrl Pts',(-3.66663282329846,1.,-0.7863229229206));
#45060=CARTESIAN_POINT('Ctrl Pts',(-3.66655932661986,-1.,-0.786369528183326));
#45061=CARTESIAN_POINT('Ctrl Pts',(-3.66655932661986,1.,-0.786369528183326));
#45062=CARTESIAN_POINT('Ctrl Pts',(-3.66657784455334,-1.,-0.786480236185696));
#45063=CARTESIAN_POINT('Ctrl Pts',(-3.66657784455334,1.,-0.786480236185696));
#45064=CARTESIAN_POINT('Ctrl Pts',(-3.66710211820482,-1.,-0.786698783542764));
#45065=CARTESIAN_POINT('Ctrl Pts',(-3.66710211820482,1.,-0.786698783542764));
#45066=CARTESIAN_POINT('Ctrl Pts',(-3.66879484801113,-1.,-0.787095252590501));
#45067=CARTESIAN_POINT('Ctrl Pts',(-3.66879484801113,1.,-0.787095252590501));
#45068=CARTESIAN_POINT('Ctrl Pts',(-3.67252923663655,-1.,-0.787758799995742));
#45069=CARTESIAN_POINT('Ctrl Pts',(-3.67252923663655,1.,-0.787758799995742));
#45070=CARTESIAN_POINT('Ctrl Pts',(-3.67777119516252,-1.,-0.788569566220285));
#45071=CARTESIAN_POINT('Ctrl Pts',(-3.67777119516252,1.,-0.788569566220285));
#45072=CARTESIAN_POINT('Ctrl Pts',(-3.68428439783905,-1.,-0.789483546064387));
#45073=CARTESIAN_POINT('Ctrl Pts',(-3.68428439783905,1.,-0.789483546064387));
#45074=CARTESIAN_POINT('Ctrl Pts',(-3.69172044327364,-1.,-0.790436284988787));
#45075=CARTESIAN_POINT('Ctrl Pts',(-3.69172044327364,1.,-0.790436284988787));
#45076=CARTESIAN_POINT('Ctrl Pts',(-3.69968940808721,-1.,-0.79135657569598));
#45077=CARTESIAN_POINT('Ctrl Pts',(-3.69968940808721,1.,-0.79135657569598));
#45078=CARTESIAN_POINT('Ctrl Pts',(-3.70781724021806,-1.,-0.792177688845818));
#45079=CARTESIAN_POINT('Ctrl Pts',(-3.70781724021806,1.,-0.792177688845818));
#45080=CARTESIAN_POINT('Ctrl Pts',(-3.71580242396124,-1.,-0.792848377370287));
#45081=CARTESIAN_POINT('Ctrl Pts',(-3.71580242396124,1.,-0.792848377370287));
#45082=CARTESIAN_POINT('Ctrl Pts',(-3.72348797293734,-1.,-0.793347023784205));
#45083=CARTESIAN_POINT('Ctrl Pts',(-3.72348797293734,1.,-0.793347023784205));
#45084=CARTESIAN_POINT('Ctrl Pts',(-3.73086914695805,-1.,-0.793682750269684));
#45085=CARTESIAN_POINT('Ctrl Pts',(-3.73086914695805,1.,-0.793682750269684));
#45086=CARTESIAN_POINT('Ctrl Pts',(-3.73803280541687,-1.,-0.793882700937017));
#45087=CARTESIAN_POINT('Ctrl Pts',(-3.73803280541687,1.,-0.793882700937017));
#45088=CARTESIAN_POINT('Ctrl Pts',(-3.74511357728861,-1.,-0.793982700459952));
#45089=CARTESIAN_POINT('Ctrl Pts',(-3.74511357728861,1.,-0.793982700459952));
#45090=CARTESIAN_POINT('Ctrl Pts',(-3.75224692493864,-1.,-0.794017347371377));
#45091=CARTESIAN_POINT('Ctrl Pts',(-3.75224692493864,1.,-0.794017347371377));
#45092=CARTESIAN_POINT('Ctrl Pts',(-3.75951468666257,-1.,-0.794008429134907));
#45093=CARTESIAN_POINT('Ctrl Pts',(-3.75951468666257,1.,-0.794008429134907));
#45094=CARTESIAN_POINT('Ctrl Pts',(-3.76692626931111,-1.,-0.793961083688991));
#45095=CARTESIAN_POINT('Ctrl Pts',(-3.76692626931111,1.,-0.793961083688991));
#45096=CARTESIAN_POINT('Ctrl Pts',(-3.77444863801212,-1.,-0.793870523787408));
#45097=CARTESIAN_POINT('Ctrl Pts',(-3.77444863801212,1.,-0.793870523787408));
#45098=CARTESIAN_POINT('Ctrl Pts',(-3.78202460377598,-1.,-0.7937262357813));
#45099=CARTESIAN_POINT('Ctrl Pts',(-3.78202460377598,1.,-0.7937262357813));
#45100=CARTESIAN_POINT('Ctrl Pts',(-3.78959439439235,-1.,-0.793516871680993));
#45101=CARTESIAN_POINT('Ctrl Pts',(-3.78959439439235,1.,-0.793516871680993));
#45102=CARTESIAN_POINT('Ctrl Pts',(-3.79711921389897,-1.,-0.793235612973273));
#45103=CARTESIAN_POINT('Ctrl Pts',(-3.79711921389897,1.,-0.793235612973273));
#45104=CARTESIAN_POINT('Ctrl Pts',(-3.80459229925637,-1.,-0.792882695234778));
#45105=CARTESIAN_POINT('Ctrl Pts',(-3.80459229925637,1.,-0.792882695234778));
#45106=CARTESIAN_POINT('Ctrl Pts',(-3.81202588694756,-1.,-0.792462483517634));
#45107=CARTESIAN_POINT('Ctrl Pts',(-3.81202588694756,1.,-0.792462483517634));
#45108=CARTESIAN_POINT('Ctrl Pts',(-3.81944345442249,-1.,-0.791981740718635));
#45109=CARTESIAN_POINT('Ctrl Pts',(-3.81944345442249,1.,-0.791981740718635));
#45110=CARTESIAN_POINT('Ctrl Pts',(-3.82687033899792,-1.,-0.791447528662369));
#45111=CARTESIAN_POINT('Ctrl Pts',(-3.82687033899792,1.,-0.791447528662369));
#45112=CARTESIAN_POINT('Ctrl Pts',(-3.83432392054786,-1.,-0.790865012705301));
#45113=CARTESIAN_POINT('Ctrl Pts',(-3.83432392054786,1.,-0.790865012705301));
#45114=CARTESIAN_POINT('Ctrl Pts',(-3.84180762342454,-1.,-0.790236124191242));
#45115=CARTESIAN_POINT('Ctrl Pts',(-3.84180762342454,1.,-0.790236124191242));
#45116=CARTESIAN_POINT('Ctrl Pts',(-3.84931637808894,-1.,-0.789560798155582));
#45117=CARTESIAN_POINT('Ctrl Pts',(-3.84931637808894,1.,-0.789560798155582));
#45118=CARTESIAN_POINT('Ctrl Pts',(-3.85683995872529,-1.,-0.788837734090672));
#45119=CARTESIAN_POINT('Ctrl Pts',(-3.85683995872529,1.,-0.788837734090672));
#45120=CARTESIAN_POINT('Ctrl Pts',(-3.86436702561345,-1.,-0.788065315093777));
#45121=CARTESIAN_POINT('Ctrl Pts',(-3.86436702561345,1.,-0.788065315093777));
#45122=CARTESIAN_POINT('Ctrl Pts',(-3.87188916600912,-1.,-0.787242527617999));
#45123=CARTESIAN_POINT('Ctrl Pts',(-3.87188916600912,1.,-0.787242527617999));
#45124=CARTESIAN_POINT('Ctrl Pts',(-3.8794040281819,-1.,-0.786369675812608));
#45125=CARTESIAN_POINT('Ctrl Pts',(-3.8794040281819,1.,-0.786369675812608));
#45126=CARTESIAN_POINT('Ctrl Pts',(-3.88691313167398,-1.,-0.78544789034073));
#45127=CARTESIAN_POINT('Ctrl Pts',(-3.88691313167398,1.,-0.78544789034073));
#45128=CARTESIAN_POINT('Ctrl Pts',(-3.89442039235103,-1.,-0.784478799358336));
#45129=CARTESIAN_POINT('Ctrl Pts',(-3.89442039235103,1.,-0.784478799358336));
#45130=CARTESIAN_POINT('Ctrl Pts',(-3.9019303904397,-1.,-0.783464141529081));
#45131=CARTESIAN_POINT('Ctrl Pts',(-3.9019303904397,1.,-0.783464141529081));
#45132=CARTESIAN_POINT('Ctrl Pts',(-3.90944671004542,-1.,-0.782405395622764));
#45133=CARTESIAN_POINT('Ctrl Pts',(-3.90944671004542,1.,-0.782405395622764));
#45134=CARTESIAN_POINT('Ctrl Pts',(-3.91697036054676,-1.,-0.781303428618366));
#45135=CARTESIAN_POINT('Ctrl Pts',(-3.91697036054676,1.,-0.781303428618366));
#45136=CARTESIAN_POINT('Ctrl Pts',(-3.92450058323823,-1.,-0.780158678615542));
#45137=CARTESIAN_POINT('Ctrl Pts',(-3.92450058323823,1.,-0.780158678615542));
#45138=CARTESIAN_POINT('Ctrl Pts',(-3.93203552473174,-1.,-0.778971308134821));
#45139=CARTESIAN_POINT('Ctrl Pts',(-3.93203552473174,1.,-0.778971308134821));
#45140=CARTESIAN_POINT('Ctrl Pts',(-3.93957296768103,-1.,-0.777741370568558));
#45141=CARTESIAN_POINT('Ctrl Pts',(-3.93957296768103,1.,-0.777741370568558));
#45142=CARTESIAN_POINT('Ctrl Pts',(-3.94711101619447,-1.,-0.776468966697921));
#45143=CARTESIAN_POINT('Ctrl Pts',(-3.94711101619447,1.,-0.776468966697921));
#45144=CARTESIAN_POINT('Ctrl Pts',(-3.9546488545231,-1.,-0.775154418039351));
#45145=CARTESIAN_POINT('Ctrl Pts',(-3.9546488545231,1.,-0.775154418039351));
#45146=CARTESIAN_POINT('Ctrl Pts',(-3.96218649639807,-1.,-0.773798212026565));
#45147=CARTESIAN_POINT('Ctrl Pts',(-3.96218649639807,1.,-0.773798212026565));
#45148=CARTESIAN_POINT('Ctrl Pts',(-3.96972446532772,-1.,-0.772400931772136));
#45149=CARTESIAN_POINT('Ctrl Pts',(-3.96972446532772,1.,-0.772400931772136));
#45150=CARTESIAN_POINT('Ctrl Pts',(-3.97726349165488,-1.,-0.770963190030471));
#45151=CARTESIAN_POINT('Ctrl Pts',(-3.97726349165488,1.,-0.770963190030471));
#45152=CARTESIAN_POINT('Ctrl Pts',(-3.98480422348451,-1.,-0.769485566245544));
#45153=CARTESIAN_POINT('Ctrl Pts',(-3.98480422348451,1.,-0.769485566245544));
#45154=CARTESIAN_POINT('Ctrl Pts',(-3.9923468788101,-1.,-0.767968531377915));
#45155=CARTESIAN_POINT('Ctrl Pts',(-3.9923468788101,1.,-0.767968531377915));
#45156=CARTESIAN_POINT('Ctrl Pts',(-3.99989129179622,-1.,-0.766412457136064));
#45157=CARTESIAN_POINT('Ctrl Pts',(-3.99989129179622,1.,-0.766412457136064));
#45158=CARTESIAN_POINT('Ctrl Pts',(-4.00743706791509,-1.,-0.764817648785197));
#45159=CARTESIAN_POINT('Ctrl Pts',(-4.00743706791509,1.,-0.764817648785197));
#45160=CARTESIAN_POINT('Ctrl Pts',(-4.01498370680496,-1.,-0.763184371182935));
#45161=CARTESIAN_POINT('Ctrl Pts',(-4.01498370680496,1.,-0.763184371182935));
#45162=CARTESIAN_POINT('Ctrl Pts',(-4.02253072741268,-1.,-0.761512875859804));
#45163=CARTESIAN_POINT('Ctrl Pts',(-4.02253072741268,1.,-0.761512875859804));
#45164=CARTESIAN_POINT('Ctrl Pts',(-4.03007781954412,-1.,-0.759803433243752));
#45165=CARTESIAN_POINT('Ctrl Pts',(-4.03007781954412,1.,-0.759803433243752));
#45166=CARTESIAN_POINT('Ctrl Pts',(-4.03762485803119,-1.,-0.758056338884944));
#45167=CARTESIAN_POINT('Ctrl Pts',(-4.03762485803119,1.,-0.758056338884944));
#45168=CARTESIAN_POINT('Ctrl Pts',(-4.04517182653997,-1.,-0.756271902369581));
#45169=CARTESIAN_POINT('Ctrl Pts',(-4.04517182653997,1.,-0.756271902369581));
#45170=CARTESIAN_POINT('Ctrl Pts',(-4.05271876687915,-1.,-0.754450441816078));
#45171=CARTESIAN_POINT('Ctrl Pts',(-4.05271876687915,1.,-0.754450441816078));
#45172=CARTESIAN_POINT('Ctrl Pts',(-4.06026572221515,-1.,-0.752592276483072));
#45173=CARTESIAN_POINT('Ctrl Pts',(-4.06026572221515,1.,-0.752592276483072));
#45174=CARTESIAN_POINT('Ctrl Pts',(-4.06781267242378,-1.,-0.750697720484036));
#45175=CARTESIAN_POINT('Ctrl Pts',(-4.06781267242378,1.,-0.750697720484036));
#45176=CARTESIAN_POINT('Ctrl Pts',(-4.07535951056152,-1.,-0.748767076680557));
#45177=CARTESIAN_POINT('Ctrl Pts',(-4.07535951056152,1.,-0.748767076680557));
#45178=CARTESIAN_POINT('Ctrl Pts',(-4.08290608095642,-1.,-0.746800631492315));
#45179=CARTESIAN_POINT('Ctrl Pts',(-4.08290608095642,1.,-0.746800631492315));
#45180=CARTESIAN_POINT('Ctrl Pts',(-4.09045220253573,-1.,-0.7447986497065));
#45181=CARTESIAN_POINT('Ctrl Pts',(-4.09045220253573,1.,-0.7447986497065));
#45182=CARTESIAN_POINT('Ctrl Pts',(-4.09799769702611,-1.,-0.742761369689841));
#45183=CARTESIAN_POINT('Ctrl Pts',(-4.09799769702611,1.,-0.742761369689841));
#45184=CARTESIAN_POINT('Ctrl Pts',(-4.10554241757547,-1.,-0.740688998553377));
#45185=CARTESIAN_POINT('Ctrl Pts',(-4.10554241757547,1.,-0.740688998553377));
#45186=CARTESIAN_POINT('Ctrl Pts',(-4.11308626951927,-1.,-0.738581708225844));
#45187=CARTESIAN_POINT('Ctrl Pts',(-4.11308626951927,1.,-0.738581708225844));
#45188=CARTESIAN_POINT('Ctrl Pts',(-4.120629196238,-1.,-0.736439634331345));
#45189=CARTESIAN_POINT('Ctrl Pts',(-4.120629196238,1.,-0.736439634331345));
#45190=CARTESIAN_POINT('Ctrl Pts',(-4.12666277570844,-1.,-0.734698226764092));
#45191=CARTESIAN_POINT('Ctrl Pts',(-4.12666277570844,1.,-0.734698226764092));
#45192=CARTESIAN_POINT('Ctrl Pts',(-4.13118752795207,-1.,-0.733376589323546));
#45193=CARTESIAN_POINT('Ctrl Pts',(-4.13118752795207,1.,-0.733376589323546));
#45194=CARTESIAN_POINT('Ctrl Pts',(-4.1342038373684,-1.,-0.732488575135159));
#45195=CARTESIAN_POINT('Ctrl Pts',(-4.1342038373684,1.,-0.732488575135159));
#45196=CARTESIAN_POINT('Ctrl Pts',(-4.13571194405636,-1.,-0.73204283740062));
#45197=CARTESIAN_POINT('Ctrl Pts',(-4.13571194405636,1.,-0.73204283740062));
#45198=CARTESIAN_POINT('',(-3.66661143271685,1.,-0.786422660831985));
#45199=CARTESIAN_POINT('Ctrl Pts',(-3.66661143271685,-1.,-0.786422660831985));
#45200=CARTESIAN_POINT('Ctrl Pts',(-3.66661143271685,-0.666666666666667,
-0.786422660831985));
#45201=CARTESIAN_POINT('Ctrl Pts',(-3.66661143271685,-0.333333333333333,
-0.786422660831985));
#45202=CARTESIAN_POINT('Ctrl Pts',(-3.66661143271685,0.333333333333333,
-0.786422660831985));
#45203=CARTESIAN_POINT('Ctrl Pts',(-3.66661143271685,0.666666666666667,
-0.786422660831985));
#45204=CARTESIAN_POINT('Ctrl Pts',(-3.66661143271685,1.,-0.786422660831985));
#45205=CARTESIAN_POINT('',(-4.13571194405636,1.,-0.73204283740062));
#45206=CARTESIAN_POINT('',(-4.13571194405636,0.,-0.73204283740062));
#45207=CARTESIAN_POINT('Ctrl Pts',(-3.66661143271685,1.,-0.786422660831985));
#45208=CARTESIAN_POINT('Ctrl Pts',(-3.6666431041522,1.,-0.786459983895432));
#45209=CARTESIAN_POINT('Ctrl Pts',(-3.66680946938292,1.,-0.786565919558984));
#45210=CARTESIAN_POINT('Ctrl Pts',(-3.66743103898702,1.,-0.786774337198062));
#45211=CARTESIAN_POINT('Ctrl Pts',(-3.66907505398677,1.,-0.787145041181545));
#45212=CARTESIAN_POINT('Ctrl Pts',(-3.67252923663655,1.,-0.787758799995742));
#45213=CARTESIAN_POINT('Ctrl Pts',(-3.67777119516252,1.,-0.788569566220285));
#45214=CARTESIAN_POINT('Ctrl Pts',(-3.68428439783905,1.,-0.789483546064387));
#45215=CARTESIAN_POINT('Ctrl Pts',(-3.69172044327364,1.,-0.790436284988787));
#45216=CARTESIAN_POINT('Ctrl Pts',(-3.69968940808721,1.,-0.79135657569598));
#45217=CARTESIAN_POINT('Ctrl Pts',(-3.70781724021806,1.,-0.792177688845818));
#45218=CARTESIAN_POINT('Ctrl Pts',(-3.71580242396124,1.,-0.792848377370287));
#45219=CARTESIAN_POINT('Ctrl Pts',(-3.72348797293734,1.,-0.793347023784205));
#45220=CARTESIAN_POINT('Ctrl Pts',(-3.73086914695805,1.,-0.793682750269684));
#45221=CARTESIAN_POINT('Ctrl Pts',(-3.73803280541687,1.,-0.793882700937017));
#45222=CARTESIAN_POINT('Ctrl Pts',(-3.74511357728861,1.,-0.793982700459952));
#45223=CARTESIAN_POINT('Ctrl Pts',(-3.75224692493864,1.,-0.794017347371377));
#45224=CARTESIAN_POINT('Ctrl Pts',(-3.75951468666257,1.,-0.794008429134907));
#45225=CARTESIAN_POINT('Ctrl Pts',(-3.76692626931111,1.,-0.793961083688991));
#45226=CARTESIAN_POINT('Ctrl Pts',(-3.77444863801212,1.,-0.793870523787408));
#45227=CARTESIAN_POINT('Ctrl Pts',(-3.78202460377598,1.,-0.7937262357813));
#45228=CARTESIAN_POINT('Ctrl Pts',(-3.78959439439235,1.,-0.793516871680993));
#45229=CARTESIAN_POINT('Ctrl Pts',(-3.79711921389897,1.,-0.793235612973273));
#45230=CARTESIAN_POINT('Ctrl Pts',(-3.80459229925637,1.,-0.792882695234778));
#45231=CARTESIAN_POINT('Ctrl Pts',(-3.81202588694756,1.,-0.792462483517634));
#45232=CARTESIAN_POINT('Ctrl Pts',(-3.81944345442249,1.,-0.791981740718635));
#45233=CARTESIAN_POINT('Ctrl Pts',(-3.82687033899792,1.,-0.791447528662369));
#45234=CARTESIAN_POINT('Ctrl Pts',(-3.83432392054786,1.,-0.790865012705301));
#45235=CARTESIAN_POINT('Ctrl Pts',(-3.84180762342454,1.,-0.790236124191242));
#45236=CARTESIAN_POINT('Ctrl Pts',(-3.84931637808894,1.,-0.789560798155582));
#45237=CARTESIAN_POINT('Ctrl Pts',(-3.85683995872529,1.,-0.788837734090672));
#45238=CARTESIAN_POINT('Ctrl Pts',(-3.86436702561345,1.,-0.788065315093777));
#45239=CARTESIAN_POINT('Ctrl Pts',(-3.87188916600912,1.,-0.787242527617999));
#45240=CARTESIAN_POINT('Ctrl Pts',(-3.8794040281819,1.,-0.786369675812608));
#45241=CARTESIAN_POINT('Ctrl Pts',(-3.88691313167398,1.,-0.78544789034073));
#45242=CARTESIAN_POINT('Ctrl Pts',(-3.89442039235103,1.,-0.784478799358336));
#45243=CARTESIAN_POINT('Ctrl Pts',(-3.9019303904397,1.,-0.783464141529081));
#45244=CARTESIAN_POINT('Ctrl Pts',(-3.90944671004542,1.,-0.782405395622764));
#45245=CARTESIAN_POINT('Ctrl Pts',(-3.91697036054676,1.,-0.781303428618366));
#45246=CARTESIAN_POINT('Ctrl Pts',(-3.92450058323823,1.,-0.780158678615542));
#45247=CARTESIAN_POINT('Ctrl Pts',(-3.93203552473174,1.,-0.778971308134821));
#45248=CARTESIAN_POINT('Ctrl Pts',(-3.93957296768103,1.,-0.777741370568558));
#45249=CARTESIAN_POINT('Ctrl Pts',(-3.94711101619447,1.,-0.776468966697921));
#45250=CARTESIAN_POINT('Ctrl Pts',(-3.9546488545231,1.,-0.775154418039351));
#45251=CARTESIAN_POINT('Ctrl Pts',(-3.96218649639807,1.,-0.773798212026565));
#45252=CARTESIAN_POINT('Ctrl Pts',(-3.96972446532772,1.,-0.772400931772136));
#45253=CARTESIAN_POINT('Ctrl Pts',(-3.97726349165488,1.,-0.770963190030471));
#45254=CARTESIAN_POINT('Ctrl Pts',(-3.98480422348451,1.,-0.769485566245544));
#45255=CARTESIAN_POINT('Ctrl Pts',(-3.9923468788101,1.,-0.767968531377915));
#45256=CARTESIAN_POINT('Ctrl Pts',(-3.99989129179622,1.,-0.766412457136064));
#45257=CARTESIAN_POINT('Ctrl Pts',(-4.00743706791509,1.,-0.764817648785197));
#45258=CARTESIAN_POINT('Ctrl Pts',(-4.01498370680496,1.,-0.763184371182935));
#45259=CARTESIAN_POINT('Ctrl Pts',(-4.02253072741268,1.,-0.761512875859804));
#45260=CARTESIAN_POINT('Ctrl Pts',(-4.03007781954412,1.,-0.759803433243752));
#45261=CARTESIAN_POINT('Ctrl Pts',(-4.03762485803119,1.,-0.758056338884944));
#45262=CARTESIAN_POINT('Ctrl Pts',(-4.04517182653997,1.,-0.756271902369581));
#45263=CARTESIAN_POINT('Ctrl Pts',(-4.05271876687915,1.,-0.754450441816078));
#45264=CARTESIAN_POINT('Ctrl Pts',(-4.06026572221515,1.,-0.752592276483072));
#45265=CARTESIAN_POINT('Ctrl Pts',(-4.06781267242378,1.,-0.750697720484036));
#45266=CARTESIAN_POINT('Ctrl Pts',(-4.07535951056152,1.,-0.748767076680557));
#45267=CARTESIAN_POINT('Ctrl Pts',(-4.08290608095642,1.,-0.746800631492315));
#45268=CARTESIAN_POINT('Ctrl Pts',(-4.09045220253573,1.,-0.7447986497065));
#45269=CARTESIAN_POINT('Ctrl Pts',(-4.09799769702611,1.,-0.742761369689841));
#45270=CARTESIAN_POINT('Ctrl Pts',(-4.10554241757547,1.,-0.740688998553377));
#45271=CARTESIAN_POINT('Ctrl Pts',(-4.11308626951927,1.,-0.738581708225844));
#45272=CARTESIAN_POINT('Ctrl Pts',(-4.120629196238,1.,-0.736439634331345));
#45273=CARTESIAN_POINT('Ctrl Pts',(-4.12666277570844,1.,-0.734698226764092));
#45274=CARTESIAN_POINT('Ctrl Pts',(-4.13118752795207,1.,-0.733376589323546));
#45275=CARTESIAN_POINT('Ctrl Pts',(-4.1342038373684,1.,-0.732488575135159));
#45276=CARTESIAN_POINT('Ctrl Pts',(-4.13571194405636,1.,-0.73204283740062));
#45277=CARTESIAN_POINT('Origin',(-4.13571194405636,0.,-0.73204283740062));
#45278=CARTESIAN_POINT('',(-4.15950947128175,1.,-0.581791163835815));
#45279=CARTESIAN_POINT('Origin',(0.,0.,0.));
#45280=CARTESIAN_POINT('',(-3.62400312501245,1.,-0.963899035117248));
#45281=CARTESIAN_POINT('Origin',(0.,1.,0.));
#45282=CARTESIAN_POINT('Ctrl Pts',(-3.62400312501245,1.,-0.963899035117249));
#45283=CARTESIAN_POINT('Ctrl Pts',(-3.62400312501245,0.666666666666667,
-0.963899035117249));
#45284=CARTESIAN_POINT('Ctrl Pts',(-3.62400312501245,0.333333333333333,
-0.963899035117249));
#45285=CARTESIAN_POINT('Ctrl Pts',(-3.62400312501245,-0.333333333333333,
-0.963899035117249));
#45286=CARTESIAN_POINT('Ctrl Pts',(-3.62400312501246,-0.666666666666667,
-0.963899035117249));
#45287=CARTESIAN_POINT('Ctrl Pts',(-3.62400312501246,-1.,-0.963899035117249));
#45288=CARTESIAN_POINT('Ctrl Pts',(-4.01728681790024,-1.,-1.22531898815164));
#45289=CARTESIAN_POINT('Ctrl Pts',(-4.01728681790024,1.,-1.22531898815164));
#45290=CARTESIAN_POINT('Ctrl Pts',(-4.0161454457032,-1.,-1.22423716681447));
#45291=CARTESIAN_POINT('Ctrl Pts',(-4.0161454457032,1.,-1.22423716681447));
#45292=CARTESIAN_POINT('Ctrl Pts',(-4.01386104434674,-1.,-1.22207656456199));
#45293=CARTESIAN_POINT('Ctrl Pts',(-4.01386104434674,1.,-1.22207656456199));
#45294=CARTESIAN_POINT('Ctrl Pts',(-4.01042947142681,-1.,-1.21884478244983));
#45295=CARTESIAN_POINT('Ctrl Pts',(-4.01042947142681,1.,-1.21884478244983));
#45296=CARTESIAN_POINT('Ctrl Pts',(-4.00584409524937,-1.,-1.21455398918813));
#45297=CARTESIAN_POINT('Ctrl Pts',(-4.00584409524937,1.,-1.21455398918813));
#45298=CARTESIAN_POINT('Ctrl Pts',(-4.00009577952534,-1.,-1.20922097030107));
#45299=CARTESIAN_POINT('Ctrl Pts',(-4.00009577952534,1.,-1.20922097030107));
#45300=CARTESIAN_POINT('Ctrl Pts',(-3.99433084800649,-1.,-1.2039185237544));
#45301=CARTESIAN_POINT('Ctrl Pts',(-3.99433084800649,1.,-1.2039185237544));
#45302=CARTESIAN_POINT('Ctrl Pts',(-3.98854928957287,-1.,-1.19864679609596));
#45303=CARTESIAN_POINT('Ctrl Pts',(-3.98854928957287,1.,-1.19864679609596));
#45304=CARTESIAN_POINT('Ctrl Pts',(-3.98275111052015,-1.,-1.19340598349307));
#45305=CARTESIAN_POINT('Ctrl Pts',(-3.98275111052015,1.,-1.19340598349307));
#45306=CARTESIAN_POINT('Ctrl Pts',(-3.97693634766926,-1.,-1.18819633715285));
#45307=CARTESIAN_POINT('Ctrl Pts',(-3.97693634766926,1.,-1.18819633715285));
#45308=CARTESIAN_POINT('Ctrl Pts',(-3.9711050516465,-1.,-1.18301815039596));
#45309=CARTESIAN_POINT('Ctrl Pts',(-3.9711050516465,1.,-1.18301815039596));
#45310=CARTESIAN_POINT('Ctrl Pts',(-3.96525726357682,-1.,-1.17787174135445));
#45311=CARTESIAN_POINT('Ctrl Pts',(-3.96525726357682,1.,-1.17787174135445));
#45312=CARTESIAN_POINT('Ctrl Pts',(-3.95939299213164,-1.,-1.17275743590327));
#45313=CARTESIAN_POINT('Ctrl Pts',(-3.95939299213164,1.,-1.17275743590327));
#45314=CARTESIAN_POINT('Ctrl Pts',(-3.95351219510062,-1.,-1.16767555244495));
#45315=CARTESIAN_POINT('Ctrl Pts',(-3.95351219510062,1.,-1.16767555244495));
#45316=CARTESIAN_POINT('Ctrl Pts',(-3.9476147478092,-1.,-1.16262637999261));
#45317=CARTESIAN_POINT('Ctrl Pts',(-3.9476147478092,1.,-1.16262637999261));
#45318=CARTESIAN_POINT('Ctrl Pts',(-3.94170046685542,-1.,-1.1576101834106));
#45319=CARTESIAN_POINT('Ctrl Pts',(-3.94170046685542,1.,-1.1576101834106));
#45320=CARTESIAN_POINT('Ctrl Pts',(-3.9357691705651,-1.,-1.1526272271639));
#45321=CARTESIAN_POINT('Ctrl Pts',(-3.9357691705651,1.,-1.1526272271639));
#45322=CARTESIAN_POINT('Ctrl Pts',(-3.92982073294334,-1.,-1.14767779451147));
#45323=CARTESIAN_POINT('Ctrl Pts',(-3.92982073294334,1.,-1.14767779451147));
#45324=CARTESIAN_POINT('Ctrl Pts',(-3.92385513133937,-1.,-1.14276220561575));
#45325=CARTESIAN_POINT('Ctrl Pts',(-3.92385513133937,1.,-1.14276220561575));
#45326=CARTESIAN_POINT('Ctrl Pts',(-3.91787251936688,-1.,-1.13788084225511));
#45327=CARTESIAN_POINT('Ctrl Pts',(-3.91787251936688,1.,-1.13788084225511));
#45328=CARTESIAN_POINT('Ctrl Pts',(-3.91187321145495,-1.,-1.13303414693849));
#45329=CARTESIAN_POINT('Ctrl Pts',(-3.91187321145495,1.,-1.13303414693849));
#45330=CARTESIAN_POINT('Ctrl Pts',(-3.90585753318622,-1.,-1.12822258281518));
#45331=CARTESIAN_POINT('Ctrl Pts',(-3.90585753318622,1.,-1.12822258281518));
#45332=CARTESIAN_POINT('Ctrl Pts',(-3.89982569749978,-1.,-1.12344660099029));
#45333=CARTESIAN_POINT('Ctrl Pts',(-3.89982569749978,1.,-1.12344660099029));
#45334=CARTESIAN_POINT('Ctrl Pts',(-3.89377768340362,-1.,-1.11870660794609));
#45335=CARTESIAN_POINT('Ctrl Pts',(-3.89377768340362,1.,-1.11870660794609));
#45336=CARTESIAN_POINT('Ctrl Pts',(-3.88771308285229,-1.,-1.11400292434447));
#45337=CARTESIAN_POINT('Ctrl Pts',(-3.88771308285229,1.,-1.11400292434447));
#45338=CARTESIAN_POINT('Ctrl Pts',(-3.88163105531791,-1.,-1.10933577224029));
#45339=CARTESIAN_POINT('Ctrl Pts',(-3.88163105531791,1.,-1.10933577224029));
#45340=CARTESIAN_POINT('Ctrl Pts',(-3.87553067187566,-1.,-1.10470536603303));
#45341=CARTESIAN_POINT('Ctrl Pts',(-3.87553067187566,1.,-1.10470536603303));
#45342=CARTESIAN_POINT('Ctrl Pts',(-3.86941120134872,-1.,-1.10011198761202));
#45343=CARTESIAN_POINT('Ctrl Pts',(-3.86941120134872,1.,-1.10011198761202));
#45344=CARTESIAN_POINT('Ctrl Pts',(-3.86327241021242,-1.,-1.09555606505012));
#45345=CARTESIAN_POINT('Ctrl Pts',(-3.86327241021242,1.,-1.09555606505012));
#45346=CARTESIAN_POINT('Ctrl Pts',(-3.85711487933911,-1.,-1.09103825516288));
#45347=CARTESIAN_POINT('Ctrl Pts',(-3.85711487933911,1.,-1.09103825516288));
#45348=CARTESIAN_POINT('Ctrl Pts',(-3.8509402522269,-1.,-1.08655950846377));
#45349=CARTESIAN_POINT('Ctrl Pts',(-3.8509402522269,1.,-1.08655950846377));
#45350=CARTESIAN_POINT('Ctrl Pts',(-3.84475048030615,-1.,-1.08212087917986));
#45351=CARTESIAN_POINT('Ctrl Pts',(-3.84475048030615,1.,-1.08212087917986));
#45352=CARTESIAN_POINT('Ctrl Pts',(-3.83854714117486,-1.,-1.07772335353856));
#45353=CARTESIAN_POINT('Ctrl Pts',(-3.83854714117486,1.,-1.07772335353856));
#45354=CARTESIAN_POINT('Ctrl Pts',(-3.83233071195145,-1.,-1.0733676663346));
#45355=CARTESIAN_POINT('Ctrl Pts',(-3.83233071195145,1.,-1.0733676663346));
#45356=CARTESIAN_POINT('Ctrl Pts',(-3.82609989967278,-1.,-1.0690541318036));
#45357=CARTESIAN_POINT('Ctrl Pts',(-3.82609989967278,1.,-1.0690541318036));
#45358=CARTESIAN_POINT('Ctrl Pts',(-3.81985083953012,-1.,-1.06478244038931));
#45359=CARTESIAN_POINT('Ctrl Pts',(-3.81985083953012,1.,-1.06478244038931));
#45360=CARTESIAN_POINT('Ctrl Pts',(-3.81357866117485,-1.,-1.06055206187298));
#45361=CARTESIAN_POINT('Ctrl Pts',(-3.81357866117485,1.,-1.06055206187298));
#45362=CARTESIAN_POINT('Ctrl Pts',(-3.80727913637784,-1.,-1.05636266918643));
#45363=CARTESIAN_POINT('Ctrl Pts',(-3.80727913637784,1.,-1.05636266918643));
#45364=CARTESIAN_POINT('Ctrl Pts',(-3.80095039790678,-1.,-1.05221457990015));
#45365=CARTESIAN_POINT('Ctrl Pts',(-3.80095039790678,1.,-1.05221457990015));
#45366=CARTESIAN_POINT('Ctrl Pts',(-3.79459440308793,-1.,-1.04810913267641));
#45367=CARTESIAN_POINT('Ctrl Pts',(-3.79459440308793,1.,-1.04810913267641));
#45368=CARTESIAN_POINT('Ctrl Pts',(-3.78821910787195,-1.,-1.04404924374426));
#45369=CARTESIAN_POINT('Ctrl Pts',(-3.78821910787195,1.,-1.04404924374426));
#45370=CARTESIAN_POINT('Ctrl Pts',(-3.78183535008192,-1.,-1.04003862055804));
#45371=CARTESIAN_POINT('Ctrl Pts',(-3.78183535008192,1.,-1.04003862055804));
#45372=CARTESIAN_POINT('Ctrl Pts',(-3.77545283140445,-1.,-1.03608074678013));
#45373=CARTESIAN_POINT('Ctrl Pts',(-3.77545283140445,1.,-1.03608074678013));
#45374=CARTESIAN_POINT('Ctrl Pts',(-3.76907609832522,-1.,-1.0321778660492));
#45375=CARTESIAN_POINT('Ctrl Pts',(-3.76907609832522,1.,-1.0321778660492));
#45376=CARTESIAN_POINT('Ctrl Pts',(-3.76270122291232,-1.,-1.02833014458181));
#45377=CARTESIAN_POINT('Ctrl Pts',(-3.76270122291232,1.,-1.02833014458181));
#45378=CARTESIAN_POINT('Ctrl Pts',(-3.75631037456194,-1.,-1.0245342944466));
#45379=CARTESIAN_POINT('Ctrl Pts',(-3.75631037456194,1.,-1.0245342944466));
#45380=CARTESIAN_POINT('Ctrl Pts',(-3.74987777155834,-1.,-1.02078510487428));
#45381=CARTESIAN_POINT('Ctrl Pts',(-3.74987777155834,1.,-1.02078510487428));
#45382=CARTESIAN_POINT('Ctrl Pts',(-3.74337942504959,-1.,-1.01707794311079));
#45383=CARTESIAN_POINT('Ctrl Pts',(-3.74337942504959,1.,-1.01707794311079));
#45384=CARTESIAN_POINT('Ctrl Pts',(-3.73680245055734,-1.,-1.01341114319903));
#45385=CARTESIAN_POINT('Ctrl Pts',(-3.73680245055734,1.,-1.01341114319903));
#45386=CARTESIAN_POINT('Ctrl Pts',(-3.73015276704426,-1.,-1.00978798539496));
#45387=CARTESIAN_POINT('Ctrl Pts',(-3.73015276704426,1.,-1.00978798539496));
#45388=CARTESIAN_POINT('Ctrl Pts',(-3.72346803750595,-1.,-1.0062200073571));
#45389=CARTESIAN_POINT('Ctrl Pts',(-3.72346803750595,1.,-1.0062200073571));
#45390=CARTESIAN_POINT('Ctrl Pts',(-3.71680667125118,-1.,-1.00272423396822));
#45391=CARTESIAN_POINT('Ctrl Pts',(-3.71680667125118,1.,-1.00272423396822));
#45392=CARTESIAN_POINT('Ctrl Pts',(-3.71022439713938,-1.,-0.99931726075653));
#45393=CARTESIAN_POINT('Ctrl Pts',(-3.71022439713938,1.,-0.99931726075653));
#45394=CARTESIAN_POINT('Ctrl Pts',(-3.70375282282138,-1.,-0.996009819772518));
#45395=CARTESIAN_POINT('Ctrl Pts',(-3.70375282282138,1.,-0.996009819772518));
#45396=CARTESIAN_POINT('Ctrl Pts',(-3.69738123415662,-1.,-0.99280221833201));
#45397=CARTESIAN_POINT('Ctrl Pts',(-3.69738123415662,1.,-0.99280221833201));
#45398=CARTESIAN_POINT('Ctrl Pts',(-3.69102682138846,-1.,-0.989676715398558));
#45399=CARTESIAN_POINT('Ctrl Pts',(-3.69102682138846,1.,-0.989676715398558));
#45400=CARTESIAN_POINT('Ctrl Pts',(-3.68455317926068,-1.,-0.986602639863837));
#45401=CARTESIAN_POINT('Ctrl Pts',(-3.68455317926068,1.,-0.986602639863837));
#45402=CARTESIAN_POINT('Ctrl Pts',(-3.67782408841715,-1.,-0.983550791470419));
#45403=CARTESIAN_POINT('Ctrl Pts',(-3.67782408841715,1.,-0.983550791470419));
#45404=CARTESIAN_POINT('Ctrl Pts',(-3.67074983340361,-1.,-0.980505922458267));
#45405=CARTESIAN_POINT('Ctrl Pts',(-3.67074983340361,1.,-0.980505922458267));
#45406=CARTESIAN_POINT('Ctrl Pts',(-3.66333049637475,-1.,-0.977478312751618));
#45407=CARTESIAN_POINT('Ctrl Pts',(-3.66333049637475,1.,-0.977478312751618));
#45408=CARTESIAN_POINT('Ctrl Pts',(-3.65571576735126,-1.,-0.974519971354848));
#45409=CARTESIAN_POINT('Ctrl Pts',(-3.65571576735126,1.,-0.974519971354848));
#45410=CARTESIAN_POINT('Ctrl Pts',(-3.64819756447455,-1.,-0.971722122061341));
#45411=CARTESIAN_POINT('Ctrl Pts',(-3.64819756447455,1.,-0.971722122061341));
#45412=CARTESIAN_POINT('Ctrl Pts',(-3.64113946505766,-1.,-0.969195124675865));
#45413=CARTESIAN_POINT('Ctrl Pts',(-3.64113946505766,1.,-0.969195124675865));
#45414=CARTESIAN_POINT('Ctrl Pts',(-3.63492122081143,-1.,-0.967052554541385));
#45415=CARTESIAN_POINT('Ctrl Pts',(-3.63492122081143,1.,-0.967052554541385));
#45416=CARTESIAN_POINT('Ctrl Pts',(-3.62988252139846,-1.,-0.965395153165293));
#45417=CARTESIAN_POINT('Ctrl Pts',(-3.62988252139846,1.,-0.965395153165293));
#45418=CARTESIAN_POINT('Ctrl Pts',(-3.62625391254797,-1.,-0.964291001273287));
#45419=CARTESIAN_POINT('Ctrl Pts',(-3.62625391254797,1.,-0.964291001273287));
#45420=CARTESIAN_POINT('Ctrl Pts',(-3.6245656860652,-1.,-0.963875774530619));
#45421=CARTESIAN_POINT('Ctrl Pts',(-3.6245656860652,1.,-0.963875774530619));
#45422=CARTESIAN_POINT('Ctrl Pts',(-3.62399933639914,-1.,-0.963832486395051));
#45423=CARTESIAN_POINT('Ctrl Pts',(-3.62399933639914,1.,-0.963832486395051));
#45424=CARTESIAN_POINT('Ctrl Pts',(-3.62393257642052,-1.,-0.963922720982193));
#45425=CARTESIAN_POINT('Ctrl Pts',(-3.62393257642052,1.,-0.963922720982193));
#45426=CARTESIAN_POINT('Ctrl Pts',(-3.62397690409552,-1.,-0.963997613369571));
#45427=CARTESIAN_POINT('Ctrl Pts',(-3.62397690409552,1.,-0.963997613369571));
#45428=CARTESIAN_POINT('',(-4.01728681790024,1.,-1.22531898815164));
#45429=CARTESIAN_POINT('Ctrl Pts',(-4.01728681790024,1.,-1.22531898815164));
#45430=CARTESIAN_POINT('Ctrl Pts',(-4.0161454457032,1.,-1.22423716681447));
#45431=CARTESIAN_POINT('Ctrl Pts',(-4.01386104434674,1.,-1.22207656456199));
#45432=CARTESIAN_POINT('Ctrl Pts',(-4.01042947142681,1.,-1.21884478244983));
#45433=CARTESIAN_POINT('Ctrl Pts',(-4.00584409524937,1.,-1.21455398918813));
#45434=CARTESIAN_POINT('Ctrl Pts',(-4.00009577952534,1.,-1.20922097030107));
#45435=CARTESIAN_POINT('Ctrl Pts',(-3.99433084800649,1.,-1.2039185237544));
#45436=CARTESIAN_POINT('Ctrl Pts',(-3.98854928957287,1.,-1.19864679609596));
#45437=CARTESIAN_POINT('Ctrl Pts',(-3.98275111052015,1.,-1.19340598349307));
#45438=CARTESIAN_POINT('Ctrl Pts',(-3.97693634766926,1.,-1.18819633715285));
#45439=CARTESIAN_POINT('Ctrl Pts',(-3.9711050516465,1.,-1.18301815039596));
#45440=CARTESIAN_POINT('Ctrl Pts',(-3.96525726357682,1.,-1.17787174135445));
#45441=CARTESIAN_POINT('Ctrl Pts',(-3.95939299213164,1.,-1.17275743590327));
#45442=CARTESIAN_POINT('Ctrl Pts',(-3.95351219510062,1.,-1.16767555244495));
#45443=CARTESIAN_POINT('Ctrl Pts',(-3.9476147478092,1.,-1.16262637999261));
#45444=CARTESIAN_POINT('Ctrl Pts',(-3.94170046685542,1.,-1.1576101834106));
#45445=CARTESIAN_POINT('Ctrl Pts',(-3.9357691705651,1.,-1.1526272271639));
#45446=CARTESIAN_POINT('Ctrl Pts',(-3.92982073294334,1.,-1.14767779451147));
#45447=CARTESIAN_POINT('Ctrl Pts',(-3.92385513133937,1.,-1.14276220561575));
#45448=CARTESIAN_POINT('Ctrl Pts',(-3.91787251936688,1.,-1.13788084225511));
#45449=CARTESIAN_POINT('Ctrl Pts',(-3.91187321145495,1.,-1.13303414693849));
#45450=CARTESIAN_POINT('Ctrl Pts',(-3.90585753318622,1.,-1.12822258281518));
#45451=CARTESIAN_POINT('Ctrl Pts',(-3.89982569749978,1.,-1.12344660099029));
#45452=CARTESIAN_POINT('Ctrl Pts',(-3.89377768340362,1.,-1.11870660794609));
#45453=CARTESIAN_POINT('Ctrl Pts',(-3.88771308285229,1.,-1.11400292434447));
#45454=CARTESIAN_POINT('Ctrl Pts',(-3.88163105531791,1.,-1.10933577224029));
#45455=CARTESIAN_POINT('Ctrl Pts',(-3.87553067187566,1.,-1.10470536603303));
#45456=CARTESIAN_POINT('Ctrl Pts',(-3.86941120134872,1.,-1.10011198761202));
#45457=CARTESIAN_POINT('Ctrl Pts',(-3.86327241021242,1.,-1.09555606505012));
#45458=CARTESIAN_POINT('Ctrl Pts',(-3.85711487933911,1.,-1.09103825516288));
#45459=CARTESIAN_POINT('Ctrl Pts',(-3.8509402522269,1.,-1.08655950846377));
#45460=CARTESIAN_POINT('Ctrl Pts',(-3.84475048030615,1.,-1.08212087917986));
#45461=CARTESIAN_POINT('Ctrl Pts',(-3.83854714117486,1.,-1.07772335353856));
#45462=CARTESIAN_POINT('Ctrl Pts',(-3.83233071195145,1.,-1.0733676663346));
#45463=CARTESIAN_POINT('Ctrl Pts',(-3.82609989967278,1.,-1.0690541318036));
#45464=CARTESIAN_POINT('Ctrl Pts',(-3.81985083953012,1.,-1.06478244038931));
#45465=CARTESIAN_POINT('Ctrl Pts',(-3.81357866117485,1.,-1.06055206187298));
#45466=CARTESIAN_POINT('Ctrl Pts',(-3.80727913637784,1.,-1.05636266918643));
#45467=CARTESIAN_POINT('Ctrl Pts',(-3.80095039790678,1.,-1.05221457990015));
#45468=CARTESIAN_POINT('Ctrl Pts',(-3.79459440308793,1.,-1.04810913267641));
#45469=CARTESIAN_POINT('Ctrl Pts',(-3.78821910787195,1.,-1.04404924374426));
#45470=CARTESIAN_POINT('Ctrl Pts',(-3.78183535008192,1.,-1.04003862055804));
#45471=CARTESIAN_POINT('Ctrl Pts',(-3.77545283140445,1.,-1.03608074678013));
#45472=CARTESIAN_POINT('Ctrl Pts',(-3.76907609832522,1.,-1.0321778660492));
#45473=CARTESIAN_POINT('Ctrl Pts',(-3.76270122291232,1.,-1.02833014458181));
#45474=CARTESIAN_POINT('Ctrl Pts',(-3.75631037456194,1.,-1.0245342944466));
#45475=CARTESIAN_POINT('Ctrl Pts',(-3.74987777155834,1.,-1.02078510487428));
#45476=CARTESIAN_POINT('Ctrl Pts',(-3.74337942504959,1.,-1.01707794311079));
#45477=CARTESIAN_POINT('Ctrl Pts',(-3.73680245055734,1.,-1.01341114319903));
#45478=CARTESIAN_POINT('Ctrl Pts',(-3.73015276704426,1.,-1.00978798539496));
#45479=CARTESIAN_POINT('Ctrl Pts',(-3.72346803750595,1.,-1.0062200073571));
#45480=CARTESIAN_POINT('Ctrl Pts',(-3.71680667125118,1.,-1.00272423396822));
#45481=CARTESIAN_POINT('Ctrl Pts',(-3.71022439713938,1.,-0.99931726075653));
#45482=CARTESIAN_POINT('Ctrl Pts',(-3.70375282282138,1.,-0.996009819772518));
#45483=CARTESIAN_POINT('Ctrl Pts',(-3.69738123415662,1.,-0.99280221833201));
#45484=CARTESIAN_POINT('Ctrl Pts',(-3.69102682138846,1.,-0.989676715398558));
#45485=CARTESIAN_POINT('Ctrl Pts',(-3.68455317926068,1.,-0.986602639863837));
#45486=CARTESIAN_POINT('Ctrl Pts',(-3.67782408841715,1.,-0.983550791470419));
#45487=CARTESIAN_POINT('Ctrl Pts',(-3.67074983340361,1.,-0.980505922458267));
#45488=CARTESIAN_POINT('Ctrl Pts',(-3.66333049637475,1.,-0.977478312751618));
#45489=CARTESIAN_POINT('Ctrl Pts',(-3.65571576735126,1.,-0.974519971354848));
#45490=CARTESIAN_POINT('Ctrl Pts',(-3.64819756447455,1.,-0.971722122061341));
#45491=CARTESIAN_POINT('Ctrl Pts',(-3.64113946505766,1.,-0.969195124675865));
#45492=CARTESIAN_POINT('Ctrl Pts',(-3.63492122081143,1.,-0.967052554541385));
#45493=CARTESIAN_POINT('Ctrl Pts',(-3.62988252139846,1.,-0.965395153165293));
#45494=CARTESIAN_POINT('Ctrl Pts',(-3.62652618145335,1.,-0.964373850166458));
#45495=CARTESIAN_POINT('Ctrl Pts',(-3.62489305727662,1.,-0.963957782642843));
#45496=CARTESIAN_POINT('Ctrl Pts',(-3.62424461507588,1.,-0.963861297423241));
#45497=CARTESIAN_POINT('Ctrl Pts',(-3.6240482887845,1.,-0.963880158555582));
#45498=CARTESIAN_POINT('Ctrl Pts',(-3.62400312501245,1.,-0.963899035117249));
#45499=CARTESIAN_POINT('',(-4.01728681790024,0.,-1.22531898815164));
#45500=CARTESIAN_POINT('Ctrl Pts',(-3.49848248301936,-1.,-1.35022972712301));
#45501=CARTESIAN_POINT('Ctrl Pts',(-3.49848248301936,1.,-1.35022972712301));
#45502=CARTESIAN_POINT('Ctrl Pts',(-3.4984026005375,-1.,-1.35026426118402));
#45503=CARTESIAN_POINT('Ctrl Pts',(-3.4984026005375,1.,-1.35026426118402));
#45504=CARTESIAN_POINT('Ctrl Pts',(-3.49840357193736,-1.,-1.35037650303019));
#45505=CARTESIAN_POINT('Ctrl Pts',(-3.49840357193736,1.,-1.35037650303019));
#45506=CARTESIAN_POINT('Ctrl Pts',(-3.49888720257132,-1.,-1.35067437417483));
#45507=CARTESIAN_POINT('Ctrl Pts',(-3.49888720257132,1.,-1.35067437417483));
#45508=CARTESIAN_POINT('Ctrl Pts',(-3.5004970706414,-1.,-1.3513307633124));
#45509=CARTESIAN_POINT('Ctrl Pts',(-3.5004970706414,1.,-1.3513307633124));
#45510=CARTESIAN_POINT('Ctrl Pts',(-3.50408168106261,-1.,-1.35257032843486));
#45511=CARTESIAN_POINT('Ctrl Pts',(-3.50408168106261,1.,-1.35257032843486));
#45512=CARTESIAN_POINT('Ctrl Pts',(-3.50913227059999,-1.,-1.35419113575956));
#45513=CARTESIAN_POINT('Ctrl Pts',(-3.50913227059999,1.,-1.35419113575956));
#45514=CARTESIAN_POINT('Ctrl Pts',(-3.51542230699556,-1.,-1.35611275237152));
#45515=CARTESIAN_POINT('Ctrl Pts',(-3.51542230699556,1.,-1.35611275237152));
#45516=CARTESIAN_POINT('Ctrl Pts',(-3.52261776116748,-1.,-1.35821701528836));
#45517=CARTESIAN_POINT('Ctrl Pts',(-3.52261776116748,1.,-1.35821701528836));
#45518=CARTESIAN_POINT('Ctrl Pts',(-3.530344649616,-1.,-1.36037259643734));
#45519=CARTESIAN_POINT('Ctrl Pts',(-3.530344649616,1.,-1.36037259643734));
#45520=CARTESIAN_POINT('Ctrl Pts',(-3.53824396424961,-1.,-1.36245507339307));
#45521=CARTESIAN_POINT('Ctrl Pts',(-3.53824396424961,1.,-1.36245507339307));
#45522=CARTESIAN_POINT('Ctrl Pts',(-3.54602591832973,-1.,-1.36436666257597));
#45523=CARTESIAN_POINT('Ctrl Pts',(-3.54602591832973,1.,-1.36436666257597));
#45524=CARTESIAN_POINT('Ctrl Pts',(-3.55353883995949,-1.,-1.3660614545677));
#45525=CARTESIAN_POINT('Ctrl Pts',(-3.55353883995949,1.,-1.3660614545677));
#45526=CARTESIAN_POINT('Ctrl Pts',(-3.56077662028649,-1.,-1.36754771771233));
#45527=CARTESIAN_POINT('Ctrl Pts',(-3.56077662028649,1.,-1.36754771771233));
#45528=CARTESIAN_POINT('Ctrl Pts',(-3.5678208030466,-1.,-1.36886584973389));
#45529=CARTESIAN_POINT('Ctrl Pts',(-3.5678208030466,1.,-1.36886584973389));
#45530=CARTESIAN_POINT('Ctrl Pts',(-3.57479875549486,-1.,-1.37007229485659));
#45531=CARTESIAN_POINT('Ctrl Pts',(-3.57479875549486,1.,-1.37007229485659));
#45532=CARTESIAN_POINT('Ctrl Pts',(-3.58183885982715,-1.,-1.37122241663062));
#45533=CARTESIAN_POINT('Ctrl Pts',(-3.58183885982715,1.,-1.37122241663062));
#45534=CARTESIAN_POINT('Ctrl Pts',(-3.58901853846365,-1.,-1.37235053660976));
#45535=CARTESIAN_POINT('Ctrl Pts',(-3.58901853846365,1.,-1.37235053660976));
#45536=CARTESIAN_POINT('Ctrl Pts',(-3.59634627869048,-1.,-1.37346320103157));
#45537=CARTESIAN_POINT('Ctrl Pts',(-3.59634627869048,1.,-1.37346320103157));
#45538=CARTESIAN_POINT('Ctrl Pts',(-3.60379020123988,-1.,-1.37455051379623));
#45539=CARTESIAN_POINT('Ctrl Pts',(-3.60379020123988,1.,-1.37455051379623));
#45540=CARTESIAN_POINT('Ctrl Pts',(-3.61129546591064,-1.,-1.37559314436634));
#45541=CARTESIAN_POINT('Ctrl Pts',(-3.61129546591064,1.,-1.37559314436634));
#45542=CARTESIAN_POINT('Ctrl Pts',(-3.6188048116042,-1.,-1.37657053403107));
#45543=CARTESIAN_POINT('Ctrl Pts',(-3.6188048116042,1.,-1.37657053403107));
#45544=CARTESIAN_POINT('Ctrl Pts',(-3.62628098665145,-1.,-1.37746987919881));
#45545=CARTESIAN_POINT('Ctrl Pts',(-3.62628098665145,1.,-1.37746987919881));
#45546=CARTESIAN_POINT('Ctrl Pts',(-3.63371727442486,-1.,-1.37829035457339));
#45547=CARTESIAN_POINT('Ctrl Pts',(-3.63371727442486,1.,-1.37829035457339));
#45548=CARTESIAN_POINT('Ctrl Pts',(-3.64112507791141,-1.,-1.37903818567359));
#45549=CARTESIAN_POINT('Ctrl Pts',(-3.64112507791141,1.,-1.37903818567359));
#45550=CARTESIAN_POINT('Ctrl Pts',(-3.64852652756456,-1.,-1.37972372481603));
#45551=CARTESIAN_POINT('Ctrl Pts',(-3.64852652756456,1.,-1.37972372481603));
#45552=CARTESIAN_POINT('Ctrl Pts',(-3.6559455440439,-1.,-1.38035791051212));
#45553=CARTESIAN_POINT('Ctrl Pts',(-3.6559455440439,1.,-1.38035791051212));
#45554=CARTESIAN_POINT('Ctrl Pts',(-3.66339848520857,-1.,-1.38094856333552));
#45555=CARTESIAN_POINT('Ctrl Pts',(-3.66339848520857,1.,-1.38094856333552));
#45556=CARTESIAN_POINT('Ctrl Pts',(-3.67088843112262,-1.,-1.38149812653868));
#45557=CARTESIAN_POINT('Ctrl Pts',(-3.67088843112262,1.,-1.38149812653868));
#45558=CARTESIAN_POINT('Ctrl Pts',(-3.67841038482414,-1.,-1.3820057429062));
#45559=CARTESIAN_POINT('Ctrl Pts',(-3.67841038482414,1.,-1.3820057429062));
#45560=CARTESIAN_POINT('Ctrl Pts',(-3.68595444983837,-1.,-1.38246852827182));
#45561=CARTESIAN_POINT('Ctrl Pts',(-3.68595444983837,1.,-1.38246852827182));
#45562=CARTESIAN_POINT('Ctrl Pts',(-3.69350967899526,-1.,-1.3828831117165));
#45563=CARTESIAN_POINT('Ctrl Pts',(-3.69350967899526,1.,-1.3828831117165));
#45564=CARTESIAN_POINT('Ctrl Pts',(-3.701067921679,-1.,-1.38324717612865));
#45565=CARTESIAN_POINT('Ctrl Pts',(-3.701067921679,1.,-1.38324717612865));
#45566=CARTESIAN_POINT('Ctrl Pts',(-3.70862680753347,-1.,-1.38356065402124));
#45567=CARTESIAN_POINT('Ctrl Pts',(-3.70862680753347,1.,-1.38356065402124));
#45568=CARTESIAN_POINT('Ctrl Pts',(-3.7161876605181,-1.,-1.38382489984586));
#45569=CARTESIAN_POINT('Ctrl Pts',(-3.7161876605181,1.,-1.38382489984586));
#45570=CARTESIAN_POINT('Ctrl Pts',(-3.72375409358803,-1.,-1.3840421342895));
#45571=CARTESIAN_POINT('Ctrl Pts',(-3.72375409358803,1.,-1.3840421342895));
#45572=CARTESIAN_POINT('Ctrl Pts',(-3.73133035859282,-1.,-1.38421479111531));
#45573=CARTESIAN_POINT('Ctrl Pts',(-3.73133035859282,1.,-1.38421479111531));
#45574=CARTESIAN_POINT('Ctrl Pts',(-3.73891976418104,-1.,-1.38434489156458));
#45575=CARTESIAN_POINT('Ctrl Pts',(-3.73891976418104,1.,-1.38434489156458));
#45576=CARTESIAN_POINT('Ctrl Pts',(-3.74652317167876,-1.,-1.38443344984394));
#45577=CARTESIAN_POINT('Ctrl Pts',(-3.74652317167876,1.,-1.38443344984394));
#45578=CARTESIAN_POINT('Ctrl Pts',(-3.7541397631875,-1.,-1.38448077997163));
#45579=CARTESIAN_POINT('Ctrl Pts',(-3.7541397631875,1.,-1.38448077997163));
#45580=CARTESIAN_POINT('Ctrl Pts',(-3.76176768271367,-1.,-1.3844867525335));
#45581=CARTESIAN_POINT('Ctrl Pts',(-3.76176768271367,1.,-1.3844867525335));
#45582=CARTESIAN_POINT('Ctrl Pts',(-3.76940473185779,-1.,-1.38445107339518));
#45583=CARTESIAN_POINT('Ctrl Pts',(-3.76940473185779,1.,-1.38445107339518));
#45584=CARTESIAN_POINT('Ctrl Pts',(-3.77704902230418,-1.,-1.38437354551428));
#45585=CARTESIAN_POINT('Ctrl Pts',(-3.77704902230418,1.,-1.38437354551428));
#45586=CARTESIAN_POINT('Ctrl Pts',(-3.78469969805082,-1.,-1.38425435883756));
#45587=CARTESIAN_POINT('Ctrl Pts',(-3.78469969805082,1.,-1.38425435883756));
#45588=CARTESIAN_POINT('Ctrl Pts',(-3.79235669640841,-1.,-1.38409399694566));
#45589=CARTESIAN_POINT('Ctrl Pts',(-3.79235669640841,1.,-1.38409399694566));
#45590=CARTESIAN_POINT('Ctrl Pts',(-3.80002044322111,-1.,-1.38389311766682));
#45591=CARTESIAN_POINT('Ctrl Pts',(-3.80002044322111,1.,-1.38389311766682));
#45592=CARTESIAN_POINT('Ctrl Pts',(-3.80769156398411,-1.,-1.3836524404622));
#45593=CARTESIAN_POINT('Ctrl Pts',(-3.80769156398411,1.,-1.3836524404622));
#45594=CARTESIAN_POINT('Ctrl Pts',(-3.81537060817811,-1.,-1.38337263902782));
#45595=CARTESIAN_POINT('Ctrl Pts',(-3.81537060817811,1.,-1.38337263902782));
#45596=CARTESIAN_POINT('Ctrl Pts',(-3.82305771743829,-1.,-1.38305421262763));
#45597=CARTESIAN_POINT('Ctrl Pts',(-3.82305771743829,1.,-1.38305421262763));
#45598=CARTESIAN_POINT('Ctrl Pts',(-3.8307526698229,-1.,-1.38269750245138));
#45599=CARTESIAN_POINT('Ctrl Pts',(-3.8307526698229,1.,-1.38269750245138));
#45600=CARTESIAN_POINT('Ctrl Pts',(-3.83845502790746,-1.,-1.38230274828821));
#45601=CARTESIAN_POINT('Ctrl Pts',(-3.83845502790746,1.,-1.38230274828821));
#45602=CARTESIAN_POINT('Ctrl Pts',(-3.84616425605764,-1.,-1.38187013346109));
#45603=CARTESIAN_POINT('Ctrl Pts',(-3.84616425605764,1.,-1.38187013346109));
#45604=CARTESIAN_POINT('Ctrl Pts',(-3.85387983979481,-1.,-1.38139983115049));
#45605=CARTESIAN_POINT('Ctrl Pts',(-3.85387983979481,1.,-1.38139983115049));
#45606=CARTESIAN_POINT('Ctrl Pts',(-3.86160143043959,-1.,-1.38089205992989));
#45607=CARTESIAN_POINT('Ctrl Pts',(-3.86160143043959,1.,-1.38089205992989));
#45608=CARTESIAN_POINT('Ctrl Pts',(-3.86932885813068,-1.,-1.38034709213014));
#45609=CARTESIAN_POINT('Ctrl Pts',(-3.86932885813068,1.,-1.38034709213014));
#45610=CARTESIAN_POINT('Ctrl Pts',(-3.87706205830532,-1.,-1.37976523097073));
#45611=CARTESIAN_POINT('Ctrl Pts',(-3.87706205830532,1.,-1.37976523097073));
#45612=CARTESIAN_POINT('Ctrl Pts',(-3.88480102249277,-1.,-1.37914679719383));
#45613=CARTESIAN_POINT('Ctrl Pts',(-3.88480102249277,1.,-1.37914679719383));
#45614=CARTESIAN_POINT('Ctrl Pts',(-3.89254574338496,-1.,-1.3784921128802));
#45615=CARTESIAN_POINT('Ctrl Pts',(-3.89254574338496,1.,-1.3784921128802));
#45616=CARTESIAN_POINT('Ctrl Pts',(-3.90029615196727,-1.,-1.37780148512792));
#45617=CARTESIAN_POINT('Ctrl Pts',(-3.90029615196727,1.,-1.37780148512792));
#45618=CARTESIAN_POINT('Ctrl Pts',(-3.90805209523486,-1.,-1.3770751963402));
#45619=CARTESIAN_POINT('Ctrl Pts',(-3.90805209523486,1.,-1.3770751963402));
#45620=CARTESIAN_POINT('Ctrl Pts',(-3.91581337462644,-1.,-1.37631350505797));
#45621=CARTESIAN_POINT('Ctrl Pts',(-3.91581337462644,1.,-1.37631350505797));
#45622=CARTESIAN_POINT('Ctrl Pts',(-3.92357976987672,-1.,-1.37551664448242));
#45623=CARTESIAN_POINT('Ctrl Pts',(-3.92357976987672,1.,-1.37551664448242));
#45624=CARTESIAN_POINT('Ctrl Pts',(-3.93135106761844,-1.,-1.37468482215751));
#45625=CARTESIAN_POINT('Ctrl Pts',(-3.93135106761844,1.,-1.37468482215751));
#45626=CARTESIAN_POINT('Ctrl Pts',(-3.93912709040818,-1.,-1.37381821967165));
#45627=CARTESIAN_POINT('Ctrl Pts',(-3.93912709040818,1.,-1.37381821967165));
#45628=CARTESIAN_POINT('Ctrl Pts',(-3.94690771785133,-1.,-1.37291699202807));
#45629=CARTESIAN_POINT('Ctrl Pts',(-3.94690771785133,1.,-1.37291699202807));
#45630=CARTESIAN_POINT('Ctrl Pts',(-3.95469287280914,-1.,-1.37198126432386));
#45631=CARTESIAN_POINT('Ctrl Pts',(-3.95469287280914,1.,-1.37198126432386));
#45632=CARTESIAN_POINT('Ctrl Pts',(-3.96092458506535,-1.,-1.3712051561502));
#45633=CARTESIAN_POINT('Ctrl Pts',(-3.96092458506535,1.,-1.3712051561502));
#45634=CARTESIAN_POINT('Ctrl Pts',(-3.96560037974645,-1.,-1.37060761745635));
#45635=CARTESIAN_POINT('Ctrl Pts',(-3.96560037974645,1.,-1.37060761745635));
#45636=CARTESIAN_POINT('Ctrl Pts',(-3.9687184694131,-1.,-1.37020239094614));
#45637=CARTESIAN_POINT('Ctrl Pts',(-3.9687184694131,1.,-1.37020239094614));
#45638=CARTESIAN_POINT('Ctrl Pts',(-3.97027773754922,-1.,-1.36999806084572));
#45639=CARTESIAN_POINT('Ctrl Pts',(-3.97027773754922,1.,-1.36999806084572));
#45640=CARTESIAN_POINT('',(-3.4984457533445,1.,-1.35032489087101));
#45641=CARTESIAN_POINT('Ctrl Pts',(-3.4984457533445,-1.,-1.35032489087101));
#45642=CARTESIAN_POINT('Ctrl Pts',(-3.4984457533445,-0.666666666666667,
-1.35032489087101));
#45643=CARTESIAN_POINT('Ctrl Pts',(-3.4984457533445,-0.333333333333333,
-1.35032489087101));
#45644=CARTESIAN_POINT('Ctrl Pts',(-3.4984457533445,0.333333333333333,-1.35032489087101));
#45645=CARTESIAN_POINT('Ctrl Pts',(-3.4984457533445,0.666666666666667,-1.35032489087101));
#45646=CARTESIAN_POINT('Ctrl Pts',(-3.4984457533445,1.,-1.35032489087101));
#45647=CARTESIAN_POINT('',(-3.97027773754922,1.,-1.36999806084572));
#45648=CARTESIAN_POINT('',(-3.97027773754922,0.,-1.36999806084572));
#45649=CARTESIAN_POINT('Ctrl Pts',(-3.4984457533445,1.,-1.35032489087101));
#45650=CARTESIAN_POINT('Ctrl Pts',(-3.49847119623846,1.,-1.35036670892966));
#45651=CARTESIAN_POINT('Ctrl Pts',(-3.49861894124827,1.,-1.35049736560527));
#45652=CARTESIAN_POINT('Ctrl Pts',(-3.49920025459723,1.,-1.35080045218587));
#45653=CARTESIAN_POINT('Ctrl Pts',(-3.5007660381649,1.,-1.35142377279517));
#45654=CARTESIAN_POINT('Ctrl Pts',(-3.50408168106261,1.,-1.35257032843486));
#45655=CARTESIAN_POINT('Ctrl Pts',(-3.50913227059999,1.,-1.35419113575956));
#45656=CARTESIAN_POINT('Ctrl Pts',(-3.51542230699556,1.,-1.35611275237152));
#45657=CARTESIAN_POINT('Ctrl Pts',(-3.52261776116748,1.,-1.35821701528836));
#45658=CARTESIAN_POINT('Ctrl Pts',(-3.530344649616,1.,-1.36037259643734));
#45659=CARTESIAN_POINT('Ctrl Pts',(-3.53824396424961,1.,-1.36245507339307));
#45660=CARTESIAN_POINT('Ctrl Pts',(-3.54602591832973,1.,-1.36436666257597));
#45661=CARTESIAN_POINT('Ctrl Pts',(-3.55353883995949,1.,-1.3660614545677));
#45662=CARTESIAN_POINT('Ctrl Pts',(-3.56077662028649,1.,-1.36754771771233));
#45663=CARTESIAN_POINT('Ctrl Pts',(-3.5678208030466,1.,-1.36886584973389));
#45664=CARTESIAN_POINT('Ctrl Pts',(-3.57479875549486,1.,-1.37007229485659));
#45665=CARTESIAN_POINT('Ctrl Pts',(-3.58183885982715,1.,-1.37122241663062));
#45666=CARTESIAN_POINT('Ctrl Pts',(-3.58901853846365,1.,-1.37235053660976));
#45667=CARTESIAN_POINT('Ctrl Pts',(-3.59634627869048,1.,-1.37346320103157));
#45668=CARTESIAN_POINT('Ctrl Pts',(-3.60379020123988,1.,-1.37455051379623));
#45669=CARTESIAN_POINT('Ctrl Pts',(-3.61129546591064,1.,-1.37559314436634));
#45670=CARTESIAN_POINT('Ctrl Pts',(-3.6188048116042,1.,-1.37657053403107));
#45671=CARTESIAN_POINT('Ctrl Pts',(-3.62628098665145,1.,-1.37746987919881));
#45672=CARTESIAN_POINT('Ctrl Pts',(-3.63371727442486,1.,-1.37829035457339));
#45673=CARTESIAN_POINT('Ctrl Pts',(-3.64112507791141,1.,-1.37903818567359));
#45674=CARTESIAN_POINT('Ctrl Pts',(-3.64852652756456,1.,-1.37972372481603));
#45675=CARTESIAN_POINT('Ctrl Pts',(-3.6559455440439,1.,-1.38035791051212));
#45676=CARTESIAN_POINT('Ctrl Pts',(-3.66339848520857,1.,-1.38094856333552));
#45677=CARTESIAN_POINT('Ctrl Pts',(-3.67088843112262,1.,-1.38149812653868));
#45678=CARTESIAN_POINT('Ctrl Pts',(-3.67841038482414,1.,-1.3820057429062));
#45679=CARTESIAN_POINT('Ctrl Pts',(-3.68595444983837,1.,-1.38246852827182));
#45680=CARTESIAN_POINT('Ctrl Pts',(-3.69350967899526,1.,-1.3828831117165));
#45681=CARTESIAN_POINT('Ctrl Pts',(-3.701067921679,1.,-1.38324717612865));
#45682=CARTESIAN_POINT('Ctrl Pts',(-3.70862680753347,1.,-1.38356065402124));
#45683=CARTESIAN_POINT('Ctrl Pts',(-3.7161876605181,1.,-1.38382489984586));
#45684=CARTESIAN_POINT('Ctrl Pts',(-3.72375409358803,1.,-1.3840421342895));
#45685=CARTESIAN_POINT('Ctrl Pts',(-3.73133035859282,1.,-1.38421479111531));
#45686=CARTESIAN_POINT('Ctrl Pts',(-3.73891976418104,1.,-1.38434489156458));
#45687=CARTESIAN_POINT('Ctrl Pts',(-3.74652317167876,1.,-1.38443344984394));
#45688=CARTESIAN_POINT('Ctrl Pts',(-3.7541397631875,1.,-1.38448077997163));
#45689=CARTESIAN_POINT('Ctrl Pts',(-3.76176768271367,1.,-1.3844867525335));
#45690=CARTESIAN_POINT('Ctrl Pts',(-3.76940473185779,1.,-1.38445107339518));
#45691=CARTESIAN_POINT('Ctrl Pts',(-3.77704902230418,1.,-1.38437354551428));
#45692=CARTESIAN_POINT('Ctrl Pts',(-3.78469969805082,1.,-1.38425435883756));
#45693=CARTESIAN_POINT('Ctrl Pts',(-3.79235669640841,1.,-1.38409399694566));
#45694=CARTESIAN_POINT('Ctrl Pts',(-3.80002044322111,1.,-1.38389311766682));
#45695=CARTESIAN_POINT('Ctrl Pts',(-3.80769156398411,1.,-1.3836524404622));
#45696=CARTESIAN_POINT('Ctrl Pts',(-3.81537060817811,1.,-1.38337263902782));
#45697=CARTESIAN_POINT('Ctrl Pts',(-3.82305771743829,1.,-1.38305421262763));
#45698=CARTESIAN_POINT('Ctrl Pts',(-3.8307526698229,1.,-1.38269750245138));
#45699=CARTESIAN_POINT('Ctrl Pts',(-3.83845502790746,1.,-1.38230274828821));
#45700=CARTESIAN_POINT('Ctrl Pts',(-3.84616425605764,1.,-1.38187013346109));
#45701=CARTESIAN_POINT('Ctrl Pts',(-3.85387983979481,1.,-1.38139983115049));
#45702=CARTESIAN_POINT('Ctrl Pts',(-3.86160143043959,1.,-1.38089205992989));
#45703=CARTESIAN_POINT('Ctrl Pts',(-3.86932885813068,1.,-1.38034709213014));
#45704=CARTESIAN_POINT('Ctrl Pts',(-3.87706205830532,1.,-1.37976523097073));
#45705=CARTESIAN_POINT('Ctrl Pts',(-3.88480102249277,1.,-1.37914679719383));
#45706=CARTESIAN_POINT('Ctrl Pts',(-3.89254574338496,1.,-1.3784921128802));
#45707=CARTESIAN_POINT('Ctrl Pts',(-3.90029615196727,1.,-1.37780148512792));
#45708=CARTESIAN_POINT('Ctrl Pts',(-3.90805209523486,1.,-1.3770751963402));
#45709=CARTESIAN_POINT('Ctrl Pts',(-3.91581337462644,1.,-1.37631350505797));
#45710=CARTESIAN_POINT('Ctrl Pts',(-3.92357976987672,1.,-1.37551664448242));
#45711=CARTESIAN_POINT('Ctrl Pts',(-3.93135106761844,1.,-1.37468482215751));
#45712=CARTESIAN_POINT('Ctrl Pts',(-3.93912709040818,1.,-1.37381821967165));
#45713=CARTESIAN_POINT('Ctrl Pts',(-3.94690771785133,1.,-1.37291699202807));
#45714=CARTESIAN_POINT('Ctrl Pts',(-3.95469287280914,1.,-1.37198126432386));
#45715=CARTESIAN_POINT('Ctrl Pts',(-3.96092458506535,1.,-1.3712051561502));
#45716=CARTESIAN_POINT('Ctrl Pts',(-3.96560037974645,1.,-1.37060761745635));
#45717=CARTESIAN_POINT('Ctrl Pts',(-3.9687184694131,1.,-1.37020239094614));
#45718=CARTESIAN_POINT('Ctrl Pts',(-3.97027773754922,1.,-1.36999806084572));
#45719=CARTESIAN_POINT('Origin',(-3.97027773754922,0.,-1.36999806084572));
#45720=CARTESIAN_POINT('',(-4.01728681790024,1.,-1.22531898815164));
#45721=CARTESIAN_POINT('Origin',(0.,0.,0.));
#45722=CARTESIAN_POINT('',(-3.42859860294378,1.,-1.51895082866166));
#45723=CARTESIAN_POINT('Origin',(0.,1.,0.));
#45724=CARTESIAN_POINT('Ctrl Pts',(-3.42859860294378,1.,-1.51895082866166));
#45725=CARTESIAN_POINT('Ctrl Pts',(-3.42859860294378,0.666666666666667,
-1.51895082866166));
#45726=CARTESIAN_POINT('Ctrl Pts',(-3.42859860294378,0.333333333333333,
-1.51895082866166));
#45727=CARTESIAN_POINT('Ctrl Pts',(-3.42859860294378,-0.333333333333333,
-1.51895082866166));
#45728=CARTESIAN_POINT('Ctrl Pts',(-3.42859860294378,-0.666666666666667,
-1.51895082866166));
#45729=CARTESIAN_POINT('Ctrl Pts',(-3.42859860294378,-1.,-1.51895082866166));
#45730=CARTESIAN_POINT('Ctrl Pts',(-3.77614523045147,-1.,-1.83867539237861));
#45731=CARTESIAN_POINT('Ctrl Pts',(-3.77614523045147,1.,-1.83867539237861));
#45732=CARTESIAN_POINT('Ctrl Pts',(-3.77518714458232,-1.,-1.83742834010821));
#45733=CARTESIAN_POINT('Ctrl Pts',(-3.77518714458232,1.,-1.83742834010821));
#45734=CARTESIAN_POINT('Ctrl Pts',(-3.77326886065484,-1.,-1.83493697935064));
#45735=CARTESIAN_POINT('Ctrl Pts',(-3.77326886065484,1.,-1.83493697935064));
#45736=CARTESIAN_POINT('Ctrl Pts',(-3.77038509819777,-1.,-1.83120816956515));
#45737=CARTESIAN_POINT('Ctrl Pts',(-3.77038509819777,1.,-1.83120816956515));
#45738=CARTESIAN_POINT('Ctrl Pts',(-3.76652740355856,-1.,-1.82625289221933));
#45739=CARTESIAN_POINT('Ctrl Pts',(-3.76652740355856,1.,-1.82625289221933));
#45740=CARTESIAN_POINT('Ctrl Pts',(-3.76168412709652,-1.,-1.82008629694924));
#45741=CARTESIAN_POINT('Ctrl Pts',(-3.76168412709652,1.,-1.82008629694924));
#45742=CARTESIAN_POINT('Ctrl Pts',(-3.75681965683995,-1.,-1.81394729834032));
#45743=CARTESIAN_POINT('Ctrl Pts',(-3.75681965683995,1.,-1.81394729834032));
#45744=CARTESIAN_POINT('Ctrl Pts',(-3.75193395888069,-1.,-1.80783603939662));
#45745=CARTESIAN_POINT('Ctrl Pts',(-3.75193395888069,1.,-1.80783603939662));
#45746=CARTESIAN_POINT('Ctrl Pts',(-3.74702700874954,-1.,-1.80175271485519));
#45747=CARTESIAN_POINT('Ctrl Pts',(-3.74702700874954,1.,-1.80175271485519));
#45748=CARTESIAN_POINT('Ctrl Pts',(-3.74209880351667,-1.,-1.79569757859041));
#45749=CARTESIAN_POINT('Ctrl Pts',(-3.74209880351667,1.,-1.79569757859041));
#45750=CARTESIAN_POINT('Ctrl Pts',(-3.73714934729962,-1.,-1.78967092823139));
#45751=CARTESIAN_POINT('Ctrl Pts',(-3.73714934729962,1.,-1.78967092823139));
#45752=CARTESIAN_POINT('Ctrl Pts',(-3.73217863095022,-1.,-1.78367308442682));
#45753=CARTESIAN_POINT('Ctrl Pts',(-3.73217863095022,1.,-1.78367308442682));
#45754=CARTESIAN_POINT('Ctrl Pts',(-3.72718661205504,-1.,-1.77770437039606));
#45755=CARTESIAN_POINT('Ctrl Pts',(-3.72718661205504,1.,-1.77770437039606));
#45756=CARTESIAN_POINT('Ctrl Pts',(-3.72217319911429,-1.,-1.77176509401846));
#45757=CARTESIAN_POINT('Ctrl Pts',(-3.72217319911429,1.,-1.77176509401846));
#45758=CARTESIAN_POINT('Ctrl Pts',(-3.71713822377675,-1.,-1.76585552124549));
#45759=CARTESIAN_POINT('Ctrl Pts',(-3.71713822377675,1.,-1.76585552124549));
#45760=CARTESIAN_POINT('Ctrl Pts',(-3.71208146346454,-1.,-1.75997588499021));
#45761=CARTESIAN_POINT('Ctrl Pts',(-3.71208146346454,1.,-1.75997588499021));
#45762=CARTESIAN_POINT('Ctrl Pts',(-3.70700269736876,-1.,-1.75412641804148));
#45763=CARTESIAN_POINT('Ctrl Pts',(-3.70700269736876,1.,-1.75412641804148));
#45764=CARTESIAN_POINT('Ctrl Pts',(-3.70190175673422,-1.,-1.74830738046092));
#45765=CARTESIAN_POINT('Ctrl Pts',(-3.70190175673422,1.,-1.74830738046092));
#45766=CARTESIAN_POINT('Ctrl Pts',(-3.6967785691046,-1.,-1.74251908492589));
#45767=CARTESIAN_POINT('Ctrl Pts',(-3.6967785691046,1.,-1.74251908492589));
#45768=CARTESIAN_POINT('Ctrl Pts',(-3.69163322647906,-1.,-1.73676193254493));
#45769=CARTESIAN_POINT('Ctrl Pts',(-3.69163322647906,1.,-1.73676193254493));
#45770=CARTESIAN_POINT('Ctrl Pts',(-3.68646597019188,-1.,-1.73103640956647));
#45771=CARTESIAN_POINT('Ctrl Pts',(-3.68646597019188,1.,-1.73103640956647));
#45772=CARTESIAN_POINT('Ctrl Pts',(-3.68127704936472,-1.,-1.72534302437003));
#45773=CARTESIAN_POINT('Ctrl Pts',(-3.68127704936472,1.,-1.72534302437003));
#45774=CARTESIAN_POINT('Ctrl Pts',(-3.67606660374665,-1.,-1.71968225581787));
#45775=CARTESIAN_POINT('Ctrl Pts',(-3.67606660374665,1.,-1.71968225581787));
#45776=CARTESIAN_POINT('Ctrl Pts',(-3.67083454901629,-1.,-1.71405450210392));
#45777=CARTESIAN_POINT('Ctrl Pts',(-3.67083454901629,1.,-1.71405450210392));
#45778=CARTESIAN_POINT('Ctrl Pts',(-3.6655804319893,-1.,-1.70846001610983));
#45779=CARTESIAN_POINT('Ctrl Pts',(-3.6655804319893,1.,-1.70846001610983));
#45780=CARTESIAN_POINT('Ctrl Pts',(-3.6603033877491,-1.,-1.70289888566904));
#45781=CARTESIAN_POINT('Ctrl Pts',(-3.6603033877491,1.,-1.70289888566904));
#45782=CARTESIAN_POINT('Ctrl Pts',(-3.65500246526798,-1.,-1.69737117722558));
#45783=CARTESIAN_POINT('Ctrl Pts',(-3.65500246526798,1.,-1.69737117722558));
#45784=CARTESIAN_POINT('Ctrl Pts',(-3.64967689827393,-1.,-1.691877054817));
#45785=CARTESIAN_POINT('Ctrl Pts',(-3.64967689827393,1.,-1.691877054817));
#45786=CARTESIAN_POINT('Ctrl Pts',(-3.64432638915199,-1.,-1.68641690471455));
#45787=CARTESIAN_POINT('Ctrl Pts',(-3.64432638915199,1.,-1.68641690471455));
#45788=CARTESIAN_POINT('Ctrl Pts',(-3.63895140887443,-1.,-1.68099146651577));
#45789=CARTESIAN_POINT('Ctrl Pts',(-3.63895140887443,1.,-1.68099146651577));
#45790=CARTESIAN_POINT('Ctrl Pts',(-3.63355343201211,-1.,-1.67560193613145));
#45791=CARTESIAN_POINT('Ctrl Pts',(-3.63355343201211,1.,-1.67560193613145));
#45792=CARTESIAN_POINT('Ctrl Pts',(-3.62813422105257,-1.,-1.67024966008037));
#45793=CARTESIAN_POINT('Ctrl Pts',(-3.62813422105257,1.,-1.67024966008037));
#45794=CARTESIAN_POINT('Ctrl Pts',(-3.62269517989104,-1.,-1.66493585923853));
#45795=CARTESIAN_POINT('Ctrl Pts',(-3.62269517989104,1.,-1.66493585923853));
#45796=CARTESIAN_POINT('Ctrl Pts',(-3.61723666482457,-1.,-1.65966133399186));
#45797=CARTESIAN_POINT('Ctrl Pts',(-3.61723666482457,1.,-1.65966133399186));
#45798=CARTESIAN_POINT('Ctrl Pts',(-3.61175734965129,-1.,-1.65442619244327));
#45799=CARTESIAN_POINT('Ctrl Pts',(-3.61175734965129,1.,-1.65442619244327));
#45800=CARTESIAN_POINT('Ctrl Pts',(-3.60625346556992,-1.,-1.64922952425833));
#45801=CARTESIAN_POINT('Ctrl Pts',(-3.60625346556992,1.,-1.64922952425833));
#45802=CARTESIAN_POINT('Ctrl Pts',(-3.6007202851384,-1.,-1.6440700438558));
#45803=CARTESIAN_POINT('Ctrl Pts',(-3.6007202851384,1.,-1.6440700438558));
#45804=CARTESIAN_POINT('Ctrl Pts',(-3.59515368334887,-1.,-1.63894676675349));
#45805=CARTESIAN_POINT('Ctrl Pts',(-3.59515368334887,1.,-1.63894676675349));
#45806=CARTESIAN_POINT('Ctrl Pts',(-3.58955176627876,-1.,-1.63385971451259));
#45807=CARTESIAN_POINT('Ctrl Pts',(-3.58955176627876,1.,-1.63385971451259));
#45808=CARTESIAN_POINT('Ctrl Pts',(-3.5839162577435,-1.,-1.62881051550748));
#45809=CARTESIAN_POINT('Ctrl Pts',(-3.5839162577435,1.,-1.62881051550748));
#45810=CARTESIAN_POINT('Ctrl Pts',(-3.57825455954405,-1.,-1.62380329464851));
#45811=CARTESIAN_POINT('Ctrl Pts',(-3.57825455954405,1.,-1.62380329464851));
#45812=CARTESIAN_POINT('Ctrl Pts',(-3.57257679609826,-1.,-1.61884340915412));
#45813=CARTESIAN_POINT('Ctrl Pts',(-3.57257679609826,1.,-1.61884340915412));
#45814=CARTESIAN_POINT('Ctrl Pts',(-3.56689200468404,-1.,-1.61393581747522));
#45815=CARTESIAN_POINT('Ctrl Pts',(-3.56689200468404,1.,-1.61393581747522));
#45816=CARTESIAN_POINT('Ctrl Pts',(-3.56120432482986,-1.,-1.60908344685459));
#45817=CARTESIAN_POINT('Ctrl Pts',(-3.56120432482986,1.,-1.60908344685459));
#45818=CARTESIAN_POINT('Ctrl Pts',(-3.55550985096117,-1.,-1.60428584699848));
#45819=CARTESIAN_POINT('Ctrl Pts',(-3.55550985096117,1.,-1.60428584699848));
#45820=CARTESIAN_POINT('Ctrl Pts',(-3.54979148634426,-1.,-1.59953698113444));
#45821=CARTESIAN_POINT('Ctrl Pts',(-3.54979148634426,1.,-1.59953698113444));
#45822=CARTESIAN_POINT('Ctrl Pts',(-3.544024581823,-1.,-1.5948276694975));
#45823=CARTESIAN_POINT('Ctrl Pts',(-3.544024581823,1.,-1.5948276694975));
#45824=CARTESIAN_POINT('Ctrl Pts',(-3.53818616861045,-1.,-1.59014958368725));
#45825=CARTESIAN_POINT('Ctrl Pts',(-3.53818616861045,1.,-1.59014958368725));
#45826=CARTESIAN_POINT('Ctrl Pts',(-3.53226378147068,-1.,-1.58549906268083));
#45827=CARTESIAN_POINT('Ctrl Pts',(-3.53226378147068,1.,-1.58549906268083));
#45828=CARTESIAN_POINT('Ctrl Pts',(-3.52626275334899,-1.,-1.58088027227856));
#45829=CARTESIAN_POINT('Ctrl Pts',(-3.52626275334899,1.,-1.58088027227856));
#45830=CARTESIAN_POINT('Ctrl Pts',(-3.52021847865961,-1.,-1.5763104998818));
#45831=CARTESIAN_POINT('Ctrl Pts',(-3.52021847865961,1.,-1.5763104998818));
#45832=CARTESIAN_POINT('Ctrl Pts',(-3.51418598431733,-1.,-1.57181569799774));
#45833=CARTESIAN_POINT('Ctrl Pts',(-3.51418598431733,1.,-1.57181569799774));
#45834=CARTESIAN_POINT('Ctrl Pts',(-3.50821771695427,-1.,-1.56742097575041));
#45835=CARTESIAN_POINT('Ctrl Pts',(-3.50821771695427,1.,-1.56742097575041));
#45836=CARTESIAN_POINT('Ctrl Pts',(-3.50234321621607,-1.,-1.56314187758689));
#45837=CARTESIAN_POINT('Ctrl Pts',(-3.50234321621607,1.,-1.56314187758689));
#45838=CARTESIAN_POINT('Ctrl Pts',(-3.49655185179623,-1.,-1.55897703097859));
#45839=CARTESIAN_POINT('Ctrl Pts',(-3.49655185179623,1.,-1.55897703097859));
#45840=CARTESIAN_POINT('Ctrl Pts',(-3.49076460877317,-1.,-1.5548959590107));
#45841=CARTESIAN_POINT('Ctrl Pts',(-3.49076460877317,1.,-1.5548959590107));
#45842=CARTESIAN_POINT('Ctrl Pts',(-3.48485155928414,-1.,-1.55084702970382));
#45843=CARTESIAN_POINT('Ctrl Pts',(-3.48485155928414,1.,-1.55084702970382));
#45844=CARTESIAN_POINT('Ctrl Pts',(-3.47868272898599,-1.,-1.54678009290206));
#45845=CARTESIAN_POINT('Ctrl Pts',(-3.47868272898599,1.,-1.54678009290206));
#45846=CARTESIAN_POINT('Ctrl Pts',(-3.47217189224576,-1.,-1.54266605398152));
#45847=CARTESIAN_POINT('Ctrl Pts',(-3.47217189224576,1.,-1.54266605398152));
#45848=CARTESIAN_POINT('Ctrl Pts',(-3.46531752207222,-1.,-1.53851507915533));
#45849=CARTESIAN_POINT('Ctrl Pts',(-3.46531752207222,1.,-1.53851507915533));
#45850=CARTESIAN_POINT('Ctrl Pts',(-3.45825932955273,-1.,-1.53440195378902));
#45851=CARTESIAN_POINT('Ctrl Pts',(-3.45825932955273,1.,-1.53440195378902));
#45852=CARTESIAN_POINT('Ctrl Pts',(-3.45127136828667,-1.,-1.530462444618));
#45853=CARTESIAN_POINT('Ctrl Pts',(-3.45127136828667,1.,-1.530462444618));
#45854=CARTESIAN_POINT('Ctrl Pts',(-3.44469547527,-1.,-1.52686242875717));
#45855=CARTESIAN_POINT('Ctrl Pts',(-3.44469547527,1.,-1.52686242875717));
#45856=CARTESIAN_POINT('Ctrl Pts',(-3.43888895974182,-1.,-1.52377348950429));
#45857=CARTESIAN_POINT('Ctrl Pts',(-3.43888895974182,1.,-1.52377348950429));
#45858=CARTESIAN_POINT('Ctrl Pts',(-3.43417156977749,-1.,-1.52134826724227));
#45859=CARTESIAN_POINT('Ctrl Pts',(-3.43417156977749,1.,-1.52134826724227));
#45860=CARTESIAN_POINT('Ctrl Pts',(-3.43076036253384,-1.,-1.51969006980792));
#45861=CARTESIAN_POINT('Ctrl Pts',(-3.43076036253384,1.,-1.51969006980792));
#45862=CARTESIAN_POINT('Ctrl Pts',(-3.42915787669388,-1.,-1.51901585838879));
#45863=CARTESIAN_POINT('Ctrl Pts',(-3.42915787669388,1.,-1.51901585838879));
#45864=CARTESIAN_POINT('Ctrl Pts',(-3.42860527148835,-1.,-1.51888450659497));
#45865=CARTESIAN_POINT('Ctrl Pts',(-3.42860527148835,1.,-1.51888450659497));
#45866=CARTESIAN_POINT('Ctrl Pts',(-3.42852521763648,-1.,-1.51896318668306));
#45867=CARTESIAN_POINT('Ctrl Pts',(-3.42852521763648,1.,-1.51896318668306));
#45868=CARTESIAN_POINT('Ctrl Pts',(-3.42855728381368,-1.,-1.519044091397));
#45869=CARTESIAN_POINT('Ctrl Pts',(-3.42855728381368,1.,-1.519044091397));
#45870=CARTESIAN_POINT('',(-3.77614523045147,1.,-1.83867539237861));
#45871=CARTESIAN_POINT('Ctrl Pts',(-3.77614523045147,1.,-1.83867539237861));
#45872=CARTESIAN_POINT('Ctrl Pts',(-3.77518714458232,1.,-1.83742834010821));
#45873=CARTESIAN_POINT('Ctrl Pts',(-3.77326886065484,1.,-1.83493697935064));
#45874=CARTESIAN_POINT('Ctrl Pts',(-3.77038509819777,1.,-1.83120816956515));
#45875=CARTESIAN_POINT('Ctrl Pts',(-3.76652740355856,1.,-1.82625289221933));
#45876=CARTESIAN_POINT('Ctrl Pts',(-3.76168412709652,1.,-1.82008629694924));
#45877=CARTESIAN_POINT('Ctrl Pts',(-3.75681965683995,1.,-1.81394729834032));
#45878=CARTESIAN_POINT('Ctrl Pts',(-3.75193395888069,1.,-1.80783603939662));
#45879=CARTESIAN_POINT('Ctrl Pts',(-3.74702700874954,1.,-1.80175271485519));
#45880=CARTESIAN_POINT('Ctrl Pts',(-3.74209880351667,1.,-1.79569757859041));
#45881=CARTESIAN_POINT('Ctrl Pts',(-3.73714934729962,1.,-1.78967092823139));
#45882=CARTESIAN_POINT('Ctrl Pts',(-3.73217863095022,1.,-1.78367308442682));
#45883=CARTESIAN_POINT('Ctrl Pts',(-3.72718661205504,1.,-1.77770437039606));
#45884=CARTESIAN_POINT('Ctrl Pts',(-3.72217319911429,1.,-1.77176509401846));
#45885=CARTESIAN_POINT('Ctrl Pts',(-3.71713822377675,1.,-1.76585552124549));
#45886=CARTESIAN_POINT('Ctrl Pts',(-3.71208146346454,1.,-1.75997588499021));
#45887=CARTESIAN_POINT('Ctrl Pts',(-3.70700269736876,1.,-1.75412641804148));
#45888=CARTESIAN_POINT('Ctrl Pts',(-3.70190175673422,1.,-1.74830738046092));
#45889=CARTESIAN_POINT('Ctrl Pts',(-3.6967785691046,1.,-1.74251908492589));
#45890=CARTESIAN_POINT('Ctrl Pts',(-3.69163322647906,1.,-1.73676193254493));
#45891=CARTESIAN_POINT('Ctrl Pts',(-3.68646597019188,1.,-1.73103640956647));
#45892=CARTESIAN_POINT('Ctrl Pts',(-3.68127704936472,1.,-1.72534302437003));
#45893=CARTESIAN_POINT('Ctrl Pts',(-3.67606660374665,1.,-1.71968225581787));
#45894=CARTESIAN_POINT('Ctrl Pts',(-3.67083454901629,1.,-1.71405450210392));
#45895=CARTESIAN_POINT('Ctrl Pts',(-3.6655804319893,1.,-1.70846001610983));
#45896=CARTESIAN_POINT('Ctrl Pts',(-3.6603033877491,1.,-1.70289888566904));
#45897=CARTESIAN_POINT('Ctrl Pts',(-3.65500246526798,1.,-1.69737117722558));
#45898=CARTESIAN_POINT('Ctrl Pts',(-3.64967689827393,1.,-1.691877054817));
#45899=CARTESIAN_POINT('Ctrl Pts',(-3.64432638915199,1.,-1.68641690471455));
#45900=CARTESIAN_POINT('Ctrl Pts',(-3.63895140887443,1.,-1.68099146651577));
#45901=CARTESIAN_POINT('Ctrl Pts',(-3.63355343201211,1.,-1.67560193613145));
#45902=CARTESIAN_POINT('Ctrl Pts',(-3.62813422105257,1.,-1.67024966008037));
#45903=CARTESIAN_POINT('Ctrl Pts',(-3.62269517989104,1.,-1.66493585923853));
#45904=CARTESIAN_POINT('Ctrl Pts',(-3.61723666482457,1.,-1.65966133399186));
#45905=CARTESIAN_POINT('Ctrl Pts',(-3.61175734965129,1.,-1.65442619244327));
#45906=CARTESIAN_POINT('Ctrl Pts',(-3.60625346556992,1.,-1.64922952425833));
#45907=CARTESIAN_POINT('Ctrl Pts',(-3.6007202851384,1.,-1.6440700438558));
#45908=CARTESIAN_POINT('Ctrl Pts',(-3.59515368334887,1.,-1.63894676675349));
#45909=CARTESIAN_POINT('Ctrl Pts',(-3.58955176627876,1.,-1.63385971451259));
#45910=CARTESIAN_POINT('Ctrl Pts',(-3.5839162577435,1.,-1.62881051550748));
#45911=CARTESIAN_POINT('Ctrl Pts',(-3.57825455954405,1.,-1.62380329464851));
#45912=CARTESIAN_POINT('Ctrl Pts',(-3.57257679609826,1.,-1.61884340915412));
#45913=CARTESIAN_POINT('Ctrl Pts',(-3.56689200468404,1.,-1.61393581747522));
#45914=CARTESIAN_POINT('Ctrl Pts',(-3.56120432482986,1.,-1.60908344685459));
#45915=CARTESIAN_POINT('Ctrl Pts',(-3.55550985096117,1.,-1.60428584699848));
#45916=CARTESIAN_POINT('Ctrl Pts',(-3.54979148634426,1.,-1.59953698113444));
#45917=CARTESIAN_POINT('Ctrl Pts',(-3.544024581823,1.,-1.5948276694975));
#45918=CARTESIAN_POINT('Ctrl Pts',(-3.53818616861045,1.,-1.59014958368725));
#45919=CARTESIAN_POINT('Ctrl Pts',(-3.53226378147068,1.,-1.58549906268083));
#45920=CARTESIAN_POINT('Ctrl Pts',(-3.52626275334899,1.,-1.58088027227856));
#45921=CARTESIAN_POINT('Ctrl Pts',(-3.52021847865961,1.,-1.5763104998818));
#45922=CARTESIAN_POINT('Ctrl Pts',(-3.51418598431733,1.,-1.57181569799774));
#45923=CARTESIAN_POINT('Ctrl Pts',(-3.50821771695427,1.,-1.56742097575041));
#45924=CARTESIAN_POINT('Ctrl Pts',(-3.50234321621607,1.,-1.56314187758689));
#45925=CARTESIAN_POINT('Ctrl Pts',(-3.49655185179623,1.,-1.55897703097859));
#45926=CARTESIAN_POINT('Ctrl Pts',(-3.49076460877317,1.,-1.5548959590107));
#45927=CARTESIAN_POINT('Ctrl Pts',(-3.48485155928414,1.,-1.55084702970382));
#45928=CARTESIAN_POINT('Ctrl Pts',(-3.47868272898599,1.,-1.54678009290206));
#45929=CARTESIAN_POINT('Ctrl Pts',(-3.47217189224576,1.,-1.54266605398152));
#45930=CARTESIAN_POINT('Ctrl Pts',(-3.46531752207222,1.,-1.53851507915533));
#45931=CARTESIAN_POINT('Ctrl Pts',(-3.45825932955273,1.,-1.53440195378902));
#45932=CARTESIAN_POINT('Ctrl Pts',(-3.45127136828667,1.,-1.530462444618));
#45933=CARTESIAN_POINT('Ctrl Pts',(-3.44469547527,1.,-1.52686242875717));
#45934=CARTESIAN_POINT('Ctrl Pts',(-3.43888895974182,1.,-1.52377348950429));
#45935=CARTESIAN_POINT('Ctrl Pts',(-3.43417156977749,1.,-1.52134826724227));
#45936=CARTESIAN_POINT('Ctrl Pts',(-3.43101631893491,1.,-1.5198144909343));
#45937=CARTESIAN_POINT('Ctrl Pts',(-3.42946838852728,1.,-1.51914806898539));
#45938=CARTESIAN_POINT('Ctrl Pts',(-3.42884302333978,1.,-1.51895133295017));
#45939=CARTESIAN_POINT('Ctrl Pts',(-3.42864616361967,1.,-1.51893924967231));
#45940=CARTESIAN_POINT('Ctrl Pts',(-3.42859860294378,1.,-1.51895082866166));
#45941=CARTESIAN_POINT('',(-3.77614523045147,0.,-1.83867539237861));
#45942=CARTESIAN_POINT('Ctrl Pts',(-3.24418789321065,-1.,-1.8808893942881));
#45943=CARTESIAN_POINT('Ctrl Pts',(-3.24418789321065,1.,-1.8808893942881));
#45944=CARTESIAN_POINT('Ctrl Pts',(-3.24410359189733,-1.,-1.8809110068042));
#45945=CARTESIAN_POINT('Ctrl Pts',(-3.24410359189733,1.,-1.8809110068042));
#45946=CARTESIAN_POINT('Ctrl Pts',(-3.24408699284449,-1.,-1.8810220187274));
#45947=CARTESIAN_POINT('Ctrl Pts',(-3.24408699284449,1.,-1.8810220187274));
#45948=CARTESIAN_POINT('Ctrl Pts',(-3.24451807186964,-1.,-1.88139187908347));
#45949=CARTESIAN_POINT('Ctrl Pts',(-3.24451807186964,1.,-1.88139187908347));
#45950=CARTESIAN_POINT('Ctrl Pts',(-3.24600543790876,-1.,-1.88229202583187));
#45951=CARTESIAN_POINT('Ctrl Pts',(-3.24600543790876,1.,-1.88229202583187));
#45952=CARTESIAN_POINT('Ctrl Pts',(-3.24935200512055,-1.,-1.88407708646435));
#45953=CARTESIAN_POINT('Ctrl Pts',(-3.24935200512055,1.,-1.88407708646435));
#45954=CARTESIAN_POINT('Ctrl Pts',(-3.25408686339298,-1.,-1.88646802523372));
#45955=CARTESIAN_POINT('Ctrl Pts',(-3.25408686339298,1.,-1.88646802523372));
#45956=CARTESIAN_POINT('Ctrl Pts',(-3.2599988519361,-1.,-1.88934996203508));
#45957=CARTESIAN_POINT('Ctrl Pts',(-3.2599988519361,1.,-1.88934996203508));
#45958=CARTESIAN_POINT('Ctrl Pts',(-3.2667765388833,-1.,-1.89255393500769));
#45959=CARTESIAN_POINT('Ctrl Pts',(-3.2667765388833,1.,-1.89255393500769));
#45960=CARTESIAN_POINT('Ctrl Pts',(-3.27407108932908,-1.,-1.89589172903662));
#45961=CARTESIAN_POINT('Ctrl Pts',(-3.27407108932908,1.,-1.89589172903662));
#45962=CARTESIAN_POINT('Ctrl Pts',(-3.28154737912287,-1.,-1.89918429230424));
#45963=CARTESIAN_POINT('Ctrl Pts',(-3.28154737912287,1.,-1.89918429230424));
#45964=CARTESIAN_POINT('Ctrl Pts',(-3.28893448600364,-1.,-1.9022897124757));
#45965=CARTESIAN_POINT('Ctrl Pts',(-3.28893448600364,1.,-1.9022897124757));
#45966=CARTESIAN_POINT('Ctrl Pts',(-3.29608978722258,-1.,-1.9051389186417));
#45967=CARTESIAN_POINT('Ctrl Pts',(-3.29608978722258,1.,-1.9051389186417));
#45968=CARTESIAN_POINT('Ctrl Pts',(-3.30300595568341,-1.,-1.90773912171424));
#45969=CARTESIAN_POINT('Ctrl Pts',(-3.30300595568341,1.,-1.90773912171424));
#45970=CARTESIAN_POINT('Ctrl Pts',(-3.30975721158694,-1.,-1.91014297830502));
#45971=CARTESIAN_POINT('Ctrl Pts',(-3.30975721158694,1.,-1.91014297830502));
#45972=CARTESIAN_POINT('Ctrl Pts',(-3.31646052426395,-1.,-1.91242616234459));
#45973=CARTESIAN_POINT('Ctrl Pts',(-3.31646052426395,1.,-1.91242616234459));
#45974=CARTESIAN_POINT('Ctrl Pts',(-3.32323403454507,-1.,-1.91466343916612));
#45975=CARTESIAN_POINT('Ctrl Pts',(-3.32323403454507,1.,-1.91466343916612));
#45976=CARTESIAN_POINT('Ctrl Pts',(-3.33014884257812,-1.,-1.91690081930297));
#45977=CARTESIAN_POINT('Ctrl Pts',(-3.33014884257812,1.,-1.91690081930297));
#45978=CARTESIAN_POINT('Ctrl Pts',(-3.33721230709948,-1.,-1.91914609610173));
#45979=CARTESIAN_POINT('Ctrl Pts',(-3.33721230709948,1.,-1.91914609610173));
#45980=CARTESIAN_POINT('Ctrl Pts',(-3.34439448941915,-1.,-1.92138450828378));
#45981=CARTESIAN_POINT('Ctrl Pts',(-3.34439448941915,1.,-1.92138450828378));
#45982=CARTESIAN_POINT('Ctrl Pts',(-3.35164424847206,-1.,-1.92358838440518));
#45983=CARTESIAN_POINT('Ctrl Pts',(-3.35164424847206,1.,-1.92358838440518));
#45984=CARTESIAN_POINT('Ctrl Pts',(-3.35890824422976,-1.,-1.92572846125763));
#45985=CARTESIAN_POINT('Ctrl Pts',(-3.35890824422976,1.,-1.92572846125763));
#45986=CARTESIAN_POINT('Ctrl Pts',(-3.36615168657597,-1.,-1.92778626543803));
#45987=CARTESIAN_POINT('Ctrl Pts',(-3.36615168657597,1.,-1.92778626543803));
#45988=CARTESIAN_POINT('Ctrl Pts',(-3.37336807068078,-1.,-1.92975993109897));
#45989=CARTESIAN_POINT('Ctrl Pts',(-3.37336807068078,1.,-1.92975993109897));
#45990=CARTESIAN_POINT('Ctrl Pts',(-3.38056768525577,-1.,-1.93165739093292));
#45991=CARTESIAN_POINT('Ctrl Pts',(-3.38056768525577,1.,-1.93165739093292));
#45992=CARTESIAN_POINT('Ctrl Pts',(-3.38777076883267,-1.,-1.93349233176794));
#45993=CARTESIAN_POINT('Ctrl Pts',(-3.38777076883267,1.,-1.93349233176794));
#45994=CARTESIAN_POINT('Ctrl Pts',(-3.39499923640789,-1.,-1.93527929945982));
#45995=CARTESIAN_POINT('Ctrl Pts',(-3.39499923640789,1.,-1.93527929945982));
#45996=CARTESIAN_POINT('Ctrl Pts',(-3.40226802104093,-1.,-1.93702857723089));
#45997=CARTESIAN_POINT('Ctrl Pts',(-3.40226802104093,1.,-1.93702857723089));
#45998=CARTESIAN_POINT('Ctrl Pts',(-3.40957978266622,-1.,-1.93874306008132));
#45999=CARTESIAN_POINT('Ctrl Pts',(-3.40957978266622,1.,-1.93874306008132));
#46000=CARTESIAN_POINT('Ctrl Pts',(-3.41692971994082,-1.,-1.94042111965237));
#46001=CARTESIAN_POINT('Ctrl Pts',(-3.41692971994082,1.,-1.94042111965237));
#46002=CARTESIAN_POINT('Ctrl Pts',(-3.42430850941497,-1.,-1.94205835913692));
#46003=CARTESIAN_POINT('Ctrl Pts',(-3.42430850941497,1.,-1.94205835913692));
#46004=CARTESIAN_POINT('Ctrl Pts',(-3.43170586602436,-1.,-1.94364973660285));
#46005=CARTESIAN_POINT('Ctrl Pts',(-3.43170586602436,1.,-1.94364973660285));
#46006=CARTESIAN_POINT('Ctrl Pts',(-3.43911410197693,-1.,-1.94519168842883));
#46007=CARTESIAN_POINT('Ctrl Pts',(-3.43911410197693,1.,-1.94519168842883));
#46008=CARTESIAN_POINT('Ctrl Pts',(-3.44653088665685,-1.,-1.94668377715332));
#46009=CARTESIAN_POINT('Ctrl Pts',(-3.44653088665685,1.,-1.94668377715332));
#46010=CARTESIAN_POINT('Ctrl Pts',(-3.45395731584051,-1.,-1.94812754766524));
#46011=CARTESIAN_POINT('Ctrl Pts',(-3.45395731584051,1.,-1.94812754766524));
#46012=CARTESIAN_POINT('Ctrl Pts',(-3.46139661060959,-1.,-1.94952575850196));
#46013=CARTESIAN_POINT('Ctrl Pts',(-3.46139661060959,1.,-1.94952575850196));
#46014=CARTESIAN_POINT('Ctrl Pts',(-3.4688525897419,-1.,-1.95088147859876));
#46015=CARTESIAN_POINT('Ctrl Pts',(-3.4688525897419,1.,-1.95088147859876));
#46016=CARTESIAN_POINT('Ctrl Pts',(-3.47632820495926,-1.,-1.95219722189878));
#46017=CARTESIAN_POINT('Ctrl Pts',(-3.47632820495926,1.,-1.95219722189878));
#46018=CARTESIAN_POINT('Ctrl Pts',(-3.48382414832648,-1.,-1.95347412486316));
#46019=CARTESIAN_POINT('Ctrl Pts',(-3.48382414832648,1.,-1.95347412486316));
#46020=CARTESIAN_POINT('Ctrl Pts',(-3.49133956289154,-1.,-1.95471236969653));
#46021=CARTESIAN_POINT('Ctrl Pts',(-3.49133956289154,1.,-1.95471236969653));
#46022=CARTESIAN_POINT('Ctrl Pts',(-3.49887263575602,-1.,-1.9559115382367));
#46023=CARTESIAN_POINT('Ctrl Pts',(-3.49887263575602,1.,-1.9559115382367));
#46024=CARTESIAN_POINT('Ctrl Pts',(-3.50642124159913,-1.,-1.95707099606513));
#46025=CARTESIAN_POINT('Ctrl Pts',(-3.50642124159913,1.,-1.95707099606513));
#46026=CARTESIAN_POINT('Ctrl Pts',(-3.51398354617772,-1.,-1.95819025316768));
#46027=CARTESIAN_POINT('Ctrl Pts',(-3.51398354617772,1.,-1.95819025316768));
#46028=CARTESIAN_POINT('Ctrl Pts',(-3.52155867431438,-1.,-1.95926936324436));
#46029=CARTESIAN_POINT('Ctrl Pts',(-3.52155867431438,1.,-1.95926936324436));
#46030=CARTESIAN_POINT('Ctrl Pts',(-3.52914648844289,-1.,-1.96030879411534));
#46031=CARTESIAN_POINT('Ctrl Pts',(-3.52914648844289,1.,-1.96030879411534));
#46032=CARTESIAN_POINT('Ctrl Pts',(-3.53674730625759,-1.,-1.96130926212661));
#46033=CARTESIAN_POINT('Ctrl Pts',(-3.53674730625759,1.,-1.96130926212661));
#46034=CARTESIAN_POINT('Ctrl Pts',(-3.54436163300425,-1.,-1.96227157573058));
#46035=CARTESIAN_POINT('Ctrl Pts',(-3.54436163300425,1.,-1.96227157573058));
#46036=CARTESIAN_POINT('Ctrl Pts',(-3.55198990600929,-1.,-1.96319648628667));
#46037=CARTESIAN_POINT('Ctrl Pts',(-3.55198990600929,1.,-1.96319648628667));
#46038=CARTESIAN_POINT('Ctrl Pts',(-3.55963218706201,-1.,-1.96408450906868));
#46039=CARTESIAN_POINT('Ctrl Pts',(-3.55963218706201,1.,-1.96408450906868));
#46040=CARTESIAN_POINT('Ctrl Pts',(-3.56728820357933,-1.,-1.96493594634643));
#46041=CARTESIAN_POINT('Ctrl Pts',(-3.56728820357933,1.,-1.96493594634643));
#46042=CARTESIAN_POINT('Ctrl Pts',(-3.57495748601088,-1.,-1.96575096652857));
#46043=CARTESIAN_POINT('Ctrl Pts',(-3.57495748601088,1.,-1.96575096652857));
#46044=CARTESIAN_POINT('Ctrl Pts',(-3.58263947663884,-1.,-1.9665296668894));
#46045=CARTESIAN_POINT('Ctrl Pts',(-3.58263947663884,1.,-1.9665296668894));
#46046=CARTESIAN_POINT('Ctrl Pts',(-3.5903336402273,-1.,-1.96727213799507));
#46047=CARTESIAN_POINT('Ctrl Pts',(-3.5903336402273,1.,-1.96727213799507));
#46048=CARTESIAN_POINT('Ctrl Pts',(-3.59803959819725,-1.,-1.96797854118257));
#46049=CARTESIAN_POINT('Ctrl Pts',(-3.59803959819725,1.,-1.96797854118257));
#46050=CARTESIAN_POINT('Ctrl Pts',(-3.60575714017676,-1.,-1.96864911885775));
#46051=CARTESIAN_POINT('Ctrl Pts',(-3.60575714017676,1.,-1.96864911885775));
#46052=CARTESIAN_POINT('Ctrl Pts',(-3.61348615496393,-1.,-1.96928416040712));
#46053=CARTESIAN_POINT('Ctrl Pts',(-3.61348615496393,1.,-1.96928416040712));
#46054=CARTESIAN_POINT('Ctrl Pts',(-3.62122658401722,-1.,-1.96988398129888));
#46055=CARTESIAN_POINT('Ctrl Pts',(-3.62122658401722,1.,-1.96988398129888));
#46056=CARTESIAN_POINT('Ctrl Pts',(-3.62897836973397,-1.,-1.97044889850518));
#46057=CARTESIAN_POINT('Ctrl Pts',(-3.62897836973397,1.,-1.97044889850518));
#46058=CARTESIAN_POINT('Ctrl Pts',(-3.63674139590853,-1.,-1.97097920454698));
#46059=CARTESIAN_POINT('Ctrl Pts',(-3.63674139590853,1.,-1.97097920454698));
#46060=CARTESIAN_POINT('Ctrl Pts',(-3.64451546724221,-1.,-1.97147515441539));
#46061=CARTESIAN_POINT('Ctrl Pts',(-3.64451546724221,1.,-1.97147515441539));
#46062=CARTESIAN_POINT('Ctrl Pts',(-3.65230034717364,-1.,-1.97193697240645));
#46063=CARTESIAN_POINT('Ctrl Pts',(-3.65230034717364,1.,-1.97193697240645));
#46064=CARTESIAN_POINT('Ctrl Pts',(-3.66009578166865,-1.,-1.97236485439317));
#46065=CARTESIAN_POINT('Ctrl Pts',(-3.66009578166865,1.,-1.97236485439317));
#46066=CARTESIAN_POINT('Ctrl Pts',(-3.66790152751984,-1.,-1.9727589719863));
#46067=CARTESIAN_POINT('Ctrl Pts',(-3.66790152751984,1.,-1.9727589719863));
#46068=CARTESIAN_POINT('Ctrl Pts',(-3.67571738106175,-1.,-1.97311947678035));
#46069=CARTESIAN_POINT('Ctrl Pts',(-3.67571738106175,1.,-1.97311947678035));
#46070=CARTESIAN_POINT('Ctrl Pts',(-3.68354319913416,-1.,-1.9734465030363));
#46071=CARTESIAN_POINT('Ctrl Pts',(-3.68354319913416,1.,-1.9734465030363));
#46072=CARTESIAN_POINT('Ctrl Pts',(-3.69137888597855,-1.,-1.97374016224397));
#46073=CARTESIAN_POINT('Ctrl Pts',(-3.69137888597855,1.,-1.97374016224397));
#46074=CARTESIAN_POINT('Ctrl Pts',(-3.69765528558292,-1.,-1.97394846382288));
#46075=CARTESIAN_POINT('Ctrl Pts',(-3.69765528558292,1.,-1.97394846382288));
#46076=CARTESIAN_POINT('Ctrl Pts',(-3.70236698911837,-1.,-1.97408973726149));
#46077=CARTESIAN_POINT('Ctrl Pts',(-3.70236698911837,1.,-1.97408973726149));
#46078=CARTESIAN_POINT('Ctrl Pts',(-3.7055100813194,-1.,-1.974177276451));
#46079=CARTESIAN_POINT('Ctrl Pts',(-3.7055100813194,1.,-1.974177276451));
#46080=CARTESIAN_POINT('Ctrl Pts',(-3.70708211654725,-1.,-1.97421938526992));
#46081=CARTESIAN_POINT('Ctrl Pts',(-3.70708211654725,1.,-1.97421938526992));
#46082=CARTESIAN_POINT('',(-3.24413672884902,1.,-1.88097764062542));
#46083=CARTESIAN_POINT('Ctrl Pts',(-3.24413672884902,-1.,-1.88097764062542));
#46084=CARTESIAN_POINT('Ctrl Pts',(-3.24413672884902,-0.666666666666667,
-1.88097764062542));
#46085=CARTESIAN_POINT('Ctrl Pts',(-3.24413672884902,-0.333333333333333,
-1.88097764062542));
#46086=CARTESIAN_POINT('Ctrl Pts',(-3.24413672884902,0.333333333333333,
-1.88097764062542));
#46087=CARTESIAN_POINT('Ctrl Pts',(-3.24413672884902,0.666666666666667,
-1.88097764062542));
#46088=CARTESIAN_POINT('Ctrl Pts',(-3.24413672884902,1.,-1.88097764062542));
#46089=CARTESIAN_POINT('',(-3.70708211654725,1.,-1.97421938526992));
#46090=CARTESIAN_POINT('',(-3.70708211654725,0.,-1.97421938526992));
#46091=CARTESIAN_POINT('Ctrl Pts',(-3.24413672884902,1.,-1.88097764062542));
#46092=CARTESIAN_POINT('Ctrl Pts',(-3.24415531671311,1.,-1.88102292397987));
#46093=CARTESIAN_POINT('Ctrl Pts',(-3.24428080352952,1.,-1.88117508446657));
#46094=CARTESIAN_POINT('Ctrl Pts',(-3.24480754675942,1.,-1.88156537699118));
#46095=CARTESIAN_POINT('Ctrl Pts',(-3.24625654410705,1.,-1.88242596600422));
#46096=CARTESIAN_POINT('Ctrl Pts',(-3.24935200512055,1.,-1.88407708646435));
#46097=CARTESIAN_POINT('Ctrl Pts',(-3.25408686339298,1.,-1.88646802523372));
#46098=CARTESIAN_POINT('Ctrl Pts',(-3.2599988519361,1.,-1.88934996203508));
#46099=CARTESIAN_POINT('Ctrl Pts',(-3.2667765388833,1.,-1.89255393500769));
#46100=CARTESIAN_POINT('Ctrl Pts',(-3.27407108932908,1.,-1.89589172903662));
#46101=CARTESIAN_POINT('Ctrl Pts',(-3.28154737912287,1.,-1.89918429230424));
#46102=CARTESIAN_POINT('Ctrl Pts',(-3.28893448600364,1.,-1.9022897124757));
#46103=CARTESIAN_POINT('Ctrl Pts',(-3.29608978722258,1.,-1.9051389186417));
#46104=CARTESIAN_POINT('Ctrl Pts',(-3.30300595568341,1.,-1.90773912171424));
#46105=CARTESIAN_POINT('Ctrl Pts',(-3.30975721158694,1.,-1.91014297830502));
#46106=CARTESIAN_POINT('Ctrl Pts',(-3.31646052426395,1.,-1.91242616234459));
#46107=CARTESIAN_POINT('Ctrl Pts',(-3.32323403454507,1.,-1.91466343916612));
#46108=CARTESIAN_POINT('Ctrl Pts',(-3.33014884257812,1.,-1.91690081930297));
#46109=CARTESIAN_POINT('Ctrl Pts',(-3.33721230709948,1.,-1.91914609610173));
#46110=CARTESIAN_POINT('Ctrl Pts',(-3.34439448941915,1.,-1.92138450828378));
#46111=CARTESIAN_POINT('Ctrl Pts',(-3.35164424847206,1.,-1.92358838440518));
#46112=CARTESIAN_POINT('Ctrl Pts',(-3.35890824422976,1.,-1.92572846125763));
#46113=CARTESIAN_POINT('Ctrl Pts',(-3.36615168657597,1.,-1.92778626543803));
#46114=CARTESIAN_POINT('Ctrl Pts',(-3.37336807068078,1.,-1.92975993109897));
#46115=CARTESIAN_POINT('Ctrl Pts',(-3.38056768525577,1.,-1.93165739093292));
#46116=CARTESIAN_POINT('Ctrl Pts',(-3.38777076883267,1.,-1.93349233176794));
#46117=CARTESIAN_POINT('Ctrl Pts',(-3.39499923640789,1.,-1.93527929945982));
#46118=CARTESIAN_POINT('Ctrl Pts',(-3.40226802104093,1.,-1.93702857723089));
#46119=CARTESIAN_POINT('Ctrl Pts',(-3.40957978266622,1.,-1.93874306008132));
#46120=CARTESIAN_POINT('Ctrl Pts',(-3.41692971994082,1.,-1.94042111965237));
#46121=CARTESIAN_POINT('Ctrl Pts',(-3.42430850941497,1.,-1.94205835913692));
#46122=CARTESIAN_POINT('Ctrl Pts',(-3.43170586602436,1.,-1.94364973660285));
#46123=CARTESIAN_POINT('Ctrl Pts',(-3.43911410197693,1.,-1.94519168842883));
#46124=CARTESIAN_POINT('Ctrl Pts',(-3.44653088665685,1.,-1.94668377715332));
#46125=CARTESIAN_POINT('Ctrl Pts',(-3.45395731584051,1.,-1.94812754766524));
#46126=CARTESIAN_POINT('Ctrl Pts',(-3.46139661060959,1.,-1.94952575850196));
#46127=CARTESIAN_POINT('Ctrl Pts',(-3.4688525897419,1.,-1.95088147859876));
#46128=CARTESIAN_POINT('Ctrl Pts',(-3.47632820495926,1.,-1.95219722189878));
#46129=CARTESIAN_POINT('Ctrl Pts',(-3.48382414832648,1.,-1.95347412486316));
#46130=CARTESIAN_POINT('Ctrl Pts',(-3.49133956289154,1.,-1.95471236969653));
#46131=CARTESIAN_POINT('Ctrl Pts',(-3.49887263575602,1.,-1.9559115382367));
#46132=CARTESIAN_POINT('Ctrl Pts',(-3.50642124159913,1.,-1.95707099606513));
#46133=CARTESIAN_POINT('Ctrl Pts',(-3.51398354617772,1.,-1.95819025316768));
#46134=CARTESIAN_POINT('Ctrl Pts',(-3.52155867431438,1.,-1.95926936324436));
#46135=CARTESIAN_POINT('Ctrl Pts',(-3.52914648844289,1.,-1.96030879411534));
#46136=CARTESIAN_POINT('Ctrl Pts',(-3.53674730625759,1.,-1.96130926212661));
#46137=CARTESIAN_POINT('Ctrl Pts',(-3.54436163300425,1.,-1.96227157573058));
#46138=CARTESIAN_POINT('Ctrl Pts',(-3.55198990600929,1.,-1.96319648628667));
#46139=CARTESIAN_POINT('Ctrl Pts',(-3.55963218706201,1.,-1.96408450906868));
#46140=CARTESIAN_POINT('Ctrl Pts',(-3.56728820357933,1.,-1.96493594634643));
#46141=CARTESIAN_POINT('Ctrl Pts',(-3.57495748601088,1.,-1.96575096652857));
#46142=CARTESIAN_POINT('Ctrl Pts',(-3.58263947663884,1.,-1.9665296668894));
#46143=CARTESIAN_POINT('Ctrl Pts',(-3.5903336402273,1.,-1.96727213799507));
#46144=CARTESIAN_POINT('Ctrl Pts',(-3.59803959819725,1.,-1.96797854118257));
#46145=CARTESIAN_POINT('Ctrl Pts',(-3.60575714017676,1.,-1.96864911885775));
#46146=CARTESIAN_POINT('Ctrl Pts',(-3.61348615496393,1.,-1.96928416040712));
#46147=CARTESIAN_POINT('Ctrl Pts',(-3.62122658401722,1.,-1.96988398129888));
#46148=CARTESIAN_POINT('Ctrl Pts',(-3.62897836973397,1.,-1.97044889850518));
#46149=CARTESIAN_POINT('Ctrl Pts',(-3.63674139590853,1.,-1.97097920454698));
#46150=CARTESIAN_POINT('Ctrl Pts',(-3.64451546724221,1.,-1.97147515441539));
#46151=CARTESIAN_POINT('Ctrl Pts',(-3.65230034717364,1.,-1.97193697240645));
#46152=CARTESIAN_POINT('Ctrl Pts',(-3.66009578166865,1.,-1.97236485439317));
#46153=CARTESIAN_POINT('Ctrl Pts',(-3.66790152751984,1.,-1.9727589719863));
#46154=CARTESIAN_POINT('Ctrl Pts',(-3.67571738106175,1.,-1.97311947678035));
#46155=CARTESIAN_POINT('Ctrl Pts',(-3.68354319913416,1.,-1.9734465030363));
#46156=CARTESIAN_POINT('Ctrl Pts',(-3.69137888597855,1.,-1.97374016224397));
#46157=CARTESIAN_POINT('Ctrl Pts',(-3.69765528558292,1.,-1.97394846382288));
#46158=CARTESIAN_POINT('Ctrl Pts',(-3.70236698911837,1.,-1.97408973726149));
#46159=CARTESIAN_POINT('Ctrl Pts',(-3.7055100813194,1.,-1.974177276451));
#46160=CARTESIAN_POINT('Ctrl Pts',(-3.70708211654725,1.,-1.97421938526992));
#46161=CARTESIAN_POINT('Origin',(-3.70708211654725,0.,-1.97421938526992));
#46162=CARTESIAN_POINT('',(-3.77614523045147,1.,-1.83867539237861));
#46163=CARTESIAN_POINT('Origin',(0.,0.,0.));
#46164=CARTESIAN_POINT('',(-3.14877060440425,1.,-2.03660101169564));
#46165=CARTESIAN_POINT('Origin',(0.,1.,0.));
#46166=CARTESIAN_POINT('Ctrl Pts',(-3.14877060440425,1.,-2.03660101169564));
#46167=CARTESIAN_POINT('Ctrl Pts',(-3.14877060440425,0.666666666666667,
-2.03660101169564));
#46168=CARTESIAN_POINT('Ctrl Pts',(-3.14877060440425,0.333333333333333,
-2.03660101169564));
#46169=CARTESIAN_POINT('Ctrl Pts',(-3.14877060440425,-0.333333333333333,
-2.03660101169564));
#46170=CARTESIAN_POINT('Ctrl Pts',(-3.14877060440425,-0.666666666666667,
-2.03660101169564));
#46171=CARTESIAN_POINT('Ctrl Pts',(-3.14877060440425,-1.,-2.03660101169564));
#46172=CARTESIAN_POINT('Ctrl Pts',(-3.44202241512147,-1.,-2.40675750623143));
#46173=CARTESIAN_POINT('Ctrl Pts',(-3.44202241512147,1.,-2.40675750623143));
#46174=CARTESIAN_POINT('Ctrl Pts',(-3.44127120683402,-1.,-2.40537592959345));
#46175=CARTESIAN_POINT('Ctrl Pts',(-3.44127120683402,1.,-2.40537592959345));
#46176=CARTESIAN_POINT('Ctrl Pts',(-3.43976627485223,-1.,-2.40261515590099));
#46177=CARTESIAN_POINT('Ctrl Pts',(-3.43976627485223,1.,-2.40261515590099));
#46178=CARTESIAN_POINT('Ctrl Pts',(-3.43750133066036,-1.,-2.39848113411429));
#46179=CARTESIAN_POINT('Ctrl Pts',(-3.43750133066036,1.,-2.39848113411429));
#46180=CARTESIAN_POINT('Ctrl Pts',(-3.43446630680436,-1.,-2.39298338805823));
#46181=CARTESIAN_POINT('Ctrl Pts',(-3.43446630680436,1.,-2.39298338805823));
#46182=CARTESIAN_POINT('Ctrl Pts',(-3.43064732714472,-1.,-2.38613505844641));
#46183=CARTESIAN_POINT('Ctrl Pts',(-3.43064732714472,1.,-2.38613505844641));
#46184=CARTESIAN_POINT('Ctrl Pts',(-3.42680309755241,-1.,-2.37931067029517));
#46185=CARTESIAN_POINT('Ctrl Pts',(-3.42680309755241,1.,-2.37931067029517));
#46186=CARTESIAN_POINT('Ctrl Pts',(-3.42293356216595,-1.,-2.37251035954351));
#46187=CARTESIAN_POINT('Ctrl Pts',(-3.42293356216595,1.,-2.37251035954351));
#46188=CARTESIAN_POINT('Ctrl Pts',(-3.41903866635384,-1.,-2.36573431470314));
#46189=CARTESIAN_POINT('Ctrl Pts',(-3.41903866635384,1.,-2.36573431470314));
#46190=CARTESIAN_POINT('Ctrl Pts',(-3.4151183675076,-1.,-2.35898278606449));
#46191=CARTESIAN_POINT('Ctrl Pts',(-3.4151183675076,1.,-2.35898278606449));
#46192=CARTESIAN_POINT('Ctrl Pts',(-3.41117262313464,-1.,-2.35225606823649));
#46193=CARTESIAN_POINT('Ctrl Pts',(-3.41117262313464,1.,-2.35225606823649));
#46194=CARTESIAN_POINT('Ctrl Pts',(-3.40720137403888,-1.,-2.34555447648901));
#46195=CARTESIAN_POINT('Ctrl Pts',(-3.40720137403888,1.,-2.34555447648901));
#46196=CARTESIAN_POINT('Ctrl Pts',(-3.40320452776646,-1.,-2.33887832342715));
#46197=CARTESIAN_POINT('Ctrl Pts',(-3.40320452776646,1.,-2.33887832342715));
#46198=CARTESIAN_POINT('Ctrl Pts',(-3.39918194578115,-1.,-2.33222789882601));
#46199=CARTESIAN_POINT('Ctrl Pts',(-3.39918194578115,1.,-2.33222789882601));
#46200=CARTESIAN_POINT('Ctrl Pts',(-3.39513342020045,-1.,-2.32560343902683));
#46201=CARTESIAN_POINT('Ctrl Pts',(-3.39513342020045,1.,-2.32560343902683));
#46202=CARTESIAN_POINT('Ctrl Pts',(-3.39105869475112,-1.,-2.31900513925627));
#46203=CARTESIAN_POINT('Ctrl Pts',(-3.39105869475112,1.,-2.31900513925627));
#46204=CARTESIAN_POINT('Ctrl Pts',(-3.38695751492659,-1.,-2.31243319489505));
#46205=CARTESIAN_POINT('Ctrl Pts',(-3.38695751492659,1.,-2.31243319489505));
#46206=CARTESIAN_POINT('Ctrl Pts',(-3.38282967336676,-1.,-2.30588783640389));
#46207=CARTESIAN_POINT('Ctrl Pts',(-3.38282967336676,1.,-2.30588783640389));
#46208=CARTESIAN_POINT('Ctrl Pts',(-3.37867504959382,-1.,-2.29936936127588));
#46209=CARTESIAN_POINT('Ctrl Pts',(-3.37867504959382,1.,-2.29936936127588));
#46210=CARTESIAN_POINT('Ctrl Pts',(-3.37449367172707,-1.,-2.2928781800731));
#46211=CARTESIAN_POINT('Ctrl Pts',(-3.37449367172707,1.,-2.2928781800731));
#46212=CARTESIAN_POINT('Ctrl Pts',(-3.37028570206357,-1.,-2.28641481081045));
#46213=CARTESIAN_POINT('Ctrl Pts',(-3.37028570206357,1.,-2.28641481081045));
#46214=CARTESIAN_POINT('Ctrl Pts',(-3.36605130712978,-1.,-2.27997979457968));
#46215=CARTESIAN_POINT('Ctrl Pts',(-3.36605130712978,1.,-2.27997979457968));
#46216=CARTESIAN_POINT('Ctrl Pts',(-3.36179055004369,-1.,-2.27357362620902));
#46217=CARTESIAN_POINT('Ctrl Pts',(-3.36179055004369,1.,-2.27357362620902));
#46218=CARTESIAN_POINT('Ctrl Pts',(-3.35750328523077,-1.,-2.26719668579921));
#46219=CARTESIAN_POINT('Ctrl Pts',(-3.35750328523077,1.,-2.26719668579921));
#46220=CARTESIAN_POINT('Ctrl Pts',(-3.35318902552676,-1.,-2.26084915222484));
#46221=CARTESIAN_POINT('Ctrl Pts',(-3.35318902552676,1.,-2.26084915222484));
#46222=CARTESIAN_POINT('Ctrl Pts',(-3.34884690292342,-1.,-2.25453097693524));
#46223=CARTESIAN_POINT('Ctrl Pts',(-3.34884690292342,1.,-2.25453097693524));
#46224=CARTESIAN_POINT('Ctrl Pts',(-3.34447596770768,-1.,-2.24824207678288));
#46225=CARTESIAN_POINT('Ctrl Pts',(-3.34447596770768,1.,-2.24824207678288));
#46226=CARTESIAN_POINT('Ctrl Pts',(-3.34007543738044,-1.,-2.24198249391437));
#46227=CARTESIAN_POINT('Ctrl Pts',(-3.34007543738044,1.,-2.24198249391437));
#46228=CARTESIAN_POINT('Ctrl Pts',(-3.33564495756478,-1.,-2.2357525632881));
#46229=CARTESIAN_POINT('Ctrl Pts',(-3.33564495756478,1.,-2.2357525632881));
#46230=CARTESIAN_POINT('Ctrl Pts',(-3.33118487773593,-1.,-2.22955308907221));
#46231=CARTESIAN_POINT('Ctrl Pts',(-3.33118487773593,1.,-2.22955308907221));
#46232=CARTESIAN_POINT('Ctrl Pts',(-3.32669646722871,-1.,-2.22338548312758));
#46233=CARTESIAN_POINT('Ctrl Pts',(-3.32669646722871,1.,-2.22338548312758));
#46234=CARTESIAN_POINT('Ctrl Pts',(-3.32218125618955,-1.,-2.21725135110889));
#46235=CARTESIAN_POINT('Ctrl Pts',(-3.32218125618955,1.,-2.21725135110889));
#46236=CARTESIAN_POINT('Ctrl Pts',(-3.31764044024231,-1.,-2.21115211847872));
#46237=CARTESIAN_POINT('Ctrl Pts',(-3.31764044024231,1.,-2.21115211847872));
#46238=CARTESIAN_POINT('Ctrl Pts',(-3.3130742460895,-1.,-2.20508863150608));
#46239=CARTESIAN_POINT('Ctrl Pts',(-3.3130742460895,1.,-2.20508863150608));
#46240=CARTESIAN_POINT('Ctrl Pts',(-3.30848134694596,-1.,-2.19906078949924));
#46241=CARTESIAN_POINT('Ctrl Pts',(-3.30848134694596,1.,-2.19906078949924));
#46242=CARTESIAN_POINT('Ctrl Pts',(-3.30385816281831,-1.,-2.19306710376112));
#46243=CARTESIAN_POINT('Ctrl Pts',(-3.30385816281831,1.,-2.19306710376112));
#46244=CARTESIAN_POINT('Ctrl Pts',(-3.29920022557635,-1.,-2.18710556500325));
#46245=CARTESIAN_POINT('Ctrl Pts',(-3.29920022557635,1.,-2.18710556500325));
#46246=CARTESIAN_POINT('Ctrl Pts',(-3.29450361500484,-1.,-2.18117455557062));
#46247=CARTESIAN_POINT('Ctrl Pts',(-3.29450361500484,1.,-2.18117455557062));
#46248=CARTESIAN_POINT('Ctrl Pts',(-3.28976645712566,-1.,-2.17527380048422));
#46249=CARTESIAN_POINT('Ctrl Pts',(-3.28976645712566,1.,-2.17527380048422));
#46250=CARTESIAN_POINT('Ctrl Pts',(-3.2849901997973,-1.,-2.16940517773459));
#46251=CARTESIAN_POINT('Ctrl Pts',(-3.2849901997973,1.,-2.16940517773459));
#46252=CARTESIAN_POINT('Ctrl Pts',(-3.28018150841414,-1.,-2.16357391934434));
#46253=CARTESIAN_POINT('Ctrl Pts',(-3.28018150841414,1.,-2.16357391934434));
#46254=CARTESIAN_POINT('Ctrl Pts',(-3.27534954469206,-1.,-2.15778690038359));
#46255=CARTESIAN_POINT('Ctrl Pts',(-3.27534954469206,1.,-2.15778690038359));
#46256=CARTESIAN_POINT('Ctrl Pts',(-3.27050245897244,-1.,-2.15205043199818));
#46257=CARTESIAN_POINT('Ctrl Pts',(-3.27050245897244,1.,-2.15205043199818));
#46258=CARTESIAN_POINT('Ctrl Pts',(-3.26564388189764,-1.,-2.14636805295663));
#46259=CARTESIAN_POINT('Ctrl Pts',(-3.26564388189764,1.,-2.14636805295663));
#46260=CARTESIAN_POINT('Ctrl Pts',(-3.26077002641868,-1.,-2.14073870754257));
#46261=CARTESIAN_POINT('Ctrl Pts',(-3.26077002641868,1.,-2.14073870754257));
#46262=CARTESIAN_POINT('Ctrl Pts',(-3.25586495065027,-1.,-2.13515375878786));
#46263=CARTESIAN_POINT('Ctrl Pts',(-3.25586495065027,1.,-2.13515375878786));
#46264=CARTESIAN_POINT('Ctrl Pts',(-3.25090574493994,-1.,-2.1296002839681));
#46265=CARTESIAN_POINT('Ctrl Pts',(-3.25090574493994,1.,-2.1296002839681));
#46266=CARTESIAN_POINT('Ctrl Pts',(-3.24587102613347,-1.,-2.12406646410943));
#46267=CARTESIAN_POINT('Ctrl Pts',(-3.24587102613347,1.,-2.12406646410943));
#46268=CARTESIAN_POINT('Ctrl Pts',(-3.24074905517282,-1.,-2.11854673326972));
#46269=CARTESIAN_POINT('Ctrl Pts',(-3.24074905517282,1.,-2.11854673326972));
#46270=CARTESIAN_POINT('Ctrl Pts',(-3.23554444767115,-1.,-2.11304604021784));
#46271=CARTESIAN_POINT('Ctrl Pts',(-3.23554444767115,1.,-2.11304604021784));
#46272=CARTESIAN_POINT('Ctrl Pts',(-3.23028945793334,-1.,-2.1075869964248));
#46273=CARTESIAN_POINT('Ctrl Pts',(-3.23028945793334,1.,-2.1075869964248));
#46274=CARTESIAN_POINT('Ctrl Pts',(-3.22503437553496,-1.,-2.10220384298533));
#46275=CARTESIAN_POINT('Ctrl Pts',(-3.22503437553496,1.,-2.10220384298533));
#46276=CARTESIAN_POINT('Ctrl Pts',(-3.21982707347067,-1.,-2.09692958434933));
#46277=CARTESIAN_POINT('Ctrl Pts',(-3.21982707347067,1.,-2.09692958434933));
#46278=CARTESIAN_POINT('Ctrl Pts',(-3.2146942960168,-1.,-2.0917841946046));
#46279=CARTESIAN_POINT('Ctrl Pts',(-3.2146942960168,1.,-2.0917841946046));
#46280=CARTESIAN_POINT('Ctrl Pts',(-3.20962575845433,-1.,-2.08676465517435));
#46281=CARTESIAN_POINT('Ctrl Pts',(-3.20962575845433,1.,-2.08676465517435));
#46282=CARTESIAN_POINT('Ctrl Pts',(-3.20454818630635,-1.,-2.08182850370816));
#46283=CARTESIAN_POINT('Ctrl Pts',(-3.20454818630635,1.,-2.08182850370816));
#46284=CARTESIAN_POINT('Ctrl Pts',(-3.19934132835879,-1.,-2.0769044187063));
#46285=CARTESIAN_POINT('Ctrl Pts',(-3.19934132835879,1.,-2.0769044187063));
#46286=CARTESIAN_POINT('Ctrl Pts',(-3.19388465568113,-1.,-2.07192253497765));
#46287=CARTESIAN_POINT('Ctrl Pts',(-3.19388465568113,1.,-2.07192253497765));
#46288=CARTESIAN_POINT('Ctrl Pts',(-3.18809755562297,-1.,-2.06684062744065));
#46289=CARTESIAN_POINT('Ctrl Pts',(-3.18809755562297,1.,-2.06684062744065));
#46290=CARTESIAN_POINT('Ctrl Pts',(-3.18197692964677,-1.,-2.06166849827143));
#46291=CARTESIAN_POINT('Ctrl Pts',(-3.18197692964677,1.,-2.06166849827143));
#46292=CARTESIAN_POINT('Ctrl Pts',(-3.17564906975592,-1.,-2.05650186773279));
#46293=CARTESIAN_POINT('Ctrl Pts',(-3.17564906975592,1.,-2.05650186773279));
#46294=CARTESIAN_POINT('Ctrl Pts',(-3.16936341689859,-1.,-2.05151770247452));
#46295=CARTESIAN_POINT('Ctrl Pts',(-3.16936341689859,1.,-2.05151770247452));
#46296=CARTESIAN_POINT('Ctrl Pts',(-3.16343165059235,-1.,-2.0469333124766));
#46297=CARTESIAN_POINT('Ctrl Pts',(-3.16343165059235,1.,-2.0469333124766));
#46298=CARTESIAN_POINT('Ctrl Pts',(-3.15817983946525,-1.,-2.04297406404132));
#46299=CARTESIAN_POINT('Ctrl Pts',(-3.15817983946525,1.,-2.04297406404132));
#46300=CARTESIAN_POINT('Ctrl Pts',(-3.1538999167466,-1.,-2.03984073791432));
#46301=CARTESIAN_POINT('Ctrl Pts',(-3.1538999167466,1.,-2.03984073791432));
#46302=CARTESIAN_POINT('Ctrl Pts',(-3.15079010635326,-1.,-2.03766932526171));
#46303=CARTESIAN_POINT('Ctrl Pts',(-3.15079010635326,1.,-2.03766932526171));
#46304=CARTESIAN_POINT('Ctrl Pts',(-3.14931281967585,-1.,-2.03675273048882));
#46305=CARTESIAN_POINT('Ctrl Pts',(-3.14931281967585,1.,-2.03675273048882));
#46306=CARTESIAN_POINT('Ctrl Pts',(-3.14878756590499,-1.,-2.03653654935384));
#46307=CARTESIAN_POINT('Ctrl Pts',(-3.14878756590499,1.,-2.03653654935384));
#46308=CARTESIAN_POINT('Ctrl Pts',(-3.14869618937138,-1.,-2.036601737578));
#46309=CARTESIAN_POINT('Ctrl Pts',(-3.14869618937138,1.,-2.036601737578));
#46310=CARTESIAN_POINT('Ctrl Pts',(-3.1487152044751,-1.,-2.03668666247593));
#46311=CARTESIAN_POINT('Ctrl Pts',(-3.1487152044751,1.,-2.03668666247593));
#46312=CARTESIAN_POINT('',(-3.44202241512147,1.,-2.40675750623143));
#46313=CARTESIAN_POINT('Ctrl Pts',(-3.44202241512147,1.,-2.40675750623143));
#46314=CARTESIAN_POINT('Ctrl Pts',(-3.44127120683402,1.,-2.40537592959345));
#46315=CARTESIAN_POINT('Ctrl Pts',(-3.43976627485223,1.,-2.40261515590099));
#46316=CARTESIAN_POINT('Ctrl Pts',(-3.43750133066036,1.,-2.39848113411429));
#46317=CARTESIAN_POINT('Ctrl Pts',(-3.43446630680436,1.,-2.39298338805823));
#46318=CARTESIAN_POINT('Ctrl Pts',(-3.43064732714472,1.,-2.38613505844641));
#46319=CARTESIAN_POINT('Ctrl Pts',(-3.42680309755241,1.,-2.37931067029517));
#46320=CARTESIAN_POINT('Ctrl Pts',(-3.42293356216595,1.,-2.37251035954351));
#46321=CARTESIAN_POINT('Ctrl Pts',(-3.41903866635384,1.,-2.36573431470314));
#46322=CARTESIAN_POINT('Ctrl Pts',(-3.4151183675076,1.,-2.35898278606449));
#46323=CARTESIAN_POINT('Ctrl Pts',(-3.41117262313464,1.,-2.35225606823649));
#46324=CARTESIAN_POINT('Ctrl Pts',(-3.40720137403888,1.,-2.34555447648901));
#46325=CARTESIAN_POINT('Ctrl Pts',(-3.40320452776646,1.,-2.33887832342715));
#46326=CARTESIAN_POINT('Ctrl Pts',(-3.39918194578115,1.,-2.33222789882601));
#46327=CARTESIAN_POINT('Ctrl Pts',(-3.39513342020045,1.,-2.32560343902683));
#46328=CARTESIAN_POINT('Ctrl Pts',(-3.39105869475112,1.,-2.31900513925627));
#46329=CARTESIAN_POINT('Ctrl Pts',(-3.38695751492659,1.,-2.31243319489505));
#46330=CARTESIAN_POINT('Ctrl Pts',(-3.38282967336676,1.,-2.30588783640389));
#46331=CARTESIAN_POINT('Ctrl Pts',(-3.37867504959382,1.,-2.29936936127588));
#46332=CARTESIAN_POINT('Ctrl Pts',(-3.37449367172707,1.,-2.2928781800731));
#46333=CARTESIAN_POINT('Ctrl Pts',(-3.37028570206357,1.,-2.28641481081045));
#46334=CARTESIAN_POINT('Ctrl Pts',(-3.36605130712978,1.,-2.27997979457968));
#46335=CARTESIAN_POINT('Ctrl Pts',(-3.36179055004369,1.,-2.27357362620902));
#46336=CARTESIAN_POINT('Ctrl Pts',(-3.35750328523077,1.,-2.26719668579921));
#46337=CARTESIAN_POINT('Ctrl Pts',(-3.35318902552676,1.,-2.26084915222484));
#46338=CARTESIAN_POINT('Ctrl Pts',(-3.34884690292342,1.,-2.25453097693524));
#46339=CARTESIAN_POINT('Ctrl Pts',(-3.34447596770768,1.,-2.24824207678288));
#46340=CARTESIAN_POINT('Ctrl Pts',(-3.34007543738044,1.,-2.24198249391437));
#46341=CARTESIAN_POINT('Ctrl Pts',(-3.33564495756478,1.,-2.2357525632881));
#46342=CARTESIAN_POINT('Ctrl Pts',(-3.33118487773593,1.,-2.22955308907221));
#46343=CARTESIAN_POINT('Ctrl Pts',(-3.32669646722871,1.,-2.22338548312758));
#46344=CARTESIAN_POINT('Ctrl Pts',(-3.32218125618955,1.,-2.21725135110889));
#46345=CARTESIAN_POINT('Ctrl Pts',(-3.31764044024231,1.,-2.21115211847872));
#46346=CARTESIAN_POINT('Ctrl Pts',(-3.3130742460895,1.,-2.20508863150608));
#46347=CARTESIAN_POINT('Ctrl Pts',(-3.30848134694596,1.,-2.19906078949924));
#46348=CARTESIAN_POINT('Ctrl Pts',(-3.30385816281831,1.,-2.19306710376112));
#46349=CARTESIAN_POINT('Ctrl Pts',(-3.29920022557635,1.,-2.18710556500325));
#46350=CARTESIAN_POINT('Ctrl Pts',(-3.29450361500484,1.,-2.18117455557062));
#46351=CARTESIAN_POINT('Ctrl Pts',(-3.28976645712566,1.,-2.17527380048422));
#46352=CARTESIAN_POINT('Ctrl Pts',(-3.2849901997973,1.,-2.16940517773459));
#46353=CARTESIAN_POINT('Ctrl Pts',(-3.28018150841414,1.,-2.16357391934434));
#46354=CARTESIAN_POINT('Ctrl Pts',(-3.27534954469206,1.,-2.15778690038359));
#46355=CARTESIAN_POINT('Ctrl Pts',(-3.27050245897244,1.,-2.15205043199818));
#46356=CARTESIAN_POINT('Ctrl Pts',(-3.26564388189764,1.,-2.14636805295663));
#46357=CARTESIAN_POINT('Ctrl Pts',(-3.26077002641868,1.,-2.14073870754257));
#46358=CARTESIAN_POINT('Ctrl Pts',(-3.25586495065027,1.,-2.13515375878786));
#46359=CARTESIAN_POINT('Ctrl Pts',(-3.25090574493994,1.,-2.1296002839681));
#46360=CARTESIAN_POINT('Ctrl Pts',(-3.24587102613347,1.,-2.12406646410943));
#46361=CARTESIAN_POINT('Ctrl Pts',(-3.24074905517282,1.,-2.11854673326972));
#46362=CARTESIAN_POINT('Ctrl Pts',(-3.23554444767115,1.,-2.11304604021784));
#46363=CARTESIAN_POINT('Ctrl Pts',(-3.23028945793334,1.,-2.1075869964248));
#46364=CARTESIAN_POINT('Ctrl Pts',(-3.22503437553496,1.,-2.10220384298533));
#46365=CARTESIAN_POINT('Ctrl Pts',(-3.21982707347067,1.,-2.09692958434933));
#46366=CARTESIAN_POINT('Ctrl Pts',(-3.2146942960168,1.,-2.0917841946046));
#46367=CARTESIAN_POINT('Ctrl Pts',(-3.20962575845433,1.,-2.08676465517435));
#46368=CARTESIAN_POINT('Ctrl Pts',(-3.20454818630635,1.,-2.08182850370816));
#46369=CARTESIAN_POINT('Ctrl Pts',(-3.19934132835879,1.,-2.0769044187063));
#46370=CARTESIAN_POINT('Ctrl Pts',(-3.19388465568113,1.,-2.07192253497765));
#46371=CARTESIAN_POINT('Ctrl Pts',(-3.18809755562297,1.,-2.06684062744065));
#46372=CARTESIAN_POINT('Ctrl Pts',(-3.18197692964677,1.,-2.06166849827143));
#46373=CARTESIAN_POINT('Ctrl Pts',(-3.17564906975592,1.,-2.05650186773279));
#46374=CARTESIAN_POINT('Ctrl Pts',(-3.16936341689859,1.,-2.05151770247452));
#46375=CARTESIAN_POINT('Ctrl Pts',(-3.16343165059235,1.,-2.0469333124766));
#46376=CARTESIAN_POINT('Ctrl Pts',(-3.15817983946525,1.,-2.04297406404132));
#46377=CARTESIAN_POINT('Ctrl Pts',(-3.1538999167466,1.,-2.03984073791432));
#46378=CARTESIAN_POINT('Ctrl Pts',(-3.15102344775396,1.,-2.03783225496023));
#46379=CARTESIAN_POINT('Ctrl Pts',(-3.14959882629936,1.,-2.03693188810614));
#46380=CARTESIAN_POINT('Ctrl Pts',(-3.14901193669147,1.,-2.03663974554941));
#46381=CARTESIAN_POINT('Ctrl Pts',(-3.1488193908823,1.,-2.03659701539175));
#46382=CARTESIAN_POINT('Ctrl Pts',(-3.14877060440425,1.,-2.03660101169564));
#46383=CARTESIAN_POINT('',(-3.44202241512147,0.,-2.40675750623143));
#46384=CARTESIAN_POINT('Ctrl Pts',(-2.91001063062876,-1.,-2.36523532225181));
#46385=CARTESIAN_POINT('Ctrl Pts',(-2.91001063062876,1.,-2.36523532225181));
#46386=CARTESIAN_POINT('Ctrl Pts',(-2.90992398626211,-1.,-2.36524348105112));
#46387=CARTESIAN_POINT('Ctrl Pts',(-2.90992398626211,1.,-2.36524348105112));
#46388=CARTESIAN_POINT('Ctrl Pts',(-2.90989022548032,-1.,-2.36535052956938));
#46389=CARTESIAN_POINT('Ctrl Pts',(-2.90989022548032,1.,-2.36535052956938));
#46390=CARTESIAN_POINT('Ctrl Pts',(-2.91025813830041,-1.,-2.36578327194741));
#46391=CARTESIAN_POINT('Ctrl Pts',(-2.91025813830041,1.,-2.36578327194741));
#46392=CARTESIAN_POINT('Ctrl Pts',(-2.9115863784204,-1.,-2.36690501170627));
#46393=CARTESIAN_POINT('Ctrl Pts',(-2.9115863784204,1.,-2.36690501170627));
#46394=CARTESIAN_POINT('Ctrl Pts',(-2.9146124988314,-1.,-2.36919161373173));
#46395=CARTESIAN_POINT('Ctrl Pts',(-2.9146124988314,1.,-2.36919161373173));
#46396=CARTESIAN_POINT('Ctrl Pts',(-2.91891503791411,-1.,-2.37229381109821));
#46397=CARTESIAN_POINT('Ctrl Pts',(-2.91891503791411,1.,-2.37229381109821));
#46398=CARTESIAN_POINT('Ctrl Pts',(-2.92430340582608,-1.,-2.3760651052403));
#46399=CARTESIAN_POINT('Ctrl Pts',(-2.92430340582608,1.,-2.3760651052403));
#46400=CARTESIAN_POINT('Ctrl Pts',(-2.93049643640206,-1.,-2.38028989582073));
#46401=CARTESIAN_POINT('Ctrl Pts',(-2.93049643640206,1.,-2.38028989582073));
#46402=CARTESIAN_POINT('Ctrl Pts',(-2.93717903280391,-1.,-2.38472771516311));
#46403=CARTESIAN_POINT('Ctrl Pts',(-2.93717903280391,1.,-2.38472771516311));
#46404=CARTESIAN_POINT('Ctrl Pts',(-2.94404820669076,-1.,-2.38914929090759));
#46405=CARTESIAN_POINT('Ctrl Pts',(-2.94404820669076,1.,-2.38914929090759));
#46406=CARTESIAN_POINT('Ctrl Pts',(-2.95085857128439,-1.,-2.39337207631667));
#46407=CARTESIAN_POINT('Ctrl Pts',(-2.95085857128439,1.,-2.39337207631667));
#46408=CARTESIAN_POINT('Ctrl Pts',(-2.95748006482942,-1.,-2.39730553974517));
#46409=CARTESIAN_POINT('Ctrl Pts',(-2.95748006482942,1.,-2.39730553974517));
#46410=CARTESIAN_POINT('Ctrl Pts',(-2.96390432240312,-1.,-2.4009556571164));
#46411=CARTESIAN_POINT('Ctrl Pts',(-2.96390432240312,1.,-2.4009556571164));
#46412=CARTESIAN_POINT('Ctrl Pts',(-2.9701964131236,-1.,-2.40438604734919));
#46413=CARTESIAN_POINT('Ctrl Pts',(-2.9701964131236,1.,-2.40438604734919));
#46414=CARTESIAN_POINT('Ctrl Pts',(-2.97646002822422,-1.,-2.40768975073713));
#46415=CARTESIAN_POINT('Ctrl Pts',(-2.97646002822422,1.,-2.40768975073713));
#46416=CARTESIAN_POINT('Ctrl Pts',(-2.98280015815107,-1.,-2.41095909342571));
#46417=CARTESIAN_POINT('Ctrl Pts',(-2.98280015815107,1.,-2.41095909342571));
#46418=CARTESIAN_POINT('Ctrl Pts',(-2.98927983005796,-1.,-2.41425064199586));
#46419=CARTESIAN_POINT('Ctrl Pts',(-2.98927983005796,1.,-2.41425064199586));
#46420=CARTESIAN_POINT('Ctrl Pts',(-2.99590509293503,-1.,-2.41757324500514));
#46421=CARTESIAN_POINT('Ctrl Pts',(-2.99590509293503,1.,-2.41757324500514));
#46422=CARTESIAN_POINT('Ctrl Pts',(-3.00264868585996,-1.,-2.42090763946779));
#46423=CARTESIAN_POINT('Ctrl Pts',(-3.00264868585996,1.,-2.42090763946779));
#46424=CARTESIAN_POINT('Ctrl Pts',(-3.00946442616658,-1.,-2.42421849439613));
#46425=CARTESIAN_POINT('Ctrl Pts',(-3.00946442616658,1.,-2.42421849439613));
#46426=CARTESIAN_POINT('Ctrl Pts',(-3.01630420830504,-1.,-2.42746856264168));
#46427=CARTESIAN_POINT('Ctrl Pts',(-3.01630420830504,1.,-2.42746856264168));
#46428=CARTESIAN_POINT('Ctrl Pts',(-3.02313656036004,-1.,-2.43063415586637));
#46429=CARTESIAN_POINT('Ctrl Pts',(-3.02313656036004,1.,-2.43063415586637));
#46430=CARTESIAN_POINT('Ctrl Pts',(-3.02995534946978,-1.,-2.43371241361488));
#46431=CARTESIAN_POINT('Ctrl Pts',(-3.02995534946978,1.,-2.43371241361488));
#46432=CARTESIAN_POINT('Ctrl Pts',(-3.03676949672821,-1.,-2.43671278042414));
#46433=CARTESIAN_POINT('Ctrl Pts',(-3.03676949672821,1.,-2.43671278042414));
#46434=CARTESIAN_POINT('Ctrl Pts',(-3.04359685040555,-1.,-2.43965194061857));
#46435=CARTESIAN_POINT('Ctrl Pts',(-3.04359685040555,1.,-2.43965194061857));
#46436=CARTESIAN_POINT('Ctrl Pts',(-3.05045678021504,-1.,-2.44254768923105));
#46437=CARTESIAN_POINT('Ctrl Pts',(-3.05045678021504,1.,-2.44254768923105));
#46438=CARTESIAN_POINT('Ctrl Pts',(-3.05736242671506,-1.,-2.44541251892556));
#46439=CARTESIAN_POINT('Ctrl Pts',(-3.05736242671506,1.,-2.44541251892556));
#46440=CARTESIAN_POINT('Ctrl Pts',(-3.06431596421405,-1.,-2.44824970516544));
#46441=CARTESIAN_POINT('Ctrl Pts',(-3.06431596421405,1.,-2.44824970516544));
#46442=CARTESIAN_POINT('Ctrl Pts',(-3.07131290521297,-1.,-2.45105688854422));
#46443=CARTESIAN_POINT('Ctrl Pts',(-3.07131290521297,1.,-2.45105688854422));
#46444=CARTESIAN_POINT('Ctrl Pts',(-3.07834472886139,-1.,-2.4538282678779));
#46445=CARTESIAN_POINT('Ctrl Pts',(-3.07834472886139,1.,-2.4538282678779));
#46446=CARTESIAN_POINT('Ctrl Pts',(-3.08540206545315,-1.,-2.45655725437039));
#46447=CARTESIAN_POINT('Ctrl Pts',(-3.08540206545315,1.,-2.45655725437039));
#46448=CARTESIAN_POINT('Ctrl Pts',(-3.09247787931887,-1.,-2.4592391256388));
#46449=CARTESIAN_POINT('Ctrl Pts',(-3.09247787931887,1.,-2.4592391256388));
#46450=CARTESIAN_POINT('Ctrl Pts',(-3.09956993697052,-1.,-2.46187308501884));
#46451=CARTESIAN_POINT('Ctrl Pts',(-3.09956993697052,1.,-2.46187308501884));
#46452=CARTESIAN_POINT('Ctrl Pts',(-3.1066790790198,-1.,-2.46446082979646));
#46453=CARTESIAN_POINT('Ctrl Pts',(-3.1066790790198,1.,-2.46446082979646));
#46454=CARTESIAN_POINT('Ctrl Pts',(-3.11380805536122,-1.,-2.46700558843506));
#46455=CARTESIAN_POINT('Ctrl Pts',(-3.11380805536122,1.,-2.46700558843506));
#46456=CARTESIAN_POINT('Ctrl Pts',(-3.12096015766983,-1.,-2.46951098947469));
#46457=CARTESIAN_POINT('Ctrl Pts',(-3.12096015766983,1.,-2.46951098947469));
#46458=CARTESIAN_POINT('Ctrl Pts',(-3.12813790805952,-1.,-2.47197997765871));
#46459=CARTESIAN_POINT('Ctrl Pts',(-3.12813790805952,1.,-2.47197997765871));
#46460=CARTESIAN_POINT('Ctrl Pts',(-3.13534181229295,-1.,-2.47441378371932));
#46461=CARTESIAN_POINT('Ctrl Pts',(-3.13534181229295,1.,-2.47441378371932));
#46462=CARTESIAN_POINT('Ctrl Pts',(-3.1425709954655,-1.,-2.47681245356109));
#46463=CARTESIAN_POINT('Ctrl Pts',(-3.1425709954655,1.,-2.47681245356109));
#46464=CARTESIAN_POINT('Ctrl Pts',(-3.14982373241352,-1.,-2.47917529057029));
#46465=CARTESIAN_POINT('Ctrl Pts',(-3.14982373241352,1.,-2.47917529057029));
#46466=CARTESIAN_POINT('Ctrl Pts',(-3.15709802322739,-1.,-2.48150133566571));
#46467=CARTESIAN_POINT('Ctrl Pts',(-3.15709802322739,1.,-2.48150133566571));
#46468=CARTESIAN_POINT('Ctrl Pts',(-3.16439213290161,-1.,-2.48378981792725));
#46469=CARTESIAN_POINT('Ctrl Pts',(-3.16439213290161,1.,-2.48378981792725));
#46470=CARTESIAN_POINT('Ctrl Pts',(-3.17170518863313,-1.,-2.48604065348587));
#46471=CARTESIAN_POINT('Ctrl Pts',(-3.17170518863313,1.,-2.48604065348587));
#46472=CARTESIAN_POINT('Ctrl Pts',(-3.17903698136622,-1.,-2.48825428288201));
#46473=CARTESIAN_POINT('Ctrl Pts',(-3.17903698136622,1.,-2.48825428288201));
#46474=CARTESIAN_POINT('Ctrl Pts',(-3.18638771282266,-1.,-2.49043146334059));
#46475=CARTESIAN_POINT('Ctrl Pts',(-3.18638771282266,1.,-2.49043146334059));
#46476=CARTESIAN_POINT('Ctrl Pts',(-3.19375775555798,-1.,-2.49257307239848));
#46477=CARTESIAN_POINT('Ctrl Pts',(-3.19375775555798,1.,-2.49257307239848));
#46478=CARTESIAN_POINT('Ctrl Pts',(-3.20114742397588,-1.,-2.49467992057755));
#46479=CARTESIAN_POINT('Ctrl Pts',(-3.20114742397588,1.,-2.49467992057755));
#46480=CARTESIAN_POINT('Ctrl Pts',(-3.20855669849836,-1.,-2.4967525264737));
#46481=CARTESIAN_POINT('Ctrl Pts',(-3.20855669849836,1.,-2.4967525264737));
#46482=CARTESIAN_POINT('Ctrl Pts',(-3.21598526261286,-1.,-2.4987911459939));
#46483=CARTESIAN_POINT('Ctrl Pts',(-3.21598526261286,1.,-2.4987911459939));
#46484=CARTESIAN_POINT('Ctrl Pts',(-3.22343262620503,-1.,-2.50079587201957));
#46485=CARTESIAN_POINT('Ctrl Pts',(-3.22343262620503,1.,-2.50079587201957));
#46486=CARTESIAN_POINT('Ctrl Pts',(-3.23089822320646,-1.,-2.50276671338111));
#46487=CARTESIAN_POINT('Ctrl Pts',(-3.23089822320646,1.,-2.50276671338111));
#46488=CARTESIAN_POINT('Ctrl Pts',(-3.23838151080319,-1.,-2.5047036758003));
#46489=CARTESIAN_POINT('Ctrl Pts',(-3.23838151080319,1.,-2.5047036758003));
#46490=CARTESIAN_POINT('Ctrl Pts',(-3.24588208983849,-1.,-2.506606859405));
#46491=CARTESIAN_POINT('Ctrl Pts',(-3.24588208983849,1.,-2.506606859405));
#46492=CARTESIAN_POINT('Ctrl Pts',(-3.25339971460982,-1.,-2.50847647070723));
#46493=CARTESIAN_POINT('Ctrl Pts',(-3.25339971460982,1.,-2.50847647070723));
#46494=CARTESIAN_POINT('Ctrl Pts',(-3.26093423001434,-1.,-2.51031277813486));
#46495=CARTESIAN_POINT('Ctrl Pts',(-3.26093423001434,1.,-2.51031277813486));
#46496=CARTESIAN_POINT('Ctrl Pts',(-3.26848552888115,-1.,-2.51211608411423));
#46497=CARTESIAN_POINT('Ctrl Pts',(-3.26848552888115,1.,-2.51211608411423));
#46498=CARTESIAN_POINT('Ctrl Pts',(-3.27605350473142,-1.,-2.513886692704));
#46499=CARTESIAN_POINT('Ctrl Pts',(-3.27605350473142,1.,-2.513886692704));
#46500=CARTESIAN_POINT('Ctrl Pts',(-3.28363799702982,-1.,-2.51562487464514));
#46501=CARTESIAN_POINT('Ctrl Pts',(-3.28363799702982,1.,-2.51562487464514));
#46502=CARTESIAN_POINT('Ctrl Pts',(-3.2912387729927,-1.,-2.51733085123797));
#46503=CARTESIAN_POINT('Ctrl Pts',(-3.2912387729927,1.,-2.51733085123797));
#46504=CARTESIAN_POINT('Ctrl Pts',(-3.29885556388352,-1.,-2.51900480701069));
#46505=CARTESIAN_POINT('Ctrl Pts',(-3.29885556388352,1.,-2.51900480701069));
#46506=CARTESIAN_POINT('Ctrl Pts',(-3.30648808815442,-1.,-2.52064689568511));
#46507=CARTESIAN_POINT('Ctrl Pts',(-3.30648808815442,1.,-2.52064689568511));
#46508=CARTESIAN_POINT('Ctrl Pts',(-3.31413607874645,-1.,-2.52225724871313));
#46509=CARTESIAN_POINT('Ctrl Pts',(-3.31413607874645,1.,-2.52225724871313));
#46510=CARTESIAN_POINT('Ctrl Pts',(-3.32179931078699,-1.,-2.5238359839626));
#46511=CARTESIAN_POINT('Ctrl Pts',(-3.32179931078699,1.,-2.5238359839626));
#46512=CARTESIAN_POINT('Ctrl Pts',(-3.32947762187533,-1.,-2.52538321164634));
#46513=CARTESIAN_POINT('Ctrl Pts',(-3.32947762187533,1.,-2.52538321164634));
#46514=CARTESIAN_POINT('Ctrl Pts',(-3.33717089999103,-1.,-2.52689902690158));
#46515=CARTESIAN_POINT('Ctrl Pts',(-3.33717089999103,1.,-2.52689902690158));
#46516=CARTESIAN_POINT('Ctrl Pts',(-3.34333744115511,-1.,-2.52808660915689));
#46517=CARTESIAN_POINT('Ctrl Pts',(-3.34333744115511,1.,-2.52808660915689));
#46518=CARTESIAN_POINT('Ctrl Pts',(-3.34796903576663,-1.,-2.52896321610703));
#46519=CARTESIAN_POINT('Ctrl Pts',(-3.34796903576663,1.,-2.52896321610703));
#46520=CARTESIAN_POINT('Ctrl Pts',(-3.35105973714071,-1.,-2.5295413654909));
#46521=CARTESIAN_POINT('Ctrl Pts',(-3.35105973714071,1.,-2.5295413654909));
#46522=CARTESIAN_POINT('Ctrl Pts',(-3.35260583073571,-1.,-2.52982887637028));
#46523=CARTESIAN_POINT('Ctrl Pts',(-3.35260583073571,1.,-2.52982887637028));
#46524=CARTESIAN_POINT('',(-2.90994629141676,1.,-2.36531447826073));
#46525=CARTESIAN_POINT('Ctrl Pts',(-2.90994629141676,-1.,-2.36531447826074));
#46526=CARTESIAN_POINT('Ctrl Pts',(-2.90994629141676,-0.666666666666667,
-2.36531447826074));
#46527=CARTESIAN_POINT('Ctrl Pts',(-2.90994629141676,-0.333333333333333,
-2.36531447826074));
#46528=CARTESIAN_POINT('Ctrl Pts',(-2.90994629141676,0.333333333333333,
-2.36531447826074));
#46529=CARTESIAN_POINT('Ctrl Pts',(-2.90994629141676,0.666666666666667,
-2.36531447826074));
#46530=CARTESIAN_POINT('Ctrl Pts',(-2.90994629141676,1.,-2.36531447826074));
#46531=CARTESIAN_POINT('',(-3.35260583073571,1.,-2.52982887637028));
#46532=CARTESIAN_POINT('',(-3.35260583073571,0.,-2.52982887637028));
#46533=CARTESIAN_POINT('Ctrl Pts',(-2.90994629141676,1.,-2.36531447826073));
#46534=CARTESIAN_POINT('Ctrl Pts',(-2.90995756655606,1.,-2.36536211188453));
#46535=CARTESIAN_POINT('Ctrl Pts',(-2.91005770527719,1.,-2.36553202948613));
#46536=CARTESIAN_POINT('Ctrl Pts',(-2.91051690822156,1.,-2.36599991765749));
#46537=CARTESIAN_POINT('Ctrl Pts',(-2.91181344022549,1.,-2.36707658451664));
#46538=CARTESIAN_POINT('Ctrl Pts',(-2.9146124988314,1.,-2.36919161373173));
#46539=CARTESIAN_POINT('Ctrl Pts',(-2.91891503791411,1.,-2.37229381109821));
#46540=CARTESIAN_POINT('Ctrl Pts',(-2.92430340582608,1.,-2.3760651052403));
#46541=CARTESIAN_POINT('Ctrl Pts',(-2.93049643640206,1.,-2.38028989582073));
#46542=CARTESIAN_POINT('Ctrl Pts',(-2.93717903280391,1.,-2.38472771516311));
#46543=CARTESIAN_POINT('Ctrl Pts',(-2.94404820669076,1.,-2.38914929090759));
#46544=CARTESIAN_POINT('Ctrl Pts',(-2.95085857128439,1.,-2.39337207631667));
#46545=CARTESIAN_POINT('Ctrl Pts',(-2.95748006482942,1.,-2.39730553974517));
#46546=CARTESIAN_POINT('Ctrl Pts',(-2.96390432240312,1.,-2.4009556571164));
#46547=CARTESIAN_POINT('Ctrl Pts',(-2.9701964131236,1.,-2.40438604734919));
#46548=CARTESIAN_POINT('Ctrl Pts',(-2.97646002822422,1.,-2.40768975073713));
#46549=CARTESIAN_POINT('Ctrl Pts',(-2.98280015815107,1.,-2.41095909342571));
#46550=CARTESIAN_POINT('Ctrl Pts',(-2.98927983005796,1.,-2.41425064199586));
#46551=CARTESIAN_POINT('Ctrl Pts',(-2.99590509293503,1.,-2.41757324500514));
#46552=CARTESIAN_POINT('Ctrl Pts',(-3.00264868585996,1.,-2.42090763946779));
#46553=CARTESIAN_POINT('Ctrl Pts',(-3.00946442616658,1.,-2.42421849439613));
#46554=CARTESIAN_POINT('Ctrl Pts',(-3.01630420830504,1.,-2.42746856264168));
#46555=CARTESIAN_POINT('Ctrl Pts',(-3.02313656036004,1.,-2.43063415586637));
#46556=CARTESIAN_POINT('Ctrl Pts',(-3.02995534946978,1.,-2.43371241361488));
#46557=CARTESIAN_POINT('Ctrl Pts',(-3.03676949672821,1.,-2.43671278042414));
#46558=CARTESIAN_POINT('Ctrl Pts',(-3.04359685040555,1.,-2.43965194061857));
#46559=CARTESIAN_POINT('Ctrl Pts',(-3.05045678021504,1.,-2.44254768923105));
#46560=CARTESIAN_POINT('Ctrl Pts',(-3.05736242671506,1.,-2.44541251892556));
#46561=CARTESIAN_POINT('Ctrl Pts',(-3.06431596421405,1.,-2.44824970516544));
#46562=CARTESIAN_POINT('Ctrl Pts',(-3.07131290521297,1.,-2.45105688854422));
#46563=CARTESIAN_POINT('Ctrl Pts',(-3.07834472886139,1.,-2.4538282678779));
#46564=CARTESIAN_POINT('Ctrl Pts',(-3.08540206545315,1.,-2.45655725437039));
#46565=CARTESIAN_POINT('Ctrl Pts',(-3.09247787931887,1.,-2.4592391256388));
#46566=CARTESIAN_POINT('Ctrl Pts',(-3.09956993697052,1.,-2.46187308501884));
#46567=CARTESIAN_POINT('Ctrl Pts',(-3.1066790790198,1.,-2.46446082979646));
#46568=CARTESIAN_POINT('Ctrl Pts',(-3.11380805536122,1.,-2.46700558843506));
#46569=CARTESIAN_POINT('Ctrl Pts',(-3.12096015766983,1.,-2.46951098947469));
#46570=CARTESIAN_POINT('Ctrl Pts',(-3.12813790805952,1.,-2.47197997765871));
#46571=CARTESIAN_POINT('Ctrl Pts',(-3.13534181229295,1.,-2.47441378371932));
#46572=CARTESIAN_POINT('Ctrl Pts',(-3.1425709954655,1.,-2.47681245356109));
#46573=CARTESIAN_POINT('Ctrl Pts',(-3.14982373241352,1.,-2.47917529057029));
#46574=CARTESIAN_POINT('Ctrl Pts',(-3.15709802322739,1.,-2.48150133566571));
#46575=CARTESIAN_POINT('Ctrl Pts',(-3.16439213290161,1.,-2.48378981792725));
#46576=CARTESIAN_POINT('Ctrl Pts',(-3.17170518863313,1.,-2.48604065348587));
#46577=CARTESIAN_POINT('Ctrl Pts',(-3.17903698136622,1.,-2.48825428288201));
#46578=CARTESIAN_POINT('Ctrl Pts',(-3.18638771282266,1.,-2.49043146334059));
#46579=CARTESIAN_POINT('Ctrl Pts',(-3.19375775555798,1.,-2.49257307239848));
#46580=CARTESIAN_POINT('Ctrl Pts',(-3.20114742397588,1.,-2.49467992057755));
#46581=CARTESIAN_POINT('Ctrl Pts',(-3.20855669849836,1.,-2.4967525264737));
#46582=CARTESIAN_POINT('Ctrl Pts',(-3.21598526261286,1.,-2.4987911459939));
#46583=CARTESIAN_POINT('Ctrl Pts',(-3.22343262620503,1.,-2.50079587201957));
#46584=CARTESIAN_POINT('Ctrl Pts',(-3.23089822320646,1.,-2.50276671338111));
#46585=CARTESIAN_POINT('Ctrl Pts',(-3.23838151080319,1.,-2.5047036758003));
#46586=CARTESIAN_POINT('Ctrl Pts',(-3.24588208983849,1.,-2.506606859405));
#46587=CARTESIAN_POINT('Ctrl Pts',(-3.25339971460982,1.,-2.50847647070723));
#46588=CARTESIAN_POINT('Ctrl Pts',(-3.26093423001434,1.,-2.51031277813486));
#46589=CARTESIAN_POINT('Ctrl Pts',(-3.26848552888115,1.,-2.51211608411423));
#46590=CARTESIAN_POINT('Ctrl Pts',(-3.27605350473142,1.,-2.513886692704));
#46591=CARTESIAN_POINT('Ctrl Pts',(-3.28363799702982,1.,-2.51562487464514));
#46592=CARTESIAN_POINT('Ctrl Pts',(-3.2912387729927,1.,-2.51733085123797));
#46593=CARTESIAN_POINT('Ctrl Pts',(-3.29885556388352,1.,-2.51900480701069));
#46594=CARTESIAN_POINT('Ctrl Pts',(-3.30648808815442,1.,-2.52064689568511));
#46595=CARTESIAN_POINT('Ctrl Pts',(-3.31413607874645,1.,-2.52225724871313));
#46596=CARTESIAN_POINT('Ctrl Pts',(-3.32179931078699,1.,-2.5238359839626));
#46597=CARTESIAN_POINT('Ctrl Pts',(-3.32947762187533,1.,-2.52538321164634));
#46598=CARTESIAN_POINT('Ctrl Pts',(-3.33717089999103,1.,-2.52689902690158));
#46599=CARTESIAN_POINT('Ctrl Pts',(-3.34333744115511,1.,-2.52808660915689));
#46600=CARTESIAN_POINT('Ctrl Pts',(-3.34796903576663,1.,-2.52896321610703));
#46601=CARTESIAN_POINT('Ctrl Pts',(-3.35105973714071,1.,-2.5295413654909));
#46602=CARTESIAN_POINT('Ctrl Pts',(-3.35260583073571,1.,-2.52982887637028));
#46603=CARTESIAN_POINT('Origin',(-3.35260583073571,0.,-2.52982887637028));
#46604=CARTESIAN_POINT('',(-3.44202241512147,1.,-2.40675750623143));
#46605=CARTESIAN_POINT('Origin',(0.,0.,0.));
#46606=CARTESIAN_POINT('',(-2.79140942341378,1.,-2.50410331873042));
#46607=CARTESIAN_POINT('Origin',(0.,1.,0.));
#46608=CARTESIAN_POINT('Ctrl Pts',(-2.79140942341378,1.,-2.50410331873042));
#46609=CARTESIAN_POINT('Ctrl Pts',(-2.79140942341378,0.666666666666667,
-2.50410331873042));
#46610=CARTESIAN_POINT('Ctrl Pts',(-2.79140942341378,0.333333333333333,
-2.50410331873042));
#46611=CARTESIAN_POINT('Ctrl Pts',(-2.79140942341378,-0.333333333333333,
-2.50410331873042));
#46612=CARTESIAN_POINT('Ctrl Pts',(-2.79140942341378,-0.666666666666667,
-2.50410331873042));
#46613=CARTESIAN_POINT('Ctrl Pts',(-2.79140942341378,-1.,-2.50410331873042));
#46614=CARTESIAN_POINT('Ctrl Pts',(-3.02314558451372,-1.,-2.91557726271063));
#46615=CARTESIAN_POINT('Ctrl Pts',(-3.02314558451372,1.,-2.91557726271063));
#46616=CARTESIAN_POINT('Ctrl Pts',(-3.02261975104912,-1.,-2.91409518070707));
#46617=CARTESIAN_POINT('Ctrl Pts',(-3.02261975104912,1.,-2.91409518070707));
#46618=CARTESIAN_POINT('Ctrl Pts',(-3.02156522743299,-1.,-2.91113297349052));
#46619=CARTESIAN_POINT('Ctrl Pts',(-3.02156522743299,1.,-2.91113297349052));
#46620=CARTESIAN_POINT('Ctrl Pts',(-3.01997487194926,-1.,-2.90669553303902));
#46621=CARTESIAN_POINT('Ctrl Pts',(-3.01997487194926,1.,-2.90669553303902));
#46622=CARTESIAN_POINT('Ctrl Pts',(-3.01783725123646,-1.,-2.90079069102661));
#46623=CARTESIAN_POINT('Ctrl Pts',(-3.01783725123646,1.,-2.90079069102661));
#46624=CARTESIAN_POINT('Ctrl Pts',(-3.01513660433291,-1.,-2.8934292556764));
#46625=CARTESIAN_POINT('Ctrl Pts',(-3.01513660433291,1.,-2.8934292556764));
#46626=CARTESIAN_POINT('Ctrl Pts',(-3.01240727309568,-1.,-2.88608751706796));
#46627=CARTESIAN_POINT('Ctrl Pts',(-3.01240727309568,1.,-2.88608751706796));
#46628=CARTESIAN_POINT('Ctrl Pts',(-3.0096491810855,-1.,-2.87876560072799));
#46629=CARTESIAN_POINT('Ctrl Pts',(-3.0096491810855,1.,-2.87876560072799));
#46630=CARTESIAN_POINT('Ctrl Pts',(-3.00686224485374,-1.,-2.87146368430104));
#46631=CARTESIAN_POINT('Ctrl Pts',(-3.00686224485374,1.,-2.87146368430104));
#46632=CARTESIAN_POINT('Ctrl Pts',(-3.00404638316245,-1.,-2.86418200833065));
#46633=CARTESIAN_POINT('Ctrl Pts',(-3.00404638316245,1.,-2.86418200833065));
#46634=CARTESIAN_POINT('Ctrl Pts',(-3.0012015079552,-1.,-2.85692085715129));
#46635=CARTESIAN_POINT('Ctrl Pts',(-3.0012015079552,1.,-2.85692085715129));
#46636=CARTESIAN_POINT('Ctrl Pts',(-2.99832751144566,-1.,-2.84968053289104));
#46637=CARTESIAN_POINT('Ctrl Pts',(-2.99832751144566,1.,-2.84968053289104));
#46638=CARTESIAN_POINT('Ctrl Pts',(-2.995424253416,-1.,-2.84246132984334));
#46639=CARTESIAN_POINT('Ctrl Pts',(-2.995424253416,1.,-2.84246132984334));
#46640=CARTESIAN_POINT('Ctrl Pts',(-2.99249155170479,-1.,-2.83526351254383));
#46641=CARTESIAN_POINT('Ctrl Pts',(-2.99249155170479,1.,-2.83526351254383));
#46642=CARTESIAN_POINT('Ctrl Pts',(-2.98952916401699,-1.,-2.82808728190402));
#46643=CARTESIAN_POINT('Ctrl Pts',(-2.98952916401699,1.,-2.82808728190402));
#46644=CARTESIAN_POINT('Ctrl Pts',(-2.98653680669434,-1.,-2.82093279065704));
#46645=CARTESIAN_POINT('Ctrl Pts',(-2.98653680669434,1.,-2.82093279065704));
#46646=CARTESIAN_POINT('Ctrl Pts',(-2.9835141977994,-1.,-2.81380019196454));
#46647=CARTESIAN_POINT('Ctrl Pts',(-2.9835141977994,1.,-2.81380019196454));
#46648=CARTESIAN_POINT('Ctrl Pts',(-2.98046109647299,-1.,-2.80668968101162));
#46649=CARTESIAN_POINT('Ctrl Pts',(-2.98046109647299,1.,-2.80668968101162));
#46650=CARTESIAN_POINT('Ctrl Pts',(-2.97737733718242,-1.,-2.79960153278186));
#46651=CARTESIAN_POINT('Ctrl Pts',(-2.97737733718242,1.,-2.79960153278186));
#46652=CARTESIAN_POINT('Ctrl Pts',(-2.97426288347475,-1.,-2.79253615718147));
#46653=CARTESIAN_POINT('Ctrl Pts',(-2.97426288347475,1.,-2.79253615718147));
#46654=CARTESIAN_POINT('Ctrl Pts',(-2.97111781461349,-1.,-2.78549409123657));
#46655=CARTESIAN_POINT('Ctrl Pts',(-2.97111781461349,1.,-2.78549409123657));
#46656=CARTESIAN_POINT('Ctrl Pts',(-2.9679422104295,-1.,-2.77847589542767));
#46657=CARTESIAN_POINT('Ctrl Pts',(-2.9679422104295,1.,-2.77847589542767));
#46658=CARTESIAN_POINT('Ctrl Pts',(-2.96473605585548,-1.,-2.77148206836464));
#46659=CARTESIAN_POINT('Ctrl Pts',(-2.96473605585548,1.,-2.77148206836464));
#46660=CARTESIAN_POINT('Ctrl Pts',(-2.96149914764832,-1.,-2.76451296269571));
#46661=CARTESIAN_POINT('Ctrl Pts',(-2.96149914764832,1.,-2.76451296269571));
#46662=CARTESIAN_POINT('Ctrl Pts',(-2.9582309766594,-1.,-2.75756867888393));
#46663=CARTESIAN_POINT('Ctrl Pts',(-2.9582309766594,1.,-2.75756867888393));
#46664=CARTESIAN_POINT('Ctrl Pts',(-2.95493069316211,-1.,-2.75064903318996));
#46665=CARTESIAN_POINT('Ctrl Pts',(-2.95493069316211,1.,-2.75064903318996));
#46666=CARTESIAN_POINT('Ctrl Pts',(-2.95159737214305,-1.,-2.7437537949221));
#46667=CARTESIAN_POINT('Ctrl Pts',(-2.95159737214305,1.,-2.7437537949221));
#46668=CARTESIAN_POINT('Ctrl Pts',(-2.94823023414381,-1.,-2.73688288329825));
#46669=CARTESIAN_POINT('Ctrl Pts',(-2.94823023414381,1.,-2.73688288329825));
#46670=CARTESIAN_POINT('Ctrl Pts',(-2.94482887675139,-1.,-2.73003657371613));
#46671=CARTESIAN_POINT('Ctrl Pts',(-2.94482887675139,1.,-2.73003657371613));
#46672=CARTESIAN_POINT('Ctrl Pts',(-2.94139351933882,-1.,-2.72321571511322));
#46673=CARTESIAN_POINT('Ctrl Pts',(-2.94139351933882,1.,-2.72321571511322));
#46674=CARTESIAN_POINT('Ctrl Pts',(-2.93792519474955,-1.,-2.71642190053575));
#46675=CARTESIAN_POINT('Ctrl Pts',(-2.93792519474955,1.,-2.71642190053575));
#46676=CARTESIAN_POINT('Ctrl Pts',(-2.93442516311168,-1.,-2.70965695523776));
#46677=CARTESIAN_POINT('Ctrl Pts',(-2.93442516311168,1.,-2.70965695523776));
#46678=CARTESIAN_POINT('Ctrl Pts',(-2.93089438233746,-1.,-2.70292247416881));
#46679=CARTESIAN_POINT('Ctrl Pts',(-2.93089438233746,1.,-2.70292247416881));
#46680=CARTESIAN_POINT('Ctrl Pts',(-2.92733294395268,-1.,-2.69621932864302));
#46681=CARTESIAN_POINT('Ctrl Pts',(-2.92733294395268,1.,-2.69621932864302));
#46682=CARTESIAN_POINT('Ctrl Pts',(-2.92373955325876,-1.,-2.68954721165342));
#46683=CARTESIAN_POINT('Ctrl Pts',(-2.92373955325876,1.,-2.68954721165342));
#46684=CARTESIAN_POINT('Ctrl Pts',(-2.92011090722152,-1.,-2.68290409279689));
#46685=CARTESIAN_POINT('Ctrl Pts',(-2.92011090722152,1.,-2.68290409279689));
#46686=CARTESIAN_POINT('Ctrl Pts',(-2.91644290704281,-1.,-2.67628728855309));
#46687=CARTESIAN_POINT('Ctrl Pts',(-2.91644290704281,1.,-2.67628728855309));
#46688=CARTESIAN_POINT('Ctrl Pts',(-2.91273193382876,-1.,-2.66969458792627));
#46689=CARTESIAN_POINT('Ctrl Pts',(-2.91273193382876,1.,-2.66969458792627));
#46690=CARTESIAN_POINT('Ctrl Pts',(-2.90897617968921,-1.,-2.66312542616808));
#46691=CARTESIAN_POINT('Ctrl Pts',(-2.90897617968921,1.,-2.66312542616808));
#46692=CARTESIAN_POINT('Ctrl Pts',(-2.90517678087467,-1.,-2.65658188464287));
#46693=CARTESIAN_POINT('Ctrl Pts',(-2.90517678087467,1.,-2.65658188464287));
#46694=CARTESIAN_POINT('Ctrl Pts',(-2.90133950224879,-1.,-2.65007017365576));
#46695=CARTESIAN_POINT('Ctrl Pts',(-2.90133950224879,1.,-2.65007017365576));
#46696=CARTESIAN_POINT('Ctrl Pts',(-2.89747231723361,-1.,-2.64359851684146));
#46697=CARTESIAN_POINT('Ctrl Pts',(-2.89747231723361,1.,-2.64359851684146));
#46698=CARTESIAN_POINT('Ctrl Pts',(-2.89358228854557,-1.,-2.63717442263944));
#46699=CARTESIAN_POINT('Ctrl Pts',(-2.89358228854557,1.,-2.63717442263944));
#46700=CARTESIAN_POINT('Ctrl Pts',(-2.88967244854243,-1.,-2.63080195420771));
#46701=CARTESIAN_POINT('Ctrl Pts',(-2.88967244854243,1.,-2.63080195420771));
#46702=CARTESIAN_POINT('Ctrl Pts',(-2.88573922195049,-1.,-2.62447947640253));
#46703=CARTESIAN_POINT('Ctrl Pts',(-2.88573922195049,1.,-2.62447947640253));
#46704=CARTESIAN_POINT('Ctrl Pts',(-2.88176821427502,-1.,-2.61819596473087));
#46705=CARTESIAN_POINT('Ctrl Pts',(-2.88176821427502,1.,-2.61819596473087));
#46706=CARTESIAN_POINT('Ctrl Pts',(-2.87773881947885,-1.,-2.61193507170928));
#46707=CARTESIAN_POINT('Ctrl Pts',(-2.87773881947885,1.,-2.61193507170928));
#46708=CARTESIAN_POINT('Ctrl Pts',(-2.87363176656475,-1.,-2.6056817788128));
#46709=CARTESIAN_POINT('Ctrl Pts',(-2.87363176656475,1.,-2.6056817788128));
#46710=CARTESIAN_POINT('Ctrl Pts',(-2.86943633170712,-1.,-2.59942875223202));
#46711=CARTESIAN_POINT('Ctrl Pts',(-2.86943633170712,1.,-2.59942875223202));
#46712=CARTESIAN_POINT('Ctrl Pts',(-2.86515629953528,-1.,-2.59318160184921));
#46713=CARTESIAN_POINT('Ctrl Pts',(-2.86515629953528,1.,-2.59318160184921));
#46714=CARTESIAN_POINT('Ctrl Pts',(-2.86081999003668,-1.,-2.5869677064356));
#46715=CARTESIAN_POINT('Ctrl Pts',(-2.86081999003668,1.,-2.5869677064356));
#46716=CARTESIAN_POINT('Ctrl Pts',(-2.85647171715147,-1.,-2.58082875254407));
#46717=CARTESIAN_POINT('Ctrl Pts',(-2.85647171715147,1.,-2.58082875254407));
#46718=CARTESIAN_POINT('Ctrl Pts',(-2.85215360144483,-1.,-2.57480482727128));
#46719=CARTESIAN_POINT('Ctrl Pts',(-2.85215360144483,1.,-2.57480482727128));
#46720=CARTESIAN_POINT('Ctrl Pts',(-2.84788893329091,-1.,-2.56891984251743));
#46721=CARTESIAN_POINT('Ctrl Pts',(-2.84788893329091,1.,-2.56891984251743));
#46722=CARTESIAN_POINT('Ctrl Pts',(-2.84366802680211,-1.,-2.56316920798489));
#46723=CARTESIAN_POINT('Ctrl Pts',(-2.84366802680211,1.,-2.56316920798489));
#46724=CARTESIAN_POINT('Ctrl Pts',(-2.83942515220699,-1.,-2.55749952145165));
#46725=CARTESIAN_POINT('Ctrl Pts',(-2.83942515220699,1.,-2.55749952145165));
#46726=CARTESIAN_POINT('Ctrl Pts',(-2.83505269592412,-1.,-2.55182152806964));
#46727=CARTESIAN_POINT('Ctrl Pts',(-2.83505269592412,1.,-2.55182152806964));
#46728=CARTESIAN_POINT('Ctrl Pts',(-2.83044254225794,-1.,-2.54604736792542));
#46729=CARTESIAN_POINT('Ctrl Pts',(-2.83044254225794,1.,-2.54604736792542));
#46730=CARTESIAN_POINT('Ctrl Pts',(-2.82552167649157,-1.,-2.54012272520141));
#46731=CARTESIAN_POINT('Ctrl Pts',(-2.82552167649157,1.,-2.54012272520141));
#46732=CARTESIAN_POINT('Ctrl Pts',(-2.82028550483744,-1.,-2.53405679667463));
#46733=CARTESIAN_POINT('Ctrl Pts',(-2.82028550483744,1.,-2.53405679667463));
#46734=CARTESIAN_POINT('Ctrl Pts',(-2.8148437904867,-1.,-2.52796388055457));
#46735=CARTESIAN_POINT('Ctrl Pts',(-2.8148437904867,1.,-2.52796388055457));
#46736=CARTESIAN_POINT('Ctrl Pts',(-2.80941521967234,-1.,-2.52205778589922));
#46737=CARTESIAN_POINT('Ctrl Pts',(-2.80941521967234,1.,-2.52205778589922));
#46738=CARTESIAN_POINT('Ctrl Pts',(-2.80427363984939,-1.,-2.51660190466067));
#46739=CARTESIAN_POINT('Ctrl Pts',(-2.80427363984939,1.,-2.51660190466067));
#46740=CARTESIAN_POINT('Ctrl Pts',(-2.79970585014308,-1.,-2.51186983687947));
#46741=CARTESIAN_POINT('Ctrl Pts',(-2.79970585014308,1.,-2.51186983687947));
#46742=CARTESIAN_POINT('Ctrl Pts',(-2.7959687805717,-1.,-2.50810555977564));
#46743=CARTESIAN_POINT('Ctrl Pts',(-2.7959687805717,1.,-2.50810555977564));
#46744=CARTESIAN_POINT('Ctrl Pts',(-2.79323694088143,-1.,-2.50547439929077));
#46745=CARTESIAN_POINT('Ctrl Pts',(-2.79323694088143,1.,-2.50547439929077));
#46746=CARTESIAN_POINT('Ctrl Pts',(-2.79192122906739,-1.,-2.50433799076945));
#46747=CARTESIAN_POINT('Ctrl Pts',(-2.79192122906739,1.,-2.50433799076945));
#46748=CARTESIAN_POINT('Ctrl Pts',(-2.79143626022225,-1.,-2.50404230339032));
#46749=CARTESIAN_POINT('Ctrl Pts',(-2.79143626022225,1.,-2.50404230339032));
#46750=CARTESIAN_POINT('Ctrl Pts',(-2.79133581100044,-1.,-2.50409239460011));
#46751=CARTESIAN_POINT('Ctrl Pts',(-2.79133581100044,1.,-2.50409239460011));
#46752=CARTESIAN_POINT('Ctrl Pts',(-2.79134130681569,-1.,-2.50417924854921));
#46753=CARTESIAN_POINT('Ctrl Pts',(-2.79134130681569,1.,-2.50417924854921));
#46754=CARTESIAN_POINT('',(-3.02314558451372,1.,-2.91557726271063));
#46755=CARTESIAN_POINT('Ctrl Pts',(-3.02314558451372,1.,-2.91557726271063));
#46756=CARTESIAN_POINT('Ctrl Pts',(-3.02261975104912,1.,-2.91409518070707));
#46757=CARTESIAN_POINT('Ctrl Pts',(-3.02156522743299,1.,-2.91113297349052));
#46758=CARTESIAN_POINT('Ctrl Pts',(-3.01997487194926,1.,-2.90669553303902));
#46759=CARTESIAN_POINT('Ctrl Pts',(-3.01783725123646,1.,-2.90079069102661));
#46760=CARTESIAN_POINT('Ctrl Pts',(-3.01513660433291,1.,-2.8934292556764));
#46761=CARTESIAN_POINT('Ctrl Pts',(-3.01240727309568,1.,-2.88608751706796));
#46762=CARTESIAN_POINT('Ctrl Pts',(-3.0096491810855,1.,-2.87876560072799));
#46763=CARTESIAN_POINT('Ctrl Pts',(-3.00686224485374,1.,-2.87146368430104));
#46764=CARTESIAN_POINT('Ctrl Pts',(-3.00404638316245,1.,-2.86418200833065));
#46765=CARTESIAN_POINT('Ctrl Pts',(-3.0012015079552,1.,-2.85692085715129));
#46766=CARTESIAN_POINT('Ctrl Pts',(-2.99832751144566,1.,-2.84968053289104));
#46767=CARTESIAN_POINT('Ctrl Pts',(-2.995424253416,1.,-2.84246132984334));
#46768=CARTESIAN_POINT('Ctrl Pts',(-2.99249155170479,1.,-2.83526351254383));
#46769=CARTESIAN_POINT('Ctrl Pts',(-2.98952916401699,1.,-2.82808728190402));
#46770=CARTESIAN_POINT('Ctrl Pts',(-2.98653680669434,1.,-2.82093279065704));
#46771=CARTESIAN_POINT('Ctrl Pts',(-2.9835141977994,1.,-2.81380019196454));
#46772=CARTESIAN_POINT('Ctrl Pts',(-2.98046109647299,1.,-2.80668968101162));
#46773=CARTESIAN_POINT('Ctrl Pts',(-2.97737733718242,1.,-2.79960153278186));
#46774=CARTESIAN_POINT('Ctrl Pts',(-2.97426288347475,1.,-2.79253615718147));
#46775=CARTESIAN_POINT('Ctrl Pts',(-2.97111781461349,1.,-2.78549409123657));
#46776=CARTESIAN_POINT('Ctrl Pts',(-2.9679422104295,1.,-2.77847589542767));
#46777=CARTESIAN_POINT('Ctrl Pts',(-2.96473605585548,1.,-2.77148206836464));
#46778=CARTESIAN_POINT('Ctrl Pts',(-2.96149914764832,1.,-2.76451296269571));
#46779=CARTESIAN_POINT('Ctrl Pts',(-2.9582309766594,1.,-2.75756867888393));
#46780=CARTESIAN_POINT('Ctrl Pts',(-2.95493069316211,1.,-2.75064903318996));
#46781=CARTESIAN_POINT('Ctrl Pts',(-2.95159737214305,1.,-2.7437537949221));
#46782=CARTESIAN_POINT('Ctrl Pts',(-2.94823023414381,1.,-2.73688288329825));
#46783=CARTESIAN_POINT('Ctrl Pts',(-2.94482887675139,1.,-2.73003657371613));
#46784=CARTESIAN_POINT('Ctrl Pts',(-2.94139351933882,1.,-2.72321571511322));
#46785=CARTESIAN_POINT('Ctrl Pts',(-2.93792519474955,1.,-2.71642190053575));
#46786=CARTESIAN_POINT('Ctrl Pts',(-2.93442516311168,1.,-2.70965695523776));
#46787=CARTESIAN_POINT('Ctrl Pts',(-2.93089438233746,1.,-2.70292247416881));
#46788=CARTESIAN_POINT('Ctrl Pts',(-2.92733294395268,1.,-2.69621932864302));
#46789=CARTESIAN_POINT('Ctrl Pts',(-2.92373955325876,1.,-2.68954721165342));
#46790=CARTESIAN_POINT('Ctrl Pts',(-2.92011090722152,1.,-2.68290409279689));
#46791=CARTESIAN_POINT('Ctrl Pts',(-2.91644290704281,1.,-2.67628728855309));
#46792=CARTESIAN_POINT('Ctrl Pts',(-2.91273193382876,1.,-2.66969458792627));
#46793=CARTESIAN_POINT('Ctrl Pts',(-2.90897617968921,1.,-2.66312542616808));
#46794=CARTESIAN_POINT('Ctrl Pts',(-2.90517678087467,1.,-2.65658188464287));
#46795=CARTESIAN_POINT('Ctrl Pts',(-2.90133950224879,1.,-2.65007017365576));
#46796=CARTESIAN_POINT('Ctrl Pts',(-2.89747231723361,1.,-2.64359851684146));
#46797=CARTESIAN_POINT('Ctrl Pts',(-2.89358228854557,1.,-2.63717442263944));
#46798=CARTESIAN_POINT('Ctrl Pts',(-2.88967244854243,1.,-2.63080195420771));
#46799=CARTESIAN_POINT('Ctrl Pts',(-2.88573922195049,1.,-2.62447947640253));
#46800=CARTESIAN_POINT('Ctrl Pts',(-2.88176821427502,1.,-2.61819596473087));
#46801=CARTESIAN_POINT('Ctrl Pts',(-2.87773881947885,1.,-2.61193507170928));
#46802=CARTESIAN_POINT('Ctrl Pts',(-2.87363176656475,1.,-2.6056817788128));
#46803=CARTESIAN_POINT('Ctrl Pts',(-2.86943633170712,1.,-2.59942875223202));
#46804=CARTESIAN_POINT('Ctrl Pts',(-2.86515629953528,1.,-2.59318160184921));
#46805=CARTESIAN_POINT('Ctrl Pts',(-2.86081999003668,1.,-2.5869677064356));
#46806=CARTESIAN_POINT('Ctrl Pts',(-2.85647171715147,1.,-2.58082875254407));
#46807=CARTESIAN_POINT('Ctrl Pts',(-2.85215360144483,1.,-2.57480482727128));
#46808=CARTESIAN_POINT('Ctrl Pts',(-2.84788893329091,1.,-2.56891984251743));
#46809=CARTESIAN_POINT('Ctrl Pts',(-2.84366802680211,1.,-2.56316920798489));
#46810=CARTESIAN_POINT('Ctrl Pts',(-2.83942515220699,1.,-2.55749952145165));
#46811=CARTESIAN_POINT('Ctrl Pts',(-2.83505269592412,1.,-2.55182152806964));
#46812=CARTESIAN_POINT('Ctrl Pts',(-2.83044254225794,1.,-2.54604736792542));
#46813=CARTESIAN_POINT('Ctrl Pts',(-2.82552167649157,1.,-2.54012272520141));
#46814=CARTESIAN_POINT('Ctrl Pts',(-2.82028550483744,1.,-2.53405679667463));
#46815=CARTESIAN_POINT('Ctrl Pts',(-2.8148437904867,1.,-2.52796388055457));
#46816=CARTESIAN_POINT('Ctrl Pts',(-2.80941521967234,1.,-2.52205778589922));
#46817=CARTESIAN_POINT('Ctrl Pts',(-2.80427363984939,1.,-2.51660190466067));
#46818=CARTESIAN_POINT('Ctrl Pts',(-2.79970585014308,1.,-2.51186983687947));
#46819=CARTESIAN_POINT('Ctrl Pts',(-2.7959687805717,1.,-2.50810555977564));
#46820=CARTESIAN_POINT('Ctrl Pts',(-2.79344192164204,1.,-2.50567182569153));
#46821=CARTESIAN_POINT('Ctrl Pts',(-2.79217568804874,1.,-2.50455968395235));
#46822=CARTESIAN_POINT('Ctrl Pts',(-2.79164172519039,1.,-2.50417932839344));
#46823=CARTESIAN_POINT('Ctrl Pts',(-2.79145823440899,1.,-2.50410700351427));
#46824=CARTESIAN_POINT('Ctrl Pts',(-2.79140942341378,1.,-2.50410331873043));
#46825=CARTESIAN_POINT('',(-3.02314558451372,0.,-2.91557726271063));
#46826=CARTESIAN_POINT('Ctrl Pts',(-2.50417924854921,-1.,-2.79134130681569));
#46827=CARTESIAN_POINT('Ctrl Pts',(-2.50417924854921,1.,-2.79134130681569));
#46828=CARTESIAN_POINT('Ctrl Pts',(-2.50409239460108,-1.,-2.7913358110015));
#46829=CARTESIAN_POINT('Ctrl Pts',(-2.50409239460108,1.,-2.7913358110015));
#46830=CARTESIAN_POINT('Ctrl Pts',(-2.50404230339286,-1.,-2.79143626022503));
#46831=CARTESIAN_POINT('Ctrl Pts',(-2.50404230339286,1.,-2.79143626022503));
#46832=CARTESIAN_POINT('Ctrl Pts',(-2.5043379907732,-1.,-2.79192122907148));
#46833=CARTESIAN_POINT('Ctrl Pts',(-2.5043379907732,1.,-2.79192122907148));
#46834=CARTESIAN_POINT('Ctrl Pts',(-2.50547439929414,-1.,-2.7932369408851));
#46835=CARTESIAN_POINT('Ctrl Pts',(-2.50547439929414,1.,-2.7932369408851));
#46836=CARTESIAN_POINT('Ctrl Pts',(-2.50810555977671,-1.,-2.79596878057287));
#46837=CARTESIAN_POINT('Ctrl Pts',(-2.50810555977671,1.,-2.79596878057287));
#46838=CARTESIAN_POINT('Ctrl Pts',(-2.51186983687818,-1.,-2.79970585014168));
#46839=CARTESIAN_POINT('Ctrl Pts',(-2.51186983687818,1.,-2.79970585014168));
#46840=CARTESIAN_POINT('Ctrl Pts',(-2.51660190465805,-1.,-2.80427363984653));
#46841=CARTESIAN_POINT('Ctrl Pts',(-2.51660190465805,1.,-2.80427363984653));
#46842=CARTESIAN_POINT('Ctrl Pts',(-2.52205778589653,-1.,-2.80941521966941));
#46843=CARTESIAN_POINT('Ctrl Pts',(-2.52205778589653,1.,-2.80941521966941));
#46844=CARTESIAN_POINT('Ctrl Pts',(-2.52796388055278,-1.,-2.81484379048475));
#46845=CARTESIAN_POINT('Ctrl Pts',(-2.52796388055278,1.,-2.81484379048475));
#46846=CARTESIAN_POINT('Ctrl Pts',(-2.53405679667412,-1.,-2.82028550483689));
#46847=CARTESIAN_POINT('Ctrl Pts',(-2.53405679667412,1.,-2.82028550483689));
#46848=CARTESIAN_POINT('Ctrl Pts',(-2.54012272520199,-1.,-2.8255216764922));
#46849=CARTESIAN_POINT('Ctrl Pts',(-2.54012272520199,1.,-2.8255216764922));
#46850=CARTESIAN_POINT('Ctrl Pts',(-2.54604736792655,-1.,-2.83044254225917));
#46851=CARTESIAN_POINT('Ctrl Pts',(-2.54604736792655,1.,-2.83044254225917));
#46852=CARTESIAN_POINT('Ctrl Pts',(-2.55182152807077,-1.,-2.83505269592536));
#46853=CARTESIAN_POINT('Ctrl Pts',(-2.55182152807077,1.,-2.83505269592536));
#46854=CARTESIAN_POINT('Ctrl Pts',(-2.55749952145241,-1.,-2.83942515220782));
#46855=CARTESIAN_POINT('Ctrl Pts',(-2.55749952145241,1.,-2.83942515220782));
#46856=CARTESIAN_POINT('Ctrl Pts',(-2.56316920798513,-1.,-2.84366802680237));
#46857=CARTESIAN_POINT('Ctrl Pts',(-2.56316920798513,1.,-2.84366802680237));
#46858=CARTESIAN_POINT('Ctrl Pts',(-2.56891984251721,-1.,-2.84788893329067));
#46859=CARTESIAN_POINT('Ctrl Pts',(-2.56891984251721,1.,-2.84788893329067));
#46860=CARTESIAN_POINT('Ctrl Pts',(-2.57480482727081,-1.,-2.85215360144431));
#46861=CARTESIAN_POINT('Ctrl Pts',(-2.57480482727081,1.,-2.85215360144431));
#46862=CARTESIAN_POINT('Ctrl Pts',(-2.58082875254357,-1.,-2.85647171715092));
#46863=CARTESIAN_POINT('Ctrl Pts',(-2.58082875254357,1.,-2.85647171715092));
#46864=CARTESIAN_POINT('Ctrl Pts',(-2.58696770643524,-1.,-2.86081999003629));
#46865=CARTESIAN_POINT('Ctrl Pts',(-2.58696770643524,1.,-2.86081999003629));
#46866=CARTESIAN_POINT('Ctrl Pts',(-2.59318160184908,-1.,-2.86515629953513));
#46867=CARTESIAN_POINT('Ctrl Pts',(-2.59318160184908,1.,-2.86515629953513));
#46868=CARTESIAN_POINT('Ctrl Pts',(-2.5994287522321,-1.,-2.86943633170722));
#46869=CARTESIAN_POINT('Ctrl Pts',(-2.5994287522321,1.,-2.86943633170722));
#46870=CARTESIAN_POINT('Ctrl Pts',(-2.60568177881303,-1.,-2.87363176656501));
#46871=CARTESIAN_POINT('Ctrl Pts',(-2.60568177881303,1.,-2.87363176656501));
#46872=CARTESIAN_POINT('Ctrl Pts',(-2.61193507170955,-1.,-2.87773881947915));
#46873=CARTESIAN_POINT('Ctrl Pts',(-2.61193507170955,1.,-2.87773881947915));
#46874=CARTESIAN_POINT('Ctrl Pts',(-2.61819596473108,-1.,-2.88176821427525));
#46875=CARTESIAN_POINT('Ctrl Pts',(-2.61819596473108,1.,-2.88176821427525));
#46876=CARTESIAN_POINT('Ctrl Pts',(-2.62447947640262,-1.,-2.88573922195059));
#46877=CARTESIAN_POINT('Ctrl Pts',(-2.62447947640262,1.,-2.88573922195059));
#46878=CARTESIAN_POINT('Ctrl Pts',(-2.63080195420767,-1.,-2.88967244854239));
#46879=CARTESIAN_POINT('Ctrl Pts',(-2.63080195420767,1.,-2.88967244854239));
#46880=CARTESIAN_POINT('Ctrl Pts',(-2.63717442263932,-1.,-2.89358228854544));
#46881=CARTESIAN_POINT('Ctrl Pts',(-2.63717442263932,1.,-2.89358228854544));
#46882=CARTESIAN_POINT('Ctrl Pts',(-2.64359851684131,-1.,-2.89747231723345));
#46883=CARTESIAN_POINT('Ctrl Pts',(-2.64359851684131,1.,-2.89747231723345));
#46884=CARTESIAN_POINT('Ctrl Pts',(-2.65007017365564,-1.,-2.90133950224867));
#46885=CARTESIAN_POINT('Ctrl Pts',(-2.65007017365564,1.,-2.90133950224867));
#46886=CARTESIAN_POINT('Ctrl Pts',(-2.65658188464282,-1.,-2.90517678087461));
#46887=CARTESIAN_POINT('Ctrl Pts',(-2.65658188464282,1.,-2.90517678087461));
#46888=CARTESIAN_POINT('Ctrl Pts',(-2.6631254261681,-1.,-2.90897617968923));
#46889=CARTESIAN_POINT('Ctrl Pts',(-2.6631254261681,1.,-2.90897617968923));
#46890=CARTESIAN_POINT('Ctrl Pts',(-2.66969458792631,-1.,-2.91273193382882));
#46891=CARTESIAN_POINT('Ctrl Pts',(-2.66969458792631,1.,-2.91273193382882));
#46892=CARTESIAN_POINT('Ctrl Pts',(-2.67628728855312,-1.,-2.91644290704285));
#46893=CARTESIAN_POINT('Ctrl Pts',(-2.67628728855312,1.,-2.91644290704285));
#46894=CARTESIAN_POINT('Ctrl Pts',(-2.68290409279688,-1.,-2.92011090722152));
#46895=CARTESIAN_POINT('Ctrl Pts',(-2.68290409279688,1.,-2.92011090722152));
#46896=CARTESIAN_POINT('Ctrl Pts',(-2.68954721165339,-1.,-2.92373955325875));
#46897=CARTESIAN_POINT('Ctrl Pts',(-2.68954721165339,1.,-2.92373955325875));
#46898=CARTESIAN_POINT('Ctrl Pts',(-2.69621932864301,-1.,-2.92733294395267));
#46899=CARTESIAN_POINT('Ctrl Pts',(-2.69621932864301,1.,-2.92733294395267));
#46900=CARTESIAN_POINT('Ctrl Pts',(-2.70292247416885,-1.,-2.93089438233749));
#46901=CARTESIAN_POINT('Ctrl Pts',(-2.70292247416885,1.,-2.93089438233749));
#46902=CARTESIAN_POINT('Ctrl Pts',(-2.70965695523787,-1.,-2.93442516311179));
#46903=CARTESIAN_POINT('Ctrl Pts',(-2.70965695523787,1.,-2.93442516311179));
#46904=CARTESIAN_POINT('Ctrl Pts',(-2.71642190053592,-1.,-2.93792519474972));
#46905=CARTESIAN_POINT('Ctrl Pts',(-2.71642190053592,1.,-2.93792519474972));
#46906=CARTESIAN_POINT('Ctrl Pts',(-2.72321571511337,-1.,-2.94139351933897));
#46907=CARTESIAN_POINT('Ctrl Pts',(-2.72321571511337,1.,-2.94139351933897));
#46908=CARTESIAN_POINT('Ctrl Pts',(-2.73003657371617,-1.,-2.94482887675143));
#46909=CARTESIAN_POINT('Ctrl Pts',(-2.73003657371617,1.,-2.94482887675143));
#46910=CARTESIAN_POINT('Ctrl Pts',(-2.73688288329808,-1.,-2.94823023414364));
#46911=CARTESIAN_POINT('Ctrl Pts',(-2.73688288329808,1.,-2.94823023414364));
#46912=CARTESIAN_POINT('Ctrl Pts',(-2.74375379492172,-1.,-2.95159737214266));
#46913=CARTESIAN_POINT('Ctrl Pts',(-2.74375379492172,1.,-2.95159737214266));
#46914=CARTESIAN_POINT('Ctrl Pts',(-2.75064903318947,-1.,-2.95493069316161));
#46915=CARTESIAN_POINT('Ctrl Pts',(-2.75064903318947,1.,-2.95493069316161));
#46916=CARTESIAN_POINT('Ctrl Pts',(-2.7575686788835,-1.,-2.95823097665896));
#46917=CARTESIAN_POINT('Ctrl Pts',(-2.7575686788835,1.,-2.95823097665896));
#46918=CARTESIAN_POINT('Ctrl Pts',(-2.76451296269557,-1.,-2.96149914764818));
#46919=CARTESIAN_POINT('Ctrl Pts',(-2.76451296269557,1.,-2.96149914764818));
#46920=CARTESIAN_POINT('Ctrl Pts',(-2.77148206836498,-1.,-2.96473605585583));
#46921=CARTESIAN_POINT('Ctrl Pts',(-2.77148206836498,1.,-2.96473605585583));
#46922=CARTESIAN_POINT('Ctrl Pts',(-2.7784758954285,-1.,-2.96794221043036));
#46923=CARTESIAN_POINT('Ctrl Pts',(-2.7784758954285,1.,-2.96794221043036));
#46924=CARTESIAN_POINT('Ctrl Pts',(-2.78549409123769,-1.,-2.97111781461465));
#46925=CARTESIAN_POINT('Ctrl Pts',(-2.78549409123769,1.,-2.97111781461465));
#46926=CARTESIAN_POINT('Ctrl Pts',(-2.79253615718248,-1.,-2.9742628834758));
#46927=CARTESIAN_POINT('Ctrl Pts',(-2.79253615718248,1.,-2.9742628834758));
#46928=CARTESIAN_POINT('Ctrl Pts',(-2.7996015327823,-1.,-2.97737733718287));
#46929=CARTESIAN_POINT('Ctrl Pts',(-2.7996015327823,1.,-2.97737733718287));
#46930=CARTESIAN_POINT('Ctrl Pts',(-2.80668968101106,-1.,-2.98046109647241));
#46931=CARTESIAN_POINT('Ctrl Pts',(-2.80668968101106,1.,-2.98046109647241));
#46932=CARTESIAN_POINT('Ctrl Pts',(-2.81380019196286,-1.,-2.98351419779767));
#46933=CARTESIAN_POINT('Ctrl Pts',(-2.81380019196286,1.,-2.98351419779767));
#46934=CARTESIAN_POINT('Ctrl Pts',(-2.82093279065457,-1.,-2.9865368066918));
#46935=CARTESIAN_POINT('Ctrl Pts',(-2.82093279065457,1.,-2.9865368066918));
#46936=CARTESIAN_POINT('Ctrl Pts',(-2.82808728190157,-1.,-2.98952916401446));
#46937=CARTESIAN_POINT('Ctrl Pts',(-2.82808728190157,1.,-2.98952916401446));
#46938=CARTESIAN_POINT('Ctrl Pts',(-2.83526351254248,-1.,-2.99249155170339));
#46939=CARTESIAN_POINT('Ctrl Pts',(-2.83526351254248,1.,-2.99249155170339));
#46940=CARTESIAN_POINT('Ctrl Pts',(-2.84246132984415,-1.,-2.99542425341685));
#46941=CARTESIAN_POINT('Ctrl Pts',(-2.84246132984415,1.,-2.99542425341685));
#46942=CARTESIAN_POINT('Ctrl Pts',(-2.84968053289451,-1.,-2.99832751144925));
#46943=CARTESIAN_POINT('Ctrl Pts',(-2.84968053289451,1.,-2.99832751144925));
#46944=CARTESIAN_POINT('Ctrl Pts',(-2.85692085715686,-1.,-3.00120150796095));
#46945=CARTESIAN_POINT('Ctrl Pts',(-2.85692085715686,1.,-3.00120150796095));
#46946=CARTESIAN_POINT('Ctrl Pts',(-2.86418200833667,-1.,-3.00404638316867));
#46947=CARTESIAN_POINT('Ctrl Pts',(-2.86418200833667,1.,-3.00404638316867));
#46948=CARTESIAN_POINT('Ctrl Pts',(-2.87146368430502,-1.,-3.00686224485784));
#46949=CARTESIAN_POINT('Ctrl Pts',(-2.87146368430502,1.,-3.00686224485784));
#46950=CARTESIAN_POINT('Ctrl Pts',(-2.87876560072727,-1.,-3.00964918108476));
#46951=CARTESIAN_POINT('Ctrl Pts',(-2.87876560072727,1.,-3.00964918108476));
#46952=CARTESIAN_POINT('Ctrl Pts',(-2.8860875170608,-1.,-3.01240727308829));
#46953=CARTESIAN_POINT('Ctrl Pts',(-2.8860875170608,1.,-3.01240727308829));
#46954=CARTESIAN_POINT('Ctrl Pts',(-2.89342925566321,-1.,-3.01513660431928));
#46955=CARTESIAN_POINT('Ctrl Pts',(-2.89342925566321,1.,-3.01513660431928));
#46956=CARTESIAN_POINT('Ctrl Pts',(-2.9007906910105,-1.,-3.01783725121981));
#46957=CARTESIAN_POINT('Ctrl Pts',(-2.9007906910105,1.,-3.01783725121981));
#46958=CARTESIAN_POINT('Ctrl Pts',(-2.90669553302526,-1.,-3.01997487193503));
#46959=CARTESIAN_POINT('Ctrl Pts',(-2.90669553302526,1.,-3.01997487193503));
#46960=CARTESIAN_POINT('Ctrl Pts',(-2.91113297348212,-1.,-3.02156522742431));
#46961=CARTESIAN_POINT('Ctrl Pts',(-2.91113297348212,1.,-3.02156522742431));
#46962=CARTESIAN_POINT('Ctrl Pts',(-2.91409518070399,-1.,-3.02261975104593));
#46963=CARTESIAN_POINT('Ctrl Pts',(-2.91409518070399,1.,-3.02261975104593));
#46964=CARTESIAN_POINT('Ctrl Pts',(-2.91557726271063,-1.,-3.02314558451372));
#46965=CARTESIAN_POINT('Ctrl Pts',(-2.91557726271063,1.,-3.02314558451372));
#46966=CARTESIAN_POINT('',(-2.50410331873176,1.,-2.79140942341258));
#46967=CARTESIAN_POINT('Ctrl Pts',(-2.50410331873176,-1.,-2.79140942341258));
#46968=CARTESIAN_POINT('Ctrl Pts',(-2.50410331873176,-0.666666666666667,
-2.79140942341258));
#46969=CARTESIAN_POINT('Ctrl Pts',(-2.50410331873176,-0.333333333333333,
-2.79140942341258));
#46970=CARTESIAN_POINT('Ctrl Pts',(-2.50410331873176,0.333333333333333,
-2.79140942341258));
#46971=CARTESIAN_POINT('Ctrl Pts',(-2.50410331873176,0.666666666666667,
-2.79140942341258));
#46972=CARTESIAN_POINT('Ctrl Pts',(-2.50410331873176,1.,-2.79140942341258));
#46973=CARTESIAN_POINT('',(-2.91557726271063,1.,-3.02314558451372));
#46974=CARTESIAN_POINT('',(-2.91557726271063,0.,-3.02314558451372));
#46975=CARTESIAN_POINT('Ctrl Pts',(-2.50410331873176,1.,-2.79140942341258));
#46976=CARTESIAN_POINT('Ctrl Pts',(-2.50410700351493,1.,-2.79145823440781));
#46977=CARTESIAN_POINT('Ctrl Pts',(-2.50417932839313,1.,-2.79164172518905));
#46978=CARTESIAN_POINT('Ctrl Pts',(-2.50455968395146,1.,-2.79217568804755));
#46979=CARTESIAN_POINT('Ctrl Pts',(-2.50567182569081,1.,-2.79344192164147));
#46980=CARTESIAN_POINT('Ctrl Pts',(-2.50810555977671,1.,-2.79596878057287));
#46981=CARTESIAN_POINT('Ctrl Pts',(-2.51186983687818,1.,-2.79970585014168));
#46982=CARTESIAN_POINT('Ctrl Pts',(-2.51660190465805,1.,-2.80427363984653));
#46983=CARTESIAN_POINT('Ctrl Pts',(-2.52205778589653,1.,-2.80941521966941));
#46984=CARTESIAN_POINT('Ctrl Pts',(-2.52796388055278,1.,-2.81484379048475));
#46985=CARTESIAN_POINT('Ctrl Pts',(-2.53405679667412,1.,-2.82028550483689));
#46986=CARTESIAN_POINT('Ctrl Pts',(-2.54012272520199,1.,-2.8255216764922));
#46987=CARTESIAN_POINT('Ctrl Pts',(-2.54604736792655,1.,-2.83044254225917));
#46988=CARTESIAN_POINT('Ctrl Pts',(-2.55182152807077,1.,-2.83505269592536));
#46989=CARTESIAN_POINT('Ctrl Pts',(-2.55749952145241,1.,-2.83942515220782));
#46990=CARTESIAN_POINT('Ctrl Pts',(-2.56316920798513,1.,-2.84366802680237));
#46991=CARTESIAN_POINT('Ctrl Pts',(-2.56891984251721,1.,-2.84788893329067));
#46992=CARTESIAN_POINT('Ctrl Pts',(-2.57480482727081,1.,-2.85215360144431));
#46993=CARTESIAN_POINT('Ctrl Pts',(-2.58082875254357,1.,-2.85647171715092));
#46994=CARTESIAN_POINT('Ctrl Pts',(-2.58696770643524,1.,-2.86081999003629));
#46995=CARTESIAN_POINT('Ctrl Pts',(-2.59318160184908,1.,-2.86515629953513));
#46996=CARTESIAN_POINT('Ctrl Pts',(-2.5994287522321,1.,-2.86943633170722));
#46997=CARTESIAN_POINT('Ctrl Pts',(-2.60568177881303,1.,-2.87363176656501));
#46998=CARTESIAN_POINT('Ctrl Pts',(-2.61193507170955,1.,-2.87773881947915));
#46999=CARTESIAN_POINT('Ctrl Pts',(-2.61819596473108,1.,-2.88176821427525));
#47000=CARTESIAN_POINT('Ctrl Pts',(-2.62447947640262,1.,-2.88573922195059));
#47001=CARTESIAN_POINT('Ctrl Pts',(-2.63080195420767,1.,-2.88967244854239));
#47002=CARTESIAN_POINT('Ctrl Pts',(-2.63717442263932,1.,-2.89358228854544));
#47003=CARTESIAN_POINT('Ctrl Pts',(-2.64359851684131,1.,-2.89747231723345));
#47004=CARTESIAN_POINT('Ctrl Pts',(-2.65007017365564,1.,-2.90133950224867));
#47005=CARTESIAN_POINT('Ctrl Pts',(-2.65658188464282,1.,-2.90517678087461));
#47006=CARTESIAN_POINT('Ctrl Pts',(-2.6631254261681,1.,-2.90897617968923));
#47007=CARTESIAN_POINT('Ctrl Pts',(-2.66969458792631,1.,-2.91273193382882));
#47008=CARTESIAN_POINT('Ctrl Pts',(-2.67628728855312,1.,-2.91644290704285));
#47009=CARTESIAN_POINT('Ctrl Pts',(-2.68290409279688,1.,-2.92011090722152));
#47010=CARTESIAN_POINT('Ctrl Pts',(-2.68954721165339,1.,-2.92373955325875));
#47011=CARTESIAN_POINT('Ctrl Pts',(-2.69621932864301,1.,-2.92733294395267));
#47012=CARTESIAN_POINT('Ctrl Pts',(-2.70292247416885,1.,-2.93089438233749));
#47013=CARTESIAN_POINT('Ctrl Pts',(-2.70965695523787,1.,-2.93442516311179));
#47014=CARTESIAN_POINT('Ctrl Pts',(-2.71642190053592,1.,-2.93792519474972));
#47015=CARTESIAN_POINT('Ctrl Pts',(-2.72321571511337,1.,-2.94139351933897));
#47016=CARTESIAN_POINT('Ctrl Pts',(-2.73003657371617,1.,-2.94482887675143));
#47017=CARTESIAN_POINT('Ctrl Pts',(-2.73688288329808,1.,-2.94823023414364));
#47018=CARTESIAN_POINT('Ctrl Pts',(-2.74375379492172,1.,-2.95159737214266));
#47019=CARTESIAN_POINT('Ctrl Pts',(-2.75064903318947,1.,-2.95493069316161));
#47020=CARTESIAN_POINT('Ctrl Pts',(-2.7575686788835,1.,-2.95823097665896));
#47021=CARTESIAN_POINT('Ctrl Pts',(-2.76451296269557,1.,-2.96149914764818));
#47022=CARTESIAN_POINT('Ctrl Pts',(-2.77148206836498,1.,-2.96473605585583));
#47023=CARTESIAN_POINT('Ctrl Pts',(-2.7784758954285,1.,-2.96794221043036));
#47024=CARTESIAN_POINT('Ctrl Pts',(-2.78549409123769,1.,-2.97111781461465));
#47025=CARTESIAN_POINT('Ctrl Pts',(-2.79253615718248,1.,-2.9742628834758));
#47026=CARTESIAN_POINT('Ctrl Pts',(-2.7996015327823,1.,-2.97737733718287));
#47027=CARTESIAN_POINT('Ctrl Pts',(-2.80668968101106,1.,-2.98046109647241));
#47028=CARTESIAN_POINT('Ctrl Pts',(-2.81380019196286,1.,-2.98351419779767));
#47029=CARTESIAN_POINT('Ctrl Pts',(-2.82093279065457,1.,-2.9865368066918));
#47030=CARTESIAN_POINT('Ctrl Pts',(-2.82808728190157,1.,-2.98952916401446));
#47031=CARTESIAN_POINT('Ctrl Pts',(-2.83526351254248,1.,-2.99249155170339));
#47032=CARTESIAN_POINT('Ctrl Pts',(-2.84246132984415,1.,-2.99542425341685));
#47033=CARTESIAN_POINT('Ctrl Pts',(-2.84968053289451,1.,-2.99832751144925));
#47034=CARTESIAN_POINT('Ctrl Pts',(-2.85692085715686,1.,-3.00120150796095));
#47035=CARTESIAN_POINT('Ctrl Pts',(-2.86418200833667,1.,-3.00404638316867));
#47036=CARTESIAN_POINT('Ctrl Pts',(-2.87146368430502,1.,-3.00686224485784));
#47037=CARTESIAN_POINT('Ctrl Pts',(-2.87876560072727,1.,-3.00964918108476));
#47038=CARTESIAN_POINT('Ctrl Pts',(-2.8860875170608,1.,-3.01240727308829));
#47039=CARTESIAN_POINT('Ctrl Pts',(-2.89342925566321,1.,-3.01513660431928));
#47040=CARTESIAN_POINT('Ctrl Pts',(-2.9007906910105,1.,-3.01783725121981));
#47041=CARTESIAN_POINT('Ctrl Pts',(-2.90669553302526,1.,-3.01997487193503));
#47042=CARTESIAN_POINT('Ctrl Pts',(-2.91113297348212,1.,-3.02156522742431));
#47043=CARTESIAN_POINT('Ctrl Pts',(-2.91409518070399,1.,-3.02261975104593));
#47044=CARTESIAN_POINT('Ctrl Pts',(-2.91557726271063,1.,-3.02314558451372));
#47045=CARTESIAN_POINT('Origin',(-2.91557726271063,0.,-3.02314558451372));
#47046=CARTESIAN_POINT('',(-3.02314558451372,1.,-2.91557726271063));
#47047=CARTESIAN_POINT('Origin',(0.,0.,0.));
#47048=CARTESIAN_POINT('',(-2.36531447826213,1.,-2.90994629141562));
#47049=CARTESIAN_POINT('Origin',(0.,1.,0.));
#47050=CARTESIAN_POINT('Ctrl Pts',(-2.36531447826213,1.,-2.90994629141562));
#47051=CARTESIAN_POINT('Ctrl Pts',(-2.36531447826213,0.666666666666667,
-2.90994629141562));
#47052=CARTESIAN_POINT('Ctrl Pts',(-2.36531447826213,0.333333333333333,
-2.90994629141562));
#47053=CARTESIAN_POINT('Ctrl Pts',(-2.36531447826213,-0.333333333333333,
-2.90994629141562));
#47054=CARTESIAN_POINT('Ctrl Pts',(-2.36531447826213,-0.666666666666667,
-2.90994629141562));
#47055=CARTESIAN_POINT('Ctrl Pts',(-2.36531447826213,-1.,-2.90994629141562));
#47056=CARTESIAN_POINT('Ctrl Pts',(-2.52982887637028,-1.,-3.35260583073571));
#47057=CARTESIAN_POINT('Ctrl Pts',(-2.52982887637028,1.,-3.35260583073571));
#47058=CARTESIAN_POINT('Ctrl Pts',(-2.52954136549357,-1.,-3.35105973714426));
#47059=CARTESIAN_POINT('Ctrl Pts',(-2.52954136549357,1.,-3.35105973714426));
#47060=CARTESIAN_POINT('Ctrl Pts',(-2.5289632161143,-1.,-3.34796903577628));
#47061=CARTESIAN_POINT('Ctrl Pts',(-2.5289632161143,1.,-3.34796903577628));
#47062=CARTESIAN_POINT('Ctrl Pts',(-2.52808660916879,-1.,-3.34333744117093));
#47063=CARTESIAN_POINT('Ctrl Pts',(-2.52808660916879,1.,-3.34333744117093));
#47064=CARTESIAN_POINT('Ctrl Pts',(-2.52689902691551,-1.,-3.33717090000955));
#47065=CARTESIAN_POINT('Ctrl Pts',(-2.52689902691551,1.,-3.33717090000955));
#47066=CARTESIAN_POINT('Ctrl Pts',(-2.52538321165774,-1.,-3.32947762189049));
#47067=CARTESIAN_POINT('Ctrl Pts',(-2.52538321165774,1.,-3.32947762189049));
#47068=CARTESIAN_POINT('Ctrl Pts',(-2.52383598396878,-1.,-3.32179931079521));
#47069=CARTESIAN_POINT('Ctrl Pts',(-2.52383598396878,1.,-3.32179931079521));
#47070=CARTESIAN_POINT('Ctrl Pts',(-2.52225724871375,-1.,-3.31413607874727));
#47071=CARTESIAN_POINT('Ctrl Pts',(-2.52225724871375,1.,-3.31413607874727));
#47072=CARTESIAN_POINT('Ctrl Pts',(-2.52064689568167,-1.,-3.30648808814986));
#47073=CARTESIAN_POINT('Ctrl Pts',(-2.52064689568167,1.,-3.30648808814986));
#47074=CARTESIAN_POINT('Ctrl Pts',(-2.51900480700548,-1.,-3.29885556387661));
#47075=CARTESIAN_POINT('Ctrl Pts',(-2.51900480700548,1.,-3.29885556387661));
#47076=CARTESIAN_POINT('Ctrl Pts',(-2.51733085123316,-1.,-3.2912387729863));
#47077=CARTESIAN_POINT('Ctrl Pts',(-2.51733085123316,1.,-3.2912387729863));
#47078=CARTESIAN_POINT('Ctrl Pts',(-2.51562487464215,-1.,-3.28363799702583));
#47079=CARTESIAN_POINT('Ctrl Pts',(-2.51562487464215,1.,-3.28363799702583));
#47080=CARTESIAN_POINT('Ctrl Pts',(-2.51388669270329,-1.,-3.27605350473048));
#47081=CARTESIAN_POINT('Ctrl Pts',(-2.51388669270329,1.,-3.27605350473048));
#47082=CARTESIAN_POINT('Ctrl Pts',(-2.51211608411539,-1.,-3.26848552888271));
#47083=CARTESIAN_POINT('Ctrl Pts',(-2.51211608411539,1.,-3.26848552888271));
#47084=CARTESIAN_POINT('Ctrl Pts',(-2.51031277813697,-1.,-3.26093423001716));
#47085=CARTESIAN_POINT('Ctrl Pts',(-2.51031277813697,1.,-3.26093423001716));
#47086=CARTESIAN_POINT('Ctrl Pts',(-2.50847647070936,-1.,-3.25339971461265));
#47087=CARTESIAN_POINT('Ctrl Pts',(-2.50847647070936,1.,-3.25339971461265));
#47088=CARTESIAN_POINT('Ctrl Pts',(-2.50660685940645,-1.,-3.24588208984042));
#47089=CARTESIAN_POINT('Ctrl Pts',(-2.50660685940645,1.,-3.24588208984042));
#47090=CARTESIAN_POINT('Ctrl Pts',(-2.50470367580078,-1.,-3.23838151080383));
#47091=CARTESIAN_POINT('Ctrl Pts',(-2.50470367580078,1.,-3.23838151080383));
#47092=CARTESIAN_POINT('Ctrl Pts',(-2.50276671338074,-1.,-3.23089822320596));
#47093=CARTESIAN_POINT('Ctrl Pts',(-2.50276671338074,1.,-3.23089822320596));
#47094=CARTESIAN_POINT('Ctrl Pts',(-2.5007958720187,-1.,-3.22343262620387));
#47095=CARTESIAN_POINT('Ctrl Pts',(-2.5007958720187,1.,-3.22343262620387));
#47096=CARTESIAN_POINT('Ctrl Pts',(-2.49879114599293,-1.,-3.21598526261157));
#47097=CARTESIAN_POINT('Ctrl Pts',(-2.49879114599293,1.,-3.21598526261157));
#47098=CARTESIAN_POINT('Ctrl Pts',(-2.49675252647298,-1.,-3.2085566984974));
#47099=CARTESIAN_POINT('Ctrl Pts',(-2.49675252647298,1.,-3.2085566984974));
#47100=CARTESIAN_POINT('Ctrl Pts',(-2.49467992057726,-1.,-3.20114742397549));
#47101=CARTESIAN_POINT('Ctrl Pts',(-2.49467992057726,1.,-3.20114742397549));
#47102=CARTESIAN_POINT('Ctrl Pts',(-2.4925730723986,-1.,-3.19375775555814));
#47103=CARTESIAN_POINT('Ctrl Pts',(-2.4925730723986,1.,-3.19375775555814));
#47104=CARTESIAN_POINT('Ctrl Pts',(-2.49043146334095,-1.,-3.18638771282315));
#47105=CARTESIAN_POINT('Ctrl Pts',(-2.49043146334095,1.,-3.18638771282315));
#47106=CARTESIAN_POINT('Ctrl Pts',(-2.48825428288243,-1.,-3.17903698136679));
#47107=CARTESIAN_POINT('Ctrl Pts',(-2.48825428288243,1.,-3.17903698136679));
#47108=CARTESIAN_POINT('Ctrl Pts',(-2.48604065348619,-1.,-3.17170518863357));
#47109=CARTESIAN_POINT('Ctrl Pts',(-2.48604065348619,1.,-3.17170518863357));
#47110=CARTESIAN_POINT('Ctrl Pts',(-2.48378981792739,-1.,-3.16439213290181));
#47111=CARTESIAN_POINT('Ctrl Pts',(-2.48378981792739,1.,-3.16439213290181));
#47112=CARTESIAN_POINT('Ctrl Pts',(-2.48150133566568,-1.,-3.15709802322735));
#47113=CARTESIAN_POINT('Ctrl Pts',(-2.48150133566568,1.,-3.15709802322735));
#47114=CARTESIAN_POINT('Ctrl Pts',(-2.47917529057016,-1.,-3.14982373241335));
#47115=CARTESIAN_POINT('Ctrl Pts',(-2.47917529057016,1.,-3.14982373241335));
#47116=CARTESIAN_POINT('Ctrl Pts',(-2.47681245356095,-1.,-3.14257099546531));
#47117=CARTESIAN_POINT('Ctrl Pts',(-2.47681245356095,1.,-3.14257099546531));
#47118=CARTESIAN_POINT('Ctrl Pts',(-2.47441378371923,-1.,-3.13534181229282));
#47119=CARTESIAN_POINT('Ctrl Pts',(-2.47441378371923,1.,-3.13534181229282));
#47120=CARTESIAN_POINT('Ctrl Pts',(-2.47197997765868,-1.,-3.12813790805948));
#47121=CARTESIAN_POINT('Ctrl Pts',(-2.47197997765868,1.,-3.12813790805948));
#47122=CARTESIAN_POINT('Ctrl Pts',(-2.4695109894747,-1.,-3.12096015766984));
#47123=CARTESIAN_POINT('Ctrl Pts',(-2.4695109894747,1.,-3.12096015766984));
#47124=CARTESIAN_POINT('Ctrl Pts',(-2.46700558843507,-1.,-3.11380805536124));
#47125=CARTESIAN_POINT('Ctrl Pts',(-2.46700558843507,1.,-3.11380805536124));
#47126=CARTESIAN_POINT('Ctrl Pts',(-2.46446082979645,-1.,-3.10667907901981));
#47127=CARTESIAN_POINT('Ctrl Pts',(-2.46446082979645,1.,-3.10667907901981));
#47128=CARTESIAN_POINT('Ctrl Pts',(-2.4618730850188,-1.,-3.09956993697048));
#47129=CARTESIAN_POINT('Ctrl Pts',(-2.4618730850188,1.,-3.09956993697048));
#47130=CARTESIAN_POINT('Ctrl Pts',(-2.45923912563875,-1.,-3.09247787931881));
#47131=CARTESIAN_POINT('Ctrl Pts',(-2.45923912563875,1.,-3.09247787931881));
#47132=CARTESIAN_POINT('Ctrl Pts',(-2.45655725437037,-1.,-3.08540206545313));
#47133=CARTESIAN_POINT('Ctrl Pts',(-2.45655725437037,1.,-3.08540206545313));
#47134=CARTESIAN_POINT('Ctrl Pts',(-2.45382826787795,-1.,-3.07834472886145));
#47135=CARTESIAN_POINT('Ctrl Pts',(-2.45382826787795,1.,-3.07834472886145));
#47136=CARTESIAN_POINT('Ctrl Pts',(-2.45105688854432,-1.,-3.0713129052131));
#47137=CARTESIAN_POINT('Ctrl Pts',(-2.45105688854432,1.,-3.0713129052131));
#47138=CARTESIAN_POINT('Ctrl Pts',(-2.44824970516558,-1.,-3.06431596421422));
#47139=CARTESIAN_POINT('Ctrl Pts',(-2.44824970516558,1.,-3.06431596421422));
#47140=CARTESIAN_POINT('Ctrl Pts',(-2.44541251892568,-1.,-3.05736242671521));
#47141=CARTESIAN_POINT('Ctrl Pts',(-2.44541251892568,1.,-3.05736242671521));
#47142=CARTESIAN_POINT('Ctrl Pts',(-2.44254768923109,-1.,-3.05045678021509));
#47143=CARTESIAN_POINT('Ctrl Pts',(-2.44254768923109,1.,-3.05045678021509));
#47144=CARTESIAN_POINT('Ctrl Pts',(-2.43965194061849,-1.,-3.04359685040545));
#47145=CARTESIAN_POINT('Ctrl Pts',(-2.43965194061849,1.,-3.04359685040545));
#47146=CARTESIAN_POINT('Ctrl Pts',(-2.43671278042394,-1.,-3.03676949672797));
#47147=CARTESIAN_POINT('Ctrl Pts',(-2.43671278042394,1.,-3.03676949672797));
#47148=CARTESIAN_POINT('Ctrl Pts',(-2.43371241361462,-1.,-3.02995534946946));
#47149=CARTESIAN_POINT('Ctrl Pts',(-2.43371241361462,1.,-3.02995534946946));
#47150=CARTESIAN_POINT('Ctrl Pts',(-2.43063415586615,-1.,-3.02313656035977));
#47151=CARTESIAN_POINT('Ctrl Pts',(-2.43063415586615,1.,-3.02313656035977));
#47152=CARTESIAN_POINT('Ctrl Pts',(-2.4274685626416,-1.,-3.01630420830494));
#47153=CARTESIAN_POINT('Ctrl Pts',(-2.4274685626416,1.,-3.01630420830494));
#47154=CARTESIAN_POINT('Ctrl Pts',(-2.42421849439625,-1.,-3.00946442616674));
#47155=CARTESIAN_POINT('Ctrl Pts',(-2.42421849439625,1.,-3.00946442616674));
#47156=CARTESIAN_POINT('Ctrl Pts',(-2.42090763946812,-1.,-3.00264868586038));
#47157=CARTESIAN_POINT('Ctrl Pts',(-2.42090763946812,1.,-3.00264868586038));
#47158=CARTESIAN_POINT('Ctrl Pts',(-2.4175732450056,-1.,-2.99590509293561));
#47159=CARTESIAN_POINT('Ctrl Pts',(-2.4175732450056,1.,-2.99590509293561));
#47160=CARTESIAN_POINT('Ctrl Pts',(-2.4142506419963,-1.,-2.98927983005851));
#47161=CARTESIAN_POINT('Ctrl Pts',(-2.4142506419963,1.,-2.98927983005851));
#47162=CARTESIAN_POINT('Ctrl Pts',(-2.41095909342591,-1.,-2.98280015815132));
#47163=CARTESIAN_POINT('Ctrl Pts',(-2.41095909342591,1.,-2.98280015815132));
#47164=CARTESIAN_POINT('Ctrl Pts',(-2.40768975073691,-1.,-2.97646002822395));
#47165=CARTESIAN_POINT('Ctrl Pts',(-2.40768975073691,1.,-2.97646002822395));
#47166=CARTESIAN_POINT('Ctrl Pts',(-2.40438604734848,-1.,-2.97019641312272));
#47167=CARTESIAN_POINT('Ctrl Pts',(-2.40438604734848,1.,-2.97019641312272));
#47168=CARTESIAN_POINT('Ctrl Pts',(-2.40095565711535,-1.,-2.96390432240181));
#47169=CARTESIAN_POINT('Ctrl Pts',(-2.40095565711535,1.,-2.96390432240181));
#47170=CARTESIAN_POINT('Ctrl Pts',(-2.39730553974412,-1.,-2.95748006482811));
#47171=CARTESIAN_POINT('Ctrl Pts',(-2.39730553974412,1.,-2.95748006482811));
#47172=CARTESIAN_POINT('Ctrl Pts',(-2.39337207631613,-1.,-2.95085857128372));
#47173=CARTESIAN_POINT('Ctrl Pts',(-2.39337207631613,1.,-2.95085857128372));
#47174=CARTESIAN_POINT('Ctrl Pts',(-2.38914929090806,-1.,-2.94404820669135));
#47175=CARTESIAN_POINT('Ctrl Pts',(-2.38914929090806,1.,-2.94404820669135));
#47176=CARTESIAN_POINT('Ctrl Pts',(-2.38472771516476,-1.,-2.93717903280599));
#47177=CARTESIAN_POINT('Ctrl Pts',(-2.38472771516476,1.,-2.93717903280599));
#47178=CARTESIAN_POINT('Ctrl Pts',(-2.3802898958232,-1.,-2.93049643640517));
#47179=CARTESIAN_POINT('Ctrl Pts',(-2.3802898958232,1.,-2.93049643640517));
#47180=CARTESIAN_POINT('Ctrl Pts',(-2.37606510524271,-1.,-2.92430340582912));
#47181=CARTESIAN_POINT('Ctrl Pts',(-2.37606510524271,1.,-2.92430340582912));
#47182=CARTESIAN_POINT('Ctrl Pts',(-2.37229381109939,-1.,-2.9189150379156));
#47183=CARTESIAN_POINT('Ctrl Pts',(-2.37229381109939,1.,-2.9189150379156));
#47184=CARTESIAN_POINT('Ctrl Pts',(-2.36919161373074,-1.,-2.91461249883016));
#47185=CARTESIAN_POINT('Ctrl Pts',(-2.36919161373074,1.,-2.91461249883016));
#47186=CARTESIAN_POINT('Ctrl Pts',(-2.36690501170317,-1.,-2.9115863784165));
#47187=CARTESIAN_POINT('Ctrl Pts',(-2.36690501170317,1.,-2.9115863784165));
#47188=CARTESIAN_POINT('Ctrl Pts',(-2.36578327194396,-1.,-2.91025813829606));
#47189=CARTESIAN_POINT('Ctrl Pts',(-2.36578327194396,1.,-2.91025813829606));
#47190=CARTESIAN_POINT('Ctrl Pts',(-2.36535052956704,-1.,-2.90989022547738));
#47191=CARTESIAN_POINT('Ctrl Pts',(-2.36535052956704,1.,-2.90989022547738));
#47192=CARTESIAN_POINT('Ctrl Pts',(-2.36524348105023,-1.,-2.90992398626098));
#47193=CARTESIAN_POINT('Ctrl Pts',(-2.36524348105023,1.,-2.90992398626098));
#47194=CARTESIAN_POINT('Ctrl Pts',(-2.36523532225181,-1.,-2.91001063062876));
#47195=CARTESIAN_POINT('Ctrl Pts',(-2.36523532225181,1.,-2.91001063062876));
#47196=CARTESIAN_POINT('',(-2.52982887637028,1.,-3.35260583073571));
#47197=CARTESIAN_POINT('Ctrl Pts',(-2.52982887637028,1.,-3.35260583073571));
#47198=CARTESIAN_POINT('Ctrl Pts',(-2.52954136549357,1.,-3.35105973714426));
#47199=CARTESIAN_POINT('Ctrl Pts',(-2.5289632161143,1.,-3.34796903577628));
#47200=CARTESIAN_POINT('Ctrl Pts',(-2.52808660916879,1.,-3.34333744117093));
#47201=CARTESIAN_POINT('Ctrl Pts',(-2.52689902691551,1.,-3.33717090000955));
#47202=CARTESIAN_POINT('Ctrl Pts',(-2.52538321165774,1.,-3.32947762189049));
#47203=CARTESIAN_POINT('Ctrl Pts',(-2.52383598396878,1.,-3.32179931079521));
#47204=CARTESIAN_POINT('Ctrl Pts',(-2.52225724871375,1.,-3.31413607874727));
#47205=CARTESIAN_POINT('Ctrl Pts',(-2.52064689568167,1.,-3.30648808814986));
#47206=CARTESIAN_POINT('Ctrl Pts',(-2.51900480700548,1.,-3.29885556387661));
#47207=CARTESIAN_POINT('Ctrl Pts',(-2.51733085123316,1.,-3.2912387729863));
#47208=CARTESIAN_POINT('Ctrl Pts',(-2.51562487464215,1.,-3.28363799702583));
#47209=CARTESIAN_POINT('Ctrl Pts',(-2.51388669270329,1.,-3.27605350473048));
#47210=CARTESIAN_POINT('Ctrl Pts',(-2.51211608411539,1.,-3.26848552888271));
#47211=CARTESIAN_POINT('Ctrl Pts',(-2.51031277813697,1.,-3.26093423001716));
#47212=CARTESIAN_POINT('Ctrl Pts',(-2.50847647070936,1.,-3.25339971461265));
#47213=CARTESIAN_POINT('Ctrl Pts',(-2.50660685940645,1.,-3.24588208984042));
#47214=CARTESIAN_POINT('Ctrl Pts',(-2.50470367580078,1.,-3.23838151080383));
#47215=CARTESIAN_POINT('Ctrl Pts',(-2.50276671338074,1.,-3.23089822320596));
#47216=CARTESIAN_POINT('Ctrl Pts',(-2.5007958720187,1.,-3.22343262620387));
#47217=CARTESIAN_POINT('Ctrl Pts',(-2.49879114599293,1.,-3.21598526261157));
#47218=CARTESIAN_POINT('Ctrl Pts',(-2.49675252647298,1.,-3.2085566984974));
#47219=CARTESIAN_POINT('Ctrl Pts',(-2.49467992057726,1.,-3.20114742397549));
#47220=CARTESIAN_POINT('Ctrl Pts',(-2.4925730723986,1.,-3.19375775555814));
#47221=CARTESIAN_POINT('Ctrl Pts',(-2.49043146334095,1.,-3.18638771282315));
#47222=CARTESIAN_POINT('Ctrl Pts',(-2.48825428288243,1.,-3.17903698136679));
#47223=CARTESIAN_POINT('Ctrl Pts',(-2.48604065348619,1.,-3.17170518863357));
#47224=CARTESIAN_POINT('Ctrl Pts',(-2.48378981792739,1.,-3.16439213290181));
#47225=CARTESIAN_POINT('Ctrl Pts',(-2.48150133566568,1.,-3.15709802322735));
#47226=CARTESIAN_POINT('Ctrl Pts',(-2.47917529057016,1.,-3.14982373241335));
#47227=CARTESIAN_POINT('Ctrl Pts',(-2.47681245356095,1.,-3.14257099546531));
#47228=CARTESIAN_POINT('Ctrl Pts',(-2.47441378371923,1.,-3.13534181229282));
#47229=CARTESIAN_POINT('Ctrl Pts',(-2.47197997765868,1.,-3.12813790805948));
#47230=CARTESIAN_POINT('Ctrl Pts',(-2.4695109894747,1.,-3.12096015766984));
#47231=CARTESIAN_POINT('Ctrl Pts',(-2.46700558843507,1.,-3.11380805536124));
#47232=CARTESIAN_POINT('Ctrl Pts',(-2.46446082979645,1.,-3.10667907901981));
#47233=CARTESIAN_POINT('Ctrl Pts',(-2.4618730850188,1.,-3.09956993697048));
#47234=CARTESIAN_POINT('Ctrl Pts',(-2.45923912563875,1.,-3.09247787931881));
#47235=CARTESIAN_POINT('Ctrl Pts',(-2.45655725437037,1.,-3.08540206545313));
#47236=CARTESIAN_POINT('Ctrl Pts',(-2.45382826787795,1.,-3.07834472886145));
#47237=CARTESIAN_POINT('Ctrl Pts',(-2.45105688854432,1.,-3.0713129052131));
#47238=CARTESIAN_POINT('Ctrl Pts',(-2.44824970516558,1.,-3.06431596421422));
#47239=CARTESIAN_POINT('Ctrl Pts',(-2.44541251892568,1.,-3.05736242671521));
#47240=CARTESIAN_POINT('Ctrl Pts',(-2.44254768923109,1.,-3.05045678021509));
#47241=CARTESIAN_POINT('Ctrl Pts',(-2.43965194061849,1.,-3.04359685040545));
#47242=CARTESIAN_POINT('Ctrl Pts',(-2.43671278042394,1.,-3.03676949672797));
#47243=CARTESIAN_POINT('Ctrl Pts',(-2.43371241361462,1.,-3.02995534946946));
#47244=CARTESIAN_POINT('Ctrl Pts',(-2.43063415586615,1.,-3.02313656035977));
#47245=CARTESIAN_POINT('Ctrl Pts',(-2.4274685626416,1.,-3.01630420830494));
#47246=CARTESIAN_POINT('Ctrl Pts',(-2.42421849439625,1.,-3.00946442616674));
#47247=CARTESIAN_POINT('Ctrl Pts',(-2.42090763946812,1.,-3.00264868586038));
#47248=CARTESIAN_POINT('Ctrl Pts',(-2.4175732450056,1.,-2.99590509293561));
#47249=CARTESIAN_POINT('Ctrl Pts',(-2.4142506419963,1.,-2.98927983005851));
#47250=CARTESIAN_POINT('Ctrl Pts',(-2.41095909342591,1.,-2.98280015815132));
#47251=CARTESIAN_POINT('Ctrl Pts',(-2.40768975073691,1.,-2.97646002822395));
#47252=CARTESIAN_POINT('Ctrl Pts',(-2.40438604734848,1.,-2.97019641312272));
#47253=CARTESIAN_POINT('Ctrl Pts',(-2.40095565711535,1.,-2.96390432240181));
#47254=CARTESIAN_POINT('Ctrl Pts',(-2.39730553974412,1.,-2.95748006482811));
#47255=CARTESIAN_POINT('Ctrl Pts',(-2.39337207631613,1.,-2.95085857128372));
#47256=CARTESIAN_POINT('Ctrl Pts',(-2.38914929090806,1.,-2.94404820669135));
#47257=CARTESIAN_POINT('Ctrl Pts',(-2.38472771516476,1.,-2.93717903280599));
#47258=CARTESIAN_POINT('Ctrl Pts',(-2.3802898958232,1.,-2.93049643640517));
#47259=CARTESIAN_POINT('Ctrl Pts',(-2.37606510524271,1.,-2.92430340582912));
#47260=CARTESIAN_POINT('Ctrl Pts',(-2.37229381109939,1.,-2.9189150379156));
#47261=CARTESIAN_POINT('Ctrl Pts',(-2.36919161373074,1.,-2.91461249883016));
#47262=CARTESIAN_POINT('Ctrl Pts',(-2.36707658451709,1.,-2.91181344022628));
#47263=CARTESIAN_POINT('Ctrl Pts',(-2.36599991765853,1.,-2.91051690822262));
#47264=CARTESIAN_POINT('Ctrl Pts',(-2.36553202948741,1.,-2.9100577052777));
#47265=CARTESIAN_POINT('Ctrl Pts',(-2.3653621118858,1.,-2.90995756655559));
#47266=CARTESIAN_POINT('Ctrl Pts',(-2.36531447826213,1.,-2.90994629141563));
#47267=CARTESIAN_POINT('',(-2.52982887637028,0.,-3.35260583073571));
#47268=CARTESIAN_POINT('Ctrl Pts',(-2.03668666247593,-1.,-3.1487152044751));
#47269=CARTESIAN_POINT('Ctrl Pts',(-2.03668666247593,1.,-3.1487152044751));
#47270=CARTESIAN_POINT('Ctrl Pts',(-2.03660173757879,-1.,-3.14869618937258));
#47271=CARTESIAN_POINT('Ctrl Pts',(-2.03660173757879,1.,-3.14869618937258));
#47272=CARTESIAN_POINT('Ctrl Pts',(-2.03653654935592,-1.,-3.14878756590812));
#47273=CARTESIAN_POINT('Ctrl Pts',(-2.03653654935592,1.,-3.14878756590812));
#47274=CARTESIAN_POINT('Ctrl Pts',(-2.03675273049189,-1.,-3.14931281968048));
#47275=CARTESIAN_POINT('Ctrl Pts',(-2.03675273049189,1.,-3.14931281968048));
#47276=CARTESIAN_POINT('Ctrl Pts',(-2.03766932526445,-1.,-3.15079010635742));
#47277=CARTESIAN_POINT('Ctrl Pts',(-2.03766932526445,1.,-3.15079010635742));
#47278=CARTESIAN_POINT('Ctrl Pts',(-2.03984073791519,-1.,-3.15389991674792));
#47279=CARTESIAN_POINT('Ctrl Pts',(-2.03984073791519,1.,-3.15389991674792));
#47280=CARTESIAN_POINT('Ctrl Pts',(-2.04297406404027,-1.,-3.15817983946367));
#47281=CARTESIAN_POINT('Ctrl Pts',(-2.04297406404027,1.,-3.15817983946367));
#47282=CARTESIAN_POINT('Ctrl Pts',(-2.04693331247446,-1.,-3.16343165058912));
#47283=CARTESIAN_POINT('Ctrl Pts',(-2.04693331247446,1.,-3.16343165058912));
#47284=CARTESIAN_POINT('Ctrl Pts',(-2.05151770247233,-1.,-3.16936341689527));
#47285=CARTESIAN_POINT('Ctrl Pts',(-2.05151770247233,1.,-3.16936341689527));
#47286=CARTESIAN_POINT('Ctrl Pts',(-2.05650186773132,-1.,-3.17564906975371));
#47287=CARTESIAN_POINT('Ctrl Pts',(-2.05650186773132,1.,-3.17564906975371));
#47288=CARTESIAN_POINT('Ctrl Pts',(-2.06166849827101,-1.,-3.18197692964614));
#47289=CARTESIAN_POINT('Ctrl Pts',(-2.06166849827101,1.,-3.18197692964614));
#47290=CARTESIAN_POINT('Ctrl Pts',(-2.06684062744112,-1.,-3.18809755562368));
#47291=CARTESIAN_POINT('Ctrl Pts',(-2.06684062744112,1.,-3.18809755562368));
#47292=CARTESIAN_POINT('Ctrl Pts',(-2.07192253497857,-1.,-3.19388465568252));
#47293=CARTESIAN_POINT('Ctrl Pts',(-2.07192253497857,1.,-3.19388465568252));
#47294=CARTESIAN_POINT('Ctrl Pts',(-2.07690441870722,-1.,-3.19934132836019));
#47295=CARTESIAN_POINT('Ctrl Pts',(-2.07690441870722,1.,-3.19934132836019));
#47296=CARTESIAN_POINT('Ctrl Pts',(-2.08182850370878,-1.,-3.2045481863073));
#47297=CARTESIAN_POINT('Ctrl Pts',(-2.08182850370878,1.,-3.2045481863073));
#47298=CARTESIAN_POINT('Ctrl Pts',(-2.08676465517455,-1.,-3.20962575845463));
#47299=CARTESIAN_POINT('Ctrl Pts',(-2.08676465517455,1.,-3.20962575845463));
#47300=CARTESIAN_POINT('Ctrl Pts',(-2.09178419460443,-1.,-3.21469429601654));
#47301=CARTESIAN_POINT('Ctrl Pts',(-2.09178419460443,1.,-3.21469429601654));
#47302=CARTESIAN_POINT('Ctrl Pts',(-2.09692958434895,-1.,-3.21982707347009));
#47303=CARTESIAN_POINT('Ctrl Pts',(-2.09692958434895,1.,-3.21982707347009));
#47304=CARTESIAN_POINT('Ctrl Pts',(-2.10220384298492,-1.,-3.22503437553434));
#47305=CARTESIAN_POINT('Ctrl Pts',(-2.10220384298492,1.,-3.22503437553434));
#47306=CARTESIAN_POINT('Ctrl Pts',(-2.10758699642451,-1.,-3.23028945793289));
#47307=CARTESIAN_POINT('Ctrl Pts',(-2.10758699642451,1.,-3.23028945793289));
#47308=CARTESIAN_POINT('Ctrl Pts',(-2.11304604021773,-1.,-3.23554444767099));
#47309=CARTESIAN_POINT('Ctrl Pts',(-2.11304604021773,1.,-3.23554444767099));
#47310=CARTESIAN_POINT('Ctrl Pts',(-2.11854673326979,-1.,-3.24074905517293));
#47311=CARTESIAN_POINT('Ctrl Pts',(-2.11854673326979,1.,-3.24074905517293));
#47312=CARTESIAN_POINT('Ctrl Pts',(-2.12406646410962,-1.,-3.24587102613376));
#47313=CARTESIAN_POINT('Ctrl Pts',(-2.12406646410962,1.,-3.24587102613376));
#47314=CARTESIAN_POINT('Ctrl Pts',(-2.12960028396832,-1.,-3.25090574494028));
#47315=CARTESIAN_POINT('Ctrl Pts',(-2.12960028396832,1.,-3.25090574494028));
#47316=CARTESIAN_POINT('Ctrl Pts',(-2.13515375878803,-1.,-3.25586495065054));
#47317=CARTESIAN_POINT('Ctrl Pts',(-2.13515375878803,1.,-3.25586495065054));
#47318=CARTESIAN_POINT('Ctrl Pts',(-2.14073870754264,-1.,-3.26077002641879));
#47319=CARTESIAN_POINT('Ctrl Pts',(-2.14073870754264,1.,-3.26077002641879));
#47320=CARTESIAN_POINT('Ctrl Pts',(-2.1463680529566,-1.,-3.26564388189759));
#47321=CARTESIAN_POINT('Ctrl Pts',(-2.1463680529566,1.,-3.26564388189759));
#47322=CARTESIAN_POINT('Ctrl Pts',(-2.15205043199808,-1.,-3.27050245897228));
#47323=CARTESIAN_POINT('Ctrl Pts',(-2.15205043199808,1.,-3.27050245897228));
#47324=CARTESIAN_POINT('Ctrl Pts',(-2.15778690038347,-1.,-3.27534954469187));
#47325=CARTESIAN_POINT('Ctrl Pts',(-2.15778690038347,1.,-3.27534954469187));
#47326=CARTESIAN_POINT('Ctrl Pts',(-2.16357391934425,-1.,-3.280181508414));
#47327=CARTESIAN_POINT('Ctrl Pts',(-2.16357391934425,1.,-3.280181508414));
#47328=CARTESIAN_POINT('Ctrl Pts',(-2.16940517773455,-1.,-3.28499019979724));
#47329=CARTESIAN_POINT('Ctrl Pts',(-2.16940517773455,1.,-3.28499019979724));
#47330=CARTESIAN_POINT('Ctrl Pts',(-2.17527380048423,-1.,-3.28976645712568));
#47331=CARTESIAN_POINT('Ctrl Pts',(-2.17527380048423,1.,-3.28976645712568));
#47332=CARTESIAN_POINT('Ctrl Pts',(-2.18117455557065,-1.,-3.2945036150049));
#47333=CARTESIAN_POINT('Ctrl Pts',(-2.18117455557065,1.,-3.2945036150049));
#47334=CARTESIAN_POINT('Ctrl Pts',(-2.18710556500327,-1.,-3.29920022557639));
#47335=CARTESIAN_POINT('Ctrl Pts',(-2.18710556500327,1.,-3.29920022557639));
#47336=CARTESIAN_POINT('Ctrl Pts',(-2.19306710376111,-1.,-3.30385816281831));
#47337=CARTESIAN_POINT('Ctrl Pts',(-2.19306710376111,1.,-3.30385816281831));
#47338=CARTESIAN_POINT('Ctrl Pts',(-2.19906078949923,-1.,-3.30848134694595));
#47339=CARTESIAN_POINT('Ctrl Pts',(-2.19906078949923,1.,-3.30848134694595));
#47340=CARTESIAN_POINT('Ctrl Pts',(-2.20508863150607,-1.,-3.31307424608949));
#47341=CARTESIAN_POINT('Ctrl Pts',(-2.20508863150607,1.,-3.31307424608949));
#47342=CARTESIAN_POINT('Ctrl Pts',(-2.21115211847875,-1.,-3.31764044024235));
#47343=CARTESIAN_POINT('Ctrl Pts',(-2.21115211847875,1.,-3.31764044024235));
#47344=CARTESIAN_POINT('Ctrl Pts',(-2.21725135110898,-1.,-3.32218125618968));
#47345=CARTESIAN_POINT('Ctrl Pts',(-2.21725135110898,1.,-3.32218125618968));
#47346=CARTESIAN_POINT('Ctrl Pts',(-2.22338548312772,-1.,-3.3266964672289));
#47347=CARTESIAN_POINT('Ctrl Pts',(-2.22338548312772,1.,-3.3266964672289));
#47348=CARTESIAN_POINT('Ctrl Pts',(-2.22955308907233,-1.,-3.33118487773611));
#47349=CARTESIAN_POINT('Ctrl Pts',(-2.22955308907233,1.,-3.33118487773611));
#47350=CARTESIAN_POINT('Ctrl Pts',(-2.23575256328812,-1.,-3.33564495756482));
#47351=CARTESIAN_POINT('Ctrl Pts',(-2.23575256328812,1.,-3.33564495756482));
#47352=CARTESIAN_POINT('Ctrl Pts',(-2.24198249391422,-1.,-3.34007543738025));
#47353=CARTESIAN_POINT('Ctrl Pts',(-2.24198249391422,1.,-3.34007543738025));
#47354=CARTESIAN_POINT('Ctrl Pts',(-2.24824207678256,-1.,-3.34447596770723));
#47355=CARTESIAN_POINT('Ctrl Pts',(-2.24824207678256,1.,-3.34447596770723));
#47356=CARTESIAN_POINT('Ctrl Pts',(-2.25453097693483,-1.,-3.34884690292285));
#47357=CARTESIAN_POINT('Ctrl Pts',(-2.25453097693483,1.,-3.34884690292285));
#47358=CARTESIAN_POINT('Ctrl Pts',(-2.26084915222449,-1.,-3.35318902552626));
#47359=CARTESIAN_POINT('Ctrl Pts',(-2.26084915222449,1.,-3.35318902552626));
#47360=CARTESIAN_POINT('Ctrl Pts',(-2.2671966857991,-1.,-3.35750328523061));
#47361=CARTESIAN_POINT('Ctrl Pts',(-2.2671966857991,1.,-3.35750328523061));
#47362=CARTESIAN_POINT('Ctrl Pts',(-2.2735736262093,-1.,-3.36179055004409));
#47363=CARTESIAN_POINT('Ctrl Pts',(-2.2735736262093,1.,-3.36179055004409));
#47364=CARTESIAN_POINT('Ctrl Pts',(-2.27997979458037,-1.,-3.36605130713076));
#47365=CARTESIAN_POINT('Ctrl Pts',(-2.27997979458037,1.,-3.36605130713076));
#47366=CARTESIAN_POINT('Ctrl Pts',(-2.28641481081137,-1.,-3.37028570206488));
#47367=CARTESIAN_POINT('Ctrl Pts',(-2.28641481081137,1.,-3.37028570206488));
#47368=CARTESIAN_POINT('Ctrl Pts',(-2.29287818007393,-1.,-3.37449367172826));
#47369=CARTESIAN_POINT('Ctrl Pts',(-2.29287818007393,1.,-3.37449367172826));
#47370=CARTESIAN_POINT('Ctrl Pts',(-2.29936936127624,-1.,-3.37867504959433));
#47371=CARTESIAN_POINT('Ctrl Pts',(-2.29936936127624,1.,-3.37867504959433));
#47372=CARTESIAN_POINT('Ctrl Pts',(-2.30588783640343,-1.,-3.3828296733661));
#47373=CARTESIAN_POINT('Ctrl Pts',(-2.30588783640343,1.,-3.3828296733661));
#47374=CARTESIAN_POINT('Ctrl Pts',(-2.31243319489367,-1.,-3.38695751492462));
#47375=CARTESIAN_POINT('Ctrl Pts',(-2.31243319489367,1.,-3.38695751492462));
#47376=CARTESIAN_POINT('Ctrl Pts',(-2.31900513925424,-1.,-3.39105869474822));
#47377=CARTESIAN_POINT('Ctrl Pts',(-2.31900513925424,1.,-3.39105869474822));
#47378=CARTESIAN_POINT('Ctrl Pts',(-2.3256034390248,-1.,-3.39513342019756));
#47379=CARTESIAN_POINT('Ctrl Pts',(-2.3256034390248,1.,-3.39513342019756));
#47380=CARTESIAN_POINT('Ctrl Pts',(-2.33222789882489,-1.,-3.39918194577956));
#47381=CARTESIAN_POINT('Ctrl Pts',(-2.33222789882489,1.,-3.39918194577956));
#47382=CARTESIAN_POINT('Ctrl Pts',(-2.33887832342782,-1.,-3.40320452776743));
#47383=CARTESIAN_POINT('Ctrl Pts',(-2.33887832342782,1.,-3.40320452776743));
#47384=CARTESIAN_POINT('Ctrl Pts',(-2.34555447649188,-1.,-3.40720137404297));
#47385=CARTESIAN_POINT('Ctrl Pts',(-2.34555447649188,1.,-3.40720137404297));
#47386=CARTESIAN_POINT('Ctrl Pts',(-2.35225606824109,-1.,-3.41117262314119));
#47387=CARTESIAN_POINT('Ctrl Pts',(-2.35225606824109,1.,-3.41117262314119));
#47388=CARTESIAN_POINT('Ctrl Pts',(-2.35898278606946,-1.,-3.41511836751469));
#47389=CARTESIAN_POINT('Ctrl Pts',(-2.35898278606946,1.,-3.41511836751469));
#47390=CARTESIAN_POINT('Ctrl Pts',(-2.36573431470642,-1.,-3.41903866635852));
#47391=CARTESIAN_POINT('Ctrl Pts',(-2.36573431470642,1.,-3.41903866635852));
#47392=CARTESIAN_POINT('Ctrl Pts',(-2.37251035954292,-1.,-3.42293356216511));
#47393=CARTESIAN_POINT('Ctrl Pts',(-2.37251035954292,1.,-3.42293356216511));
#47394=CARTESIAN_POINT('Ctrl Pts',(-2.37931067028926,-1.,-3.42680309754399));
#47395=CARTESIAN_POINT('Ctrl Pts',(-2.37931067028926,1.,-3.42680309754399));
#47396=CARTESIAN_POINT('Ctrl Pts',(-2.38613505843552,-1.,-3.4306473271292));
#47397=CARTESIAN_POINT('Ctrl Pts',(-2.38613505843552,1.,-3.4306473271292));
#47398=CARTESIAN_POINT('Ctrl Pts',(-2.39298338804493,-1.,-3.4344663067854));
#47399=CARTESIAN_POINT('Ctrl Pts',(-2.39298338804493,1.,-3.4344663067854));
#47400=CARTESIAN_POINT('Ctrl Pts',(-2.39848113410292,-1.,-3.43750133064416));
#47401=CARTESIAN_POINT('Ctrl Pts',(-2.39848113410292,1.,-3.43750133064416));
#47402=CARTESIAN_POINT('Ctrl Pts',(-2.40261515589405,-1.,-3.43976627484234));
#47403=CARTESIAN_POINT('Ctrl Pts',(-2.40261515589405,1.,-3.43976627484234));
#47404=CARTESIAN_POINT('Ctrl Pts',(-2.4053759295909,-1.,-3.44127120683039));
#47405=CARTESIAN_POINT('Ctrl Pts',(-2.4053759295909,1.,-3.44127120683039));
#47406=CARTESIAN_POINT('Ctrl Pts',(-2.40675750623143,-1.,-3.44202241512147));
#47407=CARTESIAN_POINT('Ctrl Pts',(-2.40675750623143,1.,-3.44202241512147));
#47408=CARTESIAN_POINT('',(-2.03660101169714,1.,-3.14877060440328));
#47409=CARTESIAN_POINT('Ctrl Pts',(-2.03660101169715,-1.,-3.14877060440327));
#47410=CARTESIAN_POINT('Ctrl Pts',(-2.03660101169715,-0.666666666666667,
-3.14877060440327));
#47411=CARTESIAN_POINT('Ctrl Pts',(-2.03660101169715,-0.333333333333333,
-3.14877060440327));
#47412=CARTESIAN_POINT('Ctrl Pts',(-2.03660101169715,0.333333333333333,
-3.14877060440327));
#47413=CARTESIAN_POINT('Ctrl Pts',(-2.03660101169715,0.666666666666667,
-3.14877060440327));
#47414=CARTESIAN_POINT('Ctrl Pts',(-2.03660101169715,1.,-3.14877060440327));
#47415=CARTESIAN_POINT('',(-2.40675750623143,1.,-3.44202241512147));
#47416=CARTESIAN_POINT('',(-2.40675750623143,0.,-3.44202241512147));
#47417=CARTESIAN_POINT('Ctrl Pts',(-2.03660101169715,1.,-3.14877060440328));
#47418=CARTESIAN_POINT('Ctrl Pts',(-2.03659701539259,1.,-3.14881939088124));
#47419=CARTESIAN_POINT('Ctrl Pts',(-2.03663974554932,1.,-3.1490119366901));
#47420=CARTESIAN_POINT('Ctrl Pts',(-2.03693188810545,1.,-3.14959882629805));
#47421=CARTESIAN_POINT('Ctrl Pts',(-2.03783225495961,1.,-3.15102344775328));
#47422=CARTESIAN_POINT('Ctrl Pts',(-2.03984073791519,1.,-3.15389991674792));
#47423=CARTESIAN_POINT('Ctrl Pts',(-2.04297406404027,1.,-3.15817983946367));
#47424=CARTESIAN_POINT('Ctrl Pts',(-2.04693331247446,1.,-3.16343165058912));
#47425=CARTESIAN_POINT('Ctrl Pts',(-2.05151770247233,1.,-3.16936341689527));
#47426=CARTESIAN_POINT('Ctrl Pts',(-2.05650186773132,1.,-3.17564906975371));
#47427=CARTESIAN_POINT('Ctrl Pts',(-2.06166849827101,1.,-3.18197692964614));
#47428=CARTESIAN_POINT('Ctrl Pts',(-2.06684062744112,1.,-3.18809755562368));
#47429=CARTESIAN_POINT('Ctrl Pts',(-2.07192253497857,1.,-3.19388465568252));
#47430=CARTESIAN_POINT('Ctrl Pts',(-2.07690441870722,1.,-3.19934132836019));
#47431=CARTESIAN_POINT('Ctrl Pts',(-2.08182850370878,1.,-3.2045481863073));
#47432=CARTESIAN_POINT('Ctrl Pts',(-2.08676465517455,1.,-3.20962575845463));
#47433=CARTESIAN_POINT('Ctrl Pts',(-2.09178419460443,1.,-3.21469429601654));
#47434=CARTESIAN_POINT('Ctrl Pts',(-2.09692958434895,1.,-3.21982707347009));
#47435=CARTESIAN_POINT('Ctrl Pts',(-2.10220384298492,1.,-3.22503437553434));
#47436=CARTESIAN_POINT('Ctrl Pts',(-2.10758699642451,1.,-3.23028945793289));
#47437=CARTESIAN_POINT('Ctrl Pts',(-2.11304604021773,1.,-3.23554444767099));
#47438=CARTESIAN_POINT('Ctrl Pts',(-2.11854673326979,1.,-3.24074905517293));
#47439=CARTESIAN_POINT('Ctrl Pts',(-2.12406646410962,1.,-3.24587102613376));
#47440=CARTESIAN_POINT('Ctrl Pts',(-2.12960028396832,1.,-3.25090574494028));
#47441=CARTESIAN_POINT('Ctrl Pts',(-2.13515375878803,1.,-3.25586495065054));
#47442=CARTESIAN_POINT('Ctrl Pts',(-2.14073870754264,1.,-3.26077002641879));
#47443=CARTESIAN_POINT('Ctrl Pts',(-2.1463680529566,1.,-3.26564388189759));
#47444=CARTESIAN_POINT('Ctrl Pts',(-2.15205043199808,1.,-3.27050245897228));
#47445=CARTESIAN_POINT('Ctrl Pts',(-2.15778690038347,1.,-3.27534954469187));
#47446=CARTESIAN_POINT('Ctrl Pts',(-2.16357391934425,1.,-3.280181508414));
#47447=CARTESIAN_POINT('Ctrl Pts',(-2.16940517773455,1.,-3.28499019979724));
#47448=CARTESIAN_POINT('Ctrl Pts',(-2.17527380048423,1.,-3.28976645712568));
#47449=CARTESIAN_POINT('Ctrl Pts',(-2.18117455557065,1.,-3.2945036150049));
#47450=CARTESIAN_POINT('Ctrl Pts',(-2.18710556500327,1.,-3.29920022557639));
#47451=CARTESIAN_POINT('Ctrl Pts',(-2.19306710376111,1.,-3.30385816281831));
#47452=CARTESIAN_POINT('Ctrl Pts',(-2.19906078949923,1.,-3.30848134694595));
#47453=CARTESIAN_POINT('Ctrl Pts',(-2.20508863150607,1.,-3.31307424608949));
#47454=CARTESIAN_POINT('Ctrl Pts',(-2.21115211847875,1.,-3.31764044024235));
#47455=CARTESIAN_POINT('Ctrl Pts',(-2.21725135110898,1.,-3.32218125618968));
#47456=CARTESIAN_POINT('Ctrl Pts',(-2.22338548312772,1.,-3.3266964672289));
#47457=CARTESIAN_POINT('Ctrl Pts',(-2.22955308907233,1.,-3.33118487773611));
#47458=CARTESIAN_POINT('Ctrl Pts',(-2.23575256328812,1.,-3.33564495756482));
#47459=CARTESIAN_POINT('Ctrl Pts',(-2.24198249391422,1.,-3.34007543738025));
#47460=CARTESIAN_POINT('Ctrl Pts',(-2.24824207678256,1.,-3.34447596770723));
#47461=CARTESIAN_POINT('Ctrl Pts',(-2.25453097693483,1.,-3.34884690292285));
#47462=CARTESIAN_POINT('Ctrl Pts',(-2.26084915222449,1.,-3.35318902552626));
#47463=CARTESIAN_POINT('Ctrl Pts',(-2.2671966857991,1.,-3.35750328523061));
#47464=CARTESIAN_POINT('Ctrl Pts',(-2.2735736262093,1.,-3.36179055004409));
#47465=CARTESIAN_POINT('Ctrl Pts',(-2.27997979458037,1.,-3.36605130713076));
#47466=CARTESIAN_POINT('Ctrl Pts',(-2.28641481081137,1.,-3.37028570206488));
#47467=CARTESIAN_POINT('Ctrl Pts',(-2.29287818007393,1.,-3.37449367172826));
#47468=CARTESIAN_POINT('Ctrl Pts',(-2.29936936127624,1.,-3.37867504959433));
#47469=CARTESIAN_POINT('Ctrl Pts',(-2.30588783640343,1.,-3.3828296733661));
#47470=CARTESIAN_POINT('Ctrl Pts',(-2.31243319489367,1.,-3.38695751492462));
#47471=CARTESIAN_POINT('Ctrl Pts',(-2.31900513925424,1.,-3.39105869474822));
#47472=CARTESIAN_POINT('Ctrl Pts',(-2.3256034390248,1.,-3.39513342019756));
#47473=CARTESIAN_POINT('Ctrl Pts',(-2.33222789882489,1.,-3.39918194577956));
#47474=CARTESIAN_POINT('Ctrl Pts',(-2.33887832342782,1.,-3.40320452776743));
#47475=CARTESIAN_POINT('Ctrl Pts',(-2.34555447649188,1.,-3.40720137404297));
#47476=CARTESIAN_POINT('Ctrl Pts',(-2.35225606824109,1.,-3.41117262314119));
#47477=CARTESIAN_POINT('Ctrl Pts',(-2.35898278606946,1.,-3.41511836751469));
#47478=CARTESIAN_POINT('Ctrl Pts',(-2.36573431470642,1.,-3.41903866635852));
#47479=CARTESIAN_POINT('Ctrl Pts',(-2.37251035954292,1.,-3.42293356216511));
#47480=CARTESIAN_POINT('Ctrl Pts',(-2.37931067028926,1.,-3.42680309754399));
#47481=CARTESIAN_POINT('Ctrl Pts',(-2.38613505843552,1.,-3.4306473271292));
#47482=CARTESIAN_POINT('Ctrl Pts',(-2.39298338804493,1.,-3.4344663067854));
#47483=CARTESIAN_POINT('Ctrl Pts',(-2.39848113410292,1.,-3.43750133064416));
#47484=CARTESIAN_POINT('Ctrl Pts',(-2.40261515589405,1.,-3.43976627484234));
#47485=CARTESIAN_POINT('Ctrl Pts',(-2.4053759295909,1.,-3.44127120683039));
#47486=CARTESIAN_POINT('Ctrl Pts',(-2.40675750623143,1.,-3.44202241512147));
#47487=CARTESIAN_POINT('Origin',(-2.40675750623143,0.,-3.44202241512147));
#47488=CARTESIAN_POINT('',(-2.52982887637028,1.,-3.35260583073571));
#47489=CARTESIAN_POINT('Origin',(0.,0.,0.));
#47490=CARTESIAN_POINT('',(-1.88097764062697,1.,-3.24413672884812));
#47491=CARTESIAN_POINT('Origin',(0.,1.,0.));
#47492=CARTESIAN_POINT('Ctrl Pts',(-1.88097764062697,1.,-3.24413672884812));
#47493=CARTESIAN_POINT('Ctrl Pts',(-1.88097764062697,0.666666666666667,
-3.24413672884812));
#47494=CARTESIAN_POINT('Ctrl Pts',(-1.88097764062697,0.333333333333333,
-3.24413672884812));
#47495=CARTESIAN_POINT('Ctrl Pts',(-1.88097764062697,-0.333333333333333,
-3.24413672884812));
#47496=CARTESIAN_POINT('Ctrl Pts',(-1.88097764062697,-0.666666666666667,
-3.24413672884812));
#47497=CARTESIAN_POINT('Ctrl Pts',(-1.88097764062697,-1.,-3.24413672884812));
#47498=CARTESIAN_POINT('Ctrl Pts',(-1.97421938526992,-1.,-3.70708211654725));
#47499=CARTESIAN_POINT('Ctrl Pts',(-1.97421938526992,1.,-3.70708211654725));
#47500=CARTESIAN_POINT('Ctrl Pts',(-1.97417727645308,-1.,-3.70551008132332));
#47501=CARTESIAN_POINT('Ctrl Pts',(-1.97417727645308,1.,-3.70551008132332));
#47502=CARTESIAN_POINT('Ctrl Pts',(-1.97408973726715,-1.,-3.70236698912904));
#47503=CARTESIAN_POINT('Ctrl Pts',(-1.97408973726715,1.,-3.70236698912904));
#47504=CARTESIAN_POINT('Ctrl Pts',(-1.97394846383216,-1.,-3.6976552856004));
#47505=CARTESIAN_POINT('Ctrl Pts',(-1.97394846383216,1.,-3.6976552856004));
#47506=CARTESIAN_POINT('Ctrl Pts',(-1.97374016225483,-1.,-3.69137888599902));
#47507=CARTESIAN_POINT('Ctrl Pts',(-1.97374016225483,1.,-3.69137888599902));
#47508=CARTESIAN_POINT('Ctrl Pts',(-1.97344650304519,-1.,-3.68354319915092));
#47509=CARTESIAN_POINT('Ctrl Pts',(-1.97344650304519,1.,-3.68354319915092));
#47510=CARTESIAN_POINT('Ctrl Pts',(-1.97311947678517,-1.,-3.67571738107084));
#47511=CARTESIAN_POINT('Ctrl Pts',(-1.97311947678517,1.,-3.67571738107084));
#47512=CARTESIAN_POINT('Ctrl Pts',(-1.97275897198678,-1.,-3.66790152752075));
#47513=CARTESIAN_POINT('Ctrl Pts',(-1.97275897198678,1.,-3.66790152752075));
#47514=CARTESIAN_POINT('Ctrl Pts',(-1.9723648543905,-1.,-3.6600957816636));
#47515=CARTESIAN_POINT('Ctrl Pts',(-1.9723648543905,1.,-3.6600957816636));
#47516=CARTESIAN_POINT('Ctrl Pts',(-1.9719369724024,-1.,-3.652300347166));
#47517=CARTESIAN_POINT('Ctrl Pts',(-1.9719369724024,1.,-3.652300347166));
#47518=CARTESIAN_POINT('Ctrl Pts',(-1.97147515441164,-1.,-3.64451546723514));
#47519=CARTESIAN_POINT('Ctrl Pts',(-1.97147515441164,1.,-3.64451546723514));
#47520=CARTESIAN_POINT('Ctrl Pts',(-1.97097920454464,-1.,-3.63674139590412));
#47521=CARTESIAN_POINT('Ctrl Pts',(-1.97097920454464,1.,-3.63674139590412));
#47522=CARTESIAN_POINT('Ctrl Pts',(-1.97044889850463,-1.,-3.62897836973293));
#47523=CARTESIAN_POINT('Ctrl Pts',(-1.97044889850463,1.,-3.62897836973293));
#47524=CARTESIAN_POINT('Ctrl Pts',(-1.96988398129978,-1.,-3.62122658401893));
#47525=CARTESIAN_POINT('Ctrl Pts',(-1.96988398129978,1.,-3.62122658401893));
#47526=CARTESIAN_POINT('Ctrl Pts',(-1.96928416040877,-1.,-3.61348615496704));
#47527=CARTESIAN_POINT('Ctrl Pts',(-1.96928416040877,1.,-3.61348615496704));
#47528=CARTESIAN_POINT('Ctrl Pts',(-1.9686491188594,-1.,-3.60575714017989));
#47529=CARTESIAN_POINT('Ctrl Pts',(-1.9686491188594,1.,-3.60575714017989));
#47530=CARTESIAN_POINT('Ctrl Pts',(-1.96797854118369,-1.,-3.59803959819938));
#47531=CARTESIAN_POINT('Ctrl Pts',(-1.96797854118369,1.,-3.59803959819938));
#47532=CARTESIAN_POINT('Ctrl Pts',(-1.96727213799544,-1.,-3.59033364022801));
#47533=CARTESIAN_POINT('Ctrl Pts',(-1.96727213799544,1.,-3.59033364022801));
#47534=CARTESIAN_POINT('Ctrl Pts',(-1.96652966688911,-1.,-3.58263947663829));
#47535=CARTESIAN_POINT('Ctrl Pts',(-1.96652966688911,1.,-3.58263947663829));
#47536=CARTESIAN_POINT('Ctrl Pts',(-1.96575096652789,-1.,-3.57495748600959));
#47537=CARTESIAN_POINT('Ctrl Pts',(-1.96575096652789,1.,-3.57495748600959));
#47538=CARTESIAN_POINT('Ctrl Pts',(-1.96493594634567,-1.,-3.56728820357791));
#47539=CARTESIAN_POINT('Ctrl Pts',(-1.96493594634567,1.,-3.56728820357791));
#47540=CARTESIAN_POINT('Ctrl Pts',(-1.96408450906812,-1.,-3.55963218706096));
#47541=CARTESIAN_POINT('Ctrl Pts',(-1.96408450906812,1.,-3.55963218706096));
#47542=CARTESIAN_POINT('Ctrl Pts',(-1.96319648628644,-1.,-3.55198990600886));
#47543=CARTESIAN_POINT('Ctrl Pts',(-1.96319648628644,1.,-3.55198990600886));
#47544=CARTESIAN_POINT('Ctrl Pts',(-1.96227157573067,-1.,-3.54436163300443));
#47545=CARTESIAN_POINT('Ctrl Pts',(-1.96227157573067,1.,-3.54436163300443));
#47546=CARTESIAN_POINT('Ctrl Pts',(-1.96130926212689,-1.,-3.53674730625813));
#47547=CARTESIAN_POINT('Ctrl Pts',(-1.96130926212689,1.,-3.53674730625813));
#47548=CARTESIAN_POINT('Ctrl Pts',(-1.96030879411566,-1.,-3.52914648844351));
#47549=CARTESIAN_POINT('Ctrl Pts',(-1.96030879411566,1.,-3.52914648844351));
#47550=CARTESIAN_POINT('Ctrl Pts',(-1.95926936324461,-1.,-3.52155867431486));
#47551=CARTESIAN_POINT('Ctrl Pts',(-1.95926936324461,1.,-3.52155867431486));
#47552=CARTESIAN_POINT('Ctrl Pts',(-1.95819025316779,-1.,-3.51398354617794));
#47553=CARTESIAN_POINT('Ctrl Pts',(-1.95819025316779,1.,-3.51398354617794));
#47554=CARTESIAN_POINT('Ctrl Pts',(-1.95707099606511,-1.,-3.50642124159909));
#47555=CARTESIAN_POINT('Ctrl Pts',(-1.95707099606511,1.,-3.50642124159909));
#47556=CARTESIAN_POINT('Ctrl Pts',(-1.95591153823661,-1.,-3.49887263575583));
#47557=CARTESIAN_POINT('Ctrl Pts',(-1.95591153823661,1.,-3.49887263575583));
#47558=CARTESIAN_POINT('Ctrl Pts',(-1.95471236969643,-1.,-3.49133956289133));
#47559=CARTESIAN_POINT('Ctrl Pts',(-1.95471236969643,1.,-3.49133956289133));
#47560=CARTESIAN_POINT('Ctrl Pts',(-1.95347412486309,-1.,-3.48382414832634));
#47561=CARTESIAN_POINT('Ctrl Pts',(-1.95347412486309,1.,-3.48382414832634));
#47562=CARTESIAN_POINT('Ctrl Pts',(-1.95219722189876,-1.,-3.47632820495921));
#47563=CARTESIAN_POINT('Ctrl Pts',(-1.95219722189876,1.,-3.47632820495921));
#47564=CARTESIAN_POINT('Ctrl Pts',(-1.95088147859877,-1.,-3.46885258974191));
#47565=CARTESIAN_POINT('Ctrl Pts',(-1.95088147859877,1.,-3.46885258974191));
#47566=CARTESIAN_POINT('Ctrl Pts',(-1.94952575850197,-1.,-3.46139661060962));
#47567=CARTESIAN_POINT('Ctrl Pts',(-1.94952575850197,1.,-3.46139661060962));
#47568=CARTESIAN_POINT('Ctrl Pts',(-1.94812754766524,-1.,-3.45395731584051));
#47569=CARTESIAN_POINT('Ctrl Pts',(-1.94812754766524,1.,-3.45395731584051));
#47570=CARTESIAN_POINT('Ctrl Pts',(-1.94668377715329,-1.,-3.44653088665681));
#47571=CARTESIAN_POINT('Ctrl Pts',(-1.94668377715329,1.,-3.44653088665681));
#47572=CARTESIAN_POINT('Ctrl Pts',(-1.94519168842879,-1.,-3.43911410197687));
#47573=CARTESIAN_POINT('Ctrl Pts',(-1.94519168842879,1.,-3.43911410197687));
#47574=CARTESIAN_POINT('Ctrl Pts',(-1.94364973660284,-1.,-3.43170586602434));
#47575=CARTESIAN_POINT('Ctrl Pts',(-1.94364973660284,1.,-3.43170586602434));
#47576=CARTESIAN_POINT('Ctrl Pts',(-1.94205835913696,-1.,-3.42430850941503));
#47577=CARTESIAN_POINT('Ctrl Pts',(-1.94205835913696,1.,-3.42430850941503));
#47578=CARTESIAN_POINT('Ctrl Pts',(-1.94042111965246,-1.,-3.41692971994096));
#47579=CARTESIAN_POINT('Ctrl Pts',(-1.94042111965246,1.,-3.41692971994096));
#47580=CARTESIAN_POINT('Ctrl Pts',(-1.93874306008143,-1.,-3.40957978266642));
#47581=CARTESIAN_POINT('Ctrl Pts',(-1.93874306008143,1.,-3.40957978266642));
#47582=CARTESIAN_POINT('Ctrl Pts',(-1.93702857723098,-1.,-3.40226802104109));
#47583=CARTESIAN_POINT('Ctrl Pts',(-1.93702857723098,1.,-3.40226802104109));
#47584=CARTESIAN_POINT('Ctrl Pts',(-1.93527929945985,-1.,-3.39499923640795));
#47585=CARTESIAN_POINT('Ctrl Pts',(-1.93527929945985,1.,-3.39499923640795));
#47586=CARTESIAN_POINT('Ctrl Pts',(-1.93349233176788,-1.,-3.38777076883256));
#47587=CARTESIAN_POINT('Ctrl Pts',(-1.93349233176788,1.,-3.38777076883256));
#47588=CARTESIAN_POINT('Ctrl Pts',(-1.93165739093276,-1.,-3.3805676852555));
#47589=CARTESIAN_POINT('Ctrl Pts',(-1.93165739093276,1.,-3.3805676852555));
#47590=CARTESIAN_POINT('Ctrl Pts',(-1.92975993109877,-1.,-3.37336807068043));
#47591=CARTESIAN_POINT('Ctrl Pts',(-1.92975993109877,1.,-3.37336807068043));
#47592=CARTESIAN_POINT('Ctrl Pts',(-1.92778626543786,-1.,-3.36615168657567));
#47593=CARTESIAN_POINT('Ctrl Pts',(-1.92778626543786,1.,-3.36615168657567));
#47594=CARTESIAN_POINT('Ctrl Pts',(-1.92572846125756,-1.,-3.35890824422965));
#47595=CARTESIAN_POINT('Ctrl Pts',(-1.92572846125756,1.,-3.35890824422965));
#47596=CARTESIAN_POINT('Ctrl Pts',(-1.92358838440528,-1.,-3.35164424847223));
#47597=CARTESIAN_POINT('Ctrl Pts',(-1.92358838440528,1.,-3.35164424847223));
#47598=CARTESIAN_POINT('Ctrl Pts',(-1.92138450828404,-1.,-3.34439448941961));
#47599=CARTESIAN_POINT('Ctrl Pts',(-1.92138450828404,1.,-3.34439448941961));
#47600=CARTESIAN_POINT('Ctrl Pts',(-1.9191460961021,-1.,-3.33721230710012));
#47601=CARTESIAN_POINT('Ctrl Pts',(-1.9191460961021,1.,-3.33721230710012));
#47602=CARTESIAN_POINT('Ctrl Pts',(-1.91690081930331,-1.,-3.33014884257873));
#47603=CARTESIAN_POINT('Ctrl Pts',(-1.91690081930331,1.,-3.33014884257873));
#47604=CARTESIAN_POINT('Ctrl Pts',(-1.91466343916628,-1.,-3.32323403454535));
#47605=CARTESIAN_POINT('Ctrl Pts',(-1.91466343916628,1.,-3.32323403454535));
#47606=CARTESIAN_POINT('Ctrl Pts',(-1.91242616234442,-1.,-3.31646052426364));
#47607=CARTESIAN_POINT('Ctrl Pts',(-1.91242616234442,1.,-3.31646052426364));
#47608=CARTESIAN_POINT('Ctrl Pts',(-1.91014297830446,-1.,-3.30975721158596));
#47609=CARTESIAN_POINT('Ctrl Pts',(-1.91014297830446,1.,-3.30975721158596));
#47610=CARTESIAN_POINT('Ctrl Pts',(-1.90773912171341,-1.,-3.30300595568195));
#47611=CARTESIAN_POINT('Ctrl Pts',(-1.90773912171341,1.,-3.30300595568195));
#47612=CARTESIAN_POINT('Ctrl Pts',(-1.90513891864087,-1.,-3.29608978722113));
#47613=CARTESIAN_POINT('Ctrl Pts',(-1.90513891864087,1.,-3.29608978722113));
#47614=CARTESIAN_POINT('Ctrl Pts',(-1.90228971247527,-1.,-3.2889344860029));
#47615=CARTESIAN_POINT('Ctrl Pts',(-1.90228971247527,1.,-3.2889344860029));
#47616=CARTESIAN_POINT('Ctrl Pts',(-1.89918429230462,-1.,-3.28154737912352));
#47617=CARTESIAN_POINT('Ctrl Pts',(-1.89918429230462,1.,-3.28154737912352));
#47618=CARTESIAN_POINT('Ctrl Pts',(-1.89589172903793,-1.,-3.27407108933139));
#47619=CARTESIAN_POINT('Ctrl Pts',(-1.89589172903793,1.,-3.27407108933139));
#47620=CARTESIAN_POINT('Ctrl Pts',(-1.89255393500965,-1.,-3.26677653888676));
#47621=CARTESIAN_POINT('Ctrl Pts',(-1.89255393500965,1.,-3.26677653888676));
#47622=CARTESIAN_POINT('Ctrl Pts',(-1.88934996203698,-1.,-3.25999885193947));
#47623=CARTESIAN_POINT('Ctrl Pts',(-1.88934996203698,1.,-3.25999885193947));
#47624=CARTESIAN_POINT('Ctrl Pts',(-1.88646802523466,-1.,-3.25408686339463));
#47625=CARTESIAN_POINT('Ctrl Pts',(-1.88646802523466,1.,-3.25408686339463));
#47626=CARTESIAN_POINT('Ctrl Pts',(-1.88407708646357,-1.,-3.24935200511918));
#47627=CARTESIAN_POINT('Ctrl Pts',(-1.88407708646357,1.,-3.24935200511918));
#47628=CARTESIAN_POINT('Ctrl Pts',(-1.88229202582941,-1.,-3.24600543790443));
#47629=CARTESIAN_POINT('Ctrl Pts',(-1.88229202582941,1.,-3.24600543790443));
#47630=CARTESIAN_POINT('Ctrl Pts',(-1.88139187908074,-1.,-3.24451807186481));
#47631=CARTESIAN_POINT('Ctrl Pts',(-1.88139187908074,1.,-3.24451807186481));
#47632=CARTESIAN_POINT('Ctrl Pts',(-1.88102201872555,-1.,-3.24408699284121));
#47633=CARTESIAN_POINT('Ctrl Pts',(-1.88102201872555,1.,-3.24408699284121));
#47634=CARTESIAN_POINT('Ctrl Pts',(-1.88091100680349,-1.,-3.24410359189609));
#47635=CARTESIAN_POINT('Ctrl Pts',(-1.88091100680349,1.,-3.24410359189609));
#47636=CARTESIAN_POINT('Ctrl Pts',(-1.8808893942881,-1.,-3.24418789321065));
#47637=CARTESIAN_POINT('Ctrl Pts',(-1.8808893942881,1.,-3.24418789321065));
#47638=CARTESIAN_POINT('',(-1.97421938526992,1.,-3.70708211654725));
#47639=CARTESIAN_POINT('Ctrl Pts',(-1.97421938526992,1.,-3.70708211654725));
#47640=CARTESIAN_POINT('Ctrl Pts',(-1.97417727645308,1.,-3.70551008132332));
#47641=CARTESIAN_POINT('Ctrl Pts',(-1.97408973726715,1.,-3.70236698912904));
#47642=CARTESIAN_POINT('Ctrl Pts',(-1.97394846383216,1.,-3.6976552856004));
#47643=CARTESIAN_POINT('Ctrl Pts',(-1.97374016225483,1.,-3.69137888599902));
#47644=CARTESIAN_POINT('Ctrl Pts',(-1.97344650304519,1.,-3.68354319915092));
#47645=CARTESIAN_POINT('Ctrl Pts',(-1.97311947678517,1.,-3.67571738107084));
#47646=CARTESIAN_POINT('Ctrl Pts',(-1.97275897198678,1.,-3.66790152752075));
#47647=CARTESIAN_POINT('Ctrl Pts',(-1.9723648543905,1.,-3.6600957816636));
#47648=CARTESIAN_POINT('Ctrl Pts',(-1.9719369724024,1.,-3.652300347166));
#47649=CARTESIAN_POINT('Ctrl Pts',(-1.97147515441164,1.,-3.64451546723514));
#47650=CARTESIAN_POINT('Ctrl Pts',(-1.97097920454464,1.,-3.63674139590412));
#47651=CARTESIAN_POINT('Ctrl Pts',(-1.97044889850463,1.,-3.62897836973293));
#47652=CARTESIAN_POINT('Ctrl Pts',(-1.96988398129978,1.,-3.62122658401893));
#47653=CARTESIAN_POINT('Ctrl Pts',(-1.96928416040877,1.,-3.61348615496704));
#47654=CARTESIAN_POINT('Ctrl Pts',(-1.9686491188594,1.,-3.60575714017989));
#47655=CARTESIAN_POINT('Ctrl Pts',(-1.96797854118369,1.,-3.59803959819938));
#47656=CARTESIAN_POINT('Ctrl Pts',(-1.96727213799544,1.,-3.59033364022801));
#47657=CARTESIAN_POINT('Ctrl Pts',(-1.96652966688911,1.,-3.58263947663829));
#47658=CARTESIAN_POINT('Ctrl Pts',(-1.96575096652789,1.,-3.57495748600959));
#47659=CARTESIAN_POINT('Ctrl Pts',(-1.96493594634567,1.,-3.56728820357791));
#47660=CARTESIAN_POINT('Ctrl Pts',(-1.96408450906812,1.,-3.55963218706096));
#47661=CARTESIAN_POINT('Ctrl Pts',(-1.96319648628644,1.,-3.55198990600886));
#47662=CARTESIAN_POINT('Ctrl Pts',(-1.96227157573067,1.,-3.54436163300443));
#47663=CARTESIAN_POINT('Ctrl Pts',(-1.96130926212689,1.,-3.53674730625813));
#47664=CARTESIAN_POINT('Ctrl Pts',(-1.96030879411566,1.,-3.52914648844351));
#47665=CARTESIAN_POINT('Ctrl Pts',(-1.95926936324461,1.,-3.52155867431486));
#47666=CARTESIAN_POINT('Ctrl Pts',(-1.95819025316779,1.,-3.51398354617794));
#47667=CARTESIAN_POINT('Ctrl Pts',(-1.95707099606511,1.,-3.50642124159909));
#47668=CARTESIAN_POINT('Ctrl Pts',(-1.95591153823661,1.,-3.49887263575583));
#47669=CARTESIAN_POINT('Ctrl Pts',(-1.95471236969643,1.,-3.49133956289133));
#47670=CARTESIAN_POINT('Ctrl Pts',(-1.95347412486309,1.,-3.48382414832634));
#47671=CARTESIAN_POINT('Ctrl Pts',(-1.95219722189876,1.,-3.47632820495921));
#47672=CARTESIAN_POINT('Ctrl Pts',(-1.95088147859877,1.,-3.46885258974191));
#47673=CARTESIAN_POINT('Ctrl Pts',(-1.94952575850197,1.,-3.46139661060962));
#47674=CARTESIAN_POINT('Ctrl Pts',(-1.94812754766524,1.,-3.45395731584051));
#47675=CARTESIAN_POINT('Ctrl Pts',(-1.94668377715329,1.,-3.44653088665681));
#47676=CARTESIAN_POINT('Ctrl Pts',(-1.94519168842879,1.,-3.43911410197687));
#47677=CARTESIAN_POINT('Ctrl Pts',(-1.94364973660284,1.,-3.43170586602434));
#47678=CARTESIAN_POINT('Ctrl Pts',(-1.94205835913696,1.,-3.42430850941503));
#47679=CARTESIAN_POINT('Ctrl Pts',(-1.94042111965246,1.,-3.41692971994096));
#47680=CARTESIAN_POINT('Ctrl Pts',(-1.93874306008143,1.,-3.40957978266642));
#47681=CARTESIAN_POINT('Ctrl Pts',(-1.93702857723098,1.,-3.40226802104109));
#47682=CARTESIAN_POINT('Ctrl Pts',(-1.93527929945985,1.,-3.39499923640795));
#47683=CARTESIAN_POINT('Ctrl Pts',(-1.93349233176788,1.,-3.38777076883256));
#47684=CARTESIAN_POINT('Ctrl Pts',(-1.93165739093276,1.,-3.3805676852555));
#47685=CARTESIAN_POINT('Ctrl Pts',(-1.92975993109877,1.,-3.37336807068043));
#47686=CARTESIAN_POINT('Ctrl Pts',(-1.92778626543786,1.,-3.36615168657567));
#47687=CARTESIAN_POINT('Ctrl Pts',(-1.92572846125756,1.,-3.35890824422965));
#47688=CARTESIAN_POINT('Ctrl Pts',(-1.92358838440528,1.,-3.35164424847223));
#47689=CARTESIAN_POINT('Ctrl Pts',(-1.92138450828404,1.,-3.34439448941961));
#47690=CARTESIAN_POINT('Ctrl Pts',(-1.9191460961021,1.,-3.33721230710012));
#47691=CARTESIAN_POINT('Ctrl Pts',(-1.91690081930331,1.,-3.33014884257873));
#47692=CARTESIAN_POINT('Ctrl Pts',(-1.91466343916628,1.,-3.32323403454535));
#47693=CARTESIAN_POINT('Ctrl Pts',(-1.91242616234442,1.,-3.31646052426364));
#47694=CARTESIAN_POINT('Ctrl Pts',(-1.91014297830446,1.,-3.30975721158596));
#47695=CARTESIAN_POINT('Ctrl Pts',(-1.90773912171341,1.,-3.30300595568195));
#47696=CARTESIAN_POINT('Ctrl Pts',(-1.90513891864087,1.,-3.29608978722113));
#47697=CARTESIAN_POINT('Ctrl Pts',(-1.90228971247527,1.,-3.2889344860029));
#47698=CARTESIAN_POINT('Ctrl Pts',(-1.89918429230462,1.,-3.28154737912352));
#47699=CARTESIAN_POINT('Ctrl Pts',(-1.89589172903793,1.,-3.27407108933139));
#47700=CARTESIAN_POINT('Ctrl Pts',(-1.89255393500965,1.,-3.26677653888676));
#47701=CARTESIAN_POINT('Ctrl Pts',(-1.88934996203698,1.,-3.25999885193947));
#47702=CARTESIAN_POINT('Ctrl Pts',(-1.88646802523466,1.,-3.25408686339463));
#47703=CARTESIAN_POINT('Ctrl Pts',(-1.88407708646357,1.,-3.24935200511918));
#47704=CARTESIAN_POINT('Ctrl Pts',(-1.88242596600454,1.,-3.2462565441079));
#47705=CARTESIAN_POINT('Ctrl Pts',(-1.88156537699203,1.,-3.24480754676064));
#47706=CARTESIAN_POINT('Ctrl Pts',(-1.88117508446775,1.,-3.24428080353022));
#47707=CARTESIAN_POINT('Ctrl Pts',(-1.8810229239812,1.,-3.24415531671284));
#47708=CARTESIAN_POINT('Ctrl Pts',(-1.88097764062697,1.,-3.24413672884812));
#47709=CARTESIAN_POINT('',(-1.97421938526992,0.,-3.70708211654725));
#47710=CARTESIAN_POINT('Ctrl Pts',(-1.519044091397,-1.,-3.42855728381368));
#47711=CARTESIAN_POINT('Ctrl Pts',(-1.519044091397,1.,-3.42855728381368));
#47712=CARTESIAN_POINT('Ctrl Pts',(-1.51896318668366,-1.,-3.42852521763778));
#47713=CARTESIAN_POINT('Ctrl Pts',(-1.51896318668366,1.,-3.42852521763778));
#47714=CARTESIAN_POINT('Ctrl Pts',(-1.51888450659652,-1.,-3.42860527149177));
#47715=CARTESIAN_POINT('Ctrl Pts',(-1.51888450659652,1.,-3.42860527149177));
#47716=CARTESIAN_POINT('Ctrl Pts',(-1.51901585839109,-1.,-3.42915787669893));
#47717=CARTESIAN_POINT('Ctrl Pts',(-1.51901585839109,1.,-3.42915787669893));
#47718=CARTESIAN_POINT('Ctrl Pts',(-1.51969006980999,-1.,-3.43076036253837));
#47719=CARTESIAN_POINT('Ctrl Pts',(-1.51969006980999,1.,-3.43076036253837));
#47720=CARTESIAN_POINT('Ctrl Pts',(-1.52134826724293,-1.,-3.43417156977893));
#47721=CARTESIAN_POINT('Ctrl Pts',(-1.52134826724293,1.,-3.43417156977893));
#47722=CARTESIAN_POINT('Ctrl Pts',(-1.5237734895035,-1.,-3.4388889597401));
#47723=CARTESIAN_POINT('Ctrl Pts',(-1.5237734895035,1.,-3.4388889597401));
#47724=CARTESIAN_POINT('Ctrl Pts',(-1.52686242875556,-1.,-3.44469547526647));
#47725=CARTESIAN_POINT('Ctrl Pts',(-1.52686242875556,1.,-3.44469547526647));
#47726=CARTESIAN_POINT('Ctrl Pts',(-1.53046244461635,-1.,-3.45127136828305));
#47727=CARTESIAN_POINT('Ctrl Pts',(-1.53046244461635,1.,-3.45127136828305));
#47728=CARTESIAN_POINT('Ctrl Pts',(-1.53440195378792,-1.,-3.45825932955032));
#47729=CARTESIAN_POINT('Ctrl Pts',(-1.53440195378792,1.,-3.45825932955032));
#47730=CARTESIAN_POINT('Ctrl Pts',(-1.53851507915502,-1.,-3.46531752207153));
#47731=CARTESIAN_POINT('Ctrl Pts',(-1.53851507915502,1.,-3.46531752207153));
#47732=CARTESIAN_POINT('Ctrl Pts',(-1.54266605398187,-1.,-3.47217189224653));
#47733=CARTESIAN_POINT('Ctrl Pts',(-1.54266605398187,1.,-3.47217189224653));
#47734=CARTESIAN_POINT('Ctrl Pts',(-1.54678009290276,-1.,-3.47868272898751));
#47735=CARTESIAN_POINT('Ctrl Pts',(-1.54678009290276,1.,-3.47868272898751));
#47736=CARTESIAN_POINT('Ctrl Pts',(-1.55084702970452,-1.,-3.48485155928567));
#47737=CARTESIAN_POINT('Ctrl Pts',(-1.55084702970452,1.,-3.48485155928567));
#47738=CARTESIAN_POINT('Ctrl Pts',(-1.55489595901116,-1.,-3.4907646087742));
#47739=CARTESIAN_POINT('Ctrl Pts',(-1.55489595901116,1.,-3.4907646087742));
#47740=CARTESIAN_POINT('Ctrl Pts',(-1.55897703097874,-1.,-3.49655185179655));
#47741=CARTESIAN_POINT('Ctrl Pts',(-1.55897703097874,1.,-3.49655185179655));
#47742=CARTESIAN_POINT('Ctrl Pts',(-1.56314187758675,-1.,-3.50234321621578));
#47743=CARTESIAN_POINT('Ctrl Pts',(-1.56314187758675,1.,-3.50234321621578));
#47744=CARTESIAN_POINT('Ctrl Pts',(-1.56742097575012,-1.,-3.50821771695363));
#47745=CARTESIAN_POINT('Ctrl Pts',(-1.56742097575012,1.,-3.50821771695363));
#47746=CARTESIAN_POINT('Ctrl Pts',(-1.57181569799743,-1.,-3.51418598431665));
#47747=CARTESIAN_POINT('Ctrl Pts',(-1.57181569799743,1.,-3.51418598431665));
#47748=CARTESIAN_POINT('Ctrl Pts',(-1.57631049988158,-1.,-3.52021847865912));
#47749=CARTESIAN_POINT('Ctrl Pts',(-1.57631049988158,1.,-3.52021847865912));
#47750=CARTESIAN_POINT('Ctrl Pts',(-1.58088027227848,-1.,-3.52626275334881));
#47751=CARTESIAN_POINT('Ctrl Pts',(-1.58088027227848,1.,-3.52626275334881));
#47752=CARTESIAN_POINT('Ctrl Pts',(-1.58549906268088,-1.,-3.5322637814708));
#47753=CARTESIAN_POINT('Ctrl Pts',(-1.58549906268088,1.,-3.5322637814708));
#47754=CARTESIAN_POINT('Ctrl Pts',(-1.59014958368739,-1.,-3.53818616861077));
#47755=CARTESIAN_POINT('Ctrl Pts',(-1.59014958368739,1.,-3.53818616861077));
#47756=CARTESIAN_POINT('Ctrl Pts',(-1.59482766949766,-1.,-3.54402458182337));
#47757=CARTESIAN_POINT('Ctrl Pts',(-1.59482766949766,1.,-3.54402458182337));
#47758=CARTESIAN_POINT('Ctrl Pts',(-1.59953698113457,-1.,-3.54979148634454));
#47759=CARTESIAN_POINT('Ctrl Pts',(-1.59953698113457,1.,-3.54979148634454));
#47760=CARTESIAN_POINT('Ctrl Pts',(-1.60428584699853,-1.,-3.55550985096129));
#47761=CARTESIAN_POINT('Ctrl Pts',(-1.60428584699853,1.,-3.55550985096129));
#47762=CARTESIAN_POINT('Ctrl Pts',(-1.60908344685457,-1.,-3.5612043248298));
#47763=CARTESIAN_POINT('Ctrl Pts',(-1.60908344685457,1.,-3.5612043248298));
#47764=CARTESIAN_POINT('Ctrl Pts',(-1.61393581747514,-1.,-3.56689200468387));
#47765=CARTESIAN_POINT('Ctrl Pts',(-1.61393581747514,1.,-3.56689200468387));
#47766=CARTESIAN_POINT('Ctrl Pts',(-1.61884340915404,-1.,-3.57257679609806));
#47767=CARTESIAN_POINT('Ctrl Pts',(-1.61884340915404,1.,-3.57257679609806));
#47768=CARTESIAN_POINT('Ctrl Pts',(-1.62380329464844,-1.,-3.5782545595439));
#47769=CARTESIAN_POINT('Ctrl Pts',(-1.62380329464844,1.,-3.5782545595439));
#47770=CARTESIAN_POINT('Ctrl Pts',(-1.62881051550745,-1.,-3.58391625774343));
#47771=CARTESIAN_POINT('Ctrl Pts',(-1.62881051550745,1.,-3.58391625774343));
#47772=CARTESIAN_POINT('Ctrl Pts',(-1.6338597145126,-1.,-3.58955176627879));
#47773=CARTESIAN_POINT('Ctrl Pts',(-1.6338597145126,1.,-3.58955176627879));
#47774=CARTESIAN_POINT('Ctrl Pts',(-1.63894676675352,-1.,-3.59515368334893));
#47775=CARTESIAN_POINT('Ctrl Pts',(-1.63894676675352,1.,-3.59515368334893));
#47776=CARTESIAN_POINT('Ctrl Pts',(-1.64407004385582,-1.,-3.60072028513845));
#47777=CARTESIAN_POINT('Ctrl Pts',(-1.64407004385582,1.,-3.60072028513845));
#47778=CARTESIAN_POINT('Ctrl Pts',(-1.64922952425832,-1.,-3.60625346556992));
#47779=CARTESIAN_POINT('Ctrl Pts',(-1.64922952425832,1.,-3.60625346556992));
#47780=CARTESIAN_POINT('Ctrl Pts',(-1.65442619244325,-1.,-3.61175734965127));
#47781=CARTESIAN_POINT('Ctrl Pts',(-1.65442619244325,1.,-3.61175734965127));
#47782=CARTESIAN_POINT('Ctrl Pts',(-1.65966133399186,-1.,-3.61723666482456));
#47783=CARTESIAN_POINT('Ctrl Pts',(-1.65966133399186,1.,-3.61723666482456));
#47784=CARTESIAN_POINT('Ctrl Pts',(-1.66493585923855,-1.,-3.62269517989109));
#47785=CARTESIAN_POINT('Ctrl Pts',(-1.66493585923855,1.,-3.62269517989109));
#47786=CARTESIAN_POINT('Ctrl Pts',(-1.67024966008045,-1.,-3.62813422105271));
#47787=CARTESIAN_POINT('Ctrl Pts',(-1.67024966008045,1.,-3.62813422105271));
#47788=CARTESIAN_POINT('Ctrl Pts',(-1.67560193613156,-1.,-3.63355343201232));
#47789=CARTESIAN_POINT('Ctrl Pts',(-1.67560193613156,1.,-3.63355343201232));
#47790=CARTESIAN_POINT('Ctrl Pts',(-1.68099146651586,-1.,-3.63895140887462));
#47791=CARTESIAN_POINT('Ctrl Pts',(-1.68099146651586,1.,-3.63895140887462));
#47792=CARTESIAN_POINT('Ctrl Pts',(-1.68641690471457,-1.,-3.64432638915203));
#47793=CARTESIAN_POINT('Ctrl Pts',(-1.68641690471457,1.,-3.64432638915203));
#47794=CARTESIAN_POINT('Ctrl Pts',(-1.69187705481689,-1.,-3.64967689827371));
#47795=CARTESIAN_POINT('Ctrl Pts',(-1.69187705481689,1.,-3.64967689827371));
#47796=CARTESIAN_POINT('Ctrl Pts',(-1.69737117722534,-1.,-3.65500246526749));
#47797=CARTESIAN_POINT('Ctrl Pts',(-1.69737117722534,1.,-3.65500246526749));
#47798=CARTESIAN_POINT('Ctrl Pts',(-1.70289888566873,-1.,-3.66030338774847));
#47799=CARTESIAN_POINT('Ctrl Pts',(-1.70289888566873,1.,-3.66030338774847));
#47800=CARTESIAN_POINT('Ctrl Pts',(-1.70846001610956,-1.,-3.66558043198876));
#47801=CARTESIAN_POINT('Ctrl Pts',(-1.70846001610956,1.,-3.66558043198876));
#47802=CARTESIAN_POINT('Ctrl Pts',(-1.71405450210384,-1.,-3.67083454901611));
#47803=CARTESIAN_POINT('Ctrl Pts',(-1.71405450210384,1.,-3.67083454901611));
#47804=CARTESIAN_POINT('Ctrl Pts',(-1.71968225581808,-1.,-3.67606660374709));
#47805=CARTESIAN_POINT('Ctrl Pts',(-1.71968225581808,1.,-3.67606660374709));
#47806=CARTESIAN_POINT('Ctrl Pts',(-1.72534302437056,-1.,-3.68127704936579));
#47807=CARTESIAN_POINT('Ctrl Pts',(-1.72534302437056,1.,-3.68127704936579));
#47808=CARTESIAN_POINT('Ctrl Pts',(-1.73103640956717,-1.,-3.68646597019332));
#47809=CARTESIAN_POINT('Ctrl Pts',(-1.73103640956717,1.,-3.68646597019332));
#47810=CARTESIAN_POINT('Ctrl Pts',(-1.73676193254557,-1.,-3.69163322648036));
#47811=CARTESIAN_POINT('Ctrl Pts',(-1.73676193254557,1.,-3.69163322648036));
#47812=CARTESIAN_POINT('Ctrl Pts',(-1.74251908492617,-1.,-3.69677856910517));
#47813=CARTESIAN_POINT('Ctrl Pts',(-1.74251908492617,1.,-3.69677856910517));
#47814=CARTESIAN_POINT('Ctrl Pts',(-1.74830738046057,-1.,-3.7019017567335));
#47815=CARTESIAN_POINT('Ctrl Pts',(-1.74830738046057,1.,-3.7019017567335));
#47816=CARTESIAN_POINT('Ctrl Pts',(-1.75412641804042,-1.,-3.70700269736659));
#47817=CARTESIAN_POINT('Ctrl Pts',(-1.75412641804042,1.,-3.70700269736659));
#47818=CARTESIAN_POINT('Ctrl Pts',(-1.75997588498865,-1.,-3.71208146346136));
#47819=CARTESIAN_POINT('Ctrl Pts',(-1.75997588498865,1.,-3.71208146346136));
#47820=CARTESIAN_POINT('Ctrl Pts',(-1.76585552124394,-1.,-3.71713822377359));
#47821=CARTESIAN_POINT('Ctrl Pts',(-1.76585552124394,1.,-3.71713822377359));
#47822=CARTESIAN_POINT('Ctrl Pts',(-1.77176509401761,-1.,-3.72217319911254));
#47823=CARTESIAN_POINT('Ctrl Pts',(-1.77176509401761,1.,-3.72217319911254));
#47824=CARTESIAN_POINT('Ctrl Pts',(-1.77770437039658,-1.,-3.72718661205609));
#47825=CARTESIAN_POINT('Ctrl Pts',(-1.77770437039658,1.,-3.72718661205609));
#47826=CARTESIAN_POINT('Ctrl Pts',(-1.78367308442901,-1.,-3.7321786309547));
#47827=CARTESIAN_POINT('Ctrl Pts',(-1.78367308442901,1.,-3.7321786309547));
#47828=CARTESIAN_POINT('Ctrl Pts',(-1.78967092823491,-1.,-3.73714934730681));
#47829=CARTESIAN_POINT('Ctrl Pts',(-1.78967092823491,1.,-3.73714934730681));
#47830=CARTESIAN_POINT('Ctrl Pts',(-1.79569757859422,-1.,-3.74209880352445));
#47831=CARTESIAN_POINT('Ctrl Pts',(-1.79569757859422,1.,-3.74209880352445));
#47832=CARTESIAN_POINT('Ctrl Pts',(-1.8017527148577,-1.,-3.74702700875467));
#47833=CARTESIAN_POINT('Ctrl Pts',(-1.8017527148577,1.,-3.74702700875467));
#47834=CARTESIAN_POINT('Ctrl Pts',(-1.80783603939617,-1.,-3.75193395887977));
#47835=CARTESIAN_POINT('Ctrl Pts',(-1.80783603939617,1.,-3.75193395887977));
#47836=CARTESIAN_POINT('Ctrl Pts',(-1.8139472983358,-1.,-3.75681965683071));
#47837=CARTESIAN_POINT('Ctrl Pts',(-1.8139472983358,1.,-3.75681965683071));
#47838=CARTESIAN_POINT('Ctrl Pts',(-1.82008629694091,-1.,-3.76168412707948));
#47839=CARTESIAN_POINT('Ctrl Pts',(-1.82008629694091,1.,-3.76168412707948));
#47840=CARTESIAN_POINT('Ctrl Pts',(-1.82625289220915,-1.,-3.76652740353775));
#47841=CARTESIAN_POINT('Ctrl Pts',(-1.82625289220915,1.,-3.76652740353775));
#47842=CARTESIAN_POINT('Ctrl Pts',(-1.83120816955645,-1.,-3.77038509817999));
#47843=CARTESIAN_POINT('Ctrl Pts',(-1.83120816955645,1.,-3.77038509817999));
#47844=CARTESIAN_POINT('Ctrl Pts',(-1.83493697934534,-1.,-3.77326886064398));
#47845=CARTESIAN_POINT('Ctrl Pts',(-1.83493697934534,1.,-3.77326886064398));
#47846=CARTESIAN_POINT('Ctrl Pts',(-1.83742834010626,-1.,-3.77518714457833));
#47847=CARTESIAN_POINT('Ctrl Pts',(-1.83742834010626,1.,-3.77518714457833));
#47848=CARTESIAN_POINT('Ctrl Pts',(-1.83867539237861,-1.,-3.77614523045147));
#47849=CARTESIAN_POINT('Ctrl Pts',(-1.83867539237861,1.,-3.77614523045147));
#47850=CARTESIAN_POINT('',(-1.5189508286633,1.,-3.42859860294306));
#47851=CARTESIAN_POINT('Ctrl Pts',(-1.5189508286633,-1.,-3.42859860294306));
#47852=CARTESIAN_POINT('Ctrl Pts',(-1.5189508286633,-0.666666666666667,
-3.42859860294306));
#47853=CARTESIAN_POINT('Ctrl Pts',(-1.5189508286633,-0.333333333333333,
-3.42859860294306));
#47854=CARTESIAN_POINT('Ctrl Pts',(-1.5189508286633,0.333333333333333,-3.42859860294306));
#47855=CARTESIAN_POINT('Ctrl Pts',(-1.5189508286633,0.666666666666667,-3.42859860294305));
#47856=CARTESIAN_POINT('Ctrl Pts',(-1.5189508286633,1.,-3.42859860294305));
#47857=CARTESIAN_POINT('',(-1.83867539237861,1.,-3.77614523045147));
#47858=CARTESIAN_POINT('',(-1.83867539237861,0.,-3.77614523045147));
#47859=CARTESIAN_POINT('Ctrl Pts',(-1.5189508286633,1.,-3.42859860294306));
#47860=CARTESIAN_POINT('Ctrl Pts',(-1.51893924967331,1.,-3.42864616361875));
#47861=CARTESIAN_POINT('Ctrl Pts',(-1.5189513329503,1.,-3.42884302333841));
#47862=CARTESIAN_POINT('Ctrl Pts',(-1.51914806898491,1.,-3.42946838852588));
#47863=CARTESIAN_POINT('Ctrl Pts',(-1.5198144909338,1.,-3.43101631893414));
#47864=CARTESIAN_POINT('Ctrl Pts',(-1.52134826724293,1.,-3.43417156977893));
#47865=CARTESIAN_POINT('Ctrl Pts',(-1.5237734895035,1.,-3.4388889597401));
#47866=CARTESIAN_POINT('Ctrl Pts',(-1.52686242875556,1.,-3.44469547526647));
#47867=CARTESIAN_POINT('Ctrl Pts',(-1.53046244461635,1.,-3.45127136828305));
#47868=CARTESIAN_POINT('Ctrl Pts',(-1.53440195378792,1.,-3.45825932955032));
#47869=CARTESIAN_POINT('Ctrl Pts',(-1.53851507915502,1.,-3.46531752207153));
#47870=CARTESIAN_POINT('Ctrl Pts',(-1.54266605398187,1.,-3.47217189224653));
#47871=CARTESIAN_POINT('Ctrl Pts',(-1.54678009290276,1.,-3.47868272898751));
#47872=CARTESIAN_POINT('Ctrl Pts',(-1.55084702970452,1.,-3.48485155928567));
#47873=CARTESIAN_POINT('Ctrl Pts',(-1.55489595901116,1.,-3.4907646087742));
#47874=CARTESIAN_POINT('Ctrl Pts',(-1.55897703097874,1.,-3.49655185179655));
#47875=CARTESIAN_POINT('Ctrl Pts',(-1.56314187758675,1.,-3.50234321621578));
#47876=CARTESIAN_POINT('Ctrl Pts',(-1.56742097575012,1.,-3.50821771695363));
#47877=CARTESIAN_POINT('Ctrl Pts',(-1.57181569799743,1.,-3.51418598431665));
#47878=CARTESIAN_POINT('Ctrl Pts',(-1.57631049988158,1.,-3.52021847865912));
#47879=CARTESIAN_POINT('Ctrl Pts',(-1.58088027227848,1.,-3.52626275334881));
#47880=CARTESIAN_POINT('Ctrl Pts',(-1.58549906268088,1.,-3.5322637814708));
#47881=CARTESIAN_POINT('Ctrl Pts',(-1.59014958368739,1.,-3.53818616861077));
#47882=CARTESIAN_POINT('Ctrl Pts',(-1.59482766949766,1.,-3.54402458182337));
#47883=CARTESIAN_POINT('Ctrl Pts',(-1.59953698113457,1.,-3.54979148634454));
#47884=CARTESIAN_POINT('Ctrl Pts',(-1.60428584699853,1.,-3.55550985096129));
#47885=CARTESIAN_POINT('Ctrl Pts',(-1.60908344685457,1.,-3.5612043248298));
#47886=CARTESIAN_POINT('Ctrl Pts',(-1.61393581747514,1.,-3.56689200468387));
#47887=CARTESIAN_POINT('Ctrl Pts',(-1.61884340915404,1.,-3.57257679609806));
#47888=CARTESIAN_POINT('Ctrl Pts',(-1.62380329464844,1.,-3.5782545595439));
#47889=CARTESIAN_POINT('Ctrl Pts',(-1.62881051550745,1.,-3.58391625774343));
#47890=CARTESIAN_POINT('Ctrl Pts',(-1.6338597145126,1.,-3.58955176627879));
#47891=CARTESIAN_POINT('Ctrl Pts',(-1.63894676675352,1.,-3.59515368334893));
#47892=CARTESIAN_POINT('Ctrl Pts',(-1.64407004385582,1.,-3.60072028513845));
#47893=CARTESIAN_POINT('Ctrl Pts',(-1.64922952425832,1.,-3.60625346556992));
#47894=CARTESIAN_POINT('Ctrl Pts',(-1.65442619244325,1.,-3.61175734965127));
#47895=CARTESIAN_POINT('Ctrl Pts',(-1.65966133399186,1.,-3.61723666482456));
#47896=CARTESIAN_POINT('Ctrl Pts',(-1.66493585923855,1.,-3.62269517989109));
#47897=CARTESIAN_POINT('Ctrl Pts',(-1.67024966008045,1.,-3.62813422105271));
#47898=CARTESIAN_POINT('Ctrl Pts',(-1.67560193613156,1.,-3.63355343201232));
#47899=CARTESIAN_POINT('Ctrl Pts',(-1.68099146651586,1.,-3.63895140887462));
#47900=CARTESIAN_POINT('Ctrl Pts',(-1.68641690471457,1.,-3.64432638915203));
#47901=CARTESIAN_POINT('Ctrl Pts',(-1.69187705481689,1.,-3.64967689827371));
#47902=CARTESIAN_POINT('Ctrl Pts',(-1.69737117722534,1.,-3.65500246526749));
#47903=CARTESIAN_POINT('Ctrl Pts',(-1.70289888566873,1.,-3.66030338774847));
#47904=CARTESIAN_POINT('Ctrl Pts',(-1.70846001610956,1.,-3.66558043198876));
#47905=CARTESIAN_POINT('Ctrl Pts',(-1.71405450210384,1.,-3.67083454901611));
#47906=CARTESIAN_POINT('Ctrl Pts',(-1.71968225581808,1.,-3.67606660374709));
#47907=CARTESIAN_POINT('Ctrl Pts',(-1.72534302437056,1.,-3.68127704936579));
#47908=CARTESIAN_POINT('Ctrl Pts',(-1.73103640956717,1.,-3.68646597019332));
#47909=CARTESIAN_POINT('Ctrl Pts',(-1.73676193254557,1.,-3.69163322648036));
#47910=CARTESIAN_POINT('Ctrl Pts',(-1.74251908492617,1.,-3.69677856910517));
#47911=CARTESIAN_POINT('Ctrl Pts',(-1.74830738046057,1.,-3.7019017567335));
#47912=CARTESIAN_POINT('Ctrl Pts',(-1.75412641804042,1.,-3.70700269736659));
#47913=CARTESIAN_POINT('Ctrl Pts',(-1.75997588498865,1.,-3.71208146346136));
#47914=CARTESIAN_POINT('Ctrl Pts',(-1.76585552124394,1.,-3.71713822377359));
#47915=CARTESIAN_POINT('Ctrl Pts',(-1.77176509401761,1.,-3.72217319911254));
#47916=CARTESIAN_POINT('Ctrl Pts',(-1.77770437039658,1.,-3.72718661205609));
#47917=CARTESIAN_POINT('Ctrl Pts',(-1.78367308442901,1.,-3.7321786309547));
#47918=CARTESIAN_POINT('Ctrl Pts',(-1.78967092823491,1.,-3.73714934730681));
#47919=CARTESIAN_POINT('Ctrl Pts',(-1.79569757859422,1.,-3.74209880352445));
#47920=CARTESIAN_POINT('Ctrl Pts',(-1.8017527148577,1.,-3.74702700875467));
#47921=CARTESIAN_POINT('Ctrl Pts',(-1.80783603939617,1.,-3.75193395887977));
#47922=CARTESIAN_POINT('Ctrl Pts',(-1.8139472983358,1.,-3.75681965683071));
#47923=CARTESIAN_POINT('Ctrl Pts',(-1.82008629694091,1.,-3.76168412707948));
#47924=CARTESIAN_POINT('Ctrl Pts',(-1.82625289220915,1.,-3.76652740353775));
#47925=CARTESIAN_POINT('Ctrl Pts',(-1.83120816955645,1.,-3.77038509817999));
#47926=CARTESIAN_POINT('Ctrl Pts',(-1.83493697934534,1.,-3.77326886064398));
#47927=CARTESIAN_POINT('Ctrl Pts',(-1.83742834010626,1.,-3.77518714457833));
#47928=CARTESIAN_POINT('Ctrl Pts',(-1.83867539237861,1.,-3.77614523045147));
#47929=CARTESIAN_POINT('Origin',(-1.83867539237861,0.,-3.77614523045147));
#47930=CARTESIAN_POINT('',(-1.97421938526992,1.,-3.70708211654725));
#47931=CARTESIAN_POINT('Origin',(0.,0.,0.));
#47932=CARTESIAN_POINT('',(-1.35032489087269,1.,-3.49844575334386));
#47933=CARTESIAN_POINT('Origin',(0.,1.,0.));
#47934=CARTESIAN_POINT('Ctrl Pts',(-1.35032489087269,1.,-3.49844575334386));
#47935=CARTESIAN_POINT('Ctrl Pts',(-1.35032489087269,0.666666666666667,
-3.49844575334386));
#47936=CARTESIAN_POINT('Ctrl Pts',(-1.35032489087269,0.333333333333333,
-3.49844575334386));
#47937=CARTESIAN_POINT('Ctrl Pts',(-1.35032489087269,-0.333333333333333,
-3.49844575334386));
#47938=CARTESIAN_POINT('Ctrl Pts',(-1.35032489087269,-0.666666666666667,
-3.49844575334386));
#47939=CARTESIAN_POINT('Ctrl Pts',(-1.35032489087269,-1.,-3.49844575334386));
#47940=CARTESIAN_POINT('Ctrl Pts',(-1.36999806084572,-1.,-3.97027773754922));
#47941=CARTESIAN_POINT('Ctrl Pts',(-1.36999806084572,1.,-3.97027773754922));
#47942=CARTESIAN_POINT('Ctrl Pts',(-1.37020239094758,-1.,-3.9687184694173));
#47943=CARTESIAN_POINT('Ctrl Pts',(-1.37020239094758,1.,-3.9687184694173));
#47944=CARTESIAN_POINT('Ctrl Pts',(-1.37060761746027,-1.,-3.96560037975788));
#47945=CARTESIAN_POINT('Ctrl Pts',(-1.37060761746027,1.,-3.96560037975788));
#47946=CARTESIAN_POINT('Ctrl Pts',(-1.37120515615663,-1.,-3.96092458508407));
#47947=CARTESIAN_POINT('Ctrl Pts',(-1.37120515615663,1.,-3.96092458508407));
#47948=CARTESIAN_POINT('Ctrl Pts',(-1.37198126433139,-1.,-3.95469287283105));
#47949=CARTESIAN_POINT('Ctrl Pts',(-1.37198126433139,1.,-3.95469287283105));
#47950=CARTESIAN_POINT('Ctrl Pts',(-1.37291699203423,-1.,-3.94690771786926));
#47951=CARTESIAN_POINT('Ctrl Pts',(-1.37291699203423,1.,-3.94690771786926));
#47952=CARTESIAN_POINT('Ctrl Pts',(-1.37381821967499,-1.,-3.93912709041791));
#47953=CARTESIAN_POINT('Ctrl Pts',(-1.37381821967499,1.,-3.93912709041791));
#47954=CARTESIAN_POINT('Ctrl Pts',(-1.37468482215784,-1.,-3.93135106761941));
#47955=CARTESIAN_POINT('Ctrl Pts',(-1.37468482215784,1.,-3.93135106761941));
#47956=CARTESIAN_POINT('Ctrl Pts',(-1.37551664448057,-1.,-3.92357976987132));
#47957=CARTESIAN_POINT('Ctrl Pts',(-1.37551664448057,1.,-3.92357976987132));
#47958=CARTESIAN_POINT('Ctrl Pts',(-1.37631350505516,-1.,-3.91581337461825));
#47959=CARTESIAN_POINT('Ctrl Pts',(-1.37631350505516,1.,-3.91581337461825));
#47960=CARTESIAN_POINT('Ctrl Pts',(-1.3770751963376,-1.,-3.90805209522729));
#47961=CARTESIAN_POINT('Ctrl Pts',(-1.3770751963376,1.,-3.90805209522729));
#47962=CARTESIAN_POINT('Ctrl Pts',(-1.3778014851263,-1.,-3.90029615196255));
#47963=CARTESIAN_POINT('Ctrl Pts',(-1.3778014851263,1.,-3.90029615196255));
#47964=CARTESIAN_POINT('Ctrl Pts',(-1.37849211287981,-1.,-3.89254574338385));
#47965=CARTESIAN_POINT('Ctrl Pts',(-1.37849211287981,1.,-3.89254574338385));
#47966=CARTESIAN_POINT('Ctrl Pts',(-1.37914679719446,-1.,-3.88480102249461));
#47967=CARTESIAN_POINT('Ctrl Pts',(-1.37914679719446,1.,-3.88480102249461));
#47968=CARTESIAN_POINT('Ctrl Pts',(-1.37976523097187,-1.,-3.87706205830865));
#47969=CARTESIAN_POINT('Ctrl Pts',(-1.37976523097187,1.,-3.87706205830865));
#47970=CARTESIAN_POINT('Ctrl Pts',(-1.38034709213129,-1.,-3.86932885813403));
#47971=CARTESIAN_POINT('Ctrl Pts',(-1.38034709213129,1.,-3.86932885813403));
#47972=CARTESIAN_POINT('Ctrl Pts',(-1.38089205993067,-1.,-3.86160143044187));
#47973=CARTESIAN_POINT('Ctrl Pts',(-1.38089205993067,1.,-3.86160143044187));
#47974=CARTESIAN_POINT('Ctrl Pts',(-1.38139983115075,-1.,-3.85387983979557));
#47975=CARTESIAN_POINT('Ctrl Pts',(-1.38139983115075,1.,-3.85387983979557));
#47976=CARTESIAN_POINT('Ctrl Pts',(-1.38187013346089,-1.,-3.84616425605705));
#47977=CARTESIAN_POINT('Ctrl Pts',(-1.38187013346089,1.,-3.84616425605705));
#47978=CARTESIAN_POINT('Ctrl Pts',(-1.38230274828774,-1.,-3.83845502790609));
#47979=CARTESIAN_POINT('Ctrl Pts',(-1.38230274828774,1.,-3.83845502790609));
#47980=CARTESIAN_POINT('Ctrl Pts',(-1.38269750245086,-1.,-3.83075266982138));
#47981=CARTESIAN_POINT('Ctrl Pts',(-1.38269750245086,1.,-3.83075266982138));
#47982=CARTESIAN_POINT('Ctrl Pts',(-1.38305421262724,-1.,-3.82305771743715));
#47983=CARTESIAN_POINT('Ctrl Pts',(-1.38305421262724,1.,-3.82305771743715));
#47984=CARTESIAN_POINT('Ctrl Pts',(-1.38337263902766,-1.,-3.81537060817765));
#47985=CARTESIAN_POINT('Ctrl Pts',(-1.38337263902766,1.,-3.81537060817765));
#47986=CARTESIAN_POINT('Ctrl Pts',(-1.38365244046226,-1.,-3.80769156398429));
#47987=CARTESIAN_POINT('Ctrl Pts',(-1.38365244046226,1.,-3.80769156398429));
#47988=CARTESIAN_POINT('Ctrl Pts',(-1.38389311766701,-1.,-3.80002044322169));
#47989=CARTESIAN_POINT('Ctrl Pts',(-1.38389311766701,1.,-3.80002044322169));
#47990=CARTESIAN_POINT('Ctrl Pts',(-1.38409399694589,-1.,-3.79235669640907));
#47991=CARTESIAN_POINT('Ctrl Pts',(-1.38409399694589,1.,-3.79235669640907));
#47992=CARTESIAN_POINT('Ctrl Pts',(-1.38425435883773,-1.,-3.78469969805134));
#47993=CARTESIAN_POINT('Ctrl Pts',(-1.38425435883773,1.,-3.78469969805134));
#47994=CARTESIAN_POINT('Ctrl Pts',(-1.38437354551435,-1.,-3.77704902230441));
#47995=CARTESIAN_POINT('Ctrl Pts',(-1.38437354551435,1.,-3.77704902230441));
#47996=CARTESIAN_POINT('Ctrl Pts',(-1.38445107339517,-1.,-3.76940473185775));
#47997=CARTESIAN_POINT('Ctrl Pts',(-1.38445107339517,1.,-3.76940473185775));
#47998=CARTESIAN_POINT('Ctrl Pts',(-1.38448675253343,-1.,-3.76176768271347));
#47999=CARTESIAN_POINT('Ctrl Pts',(-1.38448675253343,1.,-3.76176768271347));
#48000=CARTESIAN_POINT('Ctrl Pts',(-1.38448077997155,-1.,-3.75413976318727));
#48001=CARTESIAN_POINT('Ctrl Pts',(-1.38448077997155,1.,-3.75413976318727));
#48002=CARTESIAN_POINT('Ctrl Pts',(-1.38443344984389,-1.,-3.7465231716786));
#48003=CARTESIAN_POINT('Ctrl Pts',(-1.38443344984389,1.,-3.7465231716786));
#48004=CARTESIAN_POINT('Ctrl Pts',(-1.38434489156456,-1.,-3.73891976418099));
#48005=CARTESIAN_POINT('Ctrl Pts',(-1.38434489156456,1.,-3.73891976418099));
#48006=CARTESIAN_POINT('Ctrl Pts',(-1.38421479111531,-1.,-3.73133035859283));
#48007=CARTESIAN_POINT('Ctrl Pts',(-1.38421479111531,1.,-3.73133035859283));
#48008=CARTESIAN_POINT('Ctrl Pts',(-1.3840421342895,-1.,-3.72375409358805));
#48009=CARTESIAN_POINT('Ctrl Pts',(-1.3840421342895,1.,-3.72375409358805));
#48010=CARTESIAN_POINT('Ctrl Pts',(-1.38382489984585,-1.,-3.7161876605181));
#48011=CARTESIAN_POINT('Ctrl Pts',(-1.38382489984585,1.,-3.7161876605181));
#48012=CARTESIAN_POINT('Ctrl Pts',(-1.38356065402122,-1.,-3.70862680753343));
#48013=CARTESIAN_POINT('Ctrl Pts',(-1.38356065402122,1.,-3.70862680753343));
#48014=CARTESIAN_POINT('Ctrl Pts',(-1.38324717612862,-1.,-3.70106792167894));
#48015=CARTESIAN_POINT('Ctrl Pts',(-1.38324717612862,1.,-3.70106792167894));
#48016=CARTESIAN_POINT('Ctrl Pts',(-1.38288311171649,-1.,-3.69350967899523));
#48017=CARTESIAN_POINT('Ctrl Pts',(-1.38288311171649,1.,-3.69350967899523));
#48018=CARTESIAN_POINT('Ctrl Pts',(-1.38246852827185,-1.,-3.68595444983844));
#48019=CARTESIAN_POINT('Ctrl Pts',(-1.38246852827185,1.,-3.68595444983844));
#48020=CARTESIAN_POINT('Ctrl Pts',(-1.38200574290626,-1.,-3.6784103848243));
#48021=CARTESIAN_POINT('Ctrl Pts',(-1.38200574290626,1.,-3.6784103848243));
#48022=CARTESIAN_POINT('Ctrl Pts',(-1.38149812653876,-1.,-3.67088843112282));
#48023=CARTESIAN_POINT('Ctrl Pts',(-1.38149812653876,1.,-3.67088843112282));
#48024=CARTESIAN_POINT('Ctrl Pts',(-1.38094856333558,-1.,-3.66339848520874));
#48025=CARTESIAN_POINT('Ctrl Pts',(-1.38094856333558,1.,-3.66339848520874));
#48026=CARTESIAN_POINT('Ctrl Pts',(-1.38035791051215,-1.,-3.65594554404396));
#48027=CARTESIAN_POINT('Ctrl Pts',(-1.38035791051215,1.,-3.65594554404396));
#48028=CARTESIAN_POINT('Ctrl Pts',(-1.37972372481598,-1.,-3.64852652756444));
#48029=CARTESIAN_POINT('Ctrl Pts',(-1.37972372481598,1.,-3.64852652756444));
#48030=CARTESIAN_POINT('Ctrl Pts',(-1.37903818567347,-1.,-3.64112507791112));
#48031=CARTESIAN_POINT('Ctrl Pts',(-1.37903818567347,1.,-3.64112507791112));
#48032=CARTESIAN_POINT('Ctrl Pts',(-1.37829035457324,-1.,-3.63371727442448));
#48033=CARTESIAN_POINT('Ctrl Pts',(-1.37829035457324,1.,-3.63371727442448));
#48034=CARTESIAN_POINT('Ctrl Pts',(-1.37746987919868,-1.,-3.62628098665112));
#48035=CARTESIAN_POINT('Ctrl Pts',(-1.37746987919868,1.,-3.62628098665112));
#48036=CARTESIAN_POINT('Ctrl Pts',(-1.37657053403102,-1.,-3.61880481160408));
#48037=CARTESIAN_POINT('Ctrl Pts',(-1.37657053403102,1.,-3.61880481160408));
#48038=CARTESIAN_POINT('Ctrl Pts',(-1.37559314436641,-1.,-3.61129546591082));
#48039=CARTESIAN_POINT('Ctrl Pts',(-1.37559314436641,1.,-3.61129546591082));
#48040=CARTESIAN_POINT('Ctrl Pts',(-1.37455051379642,-1.,-3.60379020124038));
#48041=CARTESIAN_POINT('Ctrl Pts',(-1.37455051379642,1.,-3.60379020124038));
#48042=CARTESIAN_POINT('Ctrl Pts',(-1.37346320103184,-1.,-3.59634627869117));
#48043=CARTESIAN_POINT('Ctrl Pts',(-1.37346320103184,1.,-3.59634627869117));
#48044=CARTESIAN_POINT('Ctrl Pts',(-1.37235053661,-1.,-3.5890185384643));
#48045=CARTESIAN_POINT('Ctrl Pts',(-1.37235053661,1.,-3.5890185384643));
#48046=CARTESIAN_POINT('Ctrl Pts',(-1.37122241663073,-1.,-3.58183885982745));
#48047=CARTESIAN_POINT('Ctrl Pts',(-1.37122241663073,1.,-3.58183885982745));
#48048=CARTESIAN_POINT('Ctrl Pts',(-1.37007229485646,-1.,-3.57479875549453));
#48049=CARTESIAN_POINT('Ctrl Pts',(-1.37007229485646,1.,-3.57479875549453));
#48050=CARTESIAN_POINT('Ctrl Pts',(-1.36886584973349,-1.,-3.56782080304554));
#48051=CARTESIAN_POINT('Ctrl Pts',(-1.36886584973349,1.,-3.56782080304554));
#48052=CARTESIAN_POINT('Ctrl Pts',(-1.36754771771174,-1.,-3.56077662028492));
#48053=CARTESIAN_POINT('Ctrl Pts',(-1.36754771771174,1.,-3.56077662028492));
#48054=CARTESIAN_POINT('Ctrl Pts',(-1.36606145456711,-1.,-3.55353883995793));
#48055=CARTESIAN_POINT('Ctrl Pts',(-1.36606145456711,1.,-3.55353883995793));
#48056=CARTESIAN_POINT('Ctrl Pts',(-1.36436666257567,-1.,-3.54602591832893));
#48057=CARTESIAN_POINT('Ctrl Pts',(-1.36436666257567,1.,-3.54602591832893));
#48058=CARTESIAN_POINT('Ctrl Pts',(-1.36245507339334,-1.,-3.53824396425032));
#48059=CARTESIAN_POINT('Ctrl Pts',(-1.36245507339334,1.,-3.53824396425032));
#48060=CARTESIAN_POINT('Ctrl Pts',(-1.36037259643827,-1.,-3.53034464961849));
#48061=CARTESIAN_POINT('Ctrl Pts',(-1.36037259643827,1.,-3.53034464961849));
#48062=CARTESIAN_POINT('Ctrl Pts',(-1.35821701528975,-1.,-3.52261776117121));
#48063=CARTESIAN_POINT('Ctrl Pts',(-1.35821701528975,1.,-3.52261776117121));
#48064=CARTESIAN_POINT('Ctrl Pts',(-1.35611275237288,-1.,-3.51542230699919));
#48065=CARTESIAN_POINT('Ctrl Pts',(-1.35611275237288,1.,-3.51542230699919));
#48066=CARTESIAN_POINT('Ctrl Pts',(-1.35419113576022,-1.,-3.50913227060177));
#48067=CARTESIAN_POINT('Ctrl Pts',(-1.35419113576022,1.,-3.50913227060177));
#48068=CARTESIAN_POINT('Ctrl Pts',(-1.3525703284343,-1.,-3.50408168106113));
#48069=CARTESIAN_POINT('Ctrl Pts',(-1.3525703284343,1.,-3.50408168106113));
#48070=CARTESIAN_POINT('Ctrl Pts',(-1.35133076331065,-1.,-3.50049707063673));
#48071=CARTESIAN_POINT('Ctrl Pts',(-1.35133076331065,1.,-3.50049707063673));
#48072=CARTESIAN_POINT('Ctrl Pts',(-1.35067437417289,-1.,-3.49888720256612));
#48073=CARTESIAN_POINT('Ctrl Pts',(-1.35067437417289,1.,-3.49888720256612));
#48074=CARTESIAN_POINT('Ctrl Pts',(-1.35037650302887,-1.,-3.49840357193384));
#48075=CARTESIAN_POINT('Ctrl Pts',(-1.35037650302887,1.,-3.49840357193384));
#48076=CARTESIAN_POINT('Ctrl Pts',(-1.35026426118351,-1.,-3.49840260053616));
#48077=CARTESIAN_POINT('Ctrl Pts',(-1.35026426118351,1.,-3.49840260053616));
#48078=CARTESIAN_POINT('Ctrl Pts',(-1.35022972712301,-1.,-3.49848248301936));
#48079=CARTESIAN_POINT('Ctrl Pts',(-1.35022972712301,1.,-3.49848248301936));
#48080=CARTESIAN_POINT('',(-1.36999806084572,1.,-3.97027773754922));
#48081=CARTESIAN_POINT('Ctrl Pts',(-1.36999806084572,1.,-3.97027773754922));
#48082=CARTESIAN_POINT('Ctrl Pts',(-1.37020239094758,1.,-3.9687184694173));
#48083=CARTESIAN_POINT('Ctrl Pts',(-1.37060761746027,1.,-3.96560037975788));
#48084=CARTESIAN_POINT('Ctrl Pts',(-1.37120515615663,1.,-3.96092458508407));
#48085=CARTESIAN_POINT('Ctrl Pts',(-1.37198126433139,1.,-3.95469287283105));
#48086=CARTESIAN_POINT('Ctrl Pts',(-1.37291699203423,1.,-3.94690771786926));
#48087=CARTESIAN_POINT('Ctrl Pts',(-1.37381821967499,1.,-3.93912709041791));
#48088=CARTESIAN_POINT('Ctrl Pts',(-1.37468482215784,1.,-3.93135106761941));
#48089=CARTESIAN_POINT('Ctrl Pts',(-1.37551664448057,1.,-3.92357976987132));
#48090=CARTESIAN_POINT('Ctrl Pts',(-1.37631350505516,1.,-3.91581337461825));
#48091=CARTESIAN_POINT('Ctrl Pts',(-1.3770751963376,1.,-3.90805209522729));
#48092=CARTESIAN_POINT('Ctrl Pts',(-1.3778014851263,1.,-3.90029615196255));
#48093=CARTESIAN_POINT('Ctrl Pts',(-1.37849211287981,1.,-3.89254574338385));
#48094=CARTESIAN_POINT('Ctrl Pts',(-1.37914679719446,1.,-3.88480102249461));
#48095=CARTESIAN_POINT('Ctrl Pts',(-1.37976523097187,1.,-3.87706205830865));
#48096=CARTESIAN_POINT('Ctrl Pts',(-1.38034709213129,1.,-3.86932885813403));
#48097=CARTESIAN_POINT('Ctrl Pts',(-1.38089205993067,1.,-3.86160143044187));
#48098=CARTESIAN_POINT('Ctrl Pts',(-1.38139983115075,1.,-3.85387983979557));
#48099=CARTESIAN_POINT('Ctrl Pts',(-1.38187013346089,1.,-3.84616425605705));
#48100=CARTESIAN_POINT('Ctrl Pts',(-1.38230274828774,1.,-3.83845502790609));
#48101=CARTESIAN_POINT('Ctrl Pts',(-1.38269750245086,1.,-3.83075266982138));
#48102=CARTESIAN_POINT('Ctrl Pts',(-1.38305421262724,1.,-3.82305771743715));
#48103=CARTESIAN_POINT('Ctrl Pts',(-1.38337263902766,1.,-3.81537060817765));
#48104=CARTESIAN_POINT('Ctrl Pts',(-1.38365244046226,1.,-3.80769156398429));
#48105=CARTESIAN_POINT('Ctrl Pts',(-1.38389311766701,1.,-3.80002044322169));
#48106=CARTESIAN_POINT('Ctrl Pts',(-1.38409399694589,1.,-3.79235669640907));
#48107=CARTESIAN_POINT('Ctrl Pts',(-1.38425435883773,1.,-3.78469969805134));
#48108=CARTESIAN_POINT('Ctrl Pts',(-1.38437354551435,1.,-3.77704902230441));
#48109=CARTESIAN_POINT('Ctrl Pts',(-1.38445107339517,1.,-3.76940473185775));
#48110=CARTESIAN_POINT('Ctrl Pts',(-1.38448675253343,1.,-3.76176768271347));
#48111=CARTESIAN_POINT('Ctrl Pts',(-1.38448077997155,1.,-3.75413976318727));
#48112=CARTESIAN_POINT('Ctrl Pts',(-1.38443344984389,1.,-3.7465231716786));
#48113=CARTESIAN_POINT('Ctrl Pts',(-1.38434489156456,1.,-3.73891976418099));
#48114=CARTESIAN_POINT('Ctrl Pts',(-1.38421479111531,1.,-3.73133035859283));
#48115=CARTESIAN_POINT('Ctrl Pts',(-1.3840421342895,1.,-3.72375409358805));
#48116=CARTESIAN_POINT('Ctrl Pts',(-1.38382489984585,1.,-3.7161876605181));
#48117=CARTESIAN_POINT('Ctrl Pts',(-1.38356065402122,1.,-3.70862680753343));
#48118=CARTESIAN_POINT('Ctrl Pts',(-1.38324717612862,1.,-3.70106792167894));
#48119=CARTESIAN_POINT('Ctrl Pts',(-1.38288311171649,1.,-3.69350967899523));
#48120=CARTESIAN_POINT('Ctrl Pts',(-1.38246852827185,1.,-3.68595444983844));
#48121=CARTESIAN_POINT('Ctrl Pts',(-1.38200574290626,1.,-3.6784103848243));
#48122=CARTESIAN_POINT('Ctrl Pts',(-1.38149812653876,1.,-3.67088843112282));
#48123=CARTESIAN_POINT('Ctrl Pts',(-1.38094856333558,1.,-3.66339848520874));
#48124=CARTESIAN_POINT('Ctrl Pts',(-1.38035791051215,1.,-3.65594554404396));
#48125=CARTESIAN_POINT('Ctrl Pts',(-1.37972372481598,1.,-3.64852652756444));
#48126=CARTESIAN_POINT('Ctrl Pts',(-1.37903818567347,1.,-3.64112507791112));
#48127=CARTESIAN_POINT('Ctrl Pts',(-1.37829035457324,1.,-3.63371727442448));
#48128=CARTESIAN_POINT('Ctrl Pts',(-1.37746987919868,1.,-3.62628098665112));
#48129=CARTESIAN_POINT('Ctrl Pts',(-1.37657053403102,1.,-3.61880481160408));
#48130=CARTESIAN_POINT('Ctrl Pts',(-1.37559314436641,1.,-3.61129546591082));
#48131=CARTESIAN_POINT('Ctrl Pts',(-1.37455051379642,1.,-3.60379020124038));
#48132=CARTESIAN_POINT('Ctrl Pts',(-1.37346320103184,1.,-3.59634627869117));
#48133=CARTESIAN_POINT('Ctrl Pts',(-1.37235053661,1.,-3.5890185384643));
#48134=CARTESIAN_POINT('Ctrl Pts',(-1.37122241663073,1.,-3.58183885982745));
#48135=CARTESIAN_POINT('Ctrl Pts',(-1.37007229485646,1.,-3.57479875549453));
#48136=CARTESIAN_POINT('Ctrl Pts',(-1.36886584973349,1.,-3.56782080304554));
#48137=CARTESIAN_POINT('Ctrl Pts',(-1.36754771771174,1.,-3.56077662028492));
#48138=CARTESIAN_POINT('Ctrl Pts',(-1.36606145456711,1.,-3.55353883995793));
#48139=CARTESIAN_POINT('Ctrl Pts',(-1.36436666257567,1.,-3.54602591832893));
#48140=CARTESIAN_POINT('Ctrl Pts',(-1.36245507339334,1.,-3.53824396425032));
#48141=CARTESIAN_POINT('Ctrl Pts',(-1.36037259643827,1.,-3.53034464961849));
#48142=CARTESIAN_POINT('Ctrl Pts',(-1.35821701528975,1.,-3.52261776117121));
#48143=CARTESIAN_POINT('Ctrl Pts',(-1.35611275237288,1.,-3.51542230699919));
#48144=CARTESIAN_POINT('Ctrl Pts',(-1.35419113576022,1.,-3.50913227060177));
#48145=CARTESIAN_POINT('Ctrl Pts',(-1.3525703284343,1.,-3.50408168106113));
#48146=CARTESIAN_POINT('Ctrl Pts',(-1.35142377279535,1.,-3.5007660381658));
#48147=CARTESIAN_POINT('Ctrl Pts',(-1.35080045218652,1.,-3.49920025459856));
#48148=CARTESIAN_POINT('Ctrl Pts',(-1.35049736560633,1.,-3.49861894124915));
#48149=CARTESIAN_POINT('Ctrl Pts',(-1.35036670893102,1.,-3.49847119623841));
#48150=CARTESIAN_POINT('Ctrl Pts',(-1.35032489087269,1.,-3.49844575334386));
#48151=CARTESIAN_POINT('',(-1.36999806084572,0.,-3.97027773754922));
#48152=CARTESIAN_POINT('Ctrl Pts',(-0.96399761336957,-1.,-3.62397690409552));
#48153=CARTESIAN_POINT('Ctrl Pts',(-0.96399761336957,1.,-3.62397690409552));
#48154=CARTESIAN_POINT('Ctrl Pts',(-0.963922720982576,-1.,-3.62393257642191));
#48155=CARTESIAN_POINT('Ctrl Pts',(-0.963922720982576,1.,-3.62393257642191));
#48156=CARTESIAN_POINT('Ctrl Pts',(-0.963832486396055,-1.,-3.62399933640277));
#48157=CARTESIAN_POINT('Ctrl Pts',(-0.963832486396055,1.,-3.62399933640277));
#48158=CARTESIAN_POINT('Ctrl Pts',(-0.963875774532103,-1.,-3.62456568607055));
#48159=CARTESIAN_POINT('Ctrl Pts',(-0.963875774532103,1.,-3.62456568607055));
#48160=CARTESIAN_POINT('Ctrl Pts',(-0.964291001274618,-1.,-3.62625391255277));
#48161=CARTESIAN_POINT('Ctrl Pts',(-0.964291001274618,1.,-3.62625391255277));
#48162=CARTESIAN_POINT('Ctrl Pts',(-0.965395153165716,-1.,-3.62988252139998));
#48163=CARTESIAN_POINT('Ctrl Pts',(-0.965395153165716,1.,-3.62988252139998));
#48164=CARTESIAN_POINT('Ctrl Pts',(-0.967052554540877,-1.,-3.6349212208096));
#48165=CARTESIAN_POINT('Ctrl Pts',(-0.967052554540877,1.,-3.6349212208096));
#48166=CARTESIAN_POINT('Ctrl Pts',(-0.969195124674829,-1.,-3.64113946505393));
#48167=CARTESIAN_POINT('Ctrl Pts',(-0.969195124674829,1.,-3.64113946505393));
#48168=CARTESIAN_POINT('Ctrl Pts',(-0.971722122060277,-1.,-3.64819756447072));
#48169=CARTESIAN_POINT('Ctrl Pts',(-0.971722122060277,1.,-3.64819756447072));
#48170=CARTESIAN_POINT('Ctrl Pts',(-0.974519971354139,-1.,-3.6557157673487));
#48171=CARTESIAN_POINT('Ctrl Pts',(-0.974519971354139,1.,-3.6557157673487));
#48172=CARTESIAN_POINT('Ctrl Pts',(-0.977478312751416,-1.,-3.66333049637403));
#48173=CARTESIAN_POINT('Ctrl Pts',(-0.977478312751416,1.,-3.66333049637403));
#48174=CARTESIAN_POINT('Ctrl Pts',(-0.980505922458494,-1.,-3.67074983340444));
#48175=CARTESIAN_POINT('Ctrl Pts',(-0.980505922458494,1.,-3.67074983340444));
#48176=CARTESIAN_POINT('Ctrl Pts',(-0.983550791470864,-1.,-3.67782408841876));
#48177=CARTESIAN_POINT('Ctrl Pts',(-0.983550791470864,1.,-3.67782408841876));
#48178=CARTESIAN_POINT('Ctrl Pts',(-0.986602639864286,-1.,-3.6845531792623));
#48179=CARTESIAN_POINT('Ctrl Pts',(-0.986602639864286,1.,-3.6845531792623));
#48180=CARTESIAN_POINT('Ctrl Pts',(-0.989676715398858,-1.,-3.69102682138955));
#48181=CARTESIAN_POINT('Ctrl Pts',(-0.989676715398858,1.,-3.69102682138955));
#48182=CARTESIAN_POINT('Ctrl Pts',(-0.992802218332104,-1.,-3.69738123415696));
#48183=CARTESIAN_POINT('Ctrl Pts',(-0.992802218332104,1.,-3.69738123415696));
#48184=CARTESIAN_POINT('Ctrl Pts',(-0.996009819772432,-1.,-3.70375282282107));
#48185=CARTESIAN_POINT('Ctrl Pts',(-0.996009819772432,1.,-3.70375282282107));
#48186=CARTESIAN_POINT('Ctrl Pts',(-0.999317260756344,-1.,-3.7102243971387));
#48187=CARTESIAN_POINT('Ctrl Pts',(-0.999317260756344,1.,-3.7102243971387));
#48188=CARTESIAN_POINT('Ctrl Pts',(-1.00272423396802,-1.,-3.71680667125047));
#48189=CARTESIAN_POINT('Ctrl Pts',(-1.00272423396802,1.,-3.71680667125047));
#48190=CARTESIAN_POINT('Ctrl Pts',(-1.00622000735696,-1.,-3.72346803750544));
#48191=CARTESIAN_POINT('Ctrl Pts',(-1.00622000735696,1.,-3.72346803750544));
#48192=CARTESIAN_POINT('Ctrl Pts',(-1.00978798539491,-1.,-3.73015276704407));
#48193=CARTESIAN_POINT('Ctrl Pts',(-1.00978798539491,1.,-3.73015276704407));
#48194=CARTESIAN_POINT('Ctrl Pts',(-1.01341114319906,-1.,-3.73680245055747));
#48195=CARTESIAN_POINT('Ctrl Pts',(-1.01341114319906,1.,-3.73680245055747));
#48196=CARTESIAN_POINT('Ctrl Pts',(-1.01707794311088,-1.,-3.74337942504993));
#48197=CARTESIAN_POINT('Ctrl Pts',(-1.01707794311088,1.,-3.74337942504993));
#48198=CARTESIAN_POINT('Ctrl Pts',(-1.02078510487439,-1.,-3.74987777155873));
#48199=CARTESIAN_POINT('Ctrl Pts',(-1.02078510487439,1.,-3.74987777155873));
#48200=CARTESIAN_POINT('Ctrl Pts',(-1.02453429444668,-1.,-3.75631037456224));
#48201=CARTESIAN_POINT('Ctrl Pts',(-1.02453429444668,1.,-3.75631037456224));
#48202=CARTESIAN_POINT('Ctrl Pts',(-1.02833014458184,-1.,-3.76270122291245));
#48203=CARTESIAN_POINT('Ctrl Pts',(-1.02833014458184,1.,-3.76270122291245));
#48204=CARTESIAN_POINT('Ctrl Pts',(-1.03217786604919,-1.,-3.76907609832516));
#48205=CARTESIAN_POINT('Ctrl Pts',(-1.03217786604919,1.,-3.76907609832516));
#48206=CARTESIAN_POINT('Ctrl Pts',(-1.03608074678008,-1.,-3.77545283140427));
#48207=CARTESIAN_POINT('Ctrl Pts',(-1.03608074678008,1.,-3.77545283140427));
#48208=CARTESIAN_POINT('Ctrl Pts',(-1.04003862055798,-1.,-3.7818353500817));
#48209=CARTESIAN_POINT('Ctrl Pts',(-1.04003862055798,1.,-3.7818353500817));
#48210=CARTESIAN_POINT('Ctrl Pts',(-1.04404924374422,-1.,-3.78821910787179));
#48211=CARTESIAN_POINT('Ctrl Pts',(-1.04404924374422,1.,-3.78821910787179));
#48212=CARTESIAN_POINT('Ctrl Pts',(-1.04810913267639,-1.,-3.79459440308786));
#48213=CARTESIAN_POINT('Ctrl Pts',(-1.04810913267639,1.,-3.79459440308786));
#48214=CARTESIAN_POINT('Ctrl Pts',(-1.05221457990016,-1.,-3.80095039790681));
#48215=CARTESIAN_POINT('Ctrl Pts',(-1.05221457990016,1.,-3.80095039790681));
#48216=CARTESIAN_POINT('Ctrl Pts',(-1.05636266918644,-1.,-3.80727913637791));
#48217=CARTESIAN_POINT('Ctrl Pts',(-1.05636266918644,1.,-3.80727913637791));
#48218=CARTESIAN_POINT('Ctrl Pts',(-1.06055206187299,-1.,-3.8135786611749));
#48219=CARTESIAN_POINT('Ctrl Pts',(-1.06055206187299,1.,-3.8135786611749));
#48220=CARTESIAN_POINT('Ctrl Pts',(-1.0647824403893,-1.,-3.81985083953012));
#48221=CARTESIAN_POINT('Ctrl Pts',(-1.0647824403893,1.,-3.81985083953012));
#48222=CARTESIAN_POINT('Ctrl Pts',(-1.06905413180359,-1.,-3.82609989967276));
#48223=CARTESIAN_POINT('Ctrl Pts',(-1.06905413180359,1.,-3.82609989967276));
#48224=CARTESIAN_POINT('Ctrl Pts',(-1.07336766633459,-1.,-3.83233071195144));
#48225=CARTESIAN_POINT('Ctrl Pts',(-1.07336766633459,1.,-3.83233071195144));
#48226=CARTESIAN_POINT('Ctrl Pts',(-1.07772335353858,-1.,-3.83854714117491));
#48227=CARTESIAN_POINT('Ctrl Pts',(-1.07772335353858,1.,-3.83854714117491));
#48228=CARTESIAN_POINT('Ctrl Pts',(-1.08212087917991,-1.,-3.8447504803063));
#48229=CARTESIAN_POINT('Ctrl Pts',(-1.08212087917991,1.,-3.8447504803063));
#48230=CARTESIAN_POINT('Ctrl Pts',(-1.08655950846384,-1.,-3.85094025222713));
#48231=CARTESIAN_POINT('Ctrl Pts',(-1.08655950846384,1.,-3.85094025222713));
#48232=CARTESIAN_POINT('Ctrl Pts',(-1.09103825516294,-1.,-3.85711487933931));
#48233=CARTESIAN_POINT('Ctrl Pts',(-1.09103825516294,1.,-3.85711487933931));
#48234=CARTESIAN_POINT('Ctrl Pts',(-1.09555606505013,-1.,-3.86327241021247));
#48235=CARTESIAN_POINT('Ctrl Pts',(-1.09555606505013,1.,-3.86327241021247));
#48236=CARTESIAN_POINT('Ctrl Pts',(-1.10011198761195,-1.,-3.86941120134849));
#48237=CARTESIAN_POINT('Ctrl Pts',(-1.10011198761195,1.,-3.86941120134849));
#48238=CARTESIAN_POINT('Ctrl Pts',(-1.10470536603287,-1.,-3.87553067187514));
#48239=CARTESIAN_POINT('Ctrl Pts',(-1.10470536603287,1.,-3.87553067187514));
#48240=CARTESIAN_POINT('Ctrl Pts',(-1.10933577224008,-1.,-3.88163105531724));
#48241=CARTESIAN_POINT('Ctrl Pts',(-1.10933577224008,1.,-3.88163105531724));
#48242=CARTESIAN_POINT('Ctrl Pts',(-1.11400292434429,-1.,-3.88771308285171));
#48243=CARTESIAN_POINT('Ctrl Pts',(-1.11400292434429,1.,-3.88771308285171));
#48244=CARTESIAN_POINT('Ctrl Pts',(-1.11870660794603,-1.,-3.89377768340344));
#48245=CARTESIAN_POINT('Ctrl Pts',(-1.11870660794603,1.,-3.89377768340344));
#48246=CARTESIAN_POINT('Ctrl Pts',(-1.12344660099043,-1.,-3.89982569750025));
#48247=CARTESIAN_POINT('Ctrl Pts',(-1.12344660099043,1.,-3.89982569750025));
#48248=CARTESIAN_POINT('Ctrl Pts',(-1.12822258281553,-1.,-3.90585753318737));
#48249=CARTESIAN_POINT('Ctrl Pts',(-1.12822258281553,1.,-3.90585753318737));
#48250=CARTESIAN_POINT('Ctrl Pts',(-1.13303414693896,-1.,-3.91187321145649));
#48251=CARTESIAN_POINT('Ctrl Pts',(-1.13303414693896,1.,-3.91187321145649));
#48252=CARTESIAN_POINT('Ctrl Pts',(-1.13788084225554,-1.,-3.91787251936827));
#48253=CARTESIAN_POINT('Ctrl Pts',(-1.13788084225554,1.,-3.91787251936827));
#48254=CARTESIAN_POINT('Ctrl Pts',(-1.14276220561593,-1.,-3.92385513133997));
#48255=CARTESIAN_POINT('Ctrl Pts',(-1.14276220561593,1.,-3.92385513133997));
#48256=CARTESIAN_POINT('Ctrl Pts',(-1.14767779451123,-1.,-3.92982073294257));
#48257=CARTESIAN_POINT('Ctrl Pts',(-1.14767779451123,1.,-3.92982073294257));
#48258=CARTESIAN_POINT('Ctrl Pts',(-1.1526272271632,-1.,-3.9357691705628));
#48259=CARTESIAN_POINT('Ctrl Pts',(-1.1526272271632,1.,-3.9357691705628));
#48260=CARTESIAN_POINT('Ctrl Pts',(-1.15761018340956,-1.,-3.94170046685203));
#48261=CARTESIAN_POINT('Ctrl Pts',(-1.15761018340956,1.,-3.94170046685203));
#48262=CARTESIAN_POINT('Ctrl Pts',(-1.16262637999157,-1.,-3.94761474780583));
#48263=CARTESIAN_POINT('Ctrl Pts',(-1.16262637999157,1.,-3.94761474780583));
#48264=CARTESIAN_POINT('Ctrl Pts',(-1.16767555244438,-1.,-3.95351219509876));
#48265=CARTESIAN_POINT('Ctrl Pts',(-1.16767555244438,1.,-3.95351219509876));
#48266=CARTESIAN_POINT('Ctrl Pts',(-1.17275743590361,-1.,-3.95939299213276));
#48267=CARTESIAN_POINT('Ctrl Pts',(-1.17275743590361,1.,-3.95939299213276));
#48268=CARTESIAN_POINT('Ctrl Pts',(-1.17787174135592,-1.,-3.96525726358159));
#48269=CARTESIAN_POINT('Ctrl Pts',(-1.17787174135592,1.,-3.96525726358159));
#48270=CARTESIAN_POINT('Ctrl Pts',(-1.18301815039831,-1.,-3.97110505165415));
#48271=CARTESIAN_POINT('Ctrl Pts',(-1.18301815039831,1.,-3.97110505165415));
#48272=CARTESIAN_POINT('Ctrl Pts',(-1.18819633715539,-1.,-3.97693634767754));
#48273=CARTESIAN_POINT('Ctrl Pts',(-1.18819633715539,1.,-3.97693634767754));
#48274=CARTESIAN_POINT('Ctrl Pts',(-1.19340598349475,-1.,-3.98275111052561));
#48275=CARTESIAN_POINT('Ctrl Pts',(-1.19340598349475,1.,-3.98275111052561));
#48276=CARTESIAN_POINT('Ctrl Pts',(-1.19864679609566,-1.,-3.98854928957189));
#48277=CARTESIAN_POINT('Ctrl Pts',(-1.19864679609566,1.,-3.98854928957189));
#48278=CARTESIAN_POINT('Ctrl Pts',(-1.20391852375139,-1.,-3.99433084799666));
#48279=CARTESIAN_POINT('Ctrl Pts',(-1.20391852375139,1.,-3.99433084799666));
#48280=CARTESIAN_POINT('Ctrl Pts',(-1.20922097029551,-1.,-4.00009577950721));
#48281=CARTESIAN_POINT('Ctrl Pts',(-1.20922097029551,1.,-4.00009577950721));
#48282=CARTESIAN_POINT('Ctrl Pts',(-1.21455398918133,-1.,-4.00584409522722));
#48283=CARTESIAN_POINT('Ctrl Pts',(-1.21455398918133,1.,-4.00584409522722));
#48284=CARTESIAN_POINT('Ctrl Pts',(-1.21884478244403,-1.,-4.01042947140789));
#48285=CARTESIAN_POINT('Ctrl Pts',(-1.21884478244403,1.,-4.01042947140789));
#48286=CARTESIAN_POINT('Ctrl Pts',(-1.22207656455845,-1.,-4.01386104433519));
#48287=CARTESIAN_POINT('Ctrl Pts',(-1.22207656455845,1.,-4.01386104433519));
#48288=CARTESIAN_POINT('Ctrl Pts',(-1.22423716681317,-1.,-4.01614544569895));
#48289=CARTESIAN_POINT('Ctrl Pts',(-1.22423716681317,1.,-4.01614544569895));
#48290=CARTESIAN_POINT('Ctrl Pts',(-1.22531898815164,-1.,-4.01728681790024));
#48291=CARTESIAN_POINT('Ctrl Pts',(-1.22531898815164,1.,-4.01728681790024));
#48292=CARTESIAN_POINT('',(-0.963899035118984,1.,-3.62400312501199));
#48293=CARTESIAN_POINT('Ctrl Pts',(-0.963899035118985,-1.,-3.62400312501199));
#48294=CARTESIAN_POINT('Ctrl Pts',(-0.963899035118985,-0.666666666666667,
-3.62400312501199));
#48295=CARTESIAN_POINT('Ctrl Pts',(-0.963899035118985,-0.333333333333333,
-3.62400312501199));
#48296=CARTESIAN_POINT('Ctrl Pts',(-0.963899035118985,0.333333333333333,
-3.62400312501199));
#48297=CARTESIAN_POINT('Ctrl Pts',(-0.963899035118986,0.666666666666667,
-3.62400312501199));
#48298=CARTESIAN_POINT('Ctrl Pts',(-0.963899035118986,1.,-3.62400312501199));
#48299=CARTESIAN_POINT('',(-1.22531898815164,1.,-4.01728681790024));
#48300=CARTESIAN_POINT('',(-1.22531898815164,0.,-4.01728681790024));
#48301=CARTESIAN_POINT('Ctrl Pts',(-0.963899035118985,1.,-3.62400312501199));
#48302=CARTESIAN_POINT('Ctrl Pts',(-0.963880158556713,1.,-3.62404828878375));
#48303=CARTESIAN_POINT('Ctrl Pts',(-0.963861297423579,1.,-3.62424461507455));
#48304=CARTESIAN_POINT('Ctrl Pts',(-0.963957782642589,1.,-3.62489305727516));
#48305=CARTESIAN_POINT('Ctrl Pts',(-0.964373850166081,1.,-3.62652618145252));
#48306=CARTESIAN_POINT('Ctrl Pts',(-0.965395153165716,1.,-3.62988252139998));
#48307=CARTESIAN_POINT('Ctrl Pts',(-0.967052554540877,1.,-3.6349212208096));
#48308=CARTESIAN_POINT('Ctrl Pts',(-0.969195124674829,1.,-3.64113946505393));
#48309=CARTESIAN_POINT('Ctrl Pts',(-0.971722122060277,1.,-3.64819756447072));
#48310=CARTESIAN_POINT('Ctrl Pts',(-0.974519971354139,1.,-3.6557157673487));
#48311=CARTESIAN_POINT('Ctrl Pts',(-0.977478312751416,1.,-3.66333049637403));
#48312=CARTESIAN_POINT('Ctrl Pts',(-0.980505922458494,1.,-3.67074983340444));
#48313=CARTESIAN_POINT('Ctrl Pts',(-0.983550791470864,1.,-3.67782408841876));
#48314=CARTESIAN_POINT('Ctrl Pts',(-0.986602639864286,1.,-3.6845531792623));
#48315=CARTESIAN_POINT('Ctrl Pts',(-0.989676715398858,1.,-3.69102682138955));
#48316=CARTESIAN_POINT('Ctrl Pts',(-0.992802218332104,1.,-3.69738123415696));
#48317=CARTESIAN_POINT('Ctrl Pts',(-0.996009819772432,1.,-3.70375282282107));
#48318=CARTESIAN_POINT('Ctrl Pts',(-0.999317260756344,1.,-3.7102243971387));
#48319=CARTESIAN_POINT('Ctrl Pts',(-1.00272423396802,1.,-3.71680667125047));
#48320=CARTESIAN_POINT('Ctrl Pts',(-1.00622000735696,1.,-3.72346803750544));
#48321=CARTESIAN_POINT('Ctrl Pts',(-1.00978798539491,1.,-3.73015276704407));
#48322=CARTESIAN_POINT('Ctrl Pts',(-1.01341114319906,1.,-3.73680245055747));
#48323=CARTESIAN_POINT('Ctrl Pts',(-1.01707794311088,1.,-3.74337942504993));
#48324=CARTESIAN_POINT('Ctrl Pts',(-1.02078510487439,1.,-3.74987777155873));
#48325=CARTESIAN_POINT('Ctrl Pts',(-1.02453429444668,1.,-3.75631037456224));
#48326=CARTESIAN_POINT('Ctrl Pts',(-1.02833014458184,1.,-3.76270122291245));
#48327=CARTESIAN_POINT('Ctrl Pts',(-1.03217786604919,1.,-3.76907609832516));
#48328=CARTESIAN_POINT('Ctrl Pts',(-1.03608074678008,1.,-3.77545283140427));
#48329=CARTESIAN_POINT('Ctrl Pts',(-1.04003862055798,1.,-3.7818353500817));
#48330=CARTESIAN_POINT('Ctrl Pts',(-1.04404924374422,1.,-3.78821910787179));
#48331=CARTESIAN_POINT('Ctrl Pts',(-1.04810913267639,1.,-3.79459440308786));
#48332=CARTESIAN_POINT('Ctrl Pts',(-1.05221457990016,1.,-3.80095039790681));
#48333=CARTESIAN_POINT('Ctrl Pts',(-1.05636266918644,1.,-3.80727913637791));
#48334=CARTESIAN_POINT('Ctrl Pts',(-1.06055206187299,1.,-3.8135786611749));
#48335=CARTESIAN_POINT('Ctrl Pts',(-1.0647824403893,1.,-3.81985083953012));
#48336=CARTESIAN_POINT('Ctrl Pts',(-1.06905413180359,1.,-3.82609989967276));
#48337=CARTESIAN_POINT('Ctrl Pts',(-1.07336766633459,1.,-3.83233071195144));
#48338=CARTESIAN_POINT('Ctrl Pts',(-1.07772335353858,1.,-3.83854714117491));
#48339=CARTESIAN_POINT('Ctrl Pts',(-1.08212087917991,1.,-3.8447504803063));
#48340=CARTESIAN_POINT('Ctrl Pts',(-1.08655950846384,1.,-3.85094025222713));
#48341=CARTESIAN_POINT('Ctrl Pts',(-1.09103825516294,1.,-3.85711487933931));
#48342=CARTESIAN_POINT('Ctrl Pts',(-1.09555606505013,1.,-3.86327241021247));
#48343=CARTESIAN_POINT('Ctrl Pts',(-1.10011198761195,1.,-3.86941120134849));
#48344=CARTESIAN_POINT('Ctrl Pts',(-1.10470536603287,1.,-3.87553067187514));
#48345=CARTESIAN_POINT('Ctrl Pts',(-1.10933577224008,1.,-3.88163105531724));
#48346=CARTESIAN_POINT('Ctrl Pts',(-1.11400292434429,1.,-3.88771308285171));
#48347=CARTESIAN_POINT('Ctrl Pts',(-1.11870660794603,1.,-3.89377768340344));
#48348=CARTESIAN_POINT('Ctrl Pts',(-1.12344660099043,1.,-3.89982569750025));
#48349=CARTESIAN_POINT('Ctrl Pts',(-1.12822258281553,1.,-3.90585753318737));
#48350=CARTESIAN_POINT('Ctrl Pts',(-1.13303414693896,1.,-3.91187321145649));
#48351=CARTESIAN_POINT('Ctrl Pts',(-1.13788084225554,1.,-3.91787251936827));
#48352=CARTESIAN_POINT('Ctrl Pts',(-1.14276220561593,1.,-3.92385513133997));
#48353=CARTESIAN_POINT('Ctrl Pts',(-1.14767779451123,1.,-3.92982073294257));
#48354=CARTESIAN_POINT('Ctrl Pts',(-1.1526272271632,1.,-3.9357691705628));
#48355=CARTESIAN_POINT('Ctrl Pts',(-1.15761018340956,1.,-3.94170046685203));
#48356=CARTESIAN_POINT('Ctrl Pts',(-1.16262637999157,1.,-3.94761474780583));
#48357=CARTESIAN_POINT('Ctrl Pts',(-1.16767555244438,1.,-3.95351219509876));
#48358=CARTESIAN_POINT('Ctrl Pts',(-1.17275743590361,1.,-3.95939299213276));
#48359=CARTESIAN_POINT('Ctrl Pts',(-1.17787174135592,1.,-3.96525726358159));
#48360=CARTESIAN_POINT('Ctrl Pts',(-1.18301815039831,1.,-3.97110505165415));
#48361=CARTESIAN_POINT('Ctrl Pts',(-1.18819633715539,1.,-3.97693634767754));
#48362=CARTESIAN_POINT('Ctrl Pts',(-1.19340598349475,1.,-3.98275111052561));
#48363=CARTESIAN_POINT('Ctrl Pts',(-1.19864679609566,1.,-3.98854928957189));
#48364=CARTESIAN_POINT('Ctrl Pts',(-1.20391852375139,1.,-3.99433084799666));
#48365=CARTESIAN_POINT('Ctrl Pts',(-1.20922097029551,1.,-4.00009577950721));
#48366=CARTESIAN_POINT('Ctrl Pts',(-1.21455398918133,1.,-4.00584409522722));
#48367=CARTESIAN_POINT('Ctrl Pts',(-1.21884478244403,1.,-4.01042947140789));
#48368=CARTESIAN_POINT('Ctrl Pts',(-1.22207656455845,1.,-4.01386104433519));
#48369=CARTESIAN_POINT('Ctrl Pts',(-1.22423716681317,1.,-4.01614544569895));
#48370=CARTESIAN_POINT('Ctrl Pts',(-1.22531898815164,1.,-4.01728681790024));
#48371=CARTESIAN_POINT('Origin',(-1.22531898815164,0.,-4.01728681790024));
#48372=CARTESIAN_POINT('',(-1.36999806084572,1.,-3.97027773754922));
#48373=CARTESIAN_POINT('Origin',(0.,0.,0.));
#48374=CARTESIAN_POINT('',(-0.786422660833743,1.,-3.66661143271648));
#48375=CARTESIAN_POINT('Origin',(0.,1.,0.));
#48376=CARTESIAN_POINT('Ctrl Pts',(-0.786422660833742,1.,-3.66661143271648));
#48377=CARTESIAN_POINT('Ctrl Pts',(-0.786422660833742,0.666666666666667,
-3.66661143271648));
#48378=CARTESIAN_POINT('Ctrl Pts',(-0.786422660833742,0.333333333333333,
-3.66661143271648));
#48379=CARTESIAN_POINT('Ctrl Pts',(-0.786422660833742,-0.333333333333333,
-3.66661143271648));
#48380=CARTESIAN_POINT('Ctrl Pts',(-0.786422660833742,-0.666666666666667,
-3.66661143271648));
#48381=CARTESIAN_POINT('Ctrl Pts',(-0.786422660833742,-1.,-3.66661143271648));
#48382=CARTESIAN_POINT('Ctrl Pts',(-0.732042837400619,-1.,-4.13571194405636));
#48383=CARTESIAN_POINT('Ctrl Pts',(-0.732042837400619,1.,-4.13571194405636));
#48384=CARTESIAN_POINT('Ctrl Pts',(-0.732488575135926,-1.,-4.13420383737278));
#48385=CARTESIAN_POINT('Ctrl Pts',(-0.732488575135926,1.,-4.13420383737278));
#48386=CARTESIAN_POINT('Ctrl Pts',(-0.733376589325634,-1.,-4.13118752796397));
#48387=CARTESIAN_POINT('Ctrl Pts',(-0.733376589325634,1.,-4.13118752796397));
#48388=CARTESIAN_POINT('Ctrl Pts',(-0.734698226767512,-1.,-4.12666277572794));
#48389=CARTESIAN_POINT('Ctrl Pts',(-0.734698226767512,1.,-4.12666277572794));
#48390=CARTESIAN_POINT('Ctrl Pts',(-0.736439634335347,-1.,-4.12062919626082));
#48391=CARTESIAN_POINT('Ctrl Pts',(-0.736439634335347,1.,-4.12062919626082));
#48392=CARTESIAN_POINT('Ctrl Pts',(-0.738581708229119,-1.,-4.11308626953795));
#48393=CARTESIAN_POINT('Ctrl Pts',(-0.738581708229119,1.,-4.11308626953795));
#48394=CARTESIAN_POINT('Ctrl Pts',(-0.740688998555152,-1.,-4.1055424175856));
#48395=CARTESIAN_POINT('Ctrl Pts',(-0.740688998555152,1.,-4.1055424175856));
#48396=CARTESIAN_POINT('Ctrl Pts',(-0.742761369690018,-1.,-4.09799769702712));
#48397=CARTESIAN_POINT('Ctrl Pts',(-0.742761369690018,1.,-4.09799769702712));
#48398=CARTESIAN_POINT('Ctrl Pts',(-0.744798649705514,-1.,-4.09045220253011));
#48399=CARTESIAN_POINT('Ctrl Pts',(-0.744798649705514,1.,-4.09045220253011));
#48400=CARTESIAN_POINT('Ctrl Pts',(-0.746800631490822,-1.,-4.08290608094789));
#48401=CARTESIAN_POINT('Ctrl Pts',(-0.746800631490822,1.,-4.08290608094789));
#48402=CARTESIAN_POINT('Ctrl Pts',(-0.748767076679177,-1.,-4.07535951055363));
#48403=CARTESIAN_POINT('Ctrl Pts',(-0.748767076679177,1.,-4.07535951055363));
#48404=CARTESIAN_POINT('Ctrl Pts',(-0.750697720483176,-1.,-4.06781267241886));
#48405=CARTESIAN_POINT('Ctrl Pts',(-0.750697720483176,1.,-4.06781267241886));
#48406=CARTESIAN_POINT('Ctrl Pts',(-0.752592276482869,-1.,-4.06026572221399));
#48407=CARTESIAN_POINT('Ctrl Pts',(-0.752592276482869,1.,-4.06026572221399));
#48408=CARTESIAN_POINT('Ctrl Pts',(-0.754450441816412,-1.,-4.05271876688106));
#48409=CARTESIAN_POINT('Ctrl Pts',(-0.754450441816412,1.,-4.05271876688106));
#48410=CARTESIAN_POINT('Ctrl Pts',(-0.756271902370187,-1.,-4.04517182654344));
#48411=CARTESIAN_POINT('Ctrl Pts',(-0.756271902370187,1.,-4.04517182654344));
#48412=CARTESIAN_POINT('Ctrl Pts',(-0.758056338885554,-1.,-4.03762485803468));
#48413=CARTESIAN_POINT('Ctrl Pts',(-0.758056338885554,1.,-4.03762485803468));
#48414=CARTESIAN_POINT('Ctrl Pts',(-0.759803433244166,-1.,-4.0300778195465));
#48415=CARTESIAN_POINT('Ctrl Pts',(-0.759803433244166,1.,-4.0300778195465));
#48416=CARTESIAN_POINT('Ctrl Pts',(-0.761512875859942,-1.,-4.02253072741347));
#48417=CARTESIAN_POINT('Ctrl Pts',(-0.761512875859942,1.,-4.02253072741347));
#48418=CARTESIAN_POINT('Ctrl Pts',(-0.763184371182827,-1.,-4.01498370680434));
#48419=CARTESIAN_POINT('Ctrl Pts',(-0.763184371182827,1.,-4.01498370680434));
#48420=CARTESIAN_POINT('Ctrl Pts',(-0.764817648784946,-1.,-4.00743706791366));
#48421=CARTESIAN_POINT('Ctrl Pts',(-0.764817648784946,1.,-4.00743706791366));
#48422=CARTESIAN_POINT('Ctrl Pts',(-0.766412457135786,-1.,-3.99989129179464));
#48423=CARTESIAN_POINT('Ctrl Pts',(-0.766412457135786,1.,-3.99989129179464));
#48424=CARTESIAN_POINT('Ctrl Pts',(-0.767968531377708,-1.,-3.99234687880892));
#48425=CARTESIAN_POINT('Ctrl Pts',(-0.767968531377708,1.,-3.99234687880892));
#48426=CARTESIAN_POINT('Ctrl Pts',(-0.769485566245459,-1.,-3.98480422348403));
#48427=CARTESIAN_POINT('Ctrl Pts',(-0.769485566245459,1.,-3.98480422348403));
#48428=CARTESIAN_POINT('Ctrl Pts',(-0.770963190030504,-1.,-3.97726349165507));
#48429=CARTESIAN_POINT('Ctrl Pts',(-0.770963190030504,1.,-3.97726349165507));
#48430=CARTESIAN_POINT('Ctrl Pts',(-0.772400931772239,-1.,-3.96972446532832));
#48431=CARTESIAN_POINT('Ctrl Pts',(-0.772400931772239,1.,-3.96972446532832));
#48432=CARTESIAN_POINT('Ctrl Pts',(-0.773798212026683,-1.,-3.96218649639876));
#48433=CARTESIAN_POINT('Ctrl Pts',(-0.773798212026683,1.,-3.96218649639876));
#48434=CARTESIAN_POINT('Ctrl Pts',(-0.775154418039441,-1.,-3.95464885452364));
#48435=CARTESIAN_POINT('Ctrl Pts',(-0.775154418039441,1.,-3.95464885452364));
#48436=CARTESIAN_POINT('Ctrl Pts',(-0.77646896669796,-1.,-3.94711101619471));
#48437=CARTESIAN_POINT('Ctrl Pts',(-0.77646896669796,1.,-3.94711101619471));
#48438=CARTESIAN_POINT('Ctrl Pts',(-0.77774137056855,-1.,-3.93957296768098));
#48439=CARTESIAN_POINT('Ctrl Pts',(-0.77774137056855,1.,-3.93957296768098));
#48440=CARTESIAN_POINT('Ctrl Pts',(-0.778971308134786,-1.,-3.93203552473153));
#48441=CARTESIAN_POINT('Ctrl Pts',(-0.778971308134786,1.,-3.93203552473153));
#48442=CARTESIAN_POINT('Ctrl Pts',(-0.780158678615507,-1.,-3.92450058323799));
#48443=CARTESIAN_POINT('Ctrl Pts',(-0.780158678615507,1.,-3.92450058323799));
#48444=CARTESIAN_POINT('Ctrl Pts',(-0.781303428618344,-1.,-3.9169703605466));
#48445=CARTESIAN_POINT('Ctrl Pts',(-0.781303428618344,1.,-3.9169703605466));
#48446=CARTESIAN_POINT('Ctrl Pts',(-0.782405395622759,-1.,-3.90944671004536));
#48447=CARTESIAN_POINT('Ctrl Pts',(-0.782405395622759,1.,-3.90944671004536));
#48448=CARTESIAN_POINT('Ctrl Pts',(-0.783464141529082,-1.,-3.90193039043971));
#48449=CARTESIAN_POINT('Ctrl Pts',(-0.783464141529082,1.,-3.90193039043971));
#48450=CARTESIAN_POINT('Ctrl Pts',(-0.784478799358336,-1.,-3.89442039235105));
#48451=CARTESIAN_POINT('Ctrl Pts',(-0.784478799358336,1.,-3.89442039235105));
#48452=CARTESIAN_POINT('Ctrl Pts',(-0.785447890340723,-1.,-3.88691313167399));
#48453=CARTESIAN_POINT('Ctrl Pts',(-0.785447890340723,1.,-3.88691313167399));
#48454=CARTESIAN_POINT('Ctrl Pts',(-0.786369675812592,-1.,-3.87940402818186));
#48455=CARTESIAN_POINT('Ctrl Pts',(-0.786369675812592,1.,-3.87940402818186));
#48456=CARTESIAN_POINT('Ctrl Pts',(-0.78724252761798,-1.,-3.87188916600905));
#48457=CARTESIAN_POINT('Ctrl Pts',(-0.78724252761798,1.,-3.87188916600905));
#48458=CARTESIAN_POINT('Ctrl Pts',(-0.788065315093771,-1.,-3.86436702561342));
#48459=CARTESIAN_POINT('Ctrl Pts',(-0.788065315093771,1.,-3.86436702561342));
#48460=CARTESIAN_POINT('Ctrl Pts',(-0.788837734090688,-1.,-3.85683995872536));
#48461=CARTESIAN_POINT('Ctrl Pts',(-0.788837734090688,1.,-3.85683995872536));
#48462=CARTESIAN_POINT('Ctrl Pts',(-0.789560798155619,-1.,-3.8493163780891));
#48463=CARTESIAN_POINT('Ctrl Pts',(-0.789560798155619,1.,-3.8493163780891));
#48464=CARTESIAN_POINT('Ctrl Pts',(-0.790236124191289,-1.,-3.84180762342476));
#48465=CARTESIAN_POINT('Ctrl Pts',(-0.790236124191289,1.,-3.84180762342476));
#48466=CARTESIAN_POINT('Ctrl Pts',(-0.79086501270534,-1.,-3.83432392054804));
#48467=CARTESIAN_POINT('Ctrl Pts',(-0.79086501270534,1.,-3.83432392054804));
#48468=CARTESIAN_POINT('Ctrl Pts',(-0.791447528662381,-1.,-3.82687033899799));
#48469=CARTESIAN_POINT('Ctrl Pts',(-0.791447528662381,1.,-3.82687033899799));
#48470=CARTESIAN_POINT('Ctrl Pts',(-0.791981740718606,-1.,-3.81944345442237));
#48471=CARTESIAN_POINT('Ctrl Pts',(-0.791981740718606,1.,-3.81944345442237));
#48472=CARTESIAN_POINT('Ctrl Pts',(-0.792462483517568,-1.,-3.81202588694726));
#48473=CARTESIAN_POINT('Ctrl Pts',(-0.792462483517568,1.,-3.81202588694726));
#48474=CARTESIAN_POINT('Ctrl Pts',(-0.792882695234693,-1.,-3.80459229925598));
#48475=CARTESIAN_POINT('Ctrl Pts',(-0.792882695234693,1.,-3.80459229925598));
#48476=CARTESIAN_POINT('Ctrl Pts',(-0.7932356129732,-1.,-3.79711921389862));
#48477=CARTESIAN_POINT('Ctrl Pts',(-0.7932356129732,1.,-3.79711921389862));
#48478=CARTESIAN_POINT('Ctrl Pts',(-0.793516871680966,-1.,-3.78959439439222));
#48479=CARTESIAN_POINT('Ctrl Pts',(-0.793516871680966,1.,-3.78959439439222));
#48480=CARTESIAN_POINT('Ctrl Pts',(-0.793726235781339,-1.,-3.78202460377617));
#48481=CARTESIAN_POINT('Ctrl Pts',(-0.793726235781339,1.,-3.78202460377617));
#48482=CARTESIAN_POINT('Ctrl Pts',(-0.793870523787515,-1.,-3.77444863801264));
#48483=CARTESIAN_POINT('Ctrl Pts',(-0.793870523787515,1.,-3.77444863801264));
#48484=CARTESIAN_POINT('Ctrl Pts',(-0.793961083689141,-1.,-3.76692626931184));
#48485=CARTESIAN_POINT('Ctrl Pts',(-0.793961083689141,1.,-3.76692626931184));
#48486=CARTESIAN_POINT('Ctrl Pts',(-0.794008429135047,-1.,-3.75951468666325));
#48487=CARTESIAN_POINT('Ctrl Pts',(-0.794008429135047,1.,-3.75951468666325));
#48488=CARTESIAN_POINT('Ctrl Pts',(-0.794017347371441,-1.,-3.75224692493895));
#48489=CARTESIAN_POINT('Ctrl Pts',(-0.794017347371441,1.,-3.75224692493895));
#48490=CARTESIAN_POINT('Ctrl Pts',(-0.79398270045988,-1.,-3.74511357728827));
#48491=CARTESIAN_POINT('Ctrl Pts',(-0.79398270045988,1.,-3.74511357728827));
#48492=CARTESIAN_POINT('Ctrl Pts',(-0.79388270093679,-1.,-3.73803280541576));
#48493=CARTESIAN_POINT('Ctrl Pts',(-0.79388270093679,1.,-3.73803280541576));
#48494=CARTESIAN_POINT('Ctrl Pts',(-0.793682750269347,-1.,-3.7308691469564));
#48495=CARTESIAN_POINT('Ctrl Pts',(-0.793682750269347,1.,-3.7308691469564));
#48496=CARTESIAN_POINT('Ctrl Pts',(-0.79334702378387,-1.,-3.7234879729357));
#48497=CARTESIAN_POINT('Ctrl Pts',(-0.79334702378387,1.,-3.7234879729357));
#48498=CARTESIAN_POINT('Ctrl Pts',(-0.792848377370115,-1.,-3.7158024239604));
#48499=CARTESIAN_POINT('Ctrl Pts',(-0.792848377370115,1.,-3.7158024239604));
#48500=CARTESIAN_POINT('Ctrl Pts',(-0.792177688845968,-1.,-3.70781724021879));
#48501=CARTESIAN_POINT('Ctrl Pts',(-0.792177688845968,1.,-3.70781724021879));
#48502=CARTESIAN_POINT('Ctrl Pts',(-0.791356575696509,-1.,-3.69968940808982));
#48503=CARTESIAN_POINT('Ctrl Pts',(-0.791356575696509,1.,-3.69968940808982));
#48504=CARTESIAN_POINT('Ctrl Pts',(-0.79043628498958,-1.,-3.69172044327754));
#48505=CARTESIAN_POINT('Ctrl Pts',(-0.79043628498958,1.,-3.69172044327754));
#48506=CARTESIAN_POINT('Ctrl Pts',(-0.789483546065158,-1.,-3.68428439784285));
#48507=CARTESIAN_POINT('Ctrl Pts',(-0.789483546065158,1.,-3.68428439784285));
#48508=CARTESIAN_POINT('Ctrl Pts',(-0.788569566220662,-1.,-3.67777119516438));
#48509=CARTESIAN_POINT('Ctrl Pts',(-0.788569566220662,1.,-3.67777119516438));
#48510=CARTESIAN_POINT('Ctrl Pts',(-0.787758799995426,-1.,-3.672529236635));
#48511=CARTESIAN_POINT('Ctrl Pts',(-0.787758799995426,1.,-3.672529236635));
#48512=CARTESIAN_POINT('Ctrl Pts',(-0.787095252589508,-1.,-3.66879484800625));
#48513=CARTESIAN_POINT('Ctrl Pts',(-0.787095252589508,1.,-3.66879484800625));
#48514=CARTESIAN_POINT('Ctrl Pts',(-0.786698783541658,-1.,-3.66710211819938));
#48515=CARTESIAN_POINT('Ctrl Pts',(-0.786698783541658,1.,-3.66710211819938));
#48516=CARTESIAN_POINT('Ctrl Pts',(-0.786480236184947,-1.,-3.66657784454965));
#48517=CARTESIAN_POINT('Ctrl Pts',(-0.786480236184947,1.,-3.66657784454965));
#48518=CARTESIAN_POINT('Ctrl Pts',(-0.786369528183039,-1.,-3.66655932661846));
#48519=CARTESIAN_POINT('Ctrl Pts',(-0.786369528183039,1.,-3.66655932661846));
#48520=CARTESIAN_POINT('Ctrl Pts',(-0.786322922920599,-1.,-3.66663282329846));
#48521=CARTESIAN_POINT('Ctrl Pts',(-0.786322922920599,1.,-3.66663282329846));
#48522=CARTESIAN_POINT('',(-0.732042837400619,1.,-4.13571194405636));
#48523=CARTESIAN_POINT('Ctrl Pts',(-0.732042837400619,1.,-4.13571194405636));
#48524=CARTESIAN_POINT('Ctrl Pts',(-0.732488575135926,1.,-4.13420383737278));
#48525=CARTESIAN_POINT('Ctrl Pts',(-0.733376589325634,1.,-4.13118752796397));
#48526=CARTESIAN_POINT('Ctrl Pts',(-0.734698226767512,1.,-4.12666277572794));
#48527=CARTESIAN_POINT('Ctrl Pts',(-0.736439634335347,1.,-4.12062919626082));
#48528=CARTESIAN_POINT('Ctrl Pts',(-0.738581708229119,1.,-4.11308626953795));
#48529=CARTESIAN_POINT('Ctrl Pts',(-0.740688998555152,1.,-4.1055424175856));
#48530=CARTESIAN_POINT('Ctrl Pts',(-0.742761369690018,1.,-4.09799769702712));
#48531=CARTESIAN_POINT('Ctrl Pts',(-0.744798649705514,1.,-4.09045220253011));
#48532=CARTESIAN_POINT('Ctrl Pts',(-0.746800631490822,1.,-4.08290608094789));
#48533=CARTESIAN_POINT('Ctrl Pts',(-0.748767076679177,1.,-4.07535951055363));
#48534=CARTESIAN_POINT('Ctrl Pts',(-0.750697720483176,1.,-4.06781267241886));
#48535=CARTESIAN_POINT('Ctrl Pts',(-0.752592276482869,1.,-4.06026572221399));
#48536=CARTESIAN_POINT('Ctrl Pts',(-0.754450441816412,1.,-4.05271876688106));
#48537=CARTESIAN_POINT('Ctrl Pts',(-0.756271902370187,1.,-4.04517182654344));
#48538=CARTESIAN_POINT('Ctrl Pts',(-0.758056338885554,1.,-4.03762485803468));
#48539=CARTESIAN_POINT('Ctrl Pts',(-0.759803433244166,1.,-4.0300778195465));
#48540=CARTESIAN_POINT('Ctrl Pts',(-0.761512875859942,1.,-4.02253072741347));
#48541=CARTESIAN_POINT('Ctrl Pts',(-0.763184371182827,1.,-4.01498370680434));
#48542=CARTESIAN_POINT('Ctrl Pts',(-0.764817648784946,1.,-4.00743706791366));
#48543=CARTESIAN_POINT('Ctrl Pts',(-0.766412457135786,1.,-3.99989129179464));
#48544=CARTESIAN_POINT('Ctrl Pts',(-0.767968531377708,1.,-3.99234687880892));
#48545=CARTESIAN_POINT('Ctrl Pts',(-0.769485566245459,1.,-3.98480422348403));
#48546=CARTESIAN_POINT('Ctrl Pts',(-0.770963190030504,1.,-3.97726349165507));
#48547=CARTESIAN_POINT('Ctrl Pts',(-0.772400931772239,1.,-3.96972446532832));
#48548=CARTESIAN_POINT('Ctrl Pts',(-0.773798212026683,1.,-3.96218649639876));
#48549=CARTESIAN_POINT('Ctrl Pts',(-0.775154418039441,1.,-3.95464885452364));
#48550=CARTESIAN_POINT('Ctrl Pts',(-0.77646896669796,1.,-3.94711101619471));
#48551=CARTESIAN_POINT('Ctrl Pts',(-0.77774137056855,1.,-3.93957296768098));
#48552=CARTESIAN_POINT('Ctrl Pts',(-0.778971308134786,1.,-3.93203552473153));
#48553=CARTESIAN_POINT('Ctrl Pts',(-0.780158678615507,1.,-3.92450058323799));
#48554=CARTESIAN_POINT('Ctrl Pts',(-0.781303428618344,1.,-3.9169703605466));
#48555=CARTESIAN_POINT('Ctrl Pts',(-0.782405395622759,1.,-3.90944671004536));
#48556=CARTESIAN_POINT('Ctrl Pts',(-0.783464141529082,1.,-3.90193039043971));
#48557=CARTESIAN_POINT('Ctrl Pts',(-0.784478799358336,1.,-3.89442039235105));
#48558=CARTESIAN_POINT('Ctrl Pts',(-0.785447890340723,1.,-3.88691313167399));
#48559=CARTESIAN_POINT('Ctrl Pts',(-0.786369675812592,1.,-3.87940402818186));
#48560=CARTESIAN_POINT('Ctrl Pts',(-0.78724252761798,1.,-3.87188916600905));
#48561=CARTESIAN_POINT('Ctrl Pts',(-0.788065315093771,1.,-3.86436702561342));
#48562=CARTESIAN_POINT('Ctrl Pts',(-0.788837734090688,1.,-3.85683995872536));
#48563=CARTESIAN_POINT('Ctrl Pts',(-0.789560798155619,1.,-3.8493163780891));
#48564=CARTESIAN_POINT('Ctrl Pts',(-0.790236124191289,1.,-3.84180762342476));
#48565=CARTESIAN_POINT('Ctrl Pts',(-0.79086501270534,1.,-3.83432392054804));
#48566=CARTESIAN_POINT('Ctrl Pts',(-0.791447528662381,1.,-3.82687033899799));
#48567=CARTESIAN_POINT('Ctrl Pts',(-0.791981740718606,1.,-3.81944345442237));
#48568=CARTESIAN_POINT('Ctrl Pts',(-0.792462483517568,1.,-3.81202588694726));
#48569=CARTESIAN_POINT('Ctrl Pts',(-0.792882695234693,1.,-3.80459229925598));
#48570=CARTESIAN_POINT('Ctrl Pts',(-0.7932356129732,1.,-3.79711921389862));
#48571=CARTESIAN_POINT('Ctrl Pts',(-0.793516871680966,1.,-3.78959439439222));
#48572=CARTESIAN_POINT('Ctrl Pts',(-0.793726235781339,1.,-3.78202460377617));
#48573=CARTESIAN_POINT('Ctrl Pts',(-0.793870523787515,1.,-3.77444863801264));
#48574=CARTESIAN_POINT('Ctrl Pts',(-0.793961083689141,1.,-3.76692626931184));
#48575=CARTESIAN_POINT('Ctrl Pts',(-0.794008429135047,1.,-3.75951468666325));
#48576=CARTESIAN_POINT('Ctrl Pts',(-0.794017347371441,1.,-3.75224692493895));
#48577=CARTESIAN_POINT('Ctrl Pts',(-0.79398270045988,1.,-3.74511357728827));
#48578=CARTESIAN_POINT('Ctrl Pts',(-0.79388270093679,1.,-3.73803280541576));
#48579=CARTESIAN_POINT('Ctrl Pts',(-0.793682750269347,1.,-3.7308691469564));
#48580=CARTESIAN_POINT('Ctrl Pts',(-0.79334702378387,1.,-3.7234879729357));
#48581=CARTESIAN_POINT('Ctrl Pts',(-0.792848377370115,1.,-3.7158024239604));
#48582=CARTESIAN_POINT('Ctrl Pts',(-0.792177688845968,1.,-3.70781724021879));
#48583=CARTESIAN_POINT('Ctrl Pts',(-0.791356575696509,1.,-3.69968940808982));
#48584=CARTESIAN_POINT('Ctrl Pts',(-0.79043628498958,1.,-3.69172044327754));
#48585=CARTESIAN_POINT('Ctrl Pts',(-0.789483546065158,1.,-3.68428439784285));
#48586=CARTESIAN_POINT('Ctrl Pts',(-0.788569566220662,1.,-3.67777119516438));
#48587=CARTESIAN_POINT('Ctrl Pts',(-0.787758799995426,1.,-3.672529236635));
#48588=CARTESIAN_POINT('Ctrl Pts',(-0.787145041181589,1.,-3.66907505398769));
#48589=CARTESIAN_POINT('Ctrl Pts',(-0.7867743371985,1.,-3.66743103898844));
#48590=CARTESIAN_POINT('Ctrl Pts',(-0.78656591955989,1.,-3.66680946938396));
#48591=CARTESIAN_POINT('Ctrl Pts',(-0.786459983896781,1.,-3.66664310415236));
#48592=CARTESIAN_POINT('Ctrl Pts',(-0.786422660833743,1.,-3.66661143271648));
#48593=CARTESIAN_POINT('',(-0.732042837400619,0.,-4.13571194405636));
#48594=CARTESIAN_POINT('Ctrl Pts',(-0.385214314776329,-1.,-3.73016218570874));
#48595=CARTESIAN_POINT('Ctrl Pts',(-0.385214314776329,1.,-3.73016218570874));
#48596=CARTESIAN_POINT('Ctrl Pts',(-0.385147278814804,-1.,-3.73010668803185));
#48597=CARTESIAN_POINT('Ctrl Pts',(-0.385147278814804,1.,-3.73010668803185));
#48598=CARTESIAN_POINT('Ctrl Pts',(-0.385047711603887,-1.,-3.73015851028729));
#48599=CARTESIAN_POINT('Ctrl Pts',(-0.385047711603887,1.,-3.73015851028729));
#48600=CARTESIAN_POINT('Ctrl Pts',(-0.385001870183841,-1.,-3.73072465900727));
#48601=CARTESIAN_POINT('Ctrl Pts',(-0.385001870183841,1.,-3.73072465900727));
#48602=CARTESIAN_POINT('Ctrl Pts',(-0.385147887989515,-1.,-3.73245705639337));
#48603=CARTESIAN_POINT('Ctrl Pts',(-0.385147887989515,1.,-3.73245705639337));
#48604=CARTESIAN_POINT('Ctrl Pts',(-0.385670806454744,-1.,-3.73621371845475));
#48605=CARTESIAN_POINT('Ctrl Pts',(-0.385670806454744,1.,-3.73621371845475));
#48606=CARTESIAN_POINT('Ctrl Pts',(-0.386519576222035,-1.,-3.74144965781088));
#48607=CARTESIAN_POINT('Ctrl Pts',(-0.386519576222035,1.,-3.74144965781088));
#48608=CARTESIAN_POINT('Ctrl Pts',(-0.387663020050396,-1.,-3.74792651696269));
#48609=CARTESIAN_POINT('Ctrl Pts',(-0.387663020050396,1.,-3.74792651696269));
#48610=CARTESIAN_POINT('Ctrl Pts',(-0.389054775898251,-1.,-3.75529302894757));
#48611=CARTESIAN_POINT('Ctrl Pts',(-0.389054775898251,1.,-3.75529302894757));
#48612=CARTESIAN_POINT('Ctrl Pts',(-0.390642072979259,-1.,-3.76315635032993));
#48613=CARTESIAN_POINT('Ctrl Pts',(-0.390642072979259,1.,-3.76315635032993));
#48614=CARTESIAN_POINT('Ctrl Pts',(-0.392372786223347,-1.,-3.77114011595892));
#48615=CARTESIAN_POINT('Ctrl Pts',(-0.392372786223347,1.,-3.77114011595892));
#48616=CARTESIAN_POINT('Ctrl Pts',(-0.394202481011595,-1.,-3.77894173114368));
#48617=CARTESIAN_POINT('Ctrl Pts',(-0.394202481011595,1.,-3.77894173114368));
#48618=CARTESIAN_POINT('Ctrl Pts',(-0.396103205335029,-1.,-3.78640521279479));
#48619=CARTESIAN_POINT('Ctrl Pts',(-0.396103205335029,1.,-3.78640521279479));
#48620=CARTESIAN_POINT('Ctrl Pts',(-0.398064818684158,-1.,-3.79352887163457));
#48621=CARTESIAN_POINT('Ctrl Pts',(-0.398064818684158,1.,-3.79352887163457));
#48622=CARTESIAN_POINT('Ctrl Pts',(-0.400088346504727,-1.,-3.80040370384659));
#48623=CARTESIAN_POINT('Ctrl Pts',(-0.400088346504727,1.,-3.80040370384659));
#48624=CARTESIAN_POINT('Ctrl Pts',(-0.402181320148475,-1.,-3.80716881962763));
#48625=CARTESIAN_POINT('Ctrl Pts',(-0.402181320148475,1.,-3.80716881962763));
#48626=CARTESIAN_POINT('Ctrl Pts',(-0.404352694628236,-1.,-3.81396374287762));
#48627=CARTESIAN_POINT('Ctrl Pts',(-0.404352694628236,1.,-3.81396374287762));
#48628=CARTESIAN_POINT('Ctrl Pts',(-0.406607038258906,-1.,-3.82087303913741));
#48629=CARTESIAN_POINT('Ctrl Pts',(-0.406607038258906,1.,-3.82087303913741));
#48630=CARTESIAN_POINT('Ctrl Pts',(-0.408942371447377,-1.,-3.82790724256397));
#48631=CARTESIAN_POINT('Ctrl Pts',(-0.408942371447377,1.,-3.82790724256397));
#48632=CARTESIAN_POINT('Ctrl Pts',(-0.41135303879846,-1.,-3.83503345578645));
#48633=CARTESIAN_POINT('Ctrl Pts',(-0.41135303879846,1.,-3.83503345578645));
#48634=CARTESIAN_POINT('Ctrl Pts',(-0.413831367016727,-1.,-3.84219403994742));
#48635=CARTESIAN_POINT('Ctrl Pts',(-0.413831367016727,1.,-3.84219403994742));
#48636=CARTESIAN_POINT('Ctrl Pts',(-0.41636967805292,-1.,-3.8493286415751));
#48637=CARTESIAN_POINT('Ctrl Pts',(-0.41636967805292,1.,-3.8493286415751));
#48638=CARTESIAN_POINT('Ctrl Pts',(-0.41896246808681,-1.,-3.85639825648031));
#48639=CARTESIAN_POINT('Ctrl Pts',(-0.41896246808681,1.,-3.85639825648031));
#48640=CARTESIAN_POINT('Ctrl Pts',(-0.421607423177576,-1.,-3.86339652542749));
#48641=CARTESIAN_POINT('Ctrl Pts',(-0.421607423177576,1.,-3.86339652542749));
#48642=CARTESIAN_POINT('Ctrl Pts',(-0.424304173195142,-1.,-3.87033643487882));
#48643=CARTESIAN_POINT('Ctrl Pts',(-0.424304173195142,1.,-3.87033643487882));
#48644=CARTESIAN_POINT('Ctrl Pts',(-0.427053541173469,-1.,-3.87724240306609));
#48645=CARTESIAN_POINT('Ctrl Pts',(-0.427053541173469,1.,-3.87724240306609));
#48646=CARTESIAN_POINT('Ctrl Pts',(-0.429856640579734,-1.,-3.88414070943334));
#48647=CARTESIAN_POINT('Ctrl Pts',(-0.429856640579734,1.,-3.88414070943334));
#48648=CARTESIAN_POINT('Ctrl Pts',(-0.432713929544439,-1.,-3.89104947940592));
#48649=CARTESIAN_POINT('Ctrl Pts',(-0.432713929544439,1.,-3.89104947940592));
#48650=CARTESIAN_POINT('Ctrl Pts',(-0.435624629433506,-1.,-3.8979725665544));
#48651=CARTESIAN_POINT('Ctrl Pts',(-0.435624629433506,1.,-3.8979725665544));
#48652=CARTESIAN_POINT('Ctrl Pts',(-0.438587235458233,-1.,-3.90490512938546));
#48653=CARTESIAN_POINT('Ctrl Pts',(-0.438587235458233,1.,-3.90490512938546));
#48654=CARTESIAN_POINT('Ctrl Pts',(-0.441599824524047,-1.,-3.91183704069146));
#48655=CARTESIAN_POINT('Ctrl Pts',(-0.441599824524047,1.,-3.91183704069146));
#48656=CARTESIAN_POINT('Ctrl Pts',(-0.444660430230593,-1.,-3.91875701610721));
#48657=CARTESIAN_POINT('Ctrl Pts',(-0.444660430230593,1.,-3.91875701610721));
#48658=CARTESIAN_POINT('Ctrl Pts',(-0.447767416837297,-1.,-3.92565674143424));
#48659=CARTESIAN_POINT('Ctrl Pts',(-0.447767416837297,1.,-3.92565674143424));
#48660=CARTESIAN_POINT('Ctrl Pts',(-0.450919768356347,-1.,-3.93253407403128));
#48661=CARTESIAN_POINT('Ctrl Pts',(-0.450919768356347,1.,-3.93253407403128));
#48662=CARTESIAN_POINT('Ctrl Pts',(-0.454116879027576,-1.,-3.93939080846298));
#48663=CARTESIAN_POINT('Ctrl Pts',(-0.454116879027576,1.,-3.93939080846298));
#48664=CARTESIAN_POINT('Ctrl Pts',(-0.457358410451674,-1.,-3.94623117206675));
#48665=CARTESIAN_POINT('Ctrl Pts',(-0.457358410451674,1.,-3.94623117206675));
#48666=CARTESIAN_POINT('Ctrl Pts',(-0.460644124429119,-1.,-3.95306005817363));
#48667=CARTESIAN_POINT('Ctrl Pts',(-0.460644124429119,1.,-3.95306005817363));
#48668=CARTESIAN_POINT('Ctrl Pts',(-0.463973722115744,-1.,-3.95988133243543));
#48669=CARTESIAN_POINT('Ctrl Pts',(-0.463973722115744,1.,-3.95988133243543));
#48670=CARTESIAN_POINT('Ctrl Pts',(-0.467346690880672,-1.,-3.96669622273946));
#48671=CARTESIAN_POINT('Ctrl Pts',(-0.467346690880672,1.,-3.96669622273946));
#48672=CARTESIAN_POINT('Ctrl Pts',(-0.470762379613477,-1.,-3.97350414289415));
#48673=CARTESIAN_POINT('Ctrl Pts',(-0.470762379613477,1.,-3.97350414289415));
#48674=CARTESIAN_POINT('Ctrl Pts',(-0.474220061019542,-1.,-3.9803033804443));
#48675=CARTESIAN_POINT('Ctrl Pts',(-0.474220061019542,1.,-3.9803033804443));
#48676=CARTESIAN_POINT('Ctrl Pts',(-0.477718999122033,-1.,-3.98709184306743));
#48677=CARTESIAN_POINT('Ctrl Pts',(-0.477718999122033,1.,-3.98709184306743));
#48678=CARTESIAN_POINT('Ctrl Pts',(-0.481258512209638,-1.,-3.99386775880655));
#48679=CARTESIAN_POINT('Ctrl Pts',(-0.481258512209638,1.,-3.99386775880655));
#48680=CARTESIAN_POINT('Ctrl Pts',(-0.484838042421754,-1.,-4.00063045119234));
#48681=CARTESIAN_POINT('Ctrl Pts',(-0.484838042421754,1.,-4.00063045119234));
#48682=CARTESIAN_POINT('Ctrl Pts',(-0.488457130424531,-1.,-4.0073800839092));
#48683=CARTESIAN_POINT('Ctrl Pts',(-0.488457130424531,1.,-4.0073800839092));
#48684=CARTESIAN_POINT('Ctrl Pts',(-0.492115383417931,-1.,-4.01411733503486));
#48685=CARTESIAN_POINT('Ctrl Pts',(-0.492115383417931,1.,-4.01411733503486));
#48686=CARTESIAN_POINT('Ctrl Pts',(-0.495812444326223,-1.,-4.02084308851813));
#48687=CARTESIAN_POINT('Ctrl Pts',(-0.495812444326223,1.,-4.02084308851813));
#48688=CARTESIAN_POINT('Ctrl Pts',(-0.49954796234089,-1.,-4.0275581398015));
#48689=CARTESIAN_POINT('Ctrl Pts',(-0.49954796234089,1.,-4.0275581398015));
#48690=CARTESIAN_POINT('Ctrl Pts',(-0.503321556915514,-1.,-4.0342628417439));
#48691=CARTESIAN_POINT('Ctrl Pts',(-0.503321556915514,1.,-4.0342628417439));
#48692=CARTESIAN_POINT('Ctrl Pts',(-0.507132823288362,-1.,-4.04095715149074));
#48693=CARTESIAN_POINT('Ctrl Pts',(-0.507132823288362,1.,-4.04095715149074));
#48694=CARTESIAN_POINT('Ctrl Pts',(-0.510981349219174,-1.,-4.04764078815591));
#48695=CARTESIAN_POINT('Ctrl Pts',(-0.510981349219174,1.,-4.04764078815591));
#48696=CARTESIAN_POINT('Ctrl Pts',(-0.514866728193104,-1.,-4.05431335771261));
#48697=CARTESIAN_POINT('Ctrl Pts',(-0.514866728193104,1.,-4.05431335771261));
#48698=CARTESIAN_POINT('Ctrl Pts',(-0.51878857233681,-1.,-4.06097448037934));
#48699=CARTESIAN_POINT('Ctrl Pts',(-0.51878857233681,1.,-4.06097448037934));
#48700=CARTESIAN_POINT('Ctrl Pts',(-0.522746528602768,-1.,-4.06762394471075));
#48701=CARTESIAN_POINT('Ctrl Pts',(-0.522746528602768,1.,-4.06762394471075));
#48702=CARTESIAN_POINT('Ctrl Pts',(-0.526740277227,-1.,-4.07426172299496));
#48703=CARTESIAN_POINT('Ctrl Pts',(-0.526740277227,1.,-4.07426172299496));
#48704=CARTESIAN_POINT('Ctrl Pts',(-0.530769518728075,-1.,-4.08088789536488));
#48705=CARTESIAN_POINT('Ctrl Pts',(-0.530769518728075,1.,-4.08088789536488));
#48706=CARTESIAN_POINT('Ctrl Pts',(-0.534833963476999,-1.,-4.08750259988693));
#48707=CARTESIAN_POINT('Ctrl Pts',(-0.534833963476999,1.,-4.08750259988693));
#48708=CARTESIAN_POINT('Ctrl Pts',(-0.538933321179921,-1.,-4.09410597627116));
#48709=CARTESIAN_POINT('Ctrl Pts',(-0.538933321179921,1.,-4.09410597627116));
#48710=CARTESIAN_POINT('Ctrl Pts',(-0.543067286878457,-1.,-4.10069810244473));
#48711=CARTESIAN_POINT('Ctrl Pts',(-0.543067286878457,1.,-4.10069810244473));
#48712=CARTESIAN_POINT('Ctrl Pts',(-0.54723553948676,-1.,-4.1072789702877));
#48713=CARTESIAN_POINT('Ctrl Pts',(-0.54723553948676,1.,-4.1072789702877));
#48714=CARTESIAN_POINT('Ctrl Pts',(-0.551437758498247,-1.,-4.11384852025578));
#48715=CARTESIAN_POINT('Ctrl Pts',(-0.551437758498247,1.,-4.11384852025578));
#48716=CARTESIAN_POINT('Ctrl Pts',(-0.555673636130778,-1.,-4.1204066619623));
#48717=CARTESIAN_POINT('Ctrl Pts',(-0.555673636130778,1.,-4.1204066619623));
#48718=CARTESIAN_POINT('Ctrl Pts',(-0.559942890594628,-1.,-4.12695329951859));
#48719=CARTESIAN_POINT('Ctrl Pts',(-0.559942890594628,1.,-4.12695329951859));
#48720=CARTESIAN_POINT('Ctrl Pts',(-0.564245279535705,-1.,-4.13348835726086));
#48721=CARTESIAN_POINT('Ctrl Pts',(-0.564245279535705,1.,-4.13348835726086));
#48722=CARTESIAN_POINT('Ctrl Pts',(-0.568580610187116,-1.,-4.14001179828669));
#48723=CARTESIAN_POINT('Ctrl Pts',(-0.568580610187116,1.,-4.14001179828669));
#48724=CARTESIAN_POINT('Ctrl Pts',(-0.572948736066277,-1.,-4.14652361065787));
#48725=CARTESIAN_POINT('Ctrl Pts',(-0.572948736066277,1.,-4.14652361065787));
#48726=CARTESIAN_POINT('Ctrl Pts',(-0.576469391673917,-1.,-4.1517237611974));
#48727=CARTESIAN_POINT('Ctrl Pts',(-0.576469391673917,1.,-4.1517237611974));
#48728=CARTESIAN_POINT('Ctrl Pts',(-0.579124568912543,-1.,-4.15561864787379));
#48729=CARTESIAN_POINT('Ctrl Pts',(-0.579124568912543,1.,-4.15561864787379));
#48730=CARTESIAN_POINT('Ctrl Pts',(-0.580901211462913,-1.,-4.15821291712391));
#48731=CARTESIAN_POINT('Ctrl Pts',(-0.580901211462913,1.,-4.15821291712391));
#48732=CARTESIAN_POINT('Ctrl Pts',(-0.581791163835814,-1.,-4.15950947128175));
#48733=CARTESIAN_POINT('Ctrl Pts',(-0.581791163835814,1.,-4.15950947128175));
#48734=CARTESIAN_POINT('',(-0.385112848332548,1.,-3.73017266276632));
#48735=CARTESIAN_POINT('Ctrl Pts',(-0.385112848332549,-1.,-3.73017266276632));
#48736=CARTESIAN_POINT('Ctrl Pts',(-0.385112848332549,-0.666666666666667,
-3.73017266276632));
#48737=CARTESIAN_POINT('Ctrl Pts',(-0.385112848332549,-0.333333333333333,
-3.73017266276632));
#48738=CARTESIAN_POINT('Ctrl Pts',(-0.385112848332549,0.333333333333333,
-3.73017266276632));
#48739=CARTESIAN_POINT('Ctrl Pts',(-0.385112848332549,0.666666666666667,
-3.73017266276632));
#48740=CARTESIAN_POINT('Ctrl Pts',(-0.385112848332549,1.,-3.73017266276632));
#48741=CARTESIAN_POINT('',(-0.581791163835814,1.,-4.15950947128175));
#48742=CARTESIAN_POINT('',(-0.581791163835814,0.,-4.15950947128175));
#48743=CARTESIAN_POINT('Ctrl Pts',(-0.385112848332549,1.,-3.73017266276632));
#48744=CARTESIAN_POINT('Ctrl Pts',(-0.385087139001609,1.,-3.73021431755218));
#48745=CARTESIAN_POINT('Ctrl Pts',(-0.385037797882046,1.,-3.73040527620929));
#48746=CARTESIAN_POINT('Ctrl Pts',(-0.385031656499142,1.,-3.731060828624));
#48747=CARTESIAN_POINT('Ctrl Pts',(-0.385187124633965,1.,-3.73273893363318));
#48748=CARTESIAN_POINT('Ctrl Pts',(-0.385670806454744,1.,-3.73621371845475));
#48749=CARTESIAN_POINT('Ctrl Pts',(-0.386519576222035,1.,-3.74144965781088));
#48750=CARTESIAN_POINT('Ctrl Pts',(-0.387663020050396,1.,-3.74792651696269));
#48751=CARTESIAN_POINT('Ctrl Pts',(-0.389054775898251,1.,-3.75529302894757));
#48752=CARTESIAN_POINT('Ctrl Pts',(-0.390642072979259,1.,-3.76315635032993));
#48753=CARTESIAN_POINT('Ctrl Pts',(-0.392372786223347,1.,-3.77114011595892));
#48754=CARTESIAN_POINT('Ctrl Pts',(-0.394202481011595,1.,-3.77894173114368));
#48755=CARTESIAN_POINT('Ctrl Pts',(-0.396103205335029,1.,-3.78640521279479));
#48756=CARTESIAN_POINT('Ctrl Pts',(-0.398064818684158,1.,-3.79352887163457));
#48757=CARTESIAN_POINT('Ctrl Pts',(-0.400088346504727,1.,-3.80040370384659));
#48758=CARTESIAN_POINT('Ctrl Pts',(-0.402181320148475,1.,-3.80716881962763));
#48759=CARTESIAN_POINT('Ctrl Pts',(-0.404352694628236,1.,-3.81396374287762));
#48760=CARTESIAN_POINT('Ctrl Pts',(-0.406607038258906,1.,-3.82087303913741));
#48761=CARTESIAN_POINT('Ctrl Pts',(-0.408942371447377,1.,-3.82790724256397));
#48762=CARTESIAN_POINT('Ctrl Pts',(-0.41135303879846,1.,-3.83503345578645));
#48763=CARTESIAN_POINT('Ctrl Pts',(-0.413831367016727,1.,-3.84219403994742));
#48764=CARTESIAN_POINT('Ctrl Pts',(-0.41636967805292,1.,-3.8493286415751));
#48765=CARTESIAN_POINT('Ctrl Pts',(-0.41896246808681,1.,-3.85639825648031));
#48766=CARTESIAN_POINT('Ctrl Pts',(-0.421607423177576,1.,-3.86339652542749));
#48767=CARTESIAN_POINT('Ctrl Pts',(-0.424304173195142,1.,-3.87033643487882));
#48768=CARTESIAN_POINT('Ctrl Pts',(-0.427053541173469,1.,-3.87724240306609));
#48769=CARTESIAN_POINT('Ctrl Pts',(-0.429856640579734,1.,-3.88414070943334));
#48770=CARTESIAN_POINT('Ctrl Pts',(-0.432713929544439,1.,-3.89104947940592));
#48771=CARTESIAN_POINT('Ctrl Pts',(-0.435624629433506,1.,-3.8979725665544));
#48772=CARTESIAN_POINT('Ctrl Pts',(-0.438587235458233,1.,-3.90490512938546));
#48773=CARTESIAN_POINT('Ctrl Pts',(-0.441599824524047,1.,-3.91183704069146));
#48774=CARTESIAN_POINT('Ctrl Pts',(-0.444660430230593,1.,-3.91875701610721));
#48775=CARTESIAN_POINT('Ctrl Pts',(-0.447767416837297,1.,-3.92565674143424));
#48776=CARTESIAN_POINT('Ctrl Pts',(-0.450919768356347,1.,-3.93253407403128));
#48777=CARTESIAN_POINT('Ctrl Pts',(-0.454116879027576,1.,-3.93939080846298));
#48778=CARTESIAN_POINT('Ctrl Pts',(-0.457358410451674,1.,-3.94623117206675));
#48779=CARTESIAN_POINT('Ctrl Pts',(-0.460644124429119,1.,-3.95306005817363));
#48780=CARTESIAN_POINT('Ctrl Pts',(-0.463973722115744,1.,-3.95988133243543));
#48781=CARTESIAN_POINT('Ctrl Pts',(-0.467346690880672,1.,-3.96669622273946));
#48782=CARTESIAN_POINT('Ctrl Pts',(-0.470762379613477,1.,-3.97350414289415));
#48783=CARTESIAN_POINT('Ctrl Pts',(-0.474220061019542,1.,-3.9803033804443));
#48784=CARTESIAN_POINT('Ctrl Pts',(-0.477718999122033,1.,-3.98709184306743));
#48785=CARTESIAN_POINT('Ctrl Pts',(-0.481258512209638,1.,-3.99386775880655));
#48786=CARTESIAN_POINT('Ctrl Pts',(-0.484838042421754,1.,-4.00063045119234));
#48787=CARTESIAN_POINT('Ctrl Pts',(-0.488457130424531,1.,-4.0073800839092));
#48788=CARTESIAN_POINT('Ctrl Pts',(-0.492115383417931,1.,-4.01411733503486));
#48789=CARTESIAN_POINT('Ctrl Pts',(-0.495812444326223,1.,-4.02084308851813));
#48790=CARTESIAN_POINT('Ctrl Pts',(-0.49954796234089,1.,-4.0275581398015));
#48791=CARTESIAN_POINT('Ctrl Pts',(-0.503321556915514,1.,-4.0342628417439));
#48792=CARTESIAN_POINT('Ctrl Pts',(-0.507132823288362,1.,-4.04095715149074));
#48793=CARTESIAN_POINT('Ctrl Pts',(-0.510981349219174,1.,-4.04764078815591));
#48794=CARTESIAN_POINT('Ctrl Pts',(-0.514866728193104,1.,-4.05431335771261));
#48795=CARTESIAN_POINT('Ctrl Pts',(-0.51878857233681,1.,-4.06097448037934));
#48796=CARTESIAN_POINT('Ctrl Pts',(-0.522746528602768,1.,-4.06762394471075));
#48797=CARTESIAN_POINT('Ctrl Pts',(-0.526740277227,1.,-4.07426172299496));
#48798=CARTESIAN_POINT('Ctrl Pts',(-0.530769518728075,1.,-4.08088789536488));
#48799=CARTESIAN_POINT('Ctrl Pts',(-0.534833963476999,1.,-4.08750259988693));
#48800=CARTESIAN_POINT('Ctrl Pts',(-0.538933321179921,1.,-4.09410597627116));
#48801=CARTESIAN_POINT('Ctrl Pts',(-0.543067286878457,1.,-4.10069810244473));
#48802=CARTESIAN_POINT('Ctrl Pts',(-0.54723553948676,1.,-4.1072789702877));
#48803=CARTESIAN_POINT('Ctrl Pts',(-0.551437758498247,1.,-4.11384852025578));
#48804=CARTESIAN_POINT('Ctrl Pts',(-0.555673636130778,1.,-4.1204066619623));
#48805=CARTESIAN_POINT('Ctrl Pts',(-0.559942890594628,1.,-4.12695329951859));
#48806=CARTESIAN_POINT('Ctrl Pts',(-0.564245279535705,1.,-4.13348835726086));
#48807=CARTESIAN_POINT('Ctrl Pts',(-0.568580610187116,1.,-4.14001179828669));
#48808=CARTESIAN_POINT('Ctrl Pts',(-0.572948736066277,1.,-4.14652361065787));
#48809=CARTESIAN_POINT('Ctrl Pts',(-0.576469391673917,1.,-4.1517237611974));
#48810=CARTESIAN_POINT('Ctrl Pts',(-0.579124568912543,1.,-4.15561864787379));
#48811=CARTESIAN_POINT('Ctrl Pts',(-0.580901211462913,1.,-4.15821291712391));
#48812=CARTESIAN_POINT('Ctrl Pts',(-0.581791163835814,1.,-4.15950947128175));
#48813=CARTESIAN_POINT('Origin',(-0.581791163835814,0.,-4.15950947128175));
#48814=CARTESIAN_POINT('',(-0.732042837400619,1.,-4.13571194405636));
#48815=CARTESIAN_POINT('Origin',(0.,0.,0.));
#48816=CARTESIAN_POINT('',(-0.203156094897896,1.,-3.74449296982994));
#48817=CARTESIAN_POINT('Origin',(0.,1.,0.));
#48818=CARTESIAN_POINT('Ctrl Pts',(-0.203156094897896,1.,-3.74449296982994));
#48819=CARTESIAN_POINT('Ctrl Pts',(-0.203156094897896,0.666666666666667,
-3.74449296982994));
#48820=CARTESIAN_POINT('Ctrl Pts',(-0.203156094897896,0.333333333333333,
-3.74449296982994));
#48821=CARTESIAN_POINT('Ctrl Pts',(-0.203156094897896,-0.333333333333333,
-3.74449296982994));
#48822=CARTESIAN_POINT('Ctrl Pts',(-0.203156094897896,-0.666666666666667,
-3.74449296982994));
#48823=CARTESIAN_POINT('Ctrl Pts',(-0.203156094897896,-1.,-3.74449296982994));
#48824=CARTESIAN_POINT('Ctrl Pts',(-0.0760622897878238,-1.,-4.19931119685982));
#48825=CARTESIAN_POINT('Ctrl Pts',(-0.0760622897878238,1.,-4.19931119685982));
#48826=CARTESIAN_POINT('Ctrl Pts',(-0.0767384596142197,-1.,-4.19789138621624));
#48827=CARTESIAN_POINT('Ctrl Pts',(-0.0767384596142197,1.,-4.19789138621624));
#48828=CARTESIAN_POINT('Ctrl Pts',(-0.0780873956244405,-1.,-4.19505112860624));
#48829=CARTESIAN_POINT('Ctrl Pts',(-0.0780873956244405,1.,-4.19505112860624));
#48830=CARTESIAN_POINT('Ctrl Pts',(-0.0801005887117605,-1.,-4.19078883322483));
#48831=CARTESIAN_POINT('Ctrl Pts',(-0.0801005887117605,1.,-4.19078883322483));
#48832=CARTESIAN_POINT('Ctrl Pts',(-0.0827644164389512,-1.,-4.1851019532944));
#48833=CARTESIAN_POINT('Ctrl Pts',(-0.0827644164389512,1.,-4.1851019532944));
#48834=CARTESIAN_POINT('Ctrl Pts',(-0.0860600915552517,-1.,-4.17798698669991));
#48835=CARTESIAN_POINT('Ctrl Pts',(-0.0860600915552517,1.,-4.17798698669991));
#48836=CARTESIAN_POINT('Ctrl Pts',(-0.089321556085033,-1.,-4.17086566491823));
#48837=CARTESIAN_POINT('Ctrl Pts',(-0.089321556085033,1.,-4.17086566491823));
#48838=CARTESIAN_POINT('Ctrl Pts',(-0.0925486672167692,-1.,-4.16373802265942));
#48839=CARTESIAN_POINT('Ctrl Pts',(-0.0925486672167692,1.,-4.16373802265942));
#48840=CARTESIAN_POINT('Ctrl Pts',(-0.095741240329707,-1.,-4.15660412653006));
#48841=CARTESIAN_POINT('Ctrl Pts',(-0.095741240329707,1.,-4.15660412653006));
#48842=CARTESIAN_POINT('Ctrl Pts',(-0.0988990478899814,-1.,-4.1494640891762));
#48843=CARTESIAN_POINT('Ctrl Pts',(-0.0988990478899814,1.,-4.1494640891762));
#48844=CARTESIAN_POINT('Ctrl Pts',(-0.102021826577454,-1.,-4.14231804938737));
#48845=CARTESIAN_POINT('Ctrl Pts',(-0.102021826577454,1.,-4.14231804938737));
#48846=CARTESIAN_POINT('Ctrl Pts',(-0.105109286538864,-1.,-4.13516614458396));
#48847=CARTESIAN_POINT('Ctrl Pts',(-0.105109286538864,1.,-4.13516614458396));
#48848=CARTESIAN_POINT('Ctrl Pts',(-0.10816112052835,-1.,-4.12800848371386));
#48849=CARTESIAN_POINT('Ctrl Pts',(-0.10816112052835,1.,-4.12800848371386));
#48850=CARTESIAN_POINT('Ctrl Pts',(-0.111177012683377,-1.,-4.12084512502444));
#48851=CARTESIAN_POINT('Ctrl Pts',(-0.111177012683377,1.,-4.12084512502444));
#48852=CARTESIAN_POINT('Ctrl Pts',(-0.114156649609602,-1.,-4.11367603925313));
#48853=CARTESIAN_POINT('Ctrl Pts',(-0.114156649609602,1.,-4.11367603925313));
#48854=CARTESIAN_POINT('Ctrl Pts',(-0.117099722731705,-1.,-4.10650113382187));
#48855=CARTESIAN_POINT('Ctrl Pts',(-0.117099722731705,1.,-4.10650113382187));
#48856=CARTESIAN_POINT('Ctrl Pts',(-0.120005924388162,-1.,-4.09932031767243));
#48857=CARTESIAN_POINT('Ctrl Pts',(-0.120005924388162,1.,-4.09932031767243));
#48858=CARTESIAN_POINT('Ctrl Pts',(-0.122874946249119,-1.,-4.09213355850836));
#48859=CARTESIAN_POINT('Ctrl Pts',(-0.122874946249119,1.,-4.09213355850836));
#48860=CARTESIAN_POINT('Ctrl Pts',(-0.125706476822529,-1.,-4.08494093372315));
#48861=CARTESIAN_POINT('Ctrl Pts',(-0.125706476822529,1.,-4.08494093372315));
#48862=CARTESIAN_POINT('Ctrl Pts',(-0.128500200484814,-1.,-4.07774270738809));
#48863=CARTESIAN_POINT('Ctrl Pts',(-0.128500200484814,1.,-4.07774270738809));
#48864=CARTESIAN_POINT('Ctrl Pts',(-0.131255793548914,-1.,-4.07053931528579));
#48865=CARTESIAN_POINT('Ctrl Pts',(-0.131255793548914,1.,-4.07053931528579));
#48866=CARTESIAN_POINT('Ctrl Pts',(-0.133972916144225,-1.,-4.06333121018476));
#48867=CARTESIAN_POINT('Ctrl Pts',(-0.133972916144225,1.,-4.06333121018476));
#48868=CARTESIAN_POINT('Ctrl Pts',(-0.136651205046111,-1.,-4.05611873400122));
#48869=CARTESIAN_POINT('Ctrl Pts',(-0.136651205046111,1.,-4.05611873400122));
#48870=CARTESIAN_POINT('Ctrl Pts',(-0.13929026718006,-1.,-4.04890199238056));
#48871=CARTESIAN_POINT('Ctrl Pts',(-0.13929026718006,1.,-4.04890199238056));
#48872=CARTESIAN_POINT('Ctrl Pts',(-0.141889671485508,-1.,-4.04168069633842));
#48873=CARTESIAN_POINT('Ctrl Pts',(-0.141889671485508,1.,-4.04168069633842));
#48874=CARTESIAN_POINT('Ctrl Pts',(-0.144448947038352,-1.,-4.03445411510403));
#48875=CARTESIAN_POINT('Ctrl Pts',(-0.144448947038352,1.,-4.03445411510403));
#48876=CARTESIAN_POINT('Ctrl Pts',(-0.146967602878999,-1.,-4.02722143147048));
#48877=CARTESIAN_POINT('Ctrl Pts',(-0.146967602878999,1.,-4.02722143147048));
#48878=CARTESIAN_POINT('Ctrl Pts',(-0.149445144968708,-1.,-4.01998203715588));
#48879=CARTESIAN_POINT('Ctrl Pts',(-0.149445144968708,1.,-4.01998203715588));
#48880=CARTESIAN_POINT('Ctrl Pts',(-0.151881094022909,-1.,-4.01273584234684));
#48881=CARTESIAN_POINT('Ctrl Pts',(-0.151881094022909,1.,-4.01273584234684));
#48882=CARTESIAN_POINT('Ctrl Pts',(-0.15427500487231,-1.,-4.00548360245297));
#48883=CARTESIAN_POINT('Ctrl Pts',(-0.15427500487231,1.,-4.00548360245297));
#48884=CARTESIAN_POINT('Ctrl Pts',(-0.156626481393736,-1.,-3.99822717425869));
#48885=CARTESIAN_POINT('Ctrl Pts',(-0.156626481393736,1.,-3.99822717425869));
#48886=CARTESIAN_POINT('Ctrl Pts',(-0.158935123982796,-1.,-3.99096873945862));
#48887=CARTESIAN_POINT('Ctrl Pts',(-0.158935123982796,1.,-3.99096873945862));
#48888=CARTESIAN_POINT('Ctrl Pts',(-0.161200482186088,-1.,-3.98371010319866));
#48889=CARTESIAN_POINT('Ctrl Pts',(-0.161200482186088,1.,-3.98371010319866));
#48890=CARTESIAN_POINT('Ctrl Pts',(-0.163422004609999,-1.,-3.97645194630944));
#48891=CARTESIAN_POINT('Ctrl Pts',(-0.163422004609999,1.,-3.97645194630944));
#48892=CARTESIAN_POINT('Ctrl Pts',(-0.165598992851098,-1.,-3.9691931362141));
#48893=CARTESIAN_POINT('Ctrl Pts',(-0.165598992851098,1.,-3.9691931362141));
#48894=CARTESIAN_POINT('Ctrl Pts',(-0.167730547023312,-1.,-3.96192990160296));
#48895=CARTESIAN_POINT('Ctrl Pts',(-0.167730547023312,1.,-3.96192990160296));
#48896=CARTESIAN_POINT('Ctrl Pts',(-0.16981566637413,-1.,-3.95465744665263));
#48897=CARTESIAN_POINT('Ctrl Pts',(-0.16981566637413,1.,-3.95465744665263));
#48898=CARTESIAN_POINT('Ctrl Pts',(-0.171853355369233,-1.,-3.94737164900861));
#48899=CARTESIAN_POINT('Ctrl Pts',(-0.171853355369233,1.,-3.94737164900861));
#48900=CARTESIAN_POINT('Ctrl Pts',(-0.173842734974607,-1.,-3.94007083096214));
#48901=CARTESIAN_POINT('Ctrl Pts',(-0.173842734974607,1.,-3.94007083096214));
#48902=CARTESIAN_POINT('Ctrl Pts',(-0.175783136893873,-1.,-3.93275726771049));
#48903=CARTESIAN_POINT('Ctrl Pts',(-0.175783136893873,1.,-3.93275726771049));
#48904=CARTESIAN_POINT('Ctrl Pts',(-0.177674246152328,-1.,-3.92543942697672));
#48905=CARTESIAN_POINT('Ctrl Pts',(-0.177674246152328,1.,-3.92543942697672));
#48906=CARTESIAN_POINT('Ctrl Pts',(-0.179515885822895,-1.,-3.91812876180948));
#48907=CARTESIAN_POINT('Ctrl Pts',(-0.179515885822895,1.,-3.91812876180948));
#48908=CARTESIAN_POINT('Ctrl Pts',(-0.181307740731796,-1.,-3.91083557557193));
#48909=CARTESIAN_POINT('Ctrl Pts',(-0.181307740731796,1.,-3.91083557557193));
#48910=CARTESIAN_POINT('Ctrl Pts',(-0.183049081993193,-1.,-3.90356488555138));
#48911=CARTESIAN_POINT('Ctrl Pts',(-0.183049081993193,1.,-3.90356488555138));
#48912=CARTESIAN_POINT('Ctrl Pts',(-0.184738537728035,-1.,-3.89631300742633));
#48913=CARTESIAN_POINT('Ctrl Pts',(-0.184738537728035,1.,-3.89631300742633));
#48914=CARTESIAN_POINT('Ctrl Pts',(-0.186373724985263,-1.,-3.88906196725817));
#48915=CARTESIAN_POINT('Ctrl Pts',(-0.186373724985263,1.,-3.88906196725817));
#48916=CARTESIAN_POINT('Ctrl Pts',(-0.187951632512663,-1.,-3.88178563496187));
#48917=CARTESIAN_POINT('Ctrl Pts',(-0.187951632512663,1.,-3.88178563496187));
#48918=CARTESIAN_POINT('Ctrl Pts',(-0.189469253358254,-1.,-3.87445976418377));
#48919=CARTESIAN_POINT('Ctrl Pts',(-0.189469253358254,1.,-3.87445976418377));
#48920=CARTESIAN_POINT('Ctrl Pts',(-0.190924190418613,-1.,-3.8670715862477));
#48921=CARTESIAN_POINT('Ctrl Pts',(-0.190924190418613,1.,-3.8670715862477));
#48922=CARTESIAN_POINT('Ctrl Pts',(-0.19231515304498,-1.,-3.85962774407652));
#48923=CARTESIAN_POINT('Ctrl Pts',(-0.19231515304498,1.,-3.85962774407652));
#48924=CARTESIAN_POINT('Ctrl Pts',(-0.193642806777748,-1.,-3.85216762264019));
#48925=CARTESIAN_POINT('Ctrl Pts',(-0.193642806777748,1.,-3.85216762264019));
#48926=CARTESIAN_POINT('Ctrl Pts',(-0.194909009460255,-1.,-3.84475203347052));
#48927=CARTESIAN_POINT('Ctrl Pts',(-0.194909009460255,1.,-3.84475203347052));
#48928=CARTESIAN_POINT('Ctrl Pts',(-0.19611519897189,-1.,-3.83743910616265));
#48929=CARTESIAN_POINT('Ctrl Pts',(-0.19611519897189,1.,-3.83743910616265));
#48930=CARTESIAN_POINT('Ctrl Pts',(-0.197260935827375,-1.,-3.83026221776488));
#48931=CARTESIAN_POINT('Ctrl Pts',(-0.197260935827375,1.,-3.83026221776488));
#48932=CARTESIAN_POINT('Ctrl Pts',(-0.19834261690047,-1.,-3.82321127348981));
#48933=CARTESIAN_POINT('Ctrl Pts',(-0.19834261690047,1.,-3.82321127348981));
#48934=CARTESIAN_POINT('Ctrl Pts',(-0.199351525297396,-1.,-3.81620203429702));
#48935=CARTESIAN_POINT('Ctrl Pts',(-0.199351525297396,1.,-3.81620203429702));
#48936=CARTESIAN_POINT('Ctrl Pts',(-0.20027467943329,-1.,-3.80909529318501));
#48937=CARTESIAN_POINT('Ctrl Pts',(-0.20027467943329,1.,-3.80909529318501));
#48938=CARTESIAN_POINT('Ctrl Pts',(-0.201097756307252,-1.,-3.80175247447171));
#48939=CARTESIAN_POINT('Ctrl Pts',(-0.201097756307252,1.,-3.80175247447171));
#48940=CARTESIAN_POINT('Ctrl Pts',(-0.201807533800799,-1.,-3.79408354187274));
#48941=CARTESIAN_POINT('Ctrl Pts',(-0.201807533800799,1.,-3.79408354187274));
#48942=CARTESIAN_POINT('Ctrl Pts',(-0.202394260512193,-1.,-3.78609175019317));
#48943=CARTESIAN_POINT('Ctrl Pts',(-0.202394260512193,1.,-3.78609175019317));
#48944=CARTESIAN_POINT('Ctrl Pts',(-0.202854729699197,-1.,-3.77793553476879));
#48945=CARTESIAN_POINT('Ctrl Pts',(-0.202854729699197,1.,-3.77793553476879));
#48946=CARTESIAN_POINT('Ctrl Pts',(-0.203192390045337,-1.,-3.76992071595267));
#48947=CARTESIAN_POINT('Ctrl Pts',(-0.203192390045337,1.,-3.76992071595267));
#48948=CARTESIAN_POINT('Ctrl Pts',(-0.203414634707646,-1.,-3.76242717937273));
#48949=CARTESIAN_POINT('Ctrl Pts',(-0.203414634707646,1.,-3.76242717937273));
#48950=CARTESIAN_POINT('Ctrl Pts',(-0.203530796848404,-1.,-3.75585118707924));
#48951=CARTESIAN_POINT('Ctrl Pts',(-0.203530796848404,1.,-3.75585118707924));
#48952=CARTESIAN_POINT('Ctrl Pts',(-0.203550035479097,-1.,-3.75054693397716));
#48953=CARTESIAN_POINT('Ctrl Pts',(-0.203550035479097,1.,-3.75054693397716));
#48954=CARTESIAN_POINT('Ctrl Pts',(-0.20347884453023,-1.,-3.74675472018582));
#48955=CARTESIAN_POINT('Ctrl Pts',(-0.20347884453023,1.,-3.74675472018582));
#48956=CARTESIAN_POINT('Ctrl Pts',(-0.203352057956055,-1.,-3.7450208092684));
#48957=CARTESIAN_POINT('Ctrl Pts',(-0.203352057956055,1.,-3.7450208092684));
#48958=CARTESIAN_POINT('Ctrl Pts',(-0.203218215747895,-1.,-3.74446880195845));
#48959=CARTESIAN_POINT('Ctrl Pts',(-0.203218215747895,1.,-3.74446880195845));
#48960=CARTESIAN_POINT('Ctrl Pts',(-0.20311176758786,-1.,-3.74443319346666));
#48961=CARTESIAN_POINT('Ctrl Pts',(-0.20311176758786,1.,-3.74443319346666));
#48962=CARTESIAN_POINT('Ctrl Pts',(-0.203054238699719,-1.,-3.74449849461127));
#48963=CARTESIAN_POINT('Ctrl Pts',(-0.203054238699719,1.,-3.74449849461127));
#48964=CARTESIAN_POINT('',(-0.0760622897878238,1.,-4.19931119685982));
#48965=CARTESIAN_POINT('Ctrl Pts',(-0.0760622897878238,1.,-4.19931119685982));
#48966=CARTESIAN_POINT('Ctrl Pts',(-0.0767384596142197,1.,-4.19789138621624));
#48967=CARTESIAN_POINT('Ctrl Pts',(-0.0780873956244405,1.,-4.19505112860624));
#48968=CARTESIAN_POINT('Ctrl Pts',(-0.0801005887117605,1.,-4.19078883322483));
#48969=CARTESIAN_POINT('Ctrl Pts',(-0.0827644164389512,1.,-4.1851019532944));
#48970=CARTESIAN_POINT('Ctrl Pts',(-0.0860600915552517,1.,-4.17798698669991));
#48971=CARTESIAN_POINT('Ctrl Pts',(-0.089321556085033,1.,-4.17086566491823));
#48972=CARTESIAN_POINT('Ctrl Pts',(-0.0925486672167692,1.,-4.16373802265942));
#48973=CARTESIAN_POINT('Ctrl Pts',(-0.095741240329707,1.,-4.15660412653006));
#48974=CARTESIAN_POINT('Ctrl Pts',(-0.0988990478899814,1.,-4.1494640891762));
#48975=CARTESIAN_POINT('Ctrl Pts',(-0.102021826577454,1.,-4.14231804938737));
#48976=CARTESIAN_POINT('Ctrl Pts',(-0.105109286538864,1.,-4.13516614458396));
#48977=CARTESIAN_POINT('Ctrl Pts',(-0.10816112052835,1.,-4.12800848371386));
#48978=CARTESIAN_POINT('Ctrl Pts',(-0.111177012683377,1.,-4.12084512502444));
#48979=CARTESIAN_POINT('Ctrl Pts',(-0.114156649609602,1.,-4.11367603925313));
#48980=CARTESIAN_POINT('Ctrl Pts',(-0.117099722731705,1.,-4.10650113382187));
#48981=CARTESIAN_POINT('Ctrl Pts',(-0.120005924388162,1.,-4.09932031767243));
#48982=CARTESIAN_POINT('Ctrl Pts',(-0.122874946249119,1.,-4.09213355850836));
#48983=CARTESIAN_POINT('Ctrl Pts',(-0.125706476822529,1.,-4.08494093372315));
#48984=CARTESIAN_POINT('Ctrl Pts',(-0.128500200484814,1.,-4.07774270738809));
#48985=CARTESIAN_POINT('Ctrl Pts',(-0.131255793548914,1.,-4.07053931528579));
#48986=CARTESIAN_POINT('Ctrl Pts',(-0.133972916144225,1.,-4.06333121018476));
#48987=CARTESIAN_POINT('Ctrl Pts',(-0.136651205046111,1.,-4.05611873400122));
#48988=CARTESIAN_POINT('Ctrl Pts',(-0.13929026718006,1.,-4.04890199238056));
#48989=CARTESIAN_POINT('Ctrl Pts',(-0.141889671485508,1.,-4.04168069633842));
#48990=CARTESIAN_POINT('Ctrl Pts',(-0.144448947038352,1.,-4.03445411510403));
#48991=CARTESIAN_POINT('Ctrl Pts',(-0.146967602878999,1.,-4.02722143147048));
#48992=CARTESIAN_POINT('Ctrl Pts',(-0.149445144968708,1.,-4.01998203715588));
#48993=CARTESIAN_POINT('Ctrl Pts',(-0.151881094022909,1.,-4.01273584234684));
#48994=CARTESIAN_POINT('Ctrl Pts',(-0.15427500487231,1.,-4.00548360245297));
#48995=CARTESIAN_POINT('Ctrl Pts',(-0.156626481393736,1.,-3.99822717425869));
#48996=CARTESIAN_POINT('Ctrl Pts',(-0.158935123982796,1.,-3.99096873945862));
#48997=CARTESIAN_POINT('Ctrl Pts',(-0.161200482186088,1.,-3.98371010319866));
#48998=CARTESIAN_POINT('Ctrl Pts',(-0.163422004609999,1.,-3.97645194630944));
#48999=CARTESIAN_POINT('Ctrl Pts',(-0.165598992851098,1.,-3.9691931362141));
#49000=CARTESIAN_POINT('Ctrl Pts',(-0.167730547023312,1.,-3.96192990160296));
#49001=CARTESIAN_POINT('Ctrl Pts',(-0.16981566637413,1.,-3.95465744665263));
#49002=CARTESIAN_POINT('Ctrl Pts',(-0.171853355369233,1.,-3.94737164900861));
#49003=CARTESIAN_POINT('Ctrl Pts',(-0.173842734974607,1.,-3.94007083096214));
#49004=CARTESIAN_POINT('Ctrl Pts',(-0.175783136893873,1.,-3.93275726771049));
#49005=CARTESIAN_POINT('Ctrl Pts',(-0.177674246152328,1.,-3.92543942697672));
#49006=CARTESIAN_POINT('Ctrl Pts',(-0.179515885822895,1.,-3.91812876180948));
#49007=CARTESIAN_POINT('Ctrl Pts',(-0.181307740731796,1.,-3.91083557557193));
#49008=CARTESIAN_POINT('Ctrl Pts',(-0.183049081993193,1.,-3.90356488555138));
#49009=CARTESIAN_POINT('Ctrl Pts',(-0.184738537728035,1.,-3.89631300742633));
#49010=CARTESIAN_POINT('Ctrl Pts',(-0.186373724985263,1.,-3.88906196725817));
#49011=CARTESIAN_POINT('Ctrl Pts',(-0.187951632512663,1.,-3.88178563496187));
#49012=CARTESIAN_POINT('Ctrl Pts',(-0.189469253358254,1.,-3.87445976418377));
#49013=CARTESIAN_POINT('Ctrl Pts',(-0.190924190418613,1.,-3.8670715862477));
#49014=CARTESIAN_POINT('Ctrl Pts',(-0.19231515304498,1.,-3.85962774407652));
#49015=CARTESIAN_POINT('Ctrl Pts',(-0.193642806777748,1.,-3.85216762264019));
#49016=CARTESIAN_POINT('Ctrl Pts',(-0.194909009460255,1.,-3.84475203347052));
#49017=CARTESIAN_POINT('Ctrl Pts',(-0.19611519897189,1.,-3.83743910616265));
#49018=CARTESIAN_POINT('Ctrl Pts',(-0.197260935827375,1.,-3.83026221776488));
#49019=CARTESIAN_POINT('Ctrl Pts',(-0.19834261690047,1.,-3.82321127348981));
#49020=CARTESIAN_POINT('Ctrl Pts',(-0.199351525297396,1.,-3.81620203429702));
#49021=CARTESIAN_POINT('Ctrl Pts',(-0.20027467943329,1.,-3.80909529318501));
#49022=CARTESIAN_POINT('Ctrl Pts',(-0.201097756307252,1.,-3.80175247447171));
#49023=CARTESIAN_POINT('Ctrl Pts',(-0.201807533800799,1.,-3.79408354187274));
#49024=CARTESIAN_POINT('Ctrl Pts',(-0.202394260512193,1.,-3.78609175019317));
#49025=CARTESIAN_POINT('Ctrl Pts',(-0.202854729699197,1.,-3.77793553476879));
#49026=CARTESIAN_POINT('Ctrl Pts',(-0.203192390045337,1.,-3.76992071595267));
#49027=CARTESIAN_POINT('Ctrl Pts',(-0.203414634707646,1.,-3.76242717937273));
#49028=CARTESIAN_POINT('Ctrl Pts',(-0.203530796848404,1.,-3.75585118707924));
#49029=CARTESIAN_POINT('Ctrl Pts',(-0.203550035479097,1.,-3.75054693397716));
#49030=CARTESIAN_POINT('Ctrl Pts',(-0.203484186269315,1.,-3.74703926501843));
#49031=CARTESIAN_POINT('Ctrl Pts',(-0.203375226874331,1.,-3.74535749969262));
#49032=CARTESIAN_POINT('Ctrl Pts',(-0.203266610111264,1.,-3.74471097893961));
#49033=CARTESIAN_POINT('Ctrl Pts',(-0.203188003947965,1.,-3.74453008995129));
#49034=CARTESIAN_POINT('Ctrl Pts',(-0.203156094897896,1.,-3.74449296982994));
#49035=CARTESIAN_POINT('',(-0.0760622897878238,0.,-4.19931119685982));
#49036=CARTESIAN_POINT('Ctrl Pts',(0.20305423869972,-1.,-3.74449849461127));
#49037=CARTESIAN_POINT('Ctrl Pts',(0.20305423869972,1.,-3.74449849461127));
#49038=CARTESIAN_POINT('Ctrl Pts',(0.203111767587923,-1.,-3.7444331934681));
#49039=CARTESIAN_POINT('Ctrl Pts',(0.203111767587923,1.,-3.7444331934681));
#49040=CARTESIAN_POINT('Ctrl Pts',(0.203218215748058,-1.,-3.7444688019622));
#49041=CARTESIAN_POINT('Ctrl Pts',(0.203218215748058,1.,-3.7444688019622));
#49042=CARTESIAN_POINT('Ctrl Pts',(0.203352057956297,-1.,-3.74502080927395));
#49043=CARTESIAN_POINT('Ctrl Pts',(0.203352057956297,1.,-3.74502080927395));
#49044=CARTESIAN_POINT('Ctrl Pts',(0.203478844530447,-1.,-3.7467547201908));
#49045=CARTESIAN_POINT('Ctrl Pts',(0.203478844530447,1.,-3.7467547201908));
#49046=CARTESIAN_POINT('Ctrl Pts',(0.203550035479166,-1.,-3.75054693397875));
#49047=CARTESIAN_POINT('Ctrl Pts',(0.203550035479166,1.,-3.75054693397875));
#49048=CARTESIAN_POINT('Ctrl Pts',(0.203530796848321,-1.,-3.75585118707734));
#49049=CARTESIAN_POINT('Ctrl Pts',(0.203530796848321,1.,-3.75585118707734));
#49050=CARTESIAN_POINT('Ctrl Pts',(0.203414634707478,-1.,-3.76242717936885));
#49051=CARTESIAN_POINT('Ctrl Pts',(0.203414634707478,1.,-3.76242717936885));
#49052=CARTESIAN_POINT('Ctrl Pts',(0.203192390045164,-1.,-3.7699207159487));
#49053=CARTESIAN_POINT('Ctrl Pts',(0.203192390045164,1.,-3.7699207159487));
#49054=CARTESIAN_POINT('Ctrl Pts',(0.202854729699081,-1.,-3.77793553476614));
#49055=CARTESIAN_POINT('Ctrl Pts',(0.202854729699081,1.,-3.77793553476614));
#49056=CARTESIAN_POINT('Ctrl Pts',(0.20239426051216,-1.,-3.78609175019242));
#49057=CARTESIAN_POINT('Ctrl Pts',(0.20239426051216,1.,-3.78609175019242));
#49058=CARTESIAN_POINT('Ctrl Pts',(0.201807533800837,-1.,-3.7940835418736));
#49059=CARTESIAN_POINT('Ctrl Pts',(0.201807533800837,1.,-3.7940835418736));
#49060=CARTESIAN_POINT('Ctrl Pts',(0.201097756307326,-1.,-3.80175247447337));
#49061=CARTESIAN_POINT('Ctrl Pts',(0.201097756307326,1.,-3.80175247447337));
#49062=CARTESIAN_POINT('Ctrl Pts',(0.200274679433364,-1.,-3.80909529318669));
#49063=CARTESIAN_POINT('Ctrl Pts',(0.200274679433364,1.,-3.80909529318669));
#49064=CARTESIAN_POINT('Ctrl Pts',(0.199351525297447,-1.,-3.81620203429815));
#49065=CARTESIAN_POINT('Ctrl Pts',(0.199351525297447,1.,-3.81620203429815));
#49066=CARTESIAN_POINT('Ctrl Pts',(0.198342616900486,-1.,-3.82321127349016));
#49067=CARTESIAN_POINT('Ctrl Pts',(0.198342616900486,1.,-3.82321127349016));
#49068=CARTESIAN_POINT('Ctrl Pts',(0.197260935827361,-1.,-3.83026221776456));
#49069=CARTESIAN_POINT('Ctrl Pts',(0.197260935827361,1.,-3.83026221776456));
#49070=CARTESIAN_POINT('Ctrl Pts',(0.196115198971859,-1.,-3.83743910616195));
#49071=CARTESIAN_POINT('Ctrl Pts',(0.196115198971859,1.,-3.83743910616195));
#49072=CARTESIAN_POINT('Ctrl Pts',(0.19490900946022,-1.,-3.84475203346977));
#49073=CARTESIAN_POINT('Ctrl Pts',(0.19490900946022,1.,-3.84475203346977));
#49074=CARTESIAN_POINT('Ctrl Pts',(0.193642806777723,-1.,-3.85216762263966));
#49075=CARTESIAN_POINT('Ctrl Pts',(0.193642806777723,1.,-3.85216762263966));
#49076=CARTESIAN_POINT('Ctrl Pts',(0.19231515304497,-1.,-3.85962774407633));
#49077=CARTESIAN_POINT('Ctrl Pts',(0.19231515304497,1.,-3.85962774407633));
#49078=CARTESIAN_POINT('Ctrl Pts',(0.19092419041862,-1.,-3.86707158624783));
#49079=CARTESIAN_POINT('Ctrl Pts',(0.19092419041862,1.,-3.86707158624783));
#49080=CARTESIAN_POINT('Ctrl Pts',(0.189469253358272,-1.,-3.87445976418412));
#49081=CARTESIAN_POINT('Ctrl Pts',(0.189469253358272,1.,-3.87445976418412));
#49082=CARTESIAN_POINT('Ctrl Pts',(0.187951632512685,-1.,-3.88178563496228));
#49083=CARTESIAN_POINT('Ctrl Pts',(0.187951632512685,1.,-3.88178563496228));
#49084=CARTESIAN_POINT('Ctrl Pts',(0.18637372498528,-1.,-3.88906196725848));
#49085=CARTESIAN_POINT('Ctrl Pts',(0.18637372498528,1.,-3.88906196725848));
#49086=CARTESIAN_POINT('Ctrl Pts',(0.184738537728043,-1.,-3.89631300742646));
#49087=CARTESIAN_POINT('Ctrl Pts',(0.184738537728043,1.,-3.89631300742646));
#49088=CARTESIAN_POINT('Ctrl Pts',(0.18304908199319,-1.,-3.90356488555132));
#49089=CARTESIAN_POINT('Ctrl Pts',(0.18304908199319,1.,-3.90356488555132));
#49090=CARTESIAN_POINT('Ctrl Pts',(0.181307740731785,-1.,-3.91083557557175));
#49091=CARTESIAN_POINT('Ctrl Pts',(0.181307740731785,1.,-3.91083557557175));
#49092=CARTESIAN_POINT('Ctrl Pts',(0.179515885822881,-1.,-3.91812876180926));
#49093=CARTESIAN_POINT('Ctrl Pts',(0.179515885822881,1.,-3.91812876180926));
#49094=CARTESIAN_POINT('Ctrl Pts',(0.177674246152317,-1.,-3.92543942697655));
#49095=CARTESIAN_POINT('Ctrl Pts',(0.177674246152317,1.,-3.92543942697655));
#49096=CARTESIAN_POINT('Ctrl Pts',(0.175783136893868,-1.,-3.93275726771042));
#49097=CARTESIAN_POINT('Ctrl Pts',(0.175783136893868,1.,-3.93275726771042));
#49098=CARTESIAN_POINT('Ctrl Pts',(0.173842734974609,-1.,-3.94007083096217));
#49099=CARTESIAN_POINT('Ctrl Pts',(0.173842734974609,1.,-3.94007083096217));
#49100=CARTESIAN_POINT('Ctrl Pts',(0.17185335536924,-1.,-3.94737164900868));
#49101=CARTESIAN_POINT('Ctrl Pts',(0.17185335536924,1.,-3.94737164900868));
#49102=CARTESIAN_POINT('Ctrl Pts',(0.169815666374139,-1.,-3.95465744665268));
#49103=CARTESIAN_POINT('Ctrl Pts',(0.169815666374139,1.,-3.95465744665268));
#49104=CARTESIAN_POINT('Ctrl Pts',(0.167730547023319,-1.,-3.96192990160296));
#49105=CARTESIAN_POINT('Ctrl Pts',(0.167730547023319,1.,-3.96192990160296));
#49106=CARTESIAN_POINT('Ctrl Pts',(0.165598992851102,-1.,-3.96919313621407));
#49107=CARTESIAN_POINT('Ctrl Pts',(0.165598992851102,1.,-3.96919313621407));
#49108=CARTESIAN_POINT('Ctrl Pts',(0.163422004609999,-1.,-3.97645194630943));
#49109=CARTESIAN_POINT('Ctrl Pts',(0.163422004609999,1.,-3.97645194630943));
#49110=CARTESIAN_POINT('Ctrl Pts',(0.161200482186084,-1.,-3.98371010319872));
#49111=CARTESIAN_POINT('Ctrl Pts',(0.161200482186084,1.,-3.98371010319872));
#49112=CARTESIAN_POINT('Ctrl Pts',(0.158935123982793,-1.,-3.99096873945878));
#49113=CARTESIAN_POINT('Ctrl Pts',(0.158935123982793,1.,-3.99096873945878));
#49114=CARTESIAN_POINT('Ctrl Pts',(0.156626481393734,-1.,-3.99822717425893));
#49115=CARTESIAN_POINT('Ctrl Pts',(0.156626481393734,1.,-3.99822717425893));
#49116=CARTESIAN_POINT('Ctrl Pts',(0.15427500487231,-1.,-4.00548360245319));
#49117=CARTESIAN_POINT('Ctrl Pts',(0.15427500487231,1.,-4.00548360245319));
#49118=CARTESIAN_POINT('Ctrl Pts',(0.15188109402291,-1.,-4.01273584234689));
#49119=CARTESIAN_POINT('Ctrl Pts',(0.15188109402291,1.,-4.01273584234689));
#49120=CARTESIAN_POINT('Ctrl Pts',(0.149445144968707,-1.,-4.01998203715564));
#49121=CARTESIAN_POINT('Ctrl Pts',(0.149445144968707,1.,-4.01998203715564));
#49122=CARTESIAN_POINT('Ctrl Pts',(0.146967602878994,-1.,-4.02722143146994));
#49123=CARTESIAN_POINT('Ctrl Pts',(0.146967602878994,1.,-4.02722143146994));
#49124=CARTESIAN_POINT('Ctrl Pts',(0.144448947038344,-1.,-4.03445411510333));
#49125=CARTESIAN_POINT('Ctrl Pts',(0.144448947038344,1.,-4.03445411510333));
#49126=CARTESIAN_POINT('Ctrl Pts',(0.1418896714855,-1.,-4.04168069633781));
#49127=CARTESIAN_POINT('Ctrl Pts',(0.1418896714855,1.,-4.04168069633781));
#49128=CARTESIAN_POINT('Ctrl Pts',(0.139290267180057,-1.,-4.04890199238036));
#49129=CARTESIAN_POINT('Ctrl Pts',(0.139290267180057,1.,-4.04890199238036));
#49130=CARTESIAN_POINT('Ctrl Pts',(0.136651205046119,-1.,-4.05611873400172));
#49131=CARTESIAN_POINT('Ctrl Pts',(0.136651205046119,1.,-4.05611873400172));
#49132=CARTESIAN_POINT('Ctrl Pts',(0.133972916144245,-1.,-4.06333121018596));
#49133=CARTESIAN_POINT('Ctrl Pts',(0.133972916144245,1.,-4.06333121018596));
#49134=CARTESIAN_POINT('Ctrl Pts',(0.13125579354894,-1.,-4.0705393152874));
#49135=CARTESIAN_POINT('Ctrl Pts',(0.13125579354894,1.,-4.0705393152874));
#49136=CARTESIAN_POINT('Ctrl Pts',(0.128500200484837,-1.,-4.07774270738954));
#49137=CARTESIAN_POINT('Ctrl Pts',(0.128500200484837,1.,-4.07774270738954));
#49138=CARTESIAN_POINT('Ctrl Pts',(0.12570647682254,-1.,-4.08494093372377));
#49139=CARTESIAN_POINT('Ctrl Pts',(0.12570647682254,1.,-4.08494093372377));
#49140=CARTESIAN_POINT('Ctrl Pts',(0.122874946249107,-1.,-4.09213355850756));
#49141=CARTESIAN_POINT('Ctrl Pts',(0.122874946249107,1.,-4.09213355850756));
#49142=CARTESIAN_POINT('Ctrl Pts',(0.120005924388124,-1.,-4.09932031767002));
#49143=CARTESIAN_POINT('Ctrl Pts',(0.120005924388124,1.,-4.09932031767002));
#49144=CARTESIAN_POINT('Ctrl Pts',(0.117099722731648,-1.,-4.10650113381833));
#49145=CARTESIAN_POINT('Ctrl Pts',(0.117099722731648,1.,-4.10650113381833));
#49146=CARTESIAN_POINT('Ctrl Pts',(0.114156649609545,-1.,-4.11367603924961));
#49147=CARTESIAN_POINT('Ctrl Pts',(0.114156649609545,1.,-4.11367603924961));
#49148=CARTESIAN_POINT('Ctrl Pts',(0.111177012683346,-1.,-4.1208451250225));
#49149=CARTESIAN_POINT('Ctrl Pts',(0.111177012683346,1.,-4.1208451250225));
#49150=CARTESIAN_POINT('Ctrl Pts',(0.108161120528369,-1.,-4.12800848371504));
#49151=CARTESIAN_POINT('Ctrl Pts',(0.108161120528369,1.,-4.12800848371504));
#49152=CARTESIAN_POINT('Ctrl Pts',(0.105109286538945,-1.,-4.13516614458895));
#49153=CARTESIAN_POINT('Ctrl Pts',(0.105109286538945,1.,-4.13516614458895));
#49154=CARTESIAN_POINT('Ctrl Pts',(0.102021826577584,-1.,-4.14231804939538));
#49155=CARTESIAN_POINT('Ctrl Pts',(0.102021826577584,1.,-4.14231804939538));
#49156=CARTESIAN_POINT('Ctrl Pts',(0.0988990478901223,-1.,-4.14946408918485));
#49157=CARTESIAN_POINT('Ctrl Pts',(0.0988990478901223,1.,-4.14946408918485));
#49158=CARTESIAN_POINT('Ctrl Pts',(0.0957412403298004,-1.,-4.15660412653577));
#49159=CARTESIAN_POINT('Ctrl Pts',(0.0957412403298004,1.,-4.15660412653577));
#49160=CARTESIAN_POINT('Ctrl Pts',(0.0925486672167528,-1.,-4.16373802265839));
#49161=CARTESIAN_POINT('Ctrl Pts',(0.0925486672167528,1.,-4.16373802265839));
#49162=CARTESIAN_POINT('Ctrl Pts',(0.0893215560848647,-1.,-4.17086566490794));
#49163=CARTESIAN_POINT('Ctrl Pts',(0.0893215560848647,1.,-4.17086566490794));
#49164=CARTESIAN_POINT('Ctrl Pts',(0.0860600915549394,-1.,-4.17798698668094));
#49165=CARTESIAN_POINT('Ctrl Pts',(0.0860600915549394,1.,-4.17798698668094));
#49166=CARTESIAN_POINT('Ctrl Pts',(0.0827644164385676,-1.,-4.18510195327123));
#49167=CARTESIAN_POINT('Ctrl Pts',(0.0827644164385676,1.,-4.18510195327123));
#49168=CARTESIAN_POINT('Ctrl Pts',(0.0801005887114317,-1.,-4.19078883320504));
#49169=CARTESIAN_POINT('Ctrl Pts',(0.0801005887114317,1.,-4.19078883320504));
#49170=CARTESIAN_POINT('Ctrl Pts',(0.0780873956242395,-1.,-4.19505112859416));
#49171=CARTESIAN_POINT('Ctrl Pts',(0.0780873956242395,1.,-4.19505112859416));
#49172=CARTESIAN_POINT('Ctrl Pts',(0.0767384596141462,-1.,-4.1978913862118));
#49173=CARTESIAN_POINT('Ctrl Pts',(0.0767384596141462,1.,-4.1978913862118));
#49174=CARTESIAN_POINT('Ctrl Pts',(0.0760622897878244,-1.,-4.19931119685982));
#49175=CARTESIAN_POINT('Ctrl Pts',(0.0760622897878244,1.,-4.19931119685982));
#49176=CARTESIAN_POINT('',(0.203156094896102,1.,-3.74449296983004));
#49177=CARTESIAN_POINT('Ctrl Pts',(0.2031560948961,-1.,-3.74449296983004));
#49178=CARTESIAN_POINT('Ctrl Pts',(0.2031560948961,-0.666666666666667,-3.74449296983004));
#49179=CARTESIAN_POINT('Ctrl Pts',(0.2031560948961,-0.333333333333333,-3.74449296983004));
#49180=CARTESIAN_POINT('Ctrl Pts',(0.2031560948961,0.333333333333333,-3.74449296983004));
#49181=CARTESIAN_POINT('Ctrl Pts',(0.203156094896101,0.666666666666667,
-3.74449296983004));
#49182=CARTESIAN_POINT('Ctrl Pts',(0.203156094896101,1.,-3.74449296983004));
#49183=CARTESIAN_POINT('',(0.0760622897878244,1.,-4.19931119685982));
#49184=CARTESIAN_POINT('',(0.0760622897878244,0.,-4.19931119685982));
#49185=CARTESIAN_POINT('Ctrl Pts',(0.203156094896101,1.,-3.74449296983004));
#49186=CARTESIAN_POINT('Ctrl Pts',(0.203188003946657,1.,-3.74453008995093));
#49187=CARTESIAN_POINT('Ctrl Pts',(0.203266610110531,1.,-3.74471097893845));
#49188=CARTESIAN_POINT('Ctrl Pts',(0.203375226874121,1.,-3.74535749969115));
#49189=CARTESIAN_POINT('Ctrl Pts',(0.203484186269415,1.,-3.74703926501752));
#49190=CARTESIAN_POINT('Ctrl Pts',(0.203550035479166,1.,-3.75054693397875));
#49191=CARTESIAN_POINT('Ctrl Pts',(0.203530796848321,1.,-3.75585118707734));
#49192=CARTESIAN_POINT('Ctrl Pts',(0.203414634707478,1.,-3.76242717936885));
#49193=CARTESIAN_POINT('Ctrl Pts',(0.203192390045164,1.,-3.7699207159487));
#49194=CARTESIAN_POINT('Ctrl Pts',(0.202854729699081,1.,-3.77793553476614));
#49195=CARTESIAN_POINT('Ctrl Pts',(0.20239426051216,1.,-3.78609175019242));
#49196=CARTESIAN_POINT('Ctrl Pts',(0.201807533800837,1.,-3.7940835418736));
#49197=CARTESIAN_POINT('Ctrl Pts',(0.201097756307326,1.,-3.80175247447337));
#49198=CARTESIAN_POINT('Ctrl Pts',(0.200274679433364,1.,-3.80909529318669));
#49199=CARTESIAN_POINT('Ctrl Pts',(0.199351525297447,1.,-3.81620203429815));
#49200=CARTESIAN_POINT('Ctrl Pts',(0.198342616900486,1.,-3.82321127349016));
#49201=CARTESIAN_POINT('Ctrl Pts',(0.197260935827361,1.,-3.83026221776456));
#49202=CARTESIAN_POINT('Ctrl Pts',(0.196115198971859,1.,-3.83743910616195));
#49203=CARTESIAN_POINT('Ctrl Pts',(0.19490900946022,1.,-3.84475203346977));
#49204=CARTESIAN_POINT('Ctrl Pts',(0.193642806777723,1.,-3.85216762263966));
#49205=CARTESIAN_POINT('Ctrl Pts',(0.19231515304497,1.,-3.85962774407633));
#49206=CARTESIAN_POINT('Ctrl Pts',(0.19092419041862,1.,-3.86707158624783));
#49207=CARTESIAN_POINT('Ctrl Pts',(0.189469253358272,1.,-3.87445976418412));
#49208=CARTESIAN_POINT('Ctrl Pts',(0.187951632512685,1.,-3.88178563496228));
#49209=CARTESIAN_POINT('Ctrl Pts',(0.18637372498528,1.,-3.88906196725848));
#49210=CARTESIAN_POINT('Ctrl Pts',(0.184738537728043,1.,-3.89631300742646));
#49211=CARTESIAN_POINT('Ctrl Pts',(0.18304908199319,1.,-3.90356488555132));
#49212=CARTESIAN_POINT('Ctrl Pts',(0.181307740731785,1.,-3.91083557557175));
#49213=CARTESIAN_POINT('Ctrl Pts',(0.179515885822881,1.,-3.91812876180926));
#49214=CARTESIAN_POINT('Ctrl Pts',(0.177674246152317,1.,-3.92543942697655));
#49215=CARTESIAN_POINT('Ctrl Pts',(0.175783136893868,1.,-3.93275726771042));
#49216=CARTESIAN_POINT('Ctrl Pts',(0.173842734974609,1.,-3.94007083096217));
#49217=CARTESIAN_POINT('Ctrl Pts',(0.17185335536924,1.,-3.94737164900868));
#49218=CARTESIAN_POINT('Ctrl Pts',(0.169815666374139,1.,-3.95465744665268));
#49219=CARTESIAN_POINT('Ctrl Pts',(0.167730547023319,1.,-3.96192990160296));
#49220=CARTESIAN_POINT('Ctrl Pts',(0.165598992851102,1.,-3.96919313621407));
#49221=CARTESIAN_POINT('Ctrl Pts',(0.163422004609999,1.,-3.97645194630943));
#49222=CARTESIAN_POINT('Ctrl Pts',(0.161200482186084,1.,-3.98371010319872));
#49223=CARTESIAN_POINT('Ctrl Pts',(0.158935123982793,1.,-3.99096873945878));
#49224=CARTESIAN_POINT('Ctrl Pts',(0.156626481393734,1.,-3.99822717425893));
#49225=CARTESIAN_POINT('Ctrl Pts',(0.15427500487231,1.,-4.00548360245319));
#49226=CARTESIAN_POINT('Ctrl Pts',(0.15188109402291,1.,-4.01273584234689));
#49227=CARTESIAN_POINT('Ctrl Pts',(0.149445144968707,1.,-4.01998203715564));
#49228=CARTESIAN_POINT('Ctrl Pts',(0.146967602878994,1.,-4.02722143146994));
#49229=CARTESIAN_POINT('Ctrl Pts',(0.144448947038344,1.,-4.03445411510333));
#49230=CARTESIAN_POINT('Ctrl Pts',(0.1418896714855,1.,-4.04168069633781));
#49231=CARTESIAN_POINT('Ctrl Pts',(0.139290267180057,1.,-4.04890199238036));
#49232=CARTESIAN_POINT('Ctrl Pts',(0.136651205046119,1.,-4.05611873400172));
#49233=CARTESIAN_POINT('Ctrl Pts',(0.133972916144245,1.,-4.06333121018596));
#49234=CARTESIAN_POINT('Ctrl Pts',(0.13125579354894,1.,-4.0705393152874));
#49235=CARTESIAN_POINT('Ctrl Pts',(0.128500200484837,1.,-4.07774270738954));
#49236=CARTESIAN_POINT('Ctrl Pts',(0.12570647682254,1.,-4.08494093372377));
#49237=CARTESIAN_POINT('Ctrl Pts',(0.122874946249107,1.,-4.09213355850756));
#49238=CARTESIAN_POINT('Ctrl Pts',(0.120005924388124,1.,-4.09932031767002));
#49239=CARTESIAN_POINT('Ctrl Pts',(0.117099722731648,1.,-4.10650113381833));
#49240=CARTESIAN_POINT('Ctrl Pts',(0.114156649609545,1.,-4.11367603924961));
#49241=CARTESIAN_POINT('Ctrl Pts',(0.111177012683346,1.,-4.1208451250225));
#49242=CARTESIAN_POINT('Ctrl Pts',(0.108161120528369,1.,-4.12800848371504));
#49243=CARTESIAN_POINT('Ctrl Pts',(0.105109286538945,1.,-4.13516614458895));
#49244=CARTESIAN_POINT('Ctrl Pts',(0.102021826577584,1.,-4.14231804939538));
#49245=CARTESIAN_POINT('Ctrl Pts',(0.0988990478901223,1.,-4.14946408918485));
#49246=CARTESIAN_POINT('Ctrl Pts',(0.0957412403298004,1.,-4.15660412653577));
#49247=CARTESIAN_POINT('Ctrl Pts',(0.0925486672167528,1.,-4.16373802265839));
#49248=CARTESIAN_POINT('Ctrl Pts',(0.0893215560848647,1.,-4.17086566490794));
#49249=CARTESIAN_POINT('Ctrl Pts',(0.0860600915549394,1.,-4.17798698668094));
#49250=CARTESIAN_POINT('Ctrl Pts',(0.0827644164385676,1.,-4.18510195327123));
#49251=CARTESIAN_POINT('Ctrl Pts',(0.0801005887114317,1.,-4.19078883320504));
#49252=CARTESIAN_POINT('Ctrl Pts',(0.0780873956242395,1.,-4.19505112859416));
#49253=CARTESIAN_POINT('Ctrl Pts',(0.0767384596141462,1.,-4.1978913862118));
#49254=CARTESIAN_POINT('Ctrl Pts',(0.0760622897878244,1.,-4.19931119685982));
#49255=CARTESIAN_POINT('Origin',(0.0760622897878244,0.,-4.19931119685982));
#49256=CARTESIAN_POINT('',(-0.0760622897878238,1.,-4.19931119685982));
#49257=CARTESIAN_POINT('Origin',(0.,0.,0.));
#49258=CARTESIAN_POINT('',(0.385112848330761,1.,-3.73017266276651));
#49259=CARTESIAN_POINT('Origin',(0.,1.,0.));
#49260=CARTESIAN_POINT('Ctrl Pts',(0.385112848330762,1.,-3.73017266276651));
#49261=CARTESIAN_POINT('Ctrl Pts',(0.385112848330762,0.666666666666667,
-3.73017266276651));
#49262=CARTESIAN_POINT('Ctrl Pts',(0.385112848330762,0.333333333333333,
-3.73017266276651));
#49263=CARTESIAN_POINT('Ctrl Pts',(0.385112848330762,-0.333333333333333,
-3.73017266276651));
#49264=CARTESIAN_POINT('Ctrl Pts',(0.385112848330762,-0.666666666666667,
-3.73017266276651));
#49265=CARTESIAN_POINT('Ctrl Pts',(0.385112848330762,-1.,-3.73017266276651));
#49266=CARTESIAN_POINT('Ctrl Pts',(0.581791163835815,-1.,-4.15950947128175));
#49267=CARTESIAN_POINT('Ctrl Pts',(0.581791163835815,1.,-4.15950947128175));
#49268=CARTESIAN_POINT('Ctrl Pts',(0.580901211463535,-1.,-4.1582129171283));
#49269=CARTESIAN_POINT('Ctrl Pts',(0.580901211463535,1.,-4.1582129171283));
#49270=CARTESIAN_POINT('Ctrl Pts',(0.579124568914235,-1.,-4.15561864788576));
#49271=CARTESIAN_POINT('Ctrl Pts',(0.579124568914235,1.,-4.15561864788576));
#49272=CARTESIAN_POINT('Ctrl Pts',(0.576469391676688,-1.,-4.151723761217));
#49273=CARTESIAN_POINT('Ctrl Pts',(0.576469391676688,1.,-4.151723761217));
#49274=CARTESIAN_POINT('Ctrl Pts',(0.572948736069522,-1.,-4.14652361068081));
#49275=CARTESIAN_POINT('Ctrl Pts',(0.572948736069522,1.,-4.14652361068081));
#49276=CARTESIAN_POINT('Ctrl Pts',(0.568580610189774,-1.,-4.14001179830547));
#49277=CARTESIAN_POINT('Ctrl Pts',(0.568580610189774,1.,-4.14001179830547));
#49278=CARTESIAN_POINT('Ctrl Pts',(0.564245279537148,-1.,-4.13348835727104));
#49279=CARTESIAN_POINT('Ctrl Pts',(0.564245279537148,1.,-4.13348835727104));
#49280=CARTESIAN_POINT('Ctrl Pts',(0.559942890594773,-1.,-4.12695329951961));
#49281=CARTESIAN_POINT('Ctrl Pts',(0.559942890594773,1.,-4.12695329951961));
#49282=CARTESIAN_POINT('Ctrl Pts',(0.555673636129977,-1.,-4.12040666195664));
#49283=CARTESIAN_POINT('Ctrl Pts',(0.555673636129977,1.,-4.12040666195664));
#49284=CARTESIAN_POINT('Ctrl Pts',(0.551437758497032,-1.,-4.11384852024721));
#49285=CARTESIAN_POINT('Ctrl Pts',(0.551437758497032,1.,-4.11384852024721));
#49286=CARTESIAN_POINT('Ctrl Pts',(0.547235539485636,-1.,-4.10727897027977));
#49287=CARTESIAN_POINT('Ctrl Pts',(0.547235539485636,1.,-4.10727897027977));
#49288=CARTESIAN_POINT('Ctrl Pts',(0.543067286877757,-1.,-4.10069810243979));
#49289=CARTESIAN_POINT('Ctrl Pts',(0.543067286877757,1.,-4.10069810243979));
#49290=CARTESIAN_POINT('Ctrl Pts',(0.538933321179755,-1.,-4.09410597627));
#49291=CARTESIAN_POINT('Ctrl Pts',(0.538933321179755,1.,-4.09410597627));
#49292=CARTESIAN_POINT('Ctrl Pts',(0.534833963477273,-1.,-4.08750259988885));
#49293=CARTESIAN_POINT('Ctrl Pts',(0.534833963477273,1.,-4.08750259988885));
#49294=CARTESIAN_POINT('Ctrl Pts',(0.53076951872857,-1.,-4.08088789536836));
#49295=CARTESIAN_POINT('Ctrl Pts',(0.53076951872857,1.,-4.08088789536836));
#49296=CARTESIAN_POINT('Ctrl Pts',(0.526740277227498,-1.,-4.07426172299847));
#49297=CARTESIAN_POINT('Ctrl Pts',(0.526740277227498,1.,-4.07426172299847));
#49298=CARTESIAN_POINT('Ctrl Pts',(0.522746528603107,-1.,-4.06762394471314));
#49299=CARTESIAN_POINT('Ctrl Pts',(0.522746528603107,1.,-4.06762394471314));
#49300=CARTESIAN_POINT('Ctrl Pts',(0.518788572336923,-1.,-4.06097448038013));
#49301=CARTESIAN_POINT('Ctrl Pts',(0.518788572336923,1.,-4.06097448038013));
#49302=CARTESIAN_POINT('Ctrl Pts',(0.514866728193016,-1.,-4.05431335771199));
#49303=CARTESIAN_POINT('Ctrl Pts',(0.514866728193016,1.,-4.05431335771199));
#49304=CARTESIAN_POINT('Ctrl Pts',(0.51098134921897,-1.,-4.04764078815447));
#49305=CARTESIAN_POINT('Ctrl Pts',(0.51098134921897,1.,-4.04764078815447));
#49306=CARTESIAN_POINT('Ctrl Pts',(0.507132823288136,-1.,-4.04095715148915));
#49307=CARTESIAN_POINT('Ctrl Pts',(0.507132823288136,1.,-4.04095715148915));
#49308=CARTESIAN_POINT('Ctrl Pts',(0.503321556915346,-1.,-4.03426284174272));
#49309=CARTESIAN_POINT('Ctrl Pts',(0.503321556915346,1.,-4.03426284174272));
#49310=CARTESIAN_POINT('Ctrl Pts',(0.499547962340821,-1.,-4.02755813980101));
#49311=CARTESIAN_POINT('Ctrl Pts',(0.499547962340821,1.,-4.02755813980101));
#49312=CARTESIAN_POINT('Ctrl Pts',(0.495812444326251,-1.,-4.02084308851832));
#49313=CARTESIAN_POINT('Ctrl Pts',(0.495812444326251,1.,-4.02084308851832));
#49314=CARTESIAN_POINT('Ctrl Pts',(0.492115383418018,-1.,-4.01411733503546));
#49315=CARTESIAN_POINT('Ctrl Pts',(0.492115383418018,1.,-4.01411733503546));
#49316=CARTESIAN_POINT('Ctrl Pts',(0.488457130424633,-1.,-4.0073800839099));
#49317=CARTESIAN_POINT('Ctrl Pts',(0.488457130424633,1.,-4.0073800839099));
#49318=CARTESIAN_POINT('Ctrl Pts',(0.484838042421834,-1.,-4.00063045119288));
#49319=CARTESIAN_POINT('Ctrl Pts',(0.484838042421834,1.,-4.00063045119288));
#49320=CARTESIAN_POINT('Ctrl Pts',(0.481258512209675,-1.,-3.99386775880679));
#49321=CARTESIAN_POINT('Ctrl Pts',(0.481258512209675,1.,-3.99386775880679));
#49322=CARTESIAN_POINT('Ctrl Pts',(0.477718999122027,-1.,-3.98709184306738));
#49323=CARTESIAN_POINT('Ctrl Pts',(0.477718999122027,1.,-3.98709184306738));
#49324=CARTESIAN_POINT('Ctrl Pts',(0.474220061019509,-1.,-3.98030338044409));
#49325=CARTESIAN_POINT('Ctrl Pts',(0.474220061019509,1.,-3.98030338044409));
#49326=CARTESIAN_POINT('Ctrl Pts',(0.470762379613439,-1.,-3.97350414289392));
#49327=CARTESIAN_POINT('Ctrl Pts',(0.470762379613439,1.,-3.97350414289392));
#49328=CARTESIAN_POINT('Ctrl Pts',(0.467346690880643,-1.,-3.9666962227393));
#49329=CARTESIAN_POINT('Ctrl Pts',(0.467346690880643,1.,-3.9666962227393));
#49330=CARTESIAN_POINT('Ctrl Pts',(0.463973722115733,-1.,-3.95988133243538));
#49331=CARTESIAN_POINT('Ctrl Pts',(0.463973722115733,1.,-3.95988133243538));
#49332=CARTESIAN_POINT('Ctrl Pts',(0.460644124429121,-1.,-3.95306005817364));
#49333=CARTESIAN_POINT('Ctrl Pts',(0.460644124429121,1.,-3.95306005817364));
#49334=CARTESIAN_POINT('Ctrl Pts',(0.457358410451682,-1.,-3.94623117206678));
#49335=CARTESIAN_POINT('Ctrl Pts',(0.457358410451682,1.,-3.94623117206678));
#49336=CARTESIAN_POINT('Ctrl Pts',(0.454116879027584,-1.,-3.93939080846298));
#49337=CARTESIAN_POINT('Ctrl Pts',(0.454116879027584,1.,-3.93939080846298));
#49338=CARTESIAN_POINT('Ctrl Pts',(0.450919768356348,-1.,-3.93253407403123));
#49339=CARTESIAN_POINT('Ctrl Pts',(0.450919768356348,1.,-3.93253407403123));
#49340=CARTESIAN_POINT('Ctrl Pts',(0.447767416837292,-1.,-3.92565674143416));
#49341=CARTESIAN_POINT('Ctrl Pts',(0.447767416837292,1.,-3.92565674143416));
#49342=CARTESIAN_POINT('Ctrl Pts',(0.44466043023059,-1.,-3.91875701610719));
#49343=CARTESIAN_POINT('Ctrl Pts',(0.44466043023059,1.,-3.91875701610719));
#49344=CARTESIAN_POINT('Ctrl Pts',(0.441599824524054,-1.,-3.91183704069153));
#49345=CARTESIAN_POINT('Ctrl Pts',(0.441599824524054,1.,-3.91183704069153));
#49346=CARTESIAN_POINT('Ctrl Pts',(0.438587235458249,-1.,-3.90490512938563));
#49347=CARTESIAN_POINT('Ctrl Pts',(0.438587235458249,1.,-3.90490512938563));
#49348=CARTESIAN_POINT('Ctrl Pts',(0.435624629433527,-1.,-3.89797256655462));
#49349=CARTESIAN_POINT('Ctrl Pts',(0.435624629433527,1.,-3.89797256655462));
#49350=CARTESIAN_POINT('Ctrl Pts',(0.432713929544458,-1.,-3.89104947940611));
#49351=CARTESIAN_POINT('Ctrl Pts',(0.432713929544458,1.,-3.89104947940611));
#49352=CARTESIAN_POINT('Ctrl Pts',(0.429856640579741,-1.,-3.88414070943341));
#49353=CARTESIAN_POINT('Ctrl Pts',(0.429856640579741,1.,-3.88414070943341));
#49354=CARTESIAN_POINT('Ctrl Pts',(0.427053541173457,-1.,-3.87724240306597));
#49355=CARTESIAN_POINT('Ctrl Pts',(0.427053541173457,1.,-3.87724240306597));
#49356=CARTESIAN_POINT('Ctrl Pts',(0.42430417319511,-1.,-3.87033643487851));
#49357=CARTESIAN_POINT('Ctrl Pts',(0.42430417319511,1.,-3.87033643487851));
#49358=CARTESIAN_POINT('Ctrl Pts',(0.421607423177534,-1.,-3.86339652542709));
#49359=CARTESIAN_POINT('Ctrl Pts',(0.421607423177534,1.,-3.86339652542709));
#49360=CARTESIAN_POINT('Ctrl Pts',(0.418962468086773,-1.,-3.85639825647996));
#49361=CARTESIAN_POINT('Ctrl Pts',(0.418962468086773,1.,-3.85639825647996));
#49362=CARTESIAN_POINT('Ctrl Pts',(0.416369678052906,-1.,-3.84932864157497));
#49363=CARTESIAN_POINT('Ctrl Pts',(0.416369678052906,1.,-3.84932864157497));
#49364=CARTESIAN_POINT('Ctrl Pts',(0.413831367016748,-1.,-3.84219403994762));
#49365=CARTESIAN_POINT('Ctrl Pts',(0.413831367016748,1.,-3.84219403994762));
#49366=CARTESIAN_POINT('Ctrl Pts',(0.411353038798518,-1.,-3.83503345578698));
#49367=CARTESIAN_POINT('Ctrl Pts',(0.411353038798518,1.,-3.83503345578698));
#49368=CARTESIAN_POINT('Ctrl Pts',(0.408942371447459,-1.,-3.82790724256471));
#49369=CARTESIAN_POINT('Ctrl Pts',(0.408942371447459,1.,-3.82790724256471));
#49370=CARTESIAN_POINT('Ctrl Pts',(0.406607038258985,-1.,-3.8208730391381));
#49371=CARTESIAN_POINT('Ctrl Pts',(0.406607038258985,1.,-3.8208730391381));
#49372=CARTESIAN_POINT('Ctrl Pts',(0.404352694628273,-1.,-3.81396374287793));
#49373=CARTESIAN_POINT('Ctrl Pts',(0.404352694628273,1.,-3.81396374287793));
#49374=CARTESIAN_POINT('Ctrl Pts',(0.402181320148435,-1.,-3.80716881962728));
#49375=CARTESIAN_POINT('Ctrl Pts',(0.402181320148435,1.,-3.80716881962728));
#49376=CARTESIAN_POINT('Ctrl Pts',(0.4000883465046,-1.,-3.80040370384546));
#49377=CARTESIAN_POINT('Ctrl Pts',(0.4000883465046,1.,-3.80040370384546));
#49378=CARTESIAN_POINT('Ctrl Pts',(0.398064818683969,-1.,-3.7935288716329));
#49379=CARTESIAN_POINT('Ctrl Pts',(0.398064818683969,1.,-3.7935288716329));
#49380=CARTESIAN_POINT('Ctrl Pts',(0.39610320533484,-1.,-3.78640521279313));
#49381=CARTESIAN_POINT('Ctrl Pts',(0.39610320533484,1.,-3.78640521279313));
#49382=CARTESIAN_POINT('Ctrl Pts',(0.394202481011499,-1.,-3.77894173114283));
#49383=CARTESIAN_POINT('Ctrl Pts',(0.394202481011499,1.,-3.77894173114283));
#49384=CARTESIAN_POINT('Ctrl Pts',(0.392372786223432,-1.,-3.77114011595967));
#49385=CARTESIAN_POINT('Ctrl Pts',(0.392372786223432,1.,-3.77114011595967));
#49386=CARTESIAN_POINT('Ctrl Pts',(0.390642072979559,-1.,-3.76315635033257));
#49387=CARTESIAN_POINT('Ctrl Pts',(0.390642072979559,1.,-3.76315635033257));
#49388=CARTESIAN_POINT('Ctrl Pts',(0.389054775898701,-1.,-3.75529302895152));
#49389=CARTESIAN_POINT('Ctrl Pts',(0.389054775898701,1.,-3.75529302895152));
#49390=CARTESIAN_POINT('Ctrl Pts',(0.387663020050836,-1.,-3.74792651696654));
#49391=CARTESIAN_POINT('Ctrl Pts',(0.387663020050836,1.,-3.74792651696654));
#49392=CARTESIAN_POINT('Ctrl Pts',(0.386519576222251,-1.,-3.74144965781276));
#49393=CARTESIAN_POINT('Ctrl Pts',(0.386519576222251,1.,-3.74144965781276));
#49394=CARTESIAN_POINT('Ctrl Pts',(0.385670806454565,-1.,-3.73621371845318));
#49395=CARTESIAN_POINT('Ctrl Pts',(0.385670806454565,1.,-3.73621371845318));
#49396=CARTESIAN_POINT('Ctrl Pts',(0.385147887988951,-1.,-3.73245705638843));
#49397=CARTESIAN_POINT('Ctrl Pts',(0.385147887988951,1.,-3.73245705638843));
#49398=CARTESIAN_POINT('Ctrl Pts',(0.385001870183213,-1.,-3.73072465900175));
#49399=CARTESIAN_POINT('Ctrl Pts',(0.385001870183213,1.,-3.73072465900175));
#49400=CARTESIAN_POINT('Ctrl Pts',(0.385047711603462,-1.,-3.73015851028356));
#49401=CARTESIAN_POINT('Ctrl Pts',(0.385047711603462,1.,-3.73015851028356));
#49402=CARTESIAN_POINT('Ctrl Pts',(0.385147278814642,-1.,-3.73010668803042));
#49403=CARTESIAN_POINT('Ctrl Pts',(0.385147278814642,1.,-3.73010668803042));
#49404=CARTESIAN_POINT('Ctrl Pts',(0.385214314776329,-1.,-3.73016218570874));
#49405=CARTESIAN_POINT('Ctrl Pts',(0.385214314776329,1.,-3.73016218570874));
#49406=CARTESIAN_POINT('',(0.581791163835815,1.,-4.15950947128175));
#49407=CARTESIAN_POINT('Ctrl Pts',(0.581791163835815,1.,-4.15950947128175));
#49408=CARTESIAN_POINT('Ctrl Pts',(0.580901211463535,1.,-4.1582129171283));
#49409=CARTESIAN_POINT('Ctrl Pts',(0.579124568914235,1.,-4.15561864788576));
#49410=CARTESIAN_POINT('Ctrl Pts',(0.576469391676688,1.,-4.151723761217));
#49411=CARTESIAN_POINT('Ctrl Pts',(0.572948736069522,1.,-4.14652361068081));
#49412=CARTESIAN_POINT('Ctrl Pts',(0.568580610189774,1.,-4.14001179830547));
#49413=CARTESIAN_POINT('Ctrl Pts',(0.564245279537148,1.,-4.13348835727104));
#49414=CARTESIAN_POINT('Ctrl Pts',(0.559942890594773,1.,-4.12695329951961));
#49415=CARTESIAN_POINT('Ctrl Pts',(0.555673636129977,1.,-4.12040666195664));
#49416=CARTESIAN_POINT('Ctrl Pts',(0.551437758497032,1.,-4.11384852024721));
#49417=CARTESIAN_POINT('Ctrl Pts',(0.547235539485636,1.,-4.10727897027977));
#49418=CARTESIAN_POINT('Ctrl Pts',(0.543067286877757,1.,-4.10069810243979));
#49419=CARTESIAN_POINT('Ctrl Pts',(0.538933321179755,1.,-4.09410597627));
#49420=CARTESIAN_POINT('Ctrl Pts',(0.534833963477273,1.,-4.08750259988885));
#49421=CARTESIAN_POINT('Ctrl Pts',(0.53076951872857,1.,-4.08088789536836));
#49422=CARTESIAN_POINT('Ctrl Pts',(0.526740277227498,1.,-4.07426172299847));
#49423=CARTESIAN_POINT('Ctrl Pts',(0.522746528603107,1.,-4.06762394471314));
#49424=CARTESIAN_POINT('Ctrl Pts',(0.518788572336923,1.,-4.06097448038013));
#49425=CARTESIAN_POINT('Ctrl Pts',(0.514866728193016,1.,-4.05431335771199));
#49426=CARTESIAN_POINT('Ctrl Pts',(0.51098134921897,1.,-4.04764078815447));
#49427=CARTESIAN_POINT('Ctrl Pts',(0.507132823288136,1.,-4.04095715148915));
#49428=CARTESIAN_POINT('Ctrl Pts',(0.503321556915346,1.,-4.03426284174272));
#49429=CARTESIAN_POINT('Ctrl Pts',(0.499547962340821,1.,-4.02755813980101));
#49430=CARTESIAN_POINT('Ctrl Pts',(0.495812444326251,1.,-4.02084308851832));
#49431=CARTESIAN_POINT('Ctrl Pts',(0.492115383418018,1.,-4.01411733503546));
#49432=CARTESIAN_POINT('Ctrl Pts',(0.488457130424633,1.,-4.0073800839099));
#49433=CARTESIAN_POINT('Ctrl Pts',(0.484838042421834,1.,-4.00063045119288));
#49434=CARTESIAN_POINT('Ctrl Pts',(0.481258512209675,1.,-3.99386775880679));
#49435=CARTESIAN_POINT('Ctrl Pts',(0.477718999122027,1.,-3.98709184306738));
#49436=CARTESIAN_POINT('Ctrl Pts',(0.474220061019509,1.,-3.98030338044409));
#49437=CARTESIAN_POINT('Ctrl Pts',(0.470762379613439,1.,-3.97350414289392));
#49438=CARTESIAN_POINT('Ctrl Pts',(0.467346690880643,1.,-3.9666962227393));
#49439=CARTESIAN_POINT('Ctrl Pts',(0.463973722115733,1.,-3.95988133243538));
#49440=CARTESIAN_POINT('Ctrl Pts',(0.460644124429121,1.,-3.95306005817364));
#49441=CARTESIAN_POINT('Ctrl Pts',(0.457358410451682,1.,-3.94623117206678));
#49442=CARTESIAN_POINT('Ctrl Pts',(0.454116879027584,1.,-3.93939080846298));
#49443=CARTESIAN_POINT('Ctrl Pts',(0.450919768356348,1.,-3.93253407403123));
#49444=CARTESIAN_POINT('Ctrl Pts',(0.447767416837292,1.,-3.92565674143416));
#49445=CARTESIAN_POINT('Ctrl Pts',(0.44466043023059,1.,-3.91875701610719));
#49446=CARTESIAN_POINT('Ctrl Pts',(0.441599824524054,1.,-3.91183704069153));
#49447=CARTESIAN_POINT('Ctrl Pts',(0.438587235458249,1.,-3.90490512938563));
#49448=CARTESIAN_POINT('Ctrl Pts',(0.435624629433527,1.,-3.89797256655462));
#49449=CARTESIAN_POINT('Ctrl Pts',(0.432713929544458,1.,-3.89104947940611));
#49450=CARTESIAN_POINT('Ctrl Pts',(0.429856640579741,1.,-3.88414070943341));
#49451=CARTESIAN_POINT('Ctrl Pts',(0.427053541173457,1.,-3.87724240306597));
#49452=CARTESIAN_POINT('Ctrl Pts',(0.42430417319511,1.,-3.87033643487851));
#49453=CARTESIAN_POINT('Ctrl Pts',(0.421607423177534,1.,-3.86339652542709));
#49454=CARTESIAN_POINT('Ctrl Pts',(0.418962468086773,1.,-3.85639825647996));
#49455=CARTESIAN_POINT('Ctrl Pts',(0.416369678052906,1.,-3.84932864157497));
#49456=CARTESIAN_POINT('Ctrl Pts',(0.413831367016748,1.,-3.84219403994762));
#49457=CARTESIAN_POINT('Ctrl Pts',(0.411353038798518,1.,-3.83503345578698));
#49458=CARTESIAN_POINT('Ctrl Pts',(0.408942371447459,1.,-3.82790724256471));
#49459=CARTESIAN_POINT('Ctrl Pts',(0.406607038258985,1.,-3.8208730391381));
#49460=CARTESIAN_POINT('Ctrl Pts',(0.404352694628273,1.,-3.81396374287793));
#49461=CARTESIAN_POINT('Ctrl Pts',(0.402181320148435,1.,-3.80716881962728));
#49462=CARTESIAN_POINT('Ctrl Pts',(0.4000883465046,1.,-3.80040370384546));
#49463=CARTESIAN_POINT('Ctrl Pts',(0.398064818683969,1.,-3.7935288716329));
#49464=CARTESIAN_POINT('Ctrl Pts',(0.39610320533484,1.,-3.78640521279313));
#49465=CARTESIAN_POINT('Ctrl Pts',(0.394202481011499,1.,-3.77894173114283));
#49466=CARTESIAN_POINT('Ctrl Pts',(0.392372786223432,1.,-3.77114011595967));
#49467=CARTESIAN_POINT('Ctrl Pts',(0.390642072979559,1.,-3.76315635033257));
#49468=CARTESIAN_POINT('Ctrl Pts',(0.389054775898701,1.,-3.75529302895152));
#49469=CARTESIAN_POINT('Ctrl Pts',(0.387663020050836,1.,-3.74792651696654));
#49470=CARTESIAN_POINT('Ctrl Pts',(0.386519576222251,1.,-3.74144965781276));
#49471=CARTESIAN_POINT('Ctrl Pts',(0.385670806454565,1.,-3.73621371845318));
#49472=CARTESIAN_POINT('Ctrl Pts',(0.385187124634206,1.,-3.73273893363406));
#49473=CARTESIAN_POINT('Ctrl Pts',(0.385031656499163,1.,-3.73106082862548));
#49474=CARTESIAN_POINT('Ctrl Pts',(0.385037797881504,1.,-3.73040527621055));
#49475=CARTESIAN_POINT('Ctrl Pts',(0.385087139000374,1.,-3.73021431755274));
#49476=CARTESIAN_POINT('Ctrl Pts',(0.385112848330761,1.,-3.73017266276651));
#49477=CARTESIAN_POINT('',(0.581791163835815,0.,-4.15950947128175));
#49478=CARTESIAN_POINT('Ctrl Pts',(0.786322922920599,-1.,-3.66663282329846));
#49479=CARTESIAN_POINT('Ctrl Pts',(0.786322922920599,1.,-3.66663282329846));
#49480=CARTESIAN_POINT('Ctrl Pts',(0.786369528183326,-1.,-3.66655932661986));
#49481=CARTESIAN_POINT('Ctrl Pts',(0.786369528183326,1.,-3.66655932661986));
#49482=CARTESIAN_POINT('Ctrl Pts',(0.786480236185696,-1.,-3.66657784455334));
#49483=CARTESIAN_POINT('Ctrl Pts',(0.786480236185696,1.,-3.66657784455334));
#49484=CARTESIAN_POINT('Ctrl Pts',(0.786698783542764,-1.,-3.66710211820482));
#49485=CARTESIAN_POINT('Ctrl Pts',(0.786698783542764,1.,-3.66710211820482));
#49486=CARTESIAN_POINT('Ctrl Pts',(0.787095252590501,-1.,-3.66879484801113));
#49487=CARTESIAN_POINT('Ctrl Pts',(0.787095252590501,1.,-3.66879484801113));
#49488=CARTESIAN_POINT('Ctrl Pts',(0.787758799995742,-1.,-3.67252923663655));
#49489=CARTESIAN_POINT('Ctrl Pts',(0.787758799995742,1.,-3.67252923663655));
#49490=CARTESIAN_POINT('Ctrl Pts',(0.788569566220285,-1.,-3.67777119516252));
#49491=CARTESIAN_POINT('Ctrl Pts',(0.788569566220285,1.,-3.67777119516252));
#49492=CARTESIAN_POINT('Ctrl Pts',(0.789483546064386,-1.,-3.68428439783905));
#49493=CARTESIAN_POINT('Ctrl Pts',(0.789483546064386,1.,-3.68428439783905));
#49494=CARTESIAN_POINT('Ctrl Pts',(0.790436284988787,-1.,-3.69172044327364));
#49495=CARTESIAN_POINT('Ctrl Pts',(0.790436284988787,1.,-3.69172044327364));
#49496=CARTESIAN_POINT('Ctrl Pts',(0.79135657569598,-1.,-3.69968940808721));
#49497=CARTESIAN_POINT('Ctrl Pts',(0.79135657569598,1.,-3.69968940808721));
#49498=CARTESIAN_POINT('Ctrl Pts',(0.792177688845817,-1.,-3.70781724021806));
#49499=CARTESIAN_POINT('Ctrl Pts',(0.792177688845817,1.,-3.70781724021806));
#49500=CARTESIAN_POINT('Ctrl Pts',(0.792848377370287,-1.,-3.71580242396124));
#49501=CARTESIAN_POINT('Ctrl Pts',(0.792848377370287,1.,-3.71580242396124));
#49502=CARTESIAN_POINT('Ctrl Pts',(0.793347023784204,-1.,-3.72348797293734));
#49503=CARTESIAN_POINT('Ctrl Pts',(0.793347023784204,1.,-3.72348797293734));
#49504=CARTESIAN_POINT('Ctrl Pts',(0.793682750269684,-1.,-3.73086914695805));
#49505=CARTESIAN_POINT('Ctrl Pts',(0.793682750269684,1.,-3.73086914695805));
#49506=CARTESIAN_POINT('Ctrl Pts',(0.793882700937016,-1.,-3.73803280541687));
#49507=CARTESIAN_POINT('Ctrl Pts',(0.793882700937016,1.,-3.73803280541687));
#49508=CARTESIAN_POINT('Ctrl Pts',(0.793982700459951,-1.,-3.74511357728861));
#49509=CARTESIAN_POINT('Ctrl Pts',(0.793982700459951,1.,-3.74511357728861));
#49510=CARTESIAN_POINT('Ctrl Pts',(0.794017347371377,-1.,-3.75224692493864));
#49511=CARTESIAN_POINT('Ctrl Pts',(0.794017347371377,1.,-3.75224692493864));
#49512=CARTESIAN_POINT('Ctrl Pts',(0.794008429134907,-1.,-3.75951468666257));
#49513=CARTESIAN_POINT('Ctrl Pts',(0.794008429134907,1.,-3.75951468666257));
#49514=CARTESIAN_POINT('Ctrl Pts',(0.793961083688991,-1.,-3.76692626931111));
#49515=CARTESIAN_POINT('Ctrl Pts',(0.793961083688991,1.,-3.76692626931111));
#49516=CARTESIAN_POINT('Ctrl Pts',(0.793870523787407,-1.,-3.77444863801212));
#49517=CARTESIAN_POINT('Ctrl Pts',(0.793870523787407,1.,-3.77444863801212));
#49518=CARTESIAN_POINT('Ctrl Pts',(0.7937262357813,-1.,-3.78202460377598));
#49519=CARTESIAN_POINT('Ctrl Pts',(0.7937262357813,1.,-3.78202460377598));
#49520=CARTESIAN_POINT('Ctrl Pts',(0.793516871680993,-1.,-3.78959439439235));
#49521=CARTESIAN_POINT('Ctrl Pts',(0.793516871680993,1.,-3.78959439439235));
#49522=CARTESIAN_POINT('Ctrl Pts',(0.793235612973273,-1.,-3.79711921389897));
#49523=CARTESIAN_POINT('Ctrl Pts',(0.793235612973273,1.,-3.79711921389897));
#49524=CARTESIAN_POINT('Ctrl Pts',(0.792882695234777,-1.,-3.80459229925637));
#49525=CARTESIAN_POINT('Ctrl Pts',(0.792882695234777,1.,-3.80459229925637));
#49526=CARTESIAN_POINT('Ctrl Pts',(0.792462483517634,-1.,-3.81202588694756));
#49527=CARTESIAN_POINT('Ctrl Pts',(0.792462483517634,1.,-3.81202588694756));
#49528=CARTESIAN_POINT('Ctrl Pts',(0.791981740718634,-1.,-3.81944345442249));
#49529=CARTESIAN_POINT('Ctrl Pts',(0.791981740718634,1.,-3.81944345442249));
#49530=CARTESIAN_POINT('Ctrl Pts',(0.791447528662369,-1.,-3.82687033899792));
#49531=CARTESIAN_POINT('Ctrl Pts',(0.791447528662369,1.,-3.82687033899792));
#49532=CARTESIAN_POINT('Ctrl Pts',(0.7908650127053,-1.,-3.83432392054786));
#49533=CARTESIAN_POINT('Ctrl Pts',(0.7908650127053,1.,-3.83432392054786));
#49534=CARTESIAN_POINT('Ctrl Pts',(0.790236124191242,-1.,-3.84180762342454));
#49535=CARTESIAN_POINT('Ctrl Pts',(0.790236124191242,1.,-3.84180762342454));
#49536=CARTESIAN_POINT('Ctrl Pts',(0.789560798155582,-1.,-3.84931637808894));
#49537=CARTESIAN_POINT('Ctrl Pts',(0.789560798155582,1.,-3.84931637808894));
#49538=CARTESIAN_POINT('Ctrl Pts',(0.788837734090671,-1.,-3.85683995872529));
#49539=CARTESIAN_POINT('Ctrl Pts',(0.788837734090671,1.,-3.85683995872529));
#49540=CARTESIAN_POINT('Ctrl Pts',(0.788065315093777,-1.,-3.86436702561345));
#49541=CARTESIAN_POINT('Ctrl Pts',(0.788065315093777,1.,-3.86436702561345));
#49542=CARTESIAN_POINT('Ctrl Pts',(0.787242527617999,-1.,-3.87188916600912));
#49543=CARTESIAN_POINT('Ctrl Pts',(0.787242527617999,1.,-3.87188916600912));
#49544=CARTESIAN_POINT('Ctrl Pts',(0.786369675812608,-1.,-3.8794040281819));
#49545=CARTESIAN_POINT('Ctrl Pts',(0.786369675812608,1.,-3.8794040281819));
#49546=CARTESIAN_POINT('Ctrl Pts',(0.78544789034073,-1.,-3.88691313167398));
#49547=CARTESIAN_POINT('Ctrl Pts',(0.78544789034073,1.,-3.88691313167398));
#49548=CARTESIAN_POINT('Ctrl Pts',(0.784478799358336,-1.,-3.89442039235103));
#49549=CARTESIAN_POINT('Ctrl Pts',(0.784478799358336,1.,-3.89442039235103));
#49550=CARTESIAN_POINT('Ctrl Pts',(0.783464141529081,-1.,-3.9019303904397));
#49551=CARTESIAN_POINT('Ctrl Pts',(0.783464141529081,1.,-3.9019303904397));
#49552=CARTESIAN_POINT('Ctrl Pts',(0.782405395622764,-1.,-3.90944671004542));
#49553=CARTESIAN_POINT('Ctrl Pts',(0.782405395622764,1.,-3.90944671004542));
#49554=CARTESIAN_POINT('Ctrl Pts',(0.781303428618366,-1.,-3.91697036054676));
#49555=CARTESIAN_POINT('Ctrl Pts',(0.781303428618366,1.,-3.91697036054676));
#49556=CARTESIAN_POINT('Ctrl Pts',(0.780158678615542,-1.,-3.92450058323823));
#49557=CARTESIAN_POINT('Ctrl Pts',(0.780158678615542,1.,-3.92450058323823));
#49558=CARTESIAN_POINT('Ctrl Pts',(0.77897130813482,-1.,-3.93203552473174));
#49559=CARTESIAN_POINT('Ctrl Pts',(0.77897130813482,1.,-3.93203552473174));
#49560=CARTESIAN_POINT('Ctrl Pts',(0.777741370568558,-1.,-3.93957296768103));
#49561=CARTESIAN_POINT('Ctrl Pts',(0.777741370568558,1.,-3.93957296768103));
#49562=CARTESIAN_POINT('Ctrl Pts',(0.776468966697921,-1.,-3.94711101619447));
#49563=CARTESIAN_POINT('Ctrl Pts',(0.776468966697921,1.,-3.94711101619447));
#49564=CARTESIAN_POINT('Ctrl Pts',(0.775154418039351,-1.,-3.9546488545231));
#49565=CARTESIAN_POINT('Ctrl Pts',(0.775154418039351,1.,-3.9546488545231));
#49566=CARTESIAN_POINT('Ctrl Pts',(0.773798212026565,-1.,-3.96218649639807));
#49567=CARTESIAN_POINT('Ctrl Pts',(0.773798212026565,1.,-3.96218649639807));
#49568=CARTESIAN_POINT('Ctrl Pts',(0.772400931772136,-1.,-3.96972446532772));
#49569=CARTESIAN_POINT('Ctrl Pts',(0.772400931772136,1.,-3.96972446532772));
#49570=CARTESIAN_POINT('Ctrl Pts',(0.77096319003047,-1.,-3.97726349165488));
#49571=CARTESIAN_POINT('Ctrl Pts',(0.77096319003047,1.,-3.97726349165488));
#49572=CARTESIAN_POINT('Ctrl Pts',(0.769485566245544,-1.,-3.98480422348451));
#49573=CARTESIAN_POINT('Ctrl Pts',(0.769485566245544,1.,-3.98480422348451));
#49574=CARTESIAN_POINT('Ctrl Pts',(0.767968531377914,-1.,-3.9923468788101));
#49575=CARTESIAN_POINT('Ctrl Pts',(0.767968531377914,1.,-3.9923468788101));
#49576=CARTESIAN_POINT('Ctrl Pts',(0.766412457136063,-1.,-3.99989129179622));
#49577=CARTESIAN_POINT('Ctrl Pts',(0.766412457136063,1.,-3.99989129179622));
#49578=CARTESIAN_POINT('Ctrl Pts',(0.764817648785197,-1.,-4.00743706791509));
#49579=CARTESIAN_POINT('Ctrl Pts',(0.764817648785197,1.,-4.00743706791509));
#49580=CARTESIAN_POINT('Ctrl Pts',(0.763184371182935,-1.,-4.01498370680496));
#49581=CARTESIAN_POINT('Ctrl Pts',(0.763184371182935,1.,-4.01498370680496));
#49582=CARTESIAN_POINT('Ctrl Pts',(0.761512875859804,-1.,-4.02253072741268));
#49583=CARTESIAN_POINT('Ctrl Pts',(0.761512875859804,1.,-4.02253072741268));
#49584=CARTESIAN_POINT('Ctrl Pts',(0.759803433243751,-1.,-4.03007781954412));
#49585=CARTESIAN_POINT('Ctrl Pts',(0.759803433243751,1.,-4.03007781954412));
#49586=CARTESIAN_POINT('Ctrl Pts',(0.758056338884944,-1.,-4.03762485803119));
#49587=CARTESIAN_POINT('Ctrl Pts',(0.758056338884944,1.,-4.03762485803119));
#49588=CARTESIAN_POINT('Ctrl Pts',(0.75627190236958,-1.,-4.04517182653997));
#49589=CARTESIAN_POINT('Ctrl Pts',(0.75627190236958,1.,-4.04517182653997));
#49590=CARTESIAN_POINT('Ctrl Pts',(0.754450441816078,-1.,-4.05271876687915));
#49591=CARTESIAN_POINT('Ctrl Pts',(0.754450441816078,1.,-4.05271876687915));
#49592=CARTESIAN_POINT('Ctrl Pts',(0.752592276483072,-1.,-4.06026572221515));
#49593=CARTESIAN_POINT('Ctrl Pts',(0.752592276483072,1.,-4.06026572221515));
#49594=CARTESIAN_POINT('Ctrl Pts',(0.750697720484036,-1.,-4.06781267242378));
#49595=CARTESIAN_POINT('Ctrl Pts',(0.750697720484036,1.,-4.06781267242378));
#49596=CARTESIAN_POINT('Ctrl Pts',(0.748767076680557,-1.,-4.07535951056152));
#49597=CARTESIAN_POINT('Ctrl Pts',(0.748767076680557,1.,-4.07535951056152));
#49598=CARTESIAN_POINT('Ctrl Pts',(0.746800631492315,-1.,-4.08290608095642));
#49599=CARTESIAN_POINT('Ctrl Pts',(0.746800631492315,1.,-4.08290608095642));
#49600=CARTESIAN_POINT('Ctrl Pts',(0.7447986497065,-1.,-4.09045220253573));
#49601=CARTESIAN_POINT('Ctrl Pts',(0.7447986497065,1.,-4.09045220253573));
#49602=CARTESIAN_POINT('Ctrl Pts',(0.742761369689841,-1.,-4.09799769702611));
#49603=CARTESIAN_POINT('Ctrl Pts',(0.742761369689841,1.,-4.09799769702611));
#49604=CARTESIAN_POINT('Ctrl Pts',(0.740688998553376,-1.,-4.10554241757547));
#49605=CARTESIAN_POINT('Ctrl Pts',(0.740688998553376,1.,-4.10554241757547));
#49606=CARTESIAN_POINT('Ctrl Pts',(0.738581708225843,-1.,-4.11308626951927));
#49607=CARTESIAN_POINT('Ctrl Pts',(0.738581708225843,1.,-4.11308626951927));
#49608=CARTESIAN_POINT('Ctrl Pts',(0.736439634331344,-1.,-4.120629196238));
#49609=CARTESIAN_POINT('Ctrl Pts',(0.736439634331344,1.,-4.120629196238));
#49610=CARTESIAN_POINT('Ctrl Pts',(0.734698226764092,-1.,-4.12666277570844));
#49611=CARTESIAN_POINT('Ctrl Pts',(0.734698226764092,1.,-4.12666277570844));
#49612=CARTESIAN_POINT('Ctrl Pts',(0.733376589323546,-1.,-4.13118752795207));
#49613=CARTESIAN_POINT('Ctrl Pts',(0.733376589323546,1.,-4.13118752795207));
#49614=CARTESIAN_POINT('Ctrl Pts',(0.732488575135159,-1.,-4.1342038373684));
#49615=CARTESIAN_POINT('Ctrl Pts',(0.732488575135159,1.,-4.1342038373684));
#49616=CARTESIAN_POINT('Ctrl Pts',(0.73204283740062,-1.,-4.13571194405636));
#49617=CARTESIAN_POINT('Ctrl Pts',(0.73204283740062,1.,-4.13571194405636));
#49618=CARTESIAN_POINT('',(0.786422660831986,1.,-3.66661143271685));
#49619=CARTESIAN_POINT('Ctrl Pts',(0.786422660831985,-1.,-3.66661143271685));
#49620=CARTESIAN_POINT('Ctrl Pts',(0.786422660831985,-0.666666666666667,
-3.66661143271685));
#49621=CARTESIAN_POINT('Ctrl Pts',(0.786422660831985,-0.333333333333333,
-3.66661143271685));
#49622=CARTESIAN_POINT('Ctrl Pts',(0.786422660831985,0.333333333333333,
-3.66661143271685));
#49623=CARTESIAN_POINT('Ctrl Pts',(0.786422660831985,0.666666666666667,
-3.66661143271685));
#49624=CARTESIAN_POINT('Ctrl Pts',(0.786422660831985,1.,-3.66661143271685));
#49625=CARTESIAN_POINT('',(0.73204283740062,1.,-4.13571194405636));
#49626=CARTESIAN_POINT('',(0.73204283740062,0.,-4.13571194405636));
#49627=CARTESIAN_POINT('Ctrl Pts',(0.786422660831986,1.,-3.66661143271685));
#49628=CARTESIAN_POINT('Ctrl Pts',(0.786459983895432,1.,-3.6666431041522));
#49629=CARTESIAN_POINT('Ctrl Pts',(0.786565919558984,1.,-3.66680946938293));
#49630=CARTESIAN_POINT('Ctrl Pts',(0.786774337198062,1.,-3.66743103898702));
#49631=CARTESIAN_POINT('Ctrl Pts',(0.787145041181546,1.,-3.66907505398677));
#49632=CARTESIAN_POINT('Ctrl Pts',(0.787758799995742,1.,-3.67252923663655));
#49633=CARTESIAN_POINT('Ctrl Pts',(0.788569566220285,1.,-3.67777119516252));
#49634=CARTESIAN_POINT('Ctrl Pts',(0.789483546064386,1.,-3.68428439783905));
#49635=CARTESIAN_POINT('Ctrl Pts',(0.790436284988787,1.,-3.69172044327364));
#49636=CARTESIAN_POINT('Ctrl Pts',(0.79135657569598,1.,-3.69968940808721));
#49637=CARTESIAN_POINT('Ctrl Pts',(0.792177688845817,1.,-3.70781724021806));
#49638=CARTESIAN_POINT('Ctrl Pts',(0.792848377370287,1.,-3.71580242396124));
#49639=CARTESIAN_POINT('Ctrl Pts',(0.793347023784204,1.,-3.72348797293734));
#49640=CARTESIAN_POINT('Ctrl Pts',(0.793682750269684,1.,-3.73086914695805));
#49641=CARTESIAN_POINT('Ctrl Pts',(0.793882700937016,1.,-3.73803280541687));
#49642=CARTESIAN_POINT('Ctrl Pts',(0.793982700459951,1.,-3.74511357728861));
#49643=CARTESIAN_POINT('Ctrl Pts',(0.794017347371377,1.,-3.75224692493864));
#49644=CARTESIAN_POINT('Ctrl Pts',(0.794008429134907,1.,-3.75951468666257));
#49645=CARTESIAN_POINT('Ctrl Pts',(0.793961083688991,1.,-3.76692626931111));
#49646=CARTESIAN_POINT('Ctrl Pts',(0.793870523787407,1.,-3.77444863801212));
#49647=CARTESIAN_POINT('Ctrl Pts',(0.7937262357813,1.,-3.78202460377598));
#49648=CARTESIAN_POINT('Ctrl Pts',(0.793516871680993,1.,-3.78959439439235));
#49649=CARTESIAN_POINT('Ctrl Pts',(0.793235612973273,1.,-3.79711921389897));
#49650=CARTESIAN_POINT('Ctrl Pts',(0.792882695234777,1.,-3.80459229925637));
#49651=CARTESIAN_POINT('Ctrl Pts',(0.792462483517634,1.,-3.81202588694756));
#49652=CARTESIAN_POINT('Ctrl Pts',(0.791981740718634,1.,-3.81944345442249));
#49653=CARTESIAN_POINT('Ctrl Pts',(0.791447528662369,1.,-3.82687033899792));
#49654=CARTESIAN_POINT('Ctrl Pts',(0.7908650127053,1.,-3.83432392054786));
#49655=CARTESIAN_POINT('Ctrl Pts',(0.790236124191242,1.,-3.84180762342454));
#49656=CARTESIAN_POINT('Ctrl Pts',(0.789560798155582,1.,-3.84931637808894));
#49657=CARTESIAN_POINT('Ctrl Pts',(0.788837734090671,1.,-3.85683995872529));
#49658=CARTESIAN_POINT('Ctrl Pts',(0.788065315093777,1.,-3.86436702561345));
#49659=CARTESIAN_POINT('Ctrl Pts',(0.787242527617999,1.,-3.87188916600912));
#49660=CARTESIAN_POINT('Ctrl Pts',(0.786369675812608,1.,-3.8794040281819));
#49661=CARTESIAN_POINT('Ctrl Pts',(0.78544789034073,1.,-3.88691313167398));
#49662=CARTESIAN_POINT('Ctrl Pts',(0.784478799358336,1.,-3.89442039235103));
#49663=CARTESIAN_POINT('Ctrl Pts',(0.783464141529081,1.,-3.9019303904397));
#49664=CARTESIAN_POINT('Ctrl Pts',(0.782405395622764,1.,-3.90944671004542));
#49665=CARTESIAN_POINT('Ctrl Pts',(0.781303428618366,1.,-3.91697036054676));
#49666=CARTESIAN_POINT('Ctrl Pts',(0.780158678615542,1.,-3.92450058323823));
#49667=CARTESIAN_POINT('Ctrl Pts',(0.77897130813482,1.,-3.93203552473174));
#49668=CARTESIAN_POINT('Ctrl Pts',(0.777741370568558,1.,-3.93957296768103));
#49669=CARTESIAN_POINT('Ctrl Pts',(0.776468966697921,1.,-3.94711101619447));
#49670=CARTESIAN_POINT('Ctrl Pts',(0.775154418039351,1.,-3.9546488545231));
#49671=CARTESIAN_POINT('Ctrl Pts',(0.773798212026565,1.,-3.96218649639807));
#49672=CARTESIAN_POINT('Ctrl Pts',(0.772400931772136,1.,-3.96972446532772));
#49673=CARTESIAN_POINT('Ctrl Pts',(0.77096319003047,1.,-3.97726349165488));
#49674=CARTESIAN_POINT('Ctrl Pts',(0.769485566245544,1.,-3.98480422348451));
#49675=CARTESIAN_POINT('Ctrl Pts',(0.767968531377914,1.,-3.9923468788101));
#49676=CARTESIAN_POINT('Ctrl Pts',(0.766412457136063,1.,-3.99989129179622));
#49677=CARTESIAN_POINT('Ctrl Pts',(0.764817648785197,1.,-4.00743706791509));
#49678=CARTESIAN_POINT('Ctrl Pts',(0.763184371182935,1.,-4.01498370680496));
#49679=CARTESIAN_POINT('Ctrl Pts',(0.761512875859804,1.,-4.02253072741268));
#49680=CARTESIAN_POINT('Ctrl Pts',(0.759803433243751,1.,-4.03007781954412));
#49681=CARTESIAN_POINT('Ctrl Pts',(0.758056338884944,1.,-4.03762485803119));
#49682=CARTESIAN_POINT('Ctrl Pts',(0.75627190236958,1.,-4.04517182653997));
#49683=CARTESIAN_POINT('Ctrl Pts',(0.754450441816078,1.,-4.05271876687915));
#49684=CARTESIAN_POINT('Ctrl Pts',(0.752592276483072,1.,-4.06026572221515));
#49685=CARTESIAN_POINT('Ctrl Pts',(0.750697720484036,1.,-4.06781267242378));
#49686=CARTESIAN_POINT('Ctrl Pts',(0.748767076680557,1.,-4.07535951056152));
#49687=CARTESIAN_POINT('Ctrl Pts',(0.746800631492315,1.,-4.08290608095642));
#49688=CARTESIAN_POINT('Ctrl Pts',(0.7447986497065,1.,-4.09045220253573));
#49689=CARTESIAN_POINT('Ctrl Pts',(0.742761369689841,1.,-4.09799769702611));
#49690=CARTESIAN_POINT('Ctrl Pts',(0.740688998553376,1.,-4.10554241757547));
#49691=CARTESIAN_POINT('Ctrl Pts',(0.738581708225843,1.,-4.11308626951927));
#49692=CARTESIAN_POINT('Ctrl Pts',(0.736439634331344,1.,-4.120629196238));
#49693=CARTESIAN_POINT('Ctrl Pts',(0.734698226764092,1.,-4.12666277570844));
#49694=CARTESIAN_POINT('Ctrl Pts',(0.733376589323546,1.,-4.13118752795207));
#49695=CARTESIAN_POINT('Ctrl Pts',(0.732488575135159,1.,-4.1342038373684));
#49696=CARTESIAN_POINT('Ctrl Pts',(0.73204283740062,1.,-4.13571194405636));
#49697=CARTESIAN_POINT('Origin',(0.73204283740062,0.,-4.13571194405636));
#49698=CARTESIAN_POINT('',(0.581791163835815,1.,-4.15950947128175));
#49699=CARTESIAN_POINT('Origin',(0.,0.,0.));
#49700=CARTESIAN_POINT('',(0.963899035117248,1.,-3.62400312501245));
#49701=CARTESIAN_POINT('Origin',(0.,1.,0.));
#49702=CARTESIAN_POINT('Ctrl Pts',(0.963899035117248,1.,-3.62400312501246));
#49703=CARTESIAN_POINT('Ctrl Pts',(0.963899035117248,0.666666666666667,
-3.62400312501246));
#49704=CARTESIAN_POINT('Ctrl Pts',(0.963899035117248,0.333333333333333,
-3.62400312501246));
#49705=CARTESIAN_POINT('Ctrl Pts',(0.963899035117248,-0.333333333333333,
-3.62400312501246));
#49706=CARTESIAN_POINT('Ctrl Pts',(0.963899035117249,-0.666666666666667,
-3.62400312501246));
#49707=CARTESIAN_POINT('Ctrl Pts',(0.963899035117249,-1.,-3.62400312501246));
#49708=CARTESIAN_POINT('Ctrl Pts',(1.22531898815164,-1.,-4.01728681790024));
#49709=CARTESIAN_POINT('Ctrl Pts',(1.22531898815164,1.,-4.01728681790024));
#49710=CARTESIAN_POINT('Ctrl Pts',(1.22423716681447,-1.,-4.0161454457032));
#49711=CARTESIAN_POINT('Ctrl Pts',(1.22423716681447,1.,-4.0161454457032));
#49712=CARTESIAN_POINT('Ctrl Pts',(1.22207656456199,-1.,-4.01386104434674));
#49713=CARTESIAN_POINT('Ctrl Pts',(1.22207656456199,1.,-4.01386104434674));
#49714=CARTESIAN_POINT('Ctrl Pts',(1.21884478244983,-1.,-4.01042947142681));
#49715=CARTESIAN_POINT('Ctrl Pts',(1.21884478244983,1.,-4.01042947142681));
#49716=CARTESIAN_POINT('Ctrl Pts',(1.21455398918813,-1.,-4.00584409524937));
#49717=CARTESIAN_POINT('Ctrl Pts',(1.21455398918813,1.,-4.00584409524937));
#49718=CARTESIAN_POINT('Ctrl Pts',(1.20922097030107,-1.,-4.00009577952534));
#49719=CARTESIAN_POINT('Ctrl Pts',(1.20922097030107,1.,-4.00009577952534));
#49720=CARTESIAN_POINT('Ctrl Pts',(1.2039185237544,-1.,-3.99433084800649));
#49721=CARTESIAN_POINT('Ctrl Pts',(1.2039185237544,1.,-3.99433084800649));
#49722=CARTESIAN_POINT('Ctrl Pts',(1.19864679609596,-1.,-3.98854928957287));
#49723=CARTESIAN_POINT('Ctrl Pts',(1.19864679609596,1.,-3.98854928957287));
#49724=CARTESIAN_POINT('Ctrl Pts',(1.19340598349307,-1.,-3.98275111052015));
#49725=CARTESIAN_POINT('Ctrl Pts',(1.19340598349307,1.,-3.98275111052015));
#49726=CARTESIAN_POINT('Ctrl Pts',(1.18819633715285,-1.,-3.97693634766926));
#49727=CARTESIAN_POINT('Ctrl Pts',(1.18819633715285,1.,-3.97693634766926));
#49728=CARTESIAN_POINT('Ctrl Pts',(1.18301815039596,-1.,-3.9711050516465));
#49729=CARTESIAN_POINT('Ctrl Pts',(1.18301815039596,1.,-3.9711050516465));
#49730=CARTESIAN_POINT('Ctrl Pts',(1.17787174135445,-1.,-3.96525726357682));
#49731=CARTESIAN_POINT('Ctrl Pts',(1.17787174135445,1.,-3.96525726357682));
#49732=CARTESIAN_POINT('Ctrl Pts',(1.17275743590327,-1.,-3.95939299213164));
#49733=CARTESIAN_POINT('Ctrl Pts',(1.17275743590327,1.,-3.95939299213164));
#49734=CARTESIAN_POINT('Ctrl Pts',(1.16767555244495,-1.,-3.95351219510062));
#49735=CARTESIAN_POINT('Ctrl Pts',(1.16767555244495,1.,-3.95351219510062));
#49736=CARTESIAN_POINT('Ctrl Pts',(1.16262637999261,-1.,-3.9476147478092));
#49737=CARTESIAN_POINT('Ctrl Pts',(1.16262637999261,1.,-3.9476147478092));
#49738=CARTESIAN_POINT('Ctrl Pts',(1.1576101834106,-1.,-3.94170046685542));
#49739=CARTESIAN_POINT('Ctrl Pts',(1.1576101834106,1.,-3.94170046685542));
#49740=CARTESIAN_POINT('Ctrl Pts',(1.1526272271639,-1.,-3.9357691705651));
#49741=CARTESIAN_POINT('Ctrl Pts',(1.1526272271639,1.,-3.9357691705651));
#49742=CARTESIAN_POINT('Ctrl Pts',(1.14767779451147,-1.,-3.92982073294334));
#49743=CARTESIAN_POINT('Ctrl Pts',(1.14767779451147,1.,-3.92982073294334));
#49744=CARTESIAN_POINT('Ctrl Pts',(1.14276220561575,-1.,-3.92385513133937));
#49745=CARTESIAN_POINT('Ctrl Pts',(1.14276220561575,1.,-3.92385513133937));
#49746=CARTESIAN_POINT('Ctrl Pts',(1.13788084225511,-1.,-3.91787251936688));
#49747=CARTESIAN_POINT('Ctrl Pts',(1.13788084225511,1.,-3.91787251936688));
#49748=CARTESIAN_POINT('Ctrl Pts',(1.13303414693849,-1.,-3.91187321145495));
#49749=CARTESIAN_POINT('Ctrl Pts',(1.13303414693849,1.,-3.91187321145495));
#49750=CARTESIAN_POINT('Ctrl Pts',(1.12822258281518,-1.,-3.90585753318622));
#49751=CARTESIAN_POINT('Ctrl Pts',(1.12822258281518,1.,-3.90585753318622));
#49752=CARTESIAN_POINT('Ctrl Pts',(1.12344660099029,-1.,-3.89982569749978));
#49753=CARTESIAN_POINT('Ctrl Pts',(1.12344660099029,1.,-3.89982569749978));
#49754=CARTESIAN_POINT('Ctrl Pts',(1.11870660794609,-1.,-3.89377768340362));
#49755=CARTESIAN_POINT('Ctrl Pts',(1.11870660794609,1.,-3.89377768340362));
#49756=CARTESIAN_POINT('Ctrl Pts',(1.11400292434447,-1.,-3.88771308285229));
#49757=CARTESIAN_POINT('Ctrl Pts',(1.11400292434447,1.,-3.88771308285229));
#49758=CARTESIAN_POINT('Ctrl Pts',(1.10933577224029,-1.,-3.88163105531791));
#49759=CARTESIAN_POINT('Ctrl Pts',(1.10933577224029,1.,-3.88163105531791));
#49760=CARTESIAN_POINT('Ctrl Pts',(1.10470536603303,-1.,-3.87553067187566));
#49761=CARTESIAN_POINT('Ctrl Pts',(1.10470536603303,1.,-3.87553067187566));
#49762=CARTESIAN_POINT('Ctrl Pts',(1.10011198761202,-1.,-3.86941120134872));
#49763=CARTESIAN_POINT('Ctrl Pts',(1.10011198761202,1.,-3.86941120134872));
#49764=CARTESIAN_POINT('Ctrl Pts',(1.09555606505012,-1.,-3.86327241021242));
#49765=CARTESIAN_POINT('Ctrl Pts',(1.09555606505012,1.,-3.86327241021242));
#49766=CARTESIAN_POINT('Ctrl Pts',(1.09103825516288,-1.,-3.85711487933911));
#49767=CARTESIAN_POINT('Ctrl Pts',(1.09103825516288,1.,-3.85711487933911));
#49768=CARTESIAN_POINT('Ctrl Pts',(1.08655950846377,-1.,-3.85094025222691));
#49769=CARTESIAN_POINT('Ctrl Pts',(1.08655950846377,1.,-3.85094025222691));
#49770=CARTESIAN_POINT('Ctrl Pts',(1.08212087917986,-1.,-3.84475048030615));
#49771=CARTESIAN_POINT('Ctrl Pts',(1.08212087917986,1.,-3.84475048030615));
#49772=CARTESIAN_POINT('Ctrl Pts',(1.07772335353856,-1.,-3.83854714117486));
#49773=CARTESIAN_POINT('Ctrl Pts',(1.07772335353856,1.,-3.83854714117486));
#49774=CARTESIAN_POINT('Ctrl Pts',(1.0733676663346,-1.,-3.83233071195145));
#49775=CARTESIAN_POINT('Ctrl Pts',(1.0733676663346,1.,-3.83233071195145));
#49776=CARTESIAN_POINT('Ctrl Pts',(1.0690541318036,-1.,-3.82609989967278));
#49777=CARTESIAN_POINT('Ctrl Pts',(1.0690541318036,1.,-3.82609989967278));
#49778=CARTESIAN_POINT('Ctrl Pts',(1.06478244038931,-1.,-3.81985083953012));
#49779=CARTESIAN_POINT('Ctrl Pts',(1.06478244038931,1.,-3.81985083953012));
#49780=CARTESIAN_POINT('Ctrl Pts',(1.06055206187298,-1.,-3.81357866117485));
#49781=CARTESIAN_POINT('Ctrl Pts',(1.06055206187298,1.,-3.81357866117485));
#49782=CARTESIAN_POINT('Ctrl Pts',(1.05636266918643,-1.,-3.80727913637784));
#49783=CARTESIAN_POINT('Ctrl Pts',(1.05636266918643,1.,-3.80727913637784));
#49784=CARTESIAN_POINT('Ctrl Pts',(1.05221457990015,-1.,-3.80095039790678));
#49785=CARTESIAN_POINT('Ctrl Pts',(1.05221457990015,1.,-3.80095039790678));
#49786=CARTESIAN_POINT('Ctrl Pts',(1.04810913267641,-1.,-3.79459440308793));
#49787=CARTESIAN_POINT('Ctrl Pts',(1.04810913267641,1.,-3.79459440308793));
#49788=CARTESIAN_POINT('Ctrl Pts',(1.04404924374426,-1.,-3.78821910787195));
#49789=CARTESIAN_POINT('Ctrl Pts',(1.04404924374426,1.,-3.78821910787195));
#49790=CARTESIAN_POINT('Ctrl Pts',(1.04003862055804,-1.,-3.78183535008192));
#49791=CARTESIAN_POINT('Ctrl Pts',(1.04003862055804,1.,-3.78183535008192));
#49792=CARTESIAN_POINT('Ctrl Pts',(1.03608074678013,-1.,-3.77545283140445));
#49793=CARTESIAN_POINT('Ctrl Pts',(1.03608074678013,1.,-3.77545283140445));
#49794=CARTESIAN_POINT('Ctrl Pts',(1.0321778660492,-1.,-3.76907609832522));
#49795=CARTESIAN_POINT('Ctrl Pts',(1.0321778660492,1.,-3.76907609832522));
#49796=CARTESIAN_POINT('Ctrl Pts',(1.02833014458181,-1.,-3.76270122291232));
#49797=CARTESIAN_POINT('Ctrl Pts',(1.02833014458181,1.,-3.76270122291232));
#49798=CARTESIAN_POINT('Ctrl Pts',(1.0245342944466,-1.,-3.75631037456194));
#49799=CARTESIAN_POINT('Ctrl Pts',(1.0245342944466,1.,-3.75631037456194));
#49800=CARTESIAN_POINT('Ctrl Pts',(1.02078510487428,-1.,-3.74987777155834));
#49801=CARTESIAN_POINT('Ctrl Pts',(1.02078510487428,1.,-3.74987777155834));
#49802=CARTESIAN_POINT('Ctrl Pts',(1.01707794311079,-1.,-3.74337942504959));
#49803=CARTESIAN_POINT('Ctrl Pts',(1.01707794311079,1.,-3.74337942504959));
#49804=CARTESIAN_POINT('Ctrl Pts',(1.01341114319903,-1.,-3.73680245055734));
#49805=CARTESIAN_POINT('Ctrl Pts',(1.01341114319903,1.,-3.73680245055734));
#49806=CARTESIAN_POINT('Ctrl Pts',(1.00978798539496,-1.,-3.73015276704426));
#49807=CARTESIAN_POINT('Ctrl Pts',(1.00978798539496,1.,-3.73015276704426));
#49808=CARTESIAN_POINT('Ctrl Pts',(1.0062200073571,-1.,-3.72346803750596));
#49809=CARTESIAN_POINT('Ctrl Pts',(1.0062200073571,1.,-3.72346803750596));
#49810=CARTESIAN_POINT('Ctrl Pts',(1.00272423396822,-1.,-3.71680667125119));
#49811=CARTESIAN_POINT('Ctrl Pts',(1.00272423396822,1.,-3.71680667125119));
#49812=CARTESIAN_POINT('Ctrl Pts',(0.99931726075653,-1.,-3.71022439713938));
#49813=CARTESIAN_POINT('Ctrl Pts',(0.99931726075653,1.,-3.71022439713938));
#49814=CARTESIAN_POINT('Ctrl Pts',(0.996009819772518,-1.,-3.70375282282138));
#49815=CARTESIAN_POINT('Ctrl Pts',(0.996009819772518,1.,-3.70375282282138));
#49816=CARTESIAN_POINT('Ctrl Pts',(0.99280221833201,-1.,-3.69738123415662));
#49817=CARTESIAN_POINT('Ctrl Pts',(0.99280221833201,1.,-3.69738123415662));
#49818=CARTESIAN_POINT('Ctrl Pts',(0.989676715398558,-1.,-3.69102682138847));
#49819=CARTESIAN_POINT('Ctrl Pts',(0.989676715398558,1.,-3.69102682138847));
#49820=CARTESIAN_POINT('Ctrl Pts',(0.986602639863837,-1.,-3.68455317926068));
#49821=CARTESIAN_POINT('Ctrl Pts',(0.986602639863837,1.,-3.68455317926068));
#49822=CARTESIAN_POINT('Ctrl Pts',(0.983550791470419,-1.,-3.67782408841715));
#49823=CARTESIAN_POINT('Ctrl Pts',(0.983550791470419,1.,-3.67782408841715));
#49824=CARTESIAN_POINT('Ctrl Pts',(0.980505922458267,-1.,-3.67074983340361));
#49825=CARTESIAN_POINT('Ctrl Pts',(0.980505922458267,1.,-3.67074983340361));
#49826=CARTESIAN_POINT('Ctrl Pts',(0.977478312751618,-1.,-3.66333049637475));
#49827=CARTESIAN_POINT('Ctrl Pts',(0.977478312751618,1.,-3.66333049637475));
#49828=CARTESIAN_POINT('Ctrl Pts',(0.974519971354848,-1.,-3.65571576735126));
#49829=CARTESIAN_POINT('Ctrl Pts',(0.974519971354848,1.,-3.65571576735126));
#49830=CARTESIAN_POINT('Ctrl Pts',(0.971722122061341,-1.,-3.64819756447455));
#49831=CARTESIAN_POINT('Ctrl Pts',(0.971722122061341,1.,-3.64819756447455));
#49832=CARTESIAN_POINT('Ctrl Pts',(0.969195124675865,-1.,-3.64113946505766));
#49833=CARTESIAN_POINT('Ctrl Pts',(0.969195124675865,1.,-3.64113946505766));
#49834=CARTESIAN_POINT('Ctrl Pts',(0.967052554541385,-1.,-3.63492122081143));
#49835=CARTESIAN_POINT('Ctrl Pts',(0.967052554541385,1.,-3.63492122081143));
#49836=CARTESIAN_POINT('Ctrl Pts',(0.965395153165293,-1.,-3.62988252139846));
#49837=CARTESIAN_POINT('Ctrl Pts',(0.965395153165293,1.,-3.62988252139846));
#49838=CARTESIAN_POINT('Ctrl Pts',(0.964291001273287,-1.,-3.62625391254797));
#49839=CARTESIAN_POINT('Ctrl Pts',(0.964291001273287,1.,-3.62625391254797));
#49840=CARTESIAN_POINT('Ctrl Pts',(0.963875774530619,-1.,-3.6245656860652));
#49841=CARTESIAN_POINT('Ctrl Pts',(0.963875774530619,1.,-3.6245656860652));
#49842=CARTESIAN_POINT('Ctrl Pts',(0.963832486395051,-1.,-3.62399933639915));
#49843=CARTESIAN_POINT('Ctrl Pts',(0.963832486395051,1.,-3.62399933639915));
#49844=CARTESIAN_POINT('Ctrl Pts',(0.963922720982193,-1.,-3.62393257642052));
#49845=CARTESIAN_POINT('Ctrl Pts',(0.963922720982193,1.,-3.62393257642052));
#49846=CARTESIAN_POINT('Ctrl Pts',(0.963997613369571,-1.,-3.62397690409552));
#49847=CARTESIAN_POINT('Ctrl Pts',(0.963997613369571,1.,-3.62397690409552));
#49848=CARTESIAN_POINT('',(1.22531898815164,1.,-4.01728681790024));
#49849=CARTESIAN_POINT('Ctrl Pts',(1.22531898815164,1.,-4.01728681790024));
#49850=CARTESIAN_POINT('Ctrl Pts',(1.22423716681447,1.,-4.0161454457032));
#49851=CARTESIAN_POINT('Ctrl Pts',(1.22207656456199,1.,-4.01386104434674));
#49852=CARTESIAN_POINT('Ctrl Pts',(1.21884478244983,1.,-4.01042947142681));
#49853=CARTESIAN_POINT('Ctrl Pts',(1.21455398918813,1.,-4.00584409524937));
#49854=CARTESIAN_POINT('Ctrl Pts',(1.20922097030107,1.,-4.00009577952534));
#49855=CARTESIAN_POINT('Ctrl Pts',(1.2039185237544,1.,-3.99433084800649));
#49856=CARTESIAN_POINT('Ctrl Pts',(1.19864679609596,1.,-3.98854928957287));
#49857=CARTESIAN_POINT('Ctrl Pts',(1.19340598349307,1.,-3.98275111052015));
#49858=CARTESIAN_POINT('Ctrl Pts',(1.18819633715285,1.,-3.97693634766926));
#49859=CARTESIAN_POINT('Ctrl Pts',(1.18301815039596,1.,-3.9711050516465));
#49860=CARTESIAN_POINT('Ctrl Pts',(1.17787174135445,1.,-3.96525726357682));
#49861=CARTESIAN_POINT('Ctrl Pts',(1.17275743590327,1.,-3.95939299213164));
#49862=CARTESIAN_POINT('Ctrl Pts',(1.16767555244495,1.,-3.95351219510062));
#49863=CARTESIAN_POINT('Ctrl Pts',(1.16262637999261,1.,-3.9476147478092));
#49864=CARTESIAN_POINT('Ctrl Pts',(1.1576101834106,1.,-3.94170046685542));
#49865=CARTESIAN_POINT('Ctrl Pts',(1.1526272271639,1.,-3.9357691705651));
#49866=CARTESIAN_POINT('Ctrl Pts',(1.14767779451147,1.,-3.92982073294334));
#49867=CARTESIAN_POINT('Ctrl Pts',(1.14276220561575,1.,-3.92385513133937));
#49868=CARTESIAN_POINT('Ctrl Pts',(1.13788084225511,1.,-3.91787251936688));
#49869=CARTESIAN_POINT('Ctrl Pts',(1.13303414693849,1.,-3.91187321145495));
#49870=CARTESIAN_POINT('Ctrl Pts',(1.12822258281518,1.,-3.90585753318622));
#49871=CARTESIAN_POINT('Ctrl Pts',(1.12344660099029,1.,-3.89982569749978));
#49872=CARTESIAN_POINT('Ctrl Pts',(1.11870660794609,1.,-3.89377768340362));
#49873=CARTESIAN_POINT('Ctrl Pts',(1.11400292434447,1.,-3.88771308285229));
#49874=CARTESIAN_POINT('Ctrl Pts',(1.10933577224029,1.,-3.88163105531791));
#49875=CARTESIAN_POINT('Ctrl Pts',(1.10470536603303,1.,-3.87553067187566));
#49876=CARTESIAN_POINT('Ctrl Pts',(1.10011198761202,1.,-3.86941120134872));
#49877=CARTESIAN_POINT('Ctrl Pts',(1.09555606505012,1.,-3.86327241021242));
#49878=CARTESIAN_POINT('Ctrl Pts',(1.09103825516288,1.,-3.85711487933911));
#49879=CARTESIAN_POINT('Ctrl Pts',(1.08655950846377,1.,-3.85094025222691));
#49880=CARTESIAN_POINT('Ctrl Pts',(1.08212087917986,1.,-3.84475048030615));
#49881=CARTESIAN_POINT('Ctrl Pts',(1.07772335353856,1.,-3.83854714117486));
#49882=CARTESIAN_POINT('Ctrl Pts',(1.0733676663346,1.,-3.83233071195145));
#49883=CARTESIAN_POINT('Ctrl Pts',(1.0690541318036,1.,-3.82609989967278));
#49884=CARTESIAN_POINT('Ctrl Pts',(1.06478244038931,1.,-3.81985083953012));
#49885=CARTESIAN_POINT('Ctrl Pts',(1.06055206187298,1.,-3.81357866117485));
#49886=CARTESIAN_POINT('Ctrl Pts',(1.05636266918643,1.,-3.80727913637784));
#49887=CARTESIAN_POINT('Ctrl Pts',(1.05221457990015,1.,-3.80095039790678));
#49888=CARTESIAN_POINT('Ctrl Pts',(1.04810913267641,1.,-3.79459440308793));
#49889=CARTESIAN_POINT('Ctrl Pts',(1.04404924374426,1.,-3.78821910787195));
#49890=CARTESIAN_POINT('Ctrl Pts',(1.04003862055804,1.,-3.78183535008192));
#49891=CARTESIAN_POINT('Ctrl Pts',(1.03608074678013,1.,-3.77545283140445));
#49892=CARTESIAN_POINT('Ctrl Pts',(1.0321778660492,1.,-3.76907609832522));
#49893=CARTESIAN_POINT('Ctrl Pts',(1.02833014458181,1.,-3.76270122291232));
#49894=CARTESIAN_POINT('Ctrl Pts',(1.0245342944466,1.,-3.75631037456194));
#49895=CARTESIAN_POINT('Ctrl Pts',(1.02078510487428,1.,-3.74987777155834));
#49896=CARTESIAN_POINT('Ctrl Pts',(1.01707794311079,1.,-3.74337942504959));
#49897=CARTESIAN_POINT('Ctrl Pts',(1.01341114319903,1.,-3.73680245055734));
#49898=CARTESIAN_POINT('Ctrl Pts',(1.00978798539496,1.,-3.73015276704426));
#49899=CARTESIAN_POINT('Ctrl Pts',(1.0062200073571,1.,-3.72346803750596));
#49900=CARTESIAN_POINT('Ctrl Pts',(1.00272423396822,1.,-3.71680667125119));
#49901=CARTESIAN_POINT('Ctrl Pts',(0.99931726075653,1.,-3.71022439713938));
#49902=CARTESIAN_POINT('Ctrl Pts',(0.996009819772518,1.,-3.70375282282138));
#49903=CARTESIAN_POINT('Ctrl Pts',(0.99280221833201,1.,-3.69738123415662));
#49904=CARTESIAN_POINT('Ctrl Pts',(0.989676715398558,1.,-3.69102682138847));
#49905=CARTESIAN_POINT('Ctrl Pts',(0.986602639863837,1.,-3.68455317926068));
#49906=CARTESIAN_POINT('Ctrl Pts',(0.983550791470419,1.,-3.67782408841715));
#49907=CARTESIAN_POINT('Ctrl Pts',(0.980505922458267,1.,-3.67074983340361));
#49908=CARTESIAN_POINT('Ctrl Pts',(0.977478312751618,1.,-3.66333049637475));
#49909=CARTESIAN_POINT('Ctrl Pts',(0.974519971354848,1.,-3.65571576735126));
#49910=CARTESIAN_POINT('Ctrl Pts',(0.971722122061341,1.,-3.64819756447455));
#49911=CARTESIAN_POINT('Ctrl Pts',(0.969195124675865,1.,-3.64113946505766));
#49912=CARTESIAN_POINT('Ctrl Pts',(0.967052554541385,1.,-3.63492122081143));
#49913=CARTESIAN_POINT('Ctrl Pts',(0.965395153165293,1.,-3.62988252139846));
#49914=CARTESIAN_POINT('Ctrl Pts',(0.964373850166457,1.,-3.62652618145335));
#49915=CARTESIAN_POINT('Ctrl Pts',(0.963957782642843,1.,-3.62489305727662));
#49916=CARTESIAN_POINT('Ctrl Pts',(0.963861297423241,1.,-3.62424461507588));
#49917=CARTESIAN_POINT('Ctrl Pts',(0.963880158555582,1.,-3.6240482887845));
#49918=CARTESIAN_POINT('Ctrl Pts',(0.963899035117249,1.,-3.62400312501246));
#49919=CARTESIAN_POINT('',(1.22531898815164,0.,-4.01728681790024));
#49920=CARTESIAN_POINT('Ctrl Pts',(1.35022972712301,-1.,-3.49848248301936));
#49921=CARTESIAN_POINT('Ctrl Pts',(1.35022972712301,1.,-3.49848248301936));
#49922=CARTESIAN_POINT('Ctrl Pts',(1.35026426118402,-1.,-3.4984026005375));
#49923=CARTESIAN_POINT('Ctrl Pts',(1.35026426118402,1.,-3.4984026005375));
#49924=CARTESIAN_POINT('Ctrl Pts',(1.35037650303019,-1.,-3.49840357193736));
#49925=CARTESIAN_POINT('Ctrl Pts',(1.35037650303019,1.,-3.49840357193736));
#49926=CARTESIAN_POINT('Ctrl Pts',(1.35067437417483,-1.,-3.49888720257132));
#49927=CARTESIAN_POINT('Ctrl Pts',(1.35067437417483,1.,-3.49888720257132));
#49928=CARTESIAN_POINT('Ctrl Pts',(1.3513307633124,-1.,-3.5004970706414));
#49929=CARTESIAN_POINT('Ctrl Pts',(1.3513307633124,1.,-3.5004970706414));
#49930=CARTESIAN_POINT('Ctrl Pts',(1.35257032843486,-1.,-3.50408168106261));
#49931=CARTESIAN_POINT('Ctrl Pts',(1.35257032843486,1.,-3.50408168106261));
#49932=CARTESIAN_POINT('Ctrl Pts',(1.35419113575956,-1.,-3.50913227059999));
#49933=CARTESIAN_POINT('Ctrl Pts',(1.35419113575956,1.,-3.50913227059999));
#49934=CARTESIAN_POINT('Ctrl Pts',(1.35611275237152,-1.,-3.51542230699556));
#49935=CARTESIAN_POINT('Ctrl Pts',(1.35611275237152,1.,-3.51542230699556));
#49936=CARTESIAN_POINT('Ctrl Pts',(1.35821701528836,-1.,-3.52261776116748));
#49937=CARTESIAN_POINT('Ctrl Pts',(1.35821701528836,1.,-3.52261776116748));
#49938=CARTESIAN_POINT('Ctrl Pts',(1.36037259643734,-1.,-3.530344649616));
#49939=CARTESIAN_POINT('Ctrl Pts',(1.36037259643734,1.,-3.530344649616));
#49940=CARTESIAN_POINT('Ctrl Pts',(1.36245507339307,-1.,-3.53824396424961));
#49941=CARTESIAN_POINT('Ctrl Pts',(1.36245507339307,1.,-3.53824396424961));
#49942=CARTESIAN_POINT('Ctrl Pts',(1.36436666257597,-1.,-3.54602591832973));
#49943=CARTESIAN_POINT('Ctrl Pts',(1.36436666257597,1.,-3.54602591832973));
#49944=CARTESIAN_POINT('Ctrl Pts',(1.3660614545677,-1.,-3.55353883995949));
#49945=CARTESIAN_POINT('Ctrl Pts',(1.3660614545677,1.,-3.55353883995949));
#49946=CARTESIAN_POINT('Ctrl Pts',(1.36754771771233,-1.,-3.56077662028649));
#49947=CARTESIAN_POINT('Ctrl Pts',(1.36754771771233,1.,-3.56077662028649));
#49948=CARTESIAN_POINT('Ctrl Pts',(1.36886584973389,-1.,-3.5678208030466));
#49949=CARTESIAN_POINT('Ctrl Pts',(1.36886584973389,1.,-3.5678208030466));
#49950=CARTESIAN_POINT('Ctrl Pts',(1.37007229485659,-1.,-3.57479875549486));
#49951=CARTESIAN_POINT('Ctrl Pts',(1.37007229485659,1.,-3.57479875549486));
#49952=CARTESIAN_POINT('Ctrl Pts',(1.37122241663062,-1.,-3.58183885982715));
#49953=CARTESIAN_POINT('Ctrl Pts',(1.37122241663062,1.,-3.58183885982715));
#49954=CARTESIAN_POINT('Ctrl Pts',(1.37235053660976,-1.,-3.58901853846365));
#49955=CARTESIAN_POINT('Ctrl Pts',(1.37235053660976,1.,-3.58901853846365));
#49956=CARTESIAN_POINT('Ctrl Pts',(1.37346320103157,-1.,-3.59634627869048));
#49957=CARTESIAN_POINT('Ctrl Pts',(1.37346320103157,1.,-3.59634627869048));
#49958=CARTESIAN_POINT('Ctrl Pts',(1.37455051379623,-1.,-3.60379020123988));
#49959=CARTESIAN_POINT('Ctrl Pts',(1.37455051379623,1.,-3.60379020123988));
#49960=CARTESIAN_POINT('Ctrl Pts',(1.37559314436634,-1.,-3.61129546591064));
#49961=CARTESIAN_POINT('Ctrl Pts',(1.37559314436634,1.,-3.61129546591064));
#49962=CARTESIAN_POINT('Ctrl Pts',(1.37657053403107,-1.,-3.61880481160421));
#49963=CARTESIAN_POINT('Ctrl Pts',(1.37657053403107,1.,-3.61880481160421));
#49964=CARTESIAN_POINT('Ctrl Pts',(1.37746987919881,-1.,-3.62628098665145));
#49965=CARTESIAN_POINT('Ctrl Pts',(1.37746987919881,1.,-3.62628098665145));
#49966=CARTESIAN_POINT('Ctrl Pts',(1.37829035457339,-1.,-3.63371727442486));
#49967=CARTESIAN_POINT('Ctrl Pts',(1.37829035457339,1.,-3.63371727442486));
#49968=CARTESIAN_POINT('Ctrl Pts',(1.37903818567359,-1.,-3.64112507791141));
#49969=CARTESIAN_POINT('Ctrl Pts',(1.37903818567359,1.,-3.64112507791141));
#49970=CARTESIAN_POINT('Ctrl Pts',(1.37972372481603,-1.,-3.64852652756456));
#49971=CARTESIAN_POINT('Ctrl Pts',(1.37972372481603,1.,-3.64852652756456));
#49972=CARTESIAN_POINT('Ctrl Pts',(1.38035791051212,-1.,-3.6559455440439));
#49973=CARTESIAN_POINT('Ctrl Pts',(1.38035791051212,1.,-3.6559455440439));
#49974=CARTESIAN_POINT('Ctrl Pts',(1.38094856333552,-1.,-3.66339848520857));
#49975=CARTESIAN_POINT('Ctrl Pts',(1.38094856333552,1.,-3.66339848520857));
#49976=CARTESIAN_POINT('Ctrl Pts',(1.38149812653868,-1.,-3.67088843112262));
#49977=CARTESIAN_POINT('Ctrl Pts',(1.38149812653868,1.,-3.67088843112262));
#49978=CARTESIAN_POINT('Ctrl Pts',(1.3820057429062,-1.,-3.67841038482414));
#49979=CARTESIAN_POINT('Ctrl Pts',(1.3820057429062,1.,-3.67841038482414));
#49980=CARTESIAN_POINT('Ctrl Pts',(1.38246852827182,-1.,-3.68595444983838));
#49981=CARTESIAN_POINT('Ctrl Pts',(1.38246852827182,1.,-3.68595444983838));
#49982=CARTESIAN_POINT('Ctrl Pts',(1.3828831117165,-1.,-3.69350967899526));
#49983=CARTESIAN_POINT('Ctrl Pts',(1.3828831117165,1.,-3.69350967899526));
#49984=CARTESIAN_POINT('Ctrl Pts',(1.38324717612865,-1.,-3.701067921679));
#49985=CARTESIAN_POINT('Ctrl Pts',(1.38324717612865,1.,-3.701067921679));
#49986=CARTESIAN_POINT('Ctrl Pts',(1.38356065402124,-1.,-3.70862680753347));
#49987=CARTESIAN_POINT('Ctrl Pts',(1.38356065402124,1.,-3.70862680753347));
#49988=CARTESIAN_POINT('Ctrl Pts',(1.38382489984586,-1.,-3.7161876605181));
#49989=CARTESIAN_POINT('Ctrl Pts',(1.38382489984586,1.,-3.7161876605181));
#49990=CARTESIAN_POINT('Ctrl Pts',(1.3840421342895,-1.,-3.72375409358803));
#49991=CARTESIAN_POINT('Ctrl Pts',(1.3840421342895,1.,-3.72375409358803));
#49992=CARTESIAN_POINT('Ctrl Pts',(1.38421479111531,-1.,-3.73133035859282));
#49993=CARTESIAN_POINT('Ctrl Pts',(1.38421479111531,1.,-3.73133035859282));
#49994=CARTESIAN_POINT('Ctrl Pts',(1.38434489156458,-1.,-3.73891976418104));
#49995=CARTESIAN_POINT('Ctrl Pts',(1.38434489156458,1.,-3.73891976418104));
#49996=CARTESIAN_POINT('Ctrl Pts',(1.38443344984394,-1.,-3.74652317167876));
#49997=CARTESIAN_POINT('Ctrl Pts',(1.38443344984394,1.,-3.74652317167876));
#49998=CARTESIAN_POINT('Ctrl Pts',(1.38448077997163,-1.,-3.7541397631875));
#49999=CARTESIAN_POINT('Ctrl Pts',(1.38448077997163,1.,-3.7541397631875));
#50000=CARTESIAN_POINT('Ctrl Pts',(1.3844867525335,-1.,-3.76176768271367));
#50001=CARTESIAN_POINT('Ctrl Pts',(1.3844867525335,1.,-3.76176768271367));
#50002=CARTESIAN_POINT('Ctrl Pts',(1.38445107339518,-1.,-3.76940473185779));
#50003=CARTESIAN_POINT('Ctrl Pts',(1.38445107339518,1.,-3.76940473185779));
#50004=CARTESIAN_POINT('Ctrl Pts',(1.38437354551428,-1.,-3.77704902230418));
#50005=CARTESIAN_POINT('Ctrl Pts',(1.38437354551428,1.,-3.77704902230418));
#50006=CARTESIAN_POINT('Ctrl Pts',(1.38425435883756,-1.,-3.78469969805082));
#50007=CARTESIAN_POINT('Ctrl Pts',(1.38425435883756,1.,-3.78469969805082));
#50008=CARTESIAN_POINT('Ctrl Pts',(1.38409399694566,-1.,-3.79235669640841));
#50009=CARTESIAN_POINT('Ctrl Pts',(1.38409399694566,1.,-3.79235669640841));
#50010=CARTESIAN_POINT('Ctrl Pts',(1.38389311766682,-1.,-3.80002044322111));
#50011=CARTESIAN_POINT('Ctrl Pts',(1.38389311766682,1.,-3.80002044322111));
#50012=CARTESIAN_POINT('Ctrl Pts',(1.3836524404622,-1.,-3.80769156398411));
#50013=CARTESIAN_POINT('Ctrl Pts',(1.3836524404622,1.,-3.80769156398411));
#50014=CARTESIAN_POINT('Ctrl Pts',(1.38337263902782,-1.,-3.81537060817811));
#50015=CARTESIAN_POINT('Ctrl Pts',(1.38337263902782,1.,-3.81537060817811));
#50016=CARTESIAN_POINT('Ctrl Pts',(1.38305421262763,-1.,-3.82305771743829));
#50017=CARTESIAN_POINT('Ctrl Pts',(1.38305421262763,1.,-3.82305771743829));
#50018=CARTESIAN_POINT('Ctrl Pts',(1.38269750245138,-1.,-3.8307526698229));
#50019=CARTESIAN_POINT('Ctrl Pts',(1.38269750245138,1.,-3.8307526698229));
#50020=CARTESIAN_POINT('Ctrl Pts',(1.38230274828821,-1.,-3.83845502790746));
#50021=CARTESIAN_POINT('Ctrl Pts',(1.38230274828821,1.,-3.83845502790746));
#50022=CARTESIAN_POINT('Ctrl Pts',(1.38187013346109,-1.,-3.84616425605764));
#50023=CARTESIAN_POINT('Ctrl Pts',(1.38187013346109,1.,-3.84616425605764));
#50024=CARTESIAN_POINT('Ctrl Pts',(1.38139983115049,-1.,-3.85387983979481));
#50025=CARTESIAN_POINT('Ctrl Pts',(1.38139983115049,1.,-3.85387983979481));
#50026=CARTESIAN_POINT('Ctrl Pts',(1.38089205992989,-1.,-3.86160143043959));
#50027=CARTESIAN_POINT('Ctrl Pts',(1.38089205992989,1.,-3.86160143043959));
#50028=CARTESIAN_POINT('Ctrl Pts',(1.38034709213014,-1.,-3.86932885813068));
#50029=CARTESIAN_POINT('Ctrl Pts',(1.38034709213014,1.,-3.86932885813068));
#50030=CARTESIAN_POINT('Ctrl Pts',(1.37976523097073,-1.,-3.87706205830532));
#50031=CARTESIAN_POINT('Ctrl Pts',(1.37976523097073,1.,-3.87706205830532));
#50032=CARTESIAN_POINT('Ctrl Pts',(1.37914679719383,-1.,-3.88480102249278));
#50033=CARTESIAN_POINT('Ctrl Pts',(1.37914679719383,1.,-3.88480102249278));
#50034=CARTESIAN_POINT('Ctrl Pts',(1.3784921128802,-1.,-3.89254574338496));
#50035=CARTESIAN_POINT('Ctrl Pts',(1.3784921128802,1.,-3.89254574338496));
#50036=CARTESIAN_POINT('Ctrl Pts',(1.37780148512792,-1.,-3.90029615196727));
#50037=CARTESIAN_POINT('Ctrl Pts',(1.37780148512792,1.,-3.90029615196727));
#50038=CARTESIAN_POINT('Ctrl Pts',(1.3770751963402,-1.,-3.90805209523486));
#50039=CARTESIAN_POINT('Ctrl Pts',(1.3770751963402,1.,-3.90805209523486));
#50040=CARTESIAN_POINT('Ctrl Pts',(1.37631350505797,-1.,-3.91581337462644));
#50041=CARTESIAN_POINT('Ctrl Pts',(1.37631350505797,1.,-3.91581337462644));
#50042=CARTESIAN_POINT('Ctrl Pts',(1.37551664448242,-1.,-3.92357976987672));
#50043=CARTESIAN_POINT('Ctrl Pts',(1.37551664448242,1.,-3.92357976987672));
#50044=CARTESIAN_POINT('Ctrl Pts',(1.37468482215751,-1.,-3.93135106761844));
#50045=CARTESIAN_POINT('Ctrl Pts',(1.37468482215751,1.,-3.93135106761844));
#50046=CARTESIAN_POINT('Ctrl Pts',(1.37381821967165,-1.,-3.93912709040818));
#50047=CARTESIAN_POINT('Ctrl Pts',(1.37381821967165,1.,-3.93912709040818));
#50048=CARTESIAN_POINT('Ctrl Pts',(1.37291699202807,-1.,-3.94690771785133));
#50049=CARTESIAN_POINT('Ctrl Pts',(1.37291699202807,1.,-3.94690771785133));
#50050=CARTESIAN_POINT('Ctrl Pts',(1.37198126432386,-1.,-3.95469287280914));
#50051=CARTESIAN_POINT('Ctrl Pts',(1.37198126432386,1.,-3.95469287280914));
#50052=CARTESIAN_POINT('Ctrl Pts',(1.3712051561502,-1.,-3.96092458506535));
#50053=CARTESIAN_POINT('Ctrl Pts',(1.3712051561502,1.,-3.96092458506535));
#50054=CARTESIAN_POINT('Ctrl Pts',(1.37060761745635,-1.,-3.96560037974645));
#50055=CARTESIAN_POINT('Ctrl Pts',(1.37060761745635,1.,-3.96560037974645));
#50056=CARTESIAN_POINT('Ctrl Pts',(1.37020239094614,-1.,-3.9687184694131));
#50057=CARTESIAN_POINT('Ctrl Pts',(1.37020239094614,1.,-3.9687184694131));
#50058=CARTESIAN_POINT('Ctrl Pts',(1.36999806084572,-1.,-3.97027773754922));
#50059=CARTESIAN_POINT('Ctrl Pts',(1.36999806084572,1.,-3.97027773754922));
#50060=CARTESIAN_POINT('',(1.35032489087101,1.,-3.4984457533445));
#50061=CARTESIAN_POINT('Ctrl Pts',(1.35032489087101,-1.,-3.4984457533445));
#50062=CARTESIAN_POINT('Ctrl Pts',(1.35032489087101,-0.666666666666667,
-3.4984457533445));
#50063=CARTESIAN_POINT('Ctrl Pts',(1.35032489087101,-0.333333333333333,
-3.4984457533445));
#50064=CARTESIAN_POINT('Ctrl Pts',(1.35032489087101,0.333333333333333,-3.4984457533445));
#50065=CARTESIAN_POINT('Ctrl Pts',(1.35032489087101,0.666666666666667,-3.4984457533445));
#50066=CARTESIAN_POINT('Ctrl Pts',(1.35032489087101,1.,-3.4984457533445));
#50067=CARTESIAN_POINT('',(1.36999806084572,1.,-3.97027773754922));
#50068=CARTESIAN_POINT('',(1.36999806084572,0.,-3.97027773754922));
#50069=CARTESIAN_POINT('Ctrl Pts',(1.35032489087101,1.,-3.49844575334451));
#50070=CARTESIAN_POINT('Ctrl Pts',(1.35036670892966,1.,-3.49847119623846));
#50071=CARTESIAN_POINT('Ctrl Pts',(1.35049736560527,1.,-3.49861894124827));
#50072=CARTESIAN_POINT('Ctrl Pts',(1.35080045218587,1.,-3.49920025459723));
#50073=CARTESIAN_POINT('Ctrl Pts',(1.35142377279517,1.,-3.50076603816491));
#50074=CARTESIAN_POINT('Ctrl Pts',(1.35257032843486,1.,-3.50408168106261));
#50075=CARTESIAN_POINT('Ctrl Pts',(1.35419113575956,1.,-3.50913227059999));
#50076=CARTESIAN_POINT('Ctrl Pts',(1.35611275237152,1.,-3.51542230699556));
#50077=CARTESIAN_POINT('Ctrl Pts',(1.35821701528836,1.,-3.52261776116748));
#50078=CARTESIAN_POINT('Ctrl Pts',(1.36037259643734,1.,-3.530344649616));
#50079=CARTESIAN_POINT('Ctrl Pts',(1.36245507339307,1.,-3.53824396424961));
#50080=CARTESIAN_POINT('Ctrl Pts',(1.36436666257597,1.,-3.54602591832973));
#50081=CARTESIAN_POINT('Ctrl Pts',(1.3660614545677,1.,-3.55353883995949));
#50082=CARTESIAN_POINT('Ctrl Pts',(1.36754771771233,1.,-3.56077662028649));
#50083=CARTESIAN_POINT('Ctrl Pts',(1.36886584973389,1.,-3.5678208030466));
#50084=CARTESIAN_POINT('Ctrl Pts',(1.37007229485659,1.,-3.57479875549486));
#50085=CARTESIAN_POINT('Ctrl Pts',(1.37122241663062,1.,-3.58183885982715));
#50086=CARTESIAN_POINT('Ctrl Pts',(1.37235053660976,1.,-3.58901853846365));
#50087=CARTESIAN_POINT('Ctrl Pts',(1.37346320103157,1.,-3.59634627869048));
#50088=CARTESIAN_POINT('Ctrl Pts',(1.37455051379623,1.,-3.60379020123988));
#50089=CARTESIAN_POINT('Ctrl Pts',(1.37559314436634,1.,-3.61129546591064));
#50090=CARTESIAN_POINT('Ctrl Pts',(1.37657053403107,1.,-3.61880481160421));
#50091=CARTESIAN_POINT('Ctrl Pts',(1.37746987919881,1.,-3.62628098665145));
#50092=CARTESIAN_POINT('Ctrl Pts',(1.37829035457339,1.,-3.63371727442486));
#50093=CARTESIAN_POINT('Ctrl Pts',(1.37903818567359,1.,-3.64112507791141));
#50094=CARTESIAN_POINT('Ctrl Pts',(1.37972372481603,1.,-3.64852652756456));
#50095=CARTESIAN_POINT('Ctrl Pts',(1.38035791051212,1.,-3.6559455440439));
#50096=CARTESIAN_POINT('Ctrl Pts',(1.38094856333552,1.,-3.66339848520857));
#50097=CARTESIAN_POINT('Ctrl Pts',(1.38149812653868,1.,-3.67088843112262));
#50098=CARTESIAN_POINT('Ctrl Pts',(1.3820057429062,1.,-3.67841038482414));
#50099=CARTESIAN_POINT('Ctrl Pts',(1.38246852827182,1.,-3.68595444983838));
#50100=CARTESIAN_POINT('Ctrl Pts',(1.3828831117165,1.,-3.69350967899526));
#50101=CARTESIAN_POINT('Ctrl Pts',(1.38324717612865,1.,-3.701067921679));
#50102=CARTESIAN_POINT('Ctrl Pts',(1.38356065402124,1.,-3.70862680753347));
#50103=CARTESIAN_POINT('Ctrl Pts',(1.38382489984586,1.,-3.7161876605181));
#50104=CARTESIAN_POINT('Ctrl Pts',(1.3840421342895,1.,-3.72375409358803));
#50105=CARTESIAN_POINT('Ctrl Pts',(1.38421479111531,1.,-3.73133035859282));
#50106=CARTESIAN_POINT('Ctrl Pts',(1.38434489156458,1.,-3.73891976418104));
#50107=CARTESIAN_POINT('Ctrl Pts',(1.38443344984394,1.,-3.74652317167876));
#50108=CARTESIAN_POINT('Ctrl Pts',(1.38448077997163,1.,-3.7541397631875));
#50109=CARTESIAN_POINT('Ctrl Pts',(1.3844867525335,1.,-3.76176768271367));
#50110=CARTESIAN_POINT('Ctrl Pts',(1.38445107339518,1.,-3.76940473185779));
#50111=CARTESIAN_POINT('Ctrl Pts',(1.38437354551428,1.,-3.77704902230418));
#50112=CARTESIAN_POINT('Ctrl Pts',(1.38425435883756,1.,-3.78469969805082));
#50113=CARTESIAN_POINT('Ctrl Pts',(1.38409399694566,1.,-3.79235669640841));
#50114=CARTESIAN_POINT('Ctrl Pts',(1.38389311766682,1.,-3.80002044322111));
#50115=CARTESIAN_POINT('Ctrl Pts',(1.3836524404622,1.,-3.80769156398411));
#50116=CARTESIAN_POINT('Ctrl Pts',(1.38337263902782,1.,-3.81537060817811));
#50117=CARTESIAN_POINT('Ctrl Pts',(1.38305421262763,1.,-3.82305771743829));
#50118=CARTESIAN_POINT('Ctrl Pts',(1.38269750245138,1.,-3.8307526698229));
#50119=CARTESIAN_POINT('Ctrl Pts',(1.38230274828821,1.,-3.83845502790746));
#50120=CARTESIAN_POINT('Ctrl Pts',(1.38187013346109,1.,-3.84616425605764));
#50121=CARTESIAN_POINT('Ctrl Pts',(1.38139983115049,1.,-3.85387983979481));
#50122=CARTESIAN_POINT('Ctrl Pts',(1.38089205992989,1.,-3.86160143043959));
#50123=CARTESIAN_POINT('Ctrl Pts',(1.38034709213014,1.,-3.86932885813068));
#50124=CARTESIAN_POINT('Ctrl Pts',(1.37976523097073,1.,-3.87706205830532));
#50125=CARTESIAN_POINT('Ctrl Pts',(1.37914679719383,1.,-3.88480102249278));
#50126=CARTESIAN_POINT('Ctrl Pts',(1.3784921128802,1.,-3.89254574338496));
#50127=CARTESIAN_POINT('Ctrl Pts',(1.37780148512792,1.,-3.90029615196727));
#50128=CARTESIAN_POINT('Ctrl Pts',(1.3770751963402,1.,-3.90805209523486));
#50129=CARTESIAN_POINT('Ctrl Pts',(1.37631350505797,1.,-3.91581337462644));
#50130=CARTESIAN_POINT('Ctrl Pts',(1.37551664448242,1.,-3.92357976987672));
#50131=CARTESIAN_POINT('Ctrl Pts',(1.37468482215751,1.,-3.93135106761844));
#50132=CARTESIAN_POINT('Ctrl Pts',(1.37381821967165,1.,-3.93912709040818));
#50133=CARTESIAN_POINT('Ctrl Pts',(1.37291699202807,1.,-3.94690771785133));
#50134=CARTESIAN_POINT('Ctrl Pts',(1.37198126432386,1.,-3.95469287280914));
#50135=CARTESIAN_POINT('Ctrl Pts',(1.3712051561502,1.,-3.96092458506535));
#50136=CARTESIAN_POINT('Ctrl Pts',(1.37060761745635,1.,-3.96560037974645));
#50137=CARTESIAN_POINT('Ctrl Pts',(1.37020239094614,1.,-3.9687184694131));
#50138=CARTESIAN_POINT('Ctrl Pts',(1.36999806084572,1.,-3.97027773754922));
#50139=CARTESIAN_POINT('Origin',(1.36999806084572,0.,-3.97027773754922));
#50140=CARTESIAN_POINT('',(1.22531898815164,1.,-4.01728681790024));
#50141=CARTESIAN_POINT('Origin',(0.,0.,0.));
#50142=CARTESIAN_POINT('',(1.51895082866166,1.,-3.42859860294378));
#50143=CARTESIAN_POINT('Origin',(0.,1.,0.));
#50144=CARTESIAN_POINT('Ctrl Pts',(1.51895082866166,1.,-3.42859860294378));
#50145=CARTESIAN_POINT('Ctrl Pts',(1.51895082866166,0.666666666666667,-3.42859860294378));
#50146=CARTESIAN_POINT('Ctrl Pts',(1.51895082866166,0.333333333333333,-3.42859860294378));
#50147=CARTESIAN_POINT('Ctrl Pts',(1.51895082866166,-0.333333333333333,
-3.42859860294378));
#50148=CARTESIAN_POINT('Ctrl Pts',(1.51895082866166,-0.666666666666667,
-3.42859860294378));
#50149=CARTESIAN_POINT('Ctrl Pts',(1.51895082866166,-1.,-3.42859860294378));
#50150=CARTESIAN_POINT('Ctrl Pts',(1.83867539237861,-1.,-3.77614523045147));
#50151=CARTESIAN_POINT('Ctrl Pts',(1.83867539237861,1.,-3.77614523045147));
#50152=CARTESIAN_POINT('Ctrl Pts',(1.83742834010821,-1.,-3.77518714458232));
#50153=CARTESIAN_POINT('Ctrl Pts',(1.83742834010821,1.,-3.77518714458232));
#50154=CARTESIAN_POINT('Ctrl Pts',(1.83493697935064,-1.,-3.77326886065484));
#50155=CARTESIAN_POINT('Ctrl Pts',(1.83493697935064,1.,-3.77326886065484));
#50156=CARTESIAN_POINT('Ctrl Pts',(1.83120816956515,-1.,-3.77038509819777));
#50157=CARTESIAN_POINT('Ctrl Pts',(1.83120816956515,1.,-3.77038509819777));
#50158=CARTESIAN_POINT('Ctrl Pts',(1.82625289221933,-1.,-3.76652740355856));
#50159=CARTESIAN_POINT('Ctrl Pts',(1.82625289221933,1.,-3.76652740355856));
#50160=CARTESIAN_POINT('Ctrl Pts',(1.82008629694924,-1.,-3.76168412709652));
#50161=CARTESIAN_POINT('Ctrl Pts',(1.82008629694924,1.,-3.76168412709652));
#50162=CARTESIAN_POINT('Ctrl Pts',(1.81394729834032,-1.,-3.75681965683995));
#50163=CARTESIAN_POINT('Ctrl Pts',(1.81394729834032,1.,-3.75681965683995));
#50164=CARTESIAN_POINT('Ctrl Pts',(1.80783603939662,-1.,-3.75193395888069));
#50165=CARTESIAN_POINT('Ctrl Pts',(1.80783603939662,1.,-3.75193395888069));
#50166=CARTESIAN_POINT('Ctrl Pts',(1.80175271485519,-1.,-3.74702700874954));
#50167=CARTESIAN_POINT('Ctrl Pts',(1.80175271485519,1.,-3.74702700874954));
#50168=CARTESIAN_POINT('Ctrl Pts',(1.79569757859041,-1.,-3.74209880351667));
#50169=CARTESIAN_POINT('Ctrl Pts',(1.79569757859041,1.,-3.74209880351667));
#50170=CARTESIAN_POINT('Ctrl Pts',(1.78967092823139,-1.,-3.73714934729962));
#50171=CARTESIAN_POINT('Ctrl Pts',(1.78967092823139,1.,-3.73714934729962));
#50172=CARTESIAN_POINT('Ctrl Pts',(1.78367308442682,-1.,-3.73217863095022));
#50173=CARTESIAN_POINT('Ctrl Pts',(1.78367308442682,1.,-3.73217863095022));
#50174=CARTESIAN_POINT('Ctrl Pts',(1.77770437039606,-1.,-3.72718661205504));
#50175=CARTESIAN_POINT('Ctrl Pts',(1.77770437039606,1.,-3.72718661205504));
#50176=CARTESIAN_POINT('Ctrl Pts',(1.77176509401846,-1.,-3.72217319911429));
#50177=CARTESIAN_POINT('Ctrl Pts',(1.77176509401846,1.,-3.72217319911429));
#50178=CARTESIAN_POINT('Ctrl Pts',(1.76585552124549,-1.,-3.71713822377676));
#50179=CARTESIAN_POINT('Ctrl Pts',(1.76585552124549,1.,-3.71713822377676));
#50180=CARTESIAN_POINT('Ctrl Pts',(1.75997588499021,-1.,-3.71208146346455));
#50181=CARTESIAN_POINT('Ctrl Pts',(1.75997588499021,1.,-3.71208146346455));
#50182=CARTESIAN_POINT('Ctrl Pts',(1.75412641804148,-1.,-3.70700269736876));
#50183=CARTESIAN_POINT('Ctrl Pts',(1.75412641804148,1.,-3.70700269736876));
#50184=CARTESIAN_POINT('Ctrl Pts',(1.74830738046092,-1.,-3.70190175673422));
#50185=CARTESIAN_POINT('Ctrl Pts',(1.74830738046092,1.,-3.70190175673422));
#50186=CARTESIAN_POINT('Ctrl Pts',(1.74251908492589,-1.,-3.6967785691046));
#50187=CARTESIAN_POINT('Ctrl Pts',(1.74251908492589,1.,-3.6967785691046));
#50188=CARTESIAN_POINT('Ctrl Pts',(1.73676193254493,-1.,-3.69163322647906));
#50189=CARTESIAN_POINT('Ctrl Pts',(1.73676193254493,1.,-3.69163322647906));
#50190=CARTESIAN_POINT('Ctrl Pts',(1.73103640956647,-1.,-3.68646597019188));
#50191=CARTESIAN_POINT('Ctrl Pts',(1.73103640956647,1.,-3.68646597019188));
#50192=CARTESIAN_POINT('Ctrl Pts',(1.72534302437003,-1.,-3.68127704936472));
#50193=CARTESIAN_POINT('Ctrl Pts',(1.72534302437003,1.,-3.68127704936472));
#50194=CARTESIAN_POINT('Ctrl Pts',(1.71968225581787,-1.,-3.67606660374665));
#50195=CARTESIAN_POINT('Ctrl Pts',(1.71968225581787,1.,-3.67606660374665));
#50196=CARTESIAN_POINT('Ctrl Pts',(1.71405450210392,-1.,-3.67083454901629));
#50197=CARTESIAN_POINT('Ctrl Pts',(1.71405450210392,1.,-3.67083454901629));
#50198=CARTESIAN_POINT('Ctrl Pts',(1.70846001610983,-1.,-3.6655804319893));
#50199=CARTESIAN_POINT('Ctrl Pts',(1.70846001610983,1.,-3.6655804319893));
#50200=CARTESIAN_POINT('Ctrl Pts',(1.70289888566904,-1.,-3.6603033877491));
#50201=CARTESIAN_POINT('Ctrl Pts',(1.70289888566904,1.,-3.6603033877491));
#50202=CARTESIAN_POINT('Ctrl Pts',(1.69737117722558,-1.,-3.65500246526798));
#50203=CARTESIAN_POINT('Ctrl Pts',(1.69737117722558,1.,-3.65500246526798));
#50204=CARTESIAN_POINT('Ctrl Pts',(1.691877054817,-1.,-3.64967689827393));
#50205=CARTESIAN_POINT('Ctrl Pts',(1.691877054817,1.,-3.64967689827393));
#50206=CARTESIAN_POINT('Ctrl Pts',(1.68641690471455,-1.,-3.64432638915199));
#50207=CARTESIAN_POINT('Ctrl Pts',(1.68641690471455,1.,-3.64432638915199));
#50208=CARTESIAN_POINT('Ctrl Pts',(1.68099146651577,-1.,-3.63895140887443));
#50209=CARTESIAN_POINT('Ctrl Pts',(1.68099146651577,1.,-3.63895140887443));
#50210=CARTESIAN_POINT('Ctrl Pts',(1.67560193613145,-1.,-3.63355343201211));
#50211=CARTESIAN_POINT('Ctrl Pts',(1.67560193613145,1.,-3.63355343201211));
#50212=CARTESIAN_POINT('Ctrl Pts',(1.67024966008037,-1.,-3.62813422105257));
#50213=CARTESIAN_POINT('Ctrl Pts',(1.67024966008037,1.,-3.62813422105257));
#50214=CARTESIAN_POINT('Ctrl Pts',(1.66493585923853,-1.,-3.62269517989104));
#50215=CARTESIAN_POINT('Ctrl Pts',(1.66493585923853,1.,-3.62269517989104));
#50216=CARTESIAN_POINT('Ctrl Pts',(1.65966133399186,-1.,-3.61723666482457));
#50217=CARTESIAN_POINT('Ctrl Pts',(1.65966133399186,1.,-3.61723666482457));
#50218=CARTESIAN_POINT('Ctrl Pts',(1.65442619244327,-1.,-3.61175734965129));
#50219=CARTESIAN_POINT('Ctrl Pts',(1.65442619244327,1.,-3.61175734965129));
#50220=CARTESIAN_POINT('Ctrl Pts',(1.64922952425833,-1.,-3.60625346556992));
#50221=CARTESIAN_POINT('Ctrl Pts',(1.64922952425833,1.,-3.60625346556992));
#50222=CARTESIAN_POINT('Ctrl Pts',(1.6440700438558,-1.,-3.6007202851384));
#50223=CARTESIAN_POINT('Ctrl Pts',(1.6440700438558,1.,-3.6007202851384));
#50224=CARTESIAN_POINT('Ctrl Pts',(1.63894676675349,-1.,-3.59515368334887));
#50225=CARTESIAN_POINT('Ctrl Pts',(1.63894676675349,1.,-3.59515368334887));
#50226=CARTESIAN_POINT('Ctrl Pts',(1.63385971451259,-1.,-3.58955176627876));
#50227=CARTESIAN_POINT('Ctrl Pts',(1.63385971451259,1.,-3.58955176627876));
#50228=CARTESIAN_POINT('Ctrl Pts',(1.62881051550748,-1.,-3.5839162577435));
#50229=CARTESIAN_POINT('Ctrl Pts',(1.62881051550748,1.,-3.5839162577435));
#50230=CARTESIAN_POINT('Ctrl Pts',(1.62380329464851,-1.,-3.57825455954405));
#50231=CARTESIAN_POINT('Ctrl Pts',(1.62380329464851,1.,-3.57825455954405));
#50232=CARTESIAN_POINT('Ctrl Pts',(1.61884340915412,-1.,-3.57257679609826));
#50233=CARTESIAN_POINT('Ctrl Pts',(1.61884340915412,1.,-3.57257679609826));
#50234=CARTESIAN_POINT('Ctrl Pts',(1.61393581747522,-1.,-3.56689200468404));
#50235=CARTESIAN_POINT('Ctrl Pts',(1.61393581747522,1.,-3.56689200468404));
#50236=CARTESIAN_POINT('Ctrl Pts',(1.60908344685459,-1.,-3.56120432482986));
#50237=CARTESIAN_POINT('Ctrl Pts',(1.60908344685459,1.,-3.56120432482986));
#50238=CARTESIAN_POINT('Ctrl Pts',(1.60428584699848,-1.,-3.55550985096117));
#50239=CARTESIAN_POINT('Ctrl Pts',(1.60428584699848,1.,-3.55550985096117));
#50240=CARTESIAN_POINT('Ctrl Pts',(1.59953698113444,-1.,-3.54979148634426));
#50241=CARTESIAN_POINT('Ctrl Pts',(1.59953698113444,1.,-3.54979148634426));
#50242=CARTESIAN_POINT('Ctrl Pts',(1.5948276694975,-1.,-3.544024581823));
#50243=CARTESIAN_POINT('Ctrl Pts',(1.5948276694975,1.,-3.544024581823));
#50244=CARTESIAN_POINT('Ctrl Pts',(1.59014958368725,-1.,-3.53818616861045));
#50245=CARTESIAN_POINT('Ctrl Pts',(1.59014958368725,1.,-3.53818616861045));
#50246=CARTESIAN_POINT('Ctrl Pts',(1.58549906268083,-1.,-3.53226378147068));
#50247=CARTESIAN_POINT('Ctrl Pts',(1.58549906268083,1.,-3.53226378147068));
#50248=CARTESIAN_POINT('Ctrl Pts',(1.58088027227856,-1.,-3.52626275334899));
#50249=CARTESIAN_POINT('Ctrl Pts',(1.58088027227856,1.,-3.52626275334899));
#50250=CARTESIAN_POINT('Ctrl Pts',(1.5763104998818,-1.,-3.52021847865961));
#50251=CARTESIAN_POINT('Ctrl Pts',(1.5763104998818,1.,-3.52021847865961));
#50252=CARTESIAN_POINT('Ctrl Pts',(1.57181569799774,-1.,-3.51418598431733));
#50253=CARTESIAN_POINT('Ctrl Pts',(1.57181569799774,1.,-3.51418598431733));
#50254=CARTESIAN_POINT('Ctrl Pts',(1.56742097575041,-1.,-3.50821771695427));
#50255=CARTESIAN_POINT('Ctrl Pts',(1.56742097575041,1.,-3.50821771695427));
#50256=CARTESIAN_POINT('Ctrl Pts',(1.56314187758689,-1.,-3.50234321621607));
#50257=CARTESIAN_POINT('Ctrl Pts',(1.56314187758689,1.,-3.50234321621607));
#50258=CARTESIAN_POINT('Ctrl Pts',(1.55897703097859,-1.,-3.49655185179623));
#50259=CARTESIAN_POINT('Ctrl Pts',(1.55897703097859,1.,-3.49655185179623));
#50260=CARTESIAN_POINT('Ctrl Pts',(1.5548959590107,-1.,-3.49076460877317));
#50261=CARTESIAN_POINT('Ctrl Pts',(1.5548959590107,1.,-3.49076460877317));
#50262=CARTESIAN_POINT('Ctrl Pts',(1.55084702970382,-1.,-3.48485155928414));
#50263=CARTESIAN_POINT('Ctrl Pts',(1.55084702970382,1.,-3.48485155928414));
#50264=CARTESIAN_POINT('Ctrl Pts',(1.54678009290206,-1.,-3.47868272898599));
#50265=CARTESIAN_POINT('Ctrl Pts',(1.54678009290206,1.,-3.47868272898599));
#50266=CARTESIAN_POINT('Ctrl Pts',(1.54266605398152,-1.,-3.47217189224576));
#50267=CARTESIAN_POINT('Ctrl Pts',(1.54266605398152,1.,-3.47217189224576));
#50268=CARTESIAN_POINT('Ctrl Pts',(1.53851507915533,-1.,-3.46531752207222));
#50269=CARTESIAN_POINT('Ctrl Pts',(1.53851507915533,1.,-3.46531752207222));
#50270=CARTESIAN_POINT('Ctrl Pts',(1.53440195378902,-1.,-3.45825932955273));
#50271=CARTESIAN_POINT('Ctrl Pts',(1.53440195378902,1.,-3.45825932955273));
#50272=CARTESIAN_POINT('Ctrl Pts',(1.530462444618,-1.,-3.45127136828667));
#50273=CARTESIAN_POINT('Ctrl Pts',(1.530462444618,1.,-3.45127136828667));
#50274=CARTESIAN_POINT('Ctrl Pts',(1.52686242875717,-1.,-3.44469547527));
#50275=CARTESIAN_POINT('Ctrl Pts',(1.52686242875717,1.,-3.44469547527));
#50276=CARTESIAN_POINT('Ctrl Pts',(1.52377348950429,-1.,-3.43888895974182));
#50277=CARTESIAN_POINT('Ctrl Pts',(1.52377348950429,1.,-3.43888895974182));
#50278=CARTESIAN_POINT('Ctrl Pts',(1.52134826724227,-1.,-3.43417156977749));
#50279=CARTESIAN_POINT('Ctrl Pts',(1.52134826724227,1.,-3.43417156977749));
#50280=CARTESIAN_POINT('Ctrl Pts',(1.51969006980792,-1.,-3.43076036253384));
#50281=CARTESIAN_POINT('Ctrl Pts',(1.51969006980792,1.,-3.43076036253384));
#50282=CARTESIAN_POINT('Ctrl Pts',(1.51901585838879,-1.,-3.42915787669388));
#50283=CARTESIAN_POINT('Ctrl Pts',(1.51901585838879,1.,-3.42915787669388));
#50284=CARTESIAN_POINT('Ctrl Pts',(1.51888450659497,-1.,-3.42860527148835));
#50285=CARTESIAN_POINT('Ctrl Pts',(1.51888450659497,1.,-3.42860527148835));
#50286=CARTESIAN_POINT('Ctrl Pts',(1.51896318668306,-1.,-3.42852521763648));
#50287=CARTESIAN_POINT('Ctrl Pts',(1.51896318668306,1.,-3.42852521763648));
#50288=CARTESIAN_POINT('Ctrl Pts',(1.519044091397,-1.,-3.42855728381368));
#50289=CARTESIAN_POINT('Ctrl Pts',(1.519044091397,1.,-3.42855728381368));
#50290=CARTESIAN_POINT('',(1.83867539237861,1.,-3.77614523045147));
#50291=CARTESIAN_POINT('Ctrl Pts',(1.83867539237861,1.,-3.77614523045147));
#50292=CARTESIAN_POINT('Ctrl Pts',(1.83742834010821,1.,-3.77518714458232));
#50293=CARTESIAN_POINT('Ctrl Pts',(1.83493697935064,1.,-3.77326886065484));
#50294=CARTESIAN_POINT('Ctrl Pts',(1.83120816956515,1.,-3.77038509819777));
#50295=CARTESIAN_POINT('Ctrl Pts',(1.82625289221933,1.,-3.76652740355856));
#50296=CARTESIAN_POINT('Ctrl Pts',(1.82008629694924,1.,-3.76168412709652));
#50297=CARTESIAN_POINT('Ctrl Pts',(1.81394729834032,1.,-3.75681965683995));
#50298=CARTESIAN_POINT('Ctrl Pts',(1.80783603939662,1.,-3.75193395888069));
#50299=CARTESIAN_POINT('Ctrl Pts',(1.80175271485519,1.,-3.74702700874954));
#50300=CARTESIAN_POINT('Ctrl Pts',(1.79569757859041,1.,-3.74209880351667));
#50301=CARTESIAN_POINT('Ctrl Pts',(1.78967092823139,1.,-3.73714934729962));
#50302=CARTESIAN_POINT('Ctrl Pts',(1.78367308442682,1.,-3.73217863095022));
#50303=CARTESIAN_POINT('Ctrl Pts',(1.77770437039606,1.,-3.72718661205504));
#50304=CARTESIAN_POINT('Ctrl Pts',(1.77176509401846,1.,-3.72217319911429));
#50305=CARTESIAN_POINT('Ctrl Pts',(1.76585552124549,1.,-3.71713822377676));
#50306=CARTESIAN_POINT('Ctrl Pts',(1.75997588499021,1.,-3.71208146346455));
#50307=CARTESIAN_POINT('Ctrl Pts',(1.75412641804148,1.,-3.70700269736876));
#50308=CARTESIAN_POINT('Ctrl Pts',(1.74830738046092,1.,-3.70190175673422));
#50309=CARTESIAN_POINT('Ctrl Pts',(1.74251908492589,1.,-3.6967785691046));
#50310=CARTESIAN_POINT('Ctrl Pts',(1.73676193254493,1.,-3.69163322647906));
#50311=CARTESIAN_POINT('Ctrl Pts',(1.73103640956647,1.,-3.68646597019188));
#50312=CARTESIAN_POINT('Ctrl Pts',(1.72534302437003,1.,-3.68127704936472));
#50313=CARTESIAN_POINT('Ctrl Pts',(1.71968225581787,1.,-3.67606660374665));
#50314=CARTESIAN_POINT('Ctrl Pts',(1.71405450210392,1.,-3.67083454901629));
#50315=CARTESIAN_POINT('Ctrl Pts',(1.70846001610983,1.,-3.6655804319893));
#50316=CARTESIAN_POINT('Ctrl Pts',(1.70289888566904,1.,-3.6603033877491));
#50317=CARTESIAN_POINT('Ctrl Pts',(1.69737117722558,1.,-3.65500246526798));
#50318=CARTESIAN_POINT('Ctrl Pts',(1.691877054817,1.,-3.64967689827393));
#50319=CARTESIAN_POINT('Ctrl Pts',(1.68641690471455,1.,-3.64432638915199));
#50320=CARTESIAN_POINT('Ctrl Pts',(1.68099146651577,1.,-3.63895140887443));
#50321=CARTESIAN_POINT('Ctrl Pts',(1.67560193613145,1.,-3.63355343201211));
#50322=CARTESIAN_POINT('Ctrl Pts',(1.67024966008037,1.,-3.62813422105257));
#50323=CARTESIAN_POINT('Ctrl Pts',(1.66493585923853,1.,-3.62269517989104));
#50324=CARTESIAN_POINT('Ctrl Pts',(1.65966133399186,1.,-3.61723666482457));
#50325=CARTESIAN_POINT('Ctrl Pts',(1.65442619244327,1.,-3.61175734965129));
#50326=CARTESIAN_POINT('Ctrl Pts',(1.64922952425833,1.,-3.60625346556992));
#50327=CARTESIAN_POINT('Ctrl Pts',(1.6440700438558,1.,-3.6007202851384));
#50328=CARTESIAN_POINT('Ctrl Pts',(1.63894676675349,1.,-3.59515368334887));
#50329=CARTESIAN_POINT('Ctrl Pts',(1.63385971451259,1.,-3.58955176627876));
#50330=CARTESIAN_POINT('Ctrl Pts',(1.62881051550748,1.,-3.5839162577435));
#50331=CARTESIAN_POINT('Ctrl Pts',(1.62380329464851,1.,-3.57825455954405));
#50332=CARTESIAN_POINT('Ctrl Pts',(1.61884340915412,1.,-3.57257679609826));
#50333=CARTESIAN_POINT('Ctrl Pts',(1.61393581747522,1.,-3.56689200468404));
#50334=CARTESIAN_POINT('Ctrl Pts',(1.60908344685459,1.,-3.56120432482986));
#50335=CARTESIAN_POINT('Ctrl Pts',(1.60428584699848,1.,-3.55550985096117));
#50336=CARTESIAN_POINT('Ctrl Pts',(1.59953698113444,1.,-3.54979148634426));
#50337=CARTESIAN_POINT('Ctrl Pts',(1.5948276694975,1.,-3.544024581823));
#50338=CARTESIAN_POINT('Ctrl Pts',(1.59014958368725,1.,-3.53818616861045));
#50339=CARTESIAN_POINT('Ctrl Pts',(1.58549906268083,1.,-3.53226378147068));
#50340=CARTESIAN_POINT('Ctrl Pts',(1.58088027227856,1.,-3.52626275334899));
#50341=CARTESIAN_POINT('Ctrl Pts',(1.5763104998818,1.,-3.52021847865961));
#50342=CARTESIAN_POINT('Ctrl Pts',(1.57181569799774,1.,-3.51418598431733));
#50343=CARTESIAN_POINT('Ctrl Pts',(1.56742097575041,1.,-3.50821771695427));
#50344=CARTESIAN_POINT('Ctrl Pts',(1.56314187758689,1.,-3.50234321621607));
#50345=CARTESIAN_POINT('Ctrl Pts',(1.55897703097859,1.,-3.49655185179623));
#50346=CARTESIAN_POINT('Ctrl Pts',(1.5548959590107,1.,-3.49076460877317));
#50347=CARTESIAN_POINT('Ctrl Pts',(1.55084702970382,1.,-3.48485155928414));
#50348=CARTESIAN_POINT('Ctrl Pts',(1.54678009290206,1.,-3.47868272898599));
#50349=CARTESIAN_POINT('Ctrl Pts',(1.54266605398152,1.,-3.47217189224576));
#50350=CARTESIAN_POINT('Ctrl Pts',(1.53851507915533,1.,-3.46531752207222));
#50351=CARTESIAN_POINT('Ctrl Pts',(1.53440195378902,1.,-3.45825932955273));
#50352=CARTESIAN_POINT('Ctrl Pts',(1.530462444618,1.,-3.45127136828667));
#50353=CARTESIAN_POINT('Ctrl Pts',(1.52686242875717,1.,-3.44469547527));
#50354=CARTESIAN_POINT('Ctrl Pts',(1.52377348950429,1.,-3.43888895974182));
#50355=CARTESIAN_POINT('Ctrl Pts',(1.52134826724227,1.,-3.43417156977749));
#50356=CARTESIAN_POINT('Ctrl Pts',(1.5198144909343,1.,-3.43101631893491));
#50357=CARTESIAN_POINT('Ctrl Pts',(1.51914806898539,1.,-3.42946838852728));
#50358=CARTESIAN_POINT('Ctrl Pts',(1.51895133295017,1.,-3.42884302333978));
#50359=CARTESIAN_POINT('Ctrl Pts',(1.51893924967231,1.,-3.42864616361967));
#50360=CARTESIAN_POINT('Ctrl Pts',(1.51895082866166,1.,-3.42859860294378));
#50361=CARTESIAN_POINT('',(1.83867539237861,0.,-3.77614523045147));
#50362=CARTESIAN_POINT('Ctrl Pts',(1.8808893942881,-1.,-3.24418789321065));
#50363=CARTESIAN_POINT('Ctrl Pts',(1.8808893942881,1.,-3.24418789321065));
#50364=CARTESIAN_POINT('Ctrl Pts',(1.8809110068042,-1.,-3.24410359189733));
#50365=CARTESIAN_POINT('Ctrl Pts',(1.8809110068042,1.,-3.24410359189733));
#50366=CARTESIAN_POINT('Ctrl Pts',(1.8810220187274,-1.,-3.24408699284449));
#50367=CARTESIAN_POINT('Ctrl Pts',(1.8810220187274,1.,-3.24408699284449));
#50368=CARTESIAN_POINT('Ctrl Pts',(1.88139187908347,-1.,-3.24451807186964));
#50369=CARTESIAN_POINT('Ctrl Pts',(1.88139187908347,1.,-3.24451807186964));
#50370=CARTESIAN_POINT('Ctrl Pts',(1.88229202583187,-1.,-3.24600543790876));
#50371=CARTESIAN_POINT('Ctrl Pts',(1.88229202583187,1.,-3.24600543790876));
#50372=CARTESIAN_POINT('Ctrl Pts',(1.88407708646435,-1.,-3.24935200512055));
#50373=CARTESIAN_POINT('Ctrl Pts',(1.88407708646435,1.,-3.24935200512055));
#50374=CARTESIAN_POINT('Ctrl Pts',(1.88646802523372,-1.,-3.25408686339298));
#50375=CARTESIAN_POINT('Ctrl Pts',(1.88646802523372,1.,-3.25408686339298));
#50376=CARTESIAN_POINT('Ctrl Pts',(1.88934996203508,-1.,-3.2599988519361));
#50377=CARTESIAN_POINT('Ctrl Pts',(1.88934996203508,1.,-3.2599988519361));
#50378=CARTESIAN_POINT('Ctrl Pts',(1.89255393500769,-1.,-3.2667765388833));
#50379=CARTESIAN_POINT('Ctrl Pts',(1.89255393500769,1.,-3.2667765388833));
#50380=CARTESIAN_POINT('Ctrl Pts',(1.89589172903662,-1.,-3.27407108932908));
#50381=CARTESIAN_POINT('Ctrl Pts',(1.89589172903662,1.,-3.27407108932908));
#50382=CARTESIAN_POINT('Ctrl Pts',(1.89918429230424,-1.,-3.28154737912287));
#50383=CARTESIAN_POINT('Ctrl Pts',(1.89918429230424,1.,-3.28154737912287));
#50384=CARTESIAN_POINT('Ctrl Pts',(1.9022897124757,-1.,-3.28893448600364));
#50385=CARTESIAN_POINT('Ctrl Pts',(1.9022897124757,1.,-3.28893448600364));
#50386=CARTESIAN_POINT('Ctrl Pts',(1.9051389186417,-1.,-3.29608978722258));
#50387=CARTESIAN_POINT('Ctrl Pts',(1.9051389186417,1.,-3.29608978722258));
#50388=CARTESIAN_POINT('Ctrl Pts',(1.90773912171424,-1.,-3.30300595568341));
#50389=CARTESIAN_POINT('Ctrl Pts',(1.90773912171424,1.,-3.30300595568341));
#50390=CARTESIAN_POINT('Ctrl Pts',(1.91014297830502,-1.,-3.30975721158694));
#50391=CARTESIAN_POINT('Ctrl Pts',(1.91014297830502,1.,-3.30975721158694));
#50392=CARTESIAN_POINT('Ctrl Pts',(1.91242616234459,-1.,-3.31646052426395));
#50393=CARTESIAN_POINT('Ctrl Pts',(1.91242616234459,1.,-3.31646052426395));
#50394=CARTESIAN_POINT('Ctrl Pts',(1.91466343916612,-1.,-3.32323403454507));
#50395=CARTESIAN_POINT('Ctrl Pts',(1.91466343916612,1.,-3.32323403454507));
#50396=CARTESIAN_POINT('Ctrl Pts',(1.91690081930297,-1.,-3.33014884257812));
#50397=CARTESIAN_POINT('Ctrl Pts',(1.91690081930297,1.,-3.33014884257812));
#50398=CARTESIAN_POINT('Ctrl Pts',(1.91914609610173,-1.,-3.33721230709948));
#50399=CARTESIAN_POINT('Ctrl Pts',(1.91914609610173,1.,-3.33721230709948));
#50400=CARTESIAN_POINT('Ctrl Pts',(1.92138450828378,-1.,-3.34439448941915));
#50401=CARTESIAN_POINT('Ctrl Pts',(1.92138450828378,1.,-3.34439448941915));
#50402=CARTESIAN_POINT('Ctrl Pts',(1.92358838440518,-1.,-3.35164424847207));
#50403=CARTESIAN_POINT('Ctrl Pts',(1.92358838440518,1.,-3.35164424847207));
#50404=CARTESIAN_POINT('Ctrl Pts',(1.92572846125763,-1.,-3.35890824422976));
#50405=CARTESIAN_POINT('Ctrl Pts',(1.92572846125763,1.,-3.35890824422976));
#50406=CARTESIAN_POINT('Ctrl Pts',(1.92778626543803,-1.,-3.36615168657597));
#50407=CARTESIAN_POINT('Ctrl Pts',(1.92778626543803,1.,-3.36615168657597));
#50408=CARTESIAN_POINT('Ctrl Pts',(1.92975993109897,-1.,-3.37336807068078));
#50409=CARTESIAN_POINT('Ctrl Pts',(1.92975993109897,1.,-3.37336807068078));
#50410=CARTESIAN_POINT('Ctrl Pts',(1.93165739093292,-1.,-3.38056768525577));
#50411=CARTESIAN_POINT('Ctrl Pts',(1.93165739093292,1.,-3.38056768525577));
#50412=CARTESIAN_POINT('Ctrl Pts',(1.93349233176794,-1.,-3.38777076883267));
#50413=CARTESIAN_POINT('Ctrl Pts',(1.93349233176794,1.,-3.38777076883267));
#50414=CARTESIAN_POINT('Ctrl Pts',(1.93527929945982,-1.,-3.39499923640789));
#50415=CARTESIAN_POINT('Ctrl Pts',(1.93527929945982,1.,-3.39499923640789));
#50416=CARTESIAN_POINT('Ctrl Pts',(1.93702857723089,-1.,-3.40226802104093));
#50417=CARTESIAN_POINT('Ctrl Pts',(1.93702857723089,1.,-3.40226802104093));
#50418=CARTESIAN_POINT('Ctrl Pts',(1.93874306008132,-1.,-3.40957978266623));
#50419=CARTESIAN_POINT('Ctrl Pts',(1.93874306008132,1.,-3.40957978266623));
#50420=CARTESIAN_POINT('Ctrl Pts',(1.94042111965237,-1.,-3.41692971994082));
#50421=CARTESIAN_POINT('Ctrl Pts',(1.94042111965237,1.,-3.41692971994082));
#50422=CARTESIAN_POINT('Ctrl Pts',(1.94205835913692,-1.,-3.42430850941497));
#50423=CARTESIAN_POINT('Ctrl Pts',(1.94205835913692,1.,-3.42430850941497));
#50424=CARTESIAN_POINT('Ctrl Pts',(1.94364973660285,-1.,-3.43170586602436));
#50425=CARTESIAN_POINT('Ctrl Pts',(1.94364973660285,1.,-3.43170586602436));
#50426=CARTESIAN_POINT('Ctrl Pts',(1.94519168842883,-1.,-3.43911410197693));
#50427=CARTESIAN_POINT('Ctrl Pts',(1.94519168842883,1.,-3.43911410197693));
#50428=CARTESIAN_POINT('Ctrl Pts',(1.94668377715332,-1.,-3.44653088665685));
#50429=CARTESIAN_POINT('Ctrl Pts',(1.94668377715332,1.,-3.44653088665685));
#50430=CARTESIAN_POINT('Ctrl Pts',(1.94812754766524,-1.,-3.45395731584051));
#50431=CARTESIAN_POINT('Ctrl Pts',(1.94812754766524,1.,-3.45395731584051));
#50432=CARTESIAN_POINT('Ctrl Pts',(1.94952575850196,-1.,-3.46139661060959));
#50433=CARTESIAN_POINT('Ctrl Pts',(1.94952575850196,1.,-3.46139661060959));
#50434=CARTESIAN_POINT('Ctrl Pts',(1.95088147859876,-1.,-3.4688525897419));
#50435=CARTESIAN_POINT('Ctrl Pts',(1.95088147859876,1.,-3.4688525897419));
#50436=CARTESIAN_POINT('Ctrl Pts',(1.95219722189878,-1.,-3.47632820495926));
#50437=CARTESIAN_POINT('Ctrl Pts',(1.95219722189878,1.,-3.47632820495926));
#50438=CARTESIAN_POINT('Ctrl Pts',(1.95347412486316,-1.,-3.48382414832649));
#50439=CARTESIAN_POINT('Ctrl Pts',(1.95347412486316,1.,-3.48382414832649));
#50440=CARTESIAN_POINT('Ctrl Pts',(1.95471236969653,-1.,-3.49133956289154));
#50441=CARTESIAN_POINT('Ctrl Pts',(1.95471236969653,1.,-3.49133956289154));
#50442=CARTESIAN_POINT('Ctrl Pts',(1.9559115382367,-1.,-3.49887263575602));
#50443=CARTESIAN_POINT('Ctrl Pts',(1.9559115382367,1.,-3.49887263575602));
#50444=CARTESIAN_POINT('Ctrl Pts',(1.95707099606513,-1.,-3.50642124159913));
#50445=CARTESIAN_POINT('Ctrl Pts',(1.95707099606513,1.,-3.50642124159913));
#50446=CARTESIAN_POINT('Ctrl Pts',(1.95819025316768,-1.,-3.51398354617773));
#50447=CARTESIAN_POINT('Ctrl Pts',(1.95819025316768,1.,-3.51398354617773));
#50448=CARTESIAN_POINT('Ctrl Pts',(1.95926936324436,-1.,-3.52155867431438));
#50449=CARTESIAN_POINT('Ctrl Pts',(1.95926936324436,1.,-3.52155867431438));
#50450=CARTESIAN_POINT('Ctrl Pts',(1.96030879411534,-1.,-3.52914648844289));
#50451=CARTESIAN_POINT('Ctrl Pts',(1.96030879411534,1.,-3.52914648844289));
#50452=CARTESIAN_POINT('Ctrl Pts',(1.96130926212661,-1.,-3.53674730625759));
#50453=CARTESIAN_POINT('Ctrl Pts',(1.96130926212661,1.,-3.53674730625759));
#50454=CARTESIAN_POINT('Ctrl Pts',(1.96227157573058,-1.,-3.54436163300425));
#50455=CARTESIAN_POINT('Ctrl Pts',(1.96227157573058,1.,-3.54436163300425));
#50456=CARTESIAN_POINT('Ctrl Pts',(1.96319648628667,-1.,-3.55198990600929));
#50457=CARTESIAN_POINT('Ctrl Pts',(1.96319648628667,1.,-3.55198990600929));
#50458=CARTESIAN_POINT('Ctrl Pts',(1.96408450906868,-1.,-3.55963218706201));
#50459=CARTESIAN_POINT('Ctrl Pts',(1.96408450906868,1.,-3.55963218706201));
#50460=CARTESIAN_POINT('Ctrl Pts',(1.96493594634643,-1.,-3.56728820357933));
#50461=CARTESIAN_POINT('Ctrl Pts',(1.96493594634643,1.,-3.56728820357933));
#50462=CARTESIAN_POINT('Ctrl Pts',(1.96575096652857,-1.,-3.57495748601088));
#50463=CARTESIAN_POINT('Ctrl Pts',(1.96575096652857,1.,-3.57495748601088));
#50464=CARTESIAN_POINT('Ctrl Pts',(1.9665296668894,-1.,-3.58263947663884));
#50465=CARTESIAN_POINT('Ctrl Pts',(1.9665296668894,1.,-3.58263947663884));
#50466=CARTESIAN_POINT('Ctrl Pts',(1.96727213799507,-1.,-3.5903336402273));
#50467=CARTESIAN_POINT('Ctrl Pts',(1.96727213799507,1.,-3.5903336402273));
#50468=CARTESIAN_POINT('Ctrl Pts',(1.96797854118257,-1.,-3.59803959819725));
#50469=CARTESIAN_POINT('Ctrl Pts',(1.96797854118257,1.,-3.59803959819725));
#50470=CARTESIAN_POINT('Ctrl Pts',(1.96864911885775,-1.,-3.60575714017676));
#50471=CARTESIAN_POINT('Ctrl Pts',(1.96864911885775,1.,-3.60575714017676));
#50472=CARTESIAN_POINT('Ctrl Pts',(1.96928416040712,-1.,-3.61348615496393));
#50473=CARTESIAN_POINT('Ctrl Pts',(1.96928416040712,1.,-3.61348615496393));
#50474=CARTESIAN_POINT('Ctrl Pts',(1.96988398129888,-1.,-3.62122658401722));
#50475=CARTESIAN_POINT('Ctrl Pts',(1.96988398129888,1.,-3.62122658401722));
#50476=CARTESIAN_POINT('Ctrl Pts',(1.97044889850518,-1.,-3.62897836973397));
#50477=CARTESIAN_POINT('Ctrl Pts',(1.97044889850518,1.,-3.62897836973397));
#50478=CARTESIAN_POINT('Ctrl Pts',(1.97097920454698,-1.,-3.63674139590853));
#50479=CARTESIAN_POINT('Ctrl Pts',(1.97097920454698,1.,-3.63674139590853));
#50480=CARTESIAN_POINT('Ctrl Pts',(1.97147515441539,-1.,-3.64451546724222));
#50481=CARTESIAN_POINT('Ctrl Pts',(1.97147515441539,1.,-3.64451546724222));
#50482=CARTESIAN_POINT('Ctrl Pts',(1.97193697240645,-1.,-3.65230034717364));
#50483=CARTESIAN_POINT('Ctrl Pts',(1.97193697240645,1.,-3.65230034717364));
#50484=CARTESIAN_POINT('Ctrl Pts',(1.97236485439317,-1.,-3.66009578166865));
#50485=CARTESIAN_POINT('Ctrl Pts',(1.97236485439317,1.,-3.66009578166865));
#50486=CARTESIAN_POINT('Ctrl Pts',(1.9727589719863,-1.,-3.66790152751984));
#50487=CARTESIAN_POINT('Ctrl Pts',(1.9727589719863,1.,-3.66790152751984));
#50488=CARTESIAN_POINT('Ctrl Pts',(1.97311947678035,-1.,-3.67571738106175));
#50489=CARTESIAN_POINT('Ctrl Pts',(1.97311947678035,1.,-3.67571738106175));
#50490=CARTESIAN_POINT('Ctrl Pts',(1.9734465030363,-1.,-3.68354319913416));
#50491=CARTESIAN_POINT('Ctrl Pts',(1.9734465030363,1.,-3.68354319913416));
#50492=CARTESIAN_POINT('Ctrl Pts',(1.97374016224397,-1.,-3.69137888597855));
#50493=CARTESIAN_POINT('Ctrl Pts',(1.97374016224397,1.,-3.69137888597855));
#50494=CARTESIAN_POINT('Ctrl Pts',(1.97394846382288,-1.,-3.69765528558292));
#50495=CARTESIAN_POINT('Ctrl Pts',(1.97394846382288,1.,-3.69765528558292));
#50496=CARTESIAN_POINT('Ctrl Pts',(1.97408973726149,-1.,-3.70236698911837));
#50497=CARTESIAN_POINT('Ctrl Pts',(1.97408973726149,1.,-3.70236698911837));
#50498=CARTESIAN_POINT('Ctrl Pts',(1.974177276451,-1.,-3.7055100813194));
#50499=CARTESIAN_POINT('Ctrl Pts',(1.974177276451,1.,-3.7055100813194));
#50500=CARTESIAN_POINT('Ctrl Pts',(1.97421938526992,-1.,-3.70708211654725));
#50501=CARTESIAN_POINT('Ctrl Pts',(1.97421938526992,1.,-3.70708211654725));
#50502=CARTESIAN_POINT('',(1.88097764062542,1.,-3.24413672884902));
#50503=CARTESIAN_POINT('Ctrl Pts',(1.88097764062541,-1.,-3.24413672884902));
#50504=CARTESIAN_POINT('Ctrl Pts',(1.88097764062541,-0.666666666666667,
-3.24413672884902));
#50505=CARTESIAN_POINT('Ctrl Pts',(1.88097764062541,-0.333333333333333,
-3.24413672884902));
#50506=CARTESIAN_POINT('Ctrl Pts',(1.88097764062541,0.333333333333333,-3.24413672884902));
#50507=CARTESIAN_POINT('Ctrl Pts',(1.88097764062541,0.666666666666667,-3.24413672884902));
#50508=CARTESIAN_POINT('Ctrl Pts',(1.88097764062541,1.,-3.24413672884902));
#50509=CARTESIAN_POINT('',(1.97421938526992,1.,-3.70708211654725));
#50510=CARTESIAN_POINT('',(1.97421938526992,0.,-3.70708211654725));
#50511=CARTESIAN_POINT('Ctrl Pts',(1.88097764062542,1.,-3.24413672884902));
#50512=CARTESIAN_POINT('Ctrl Pts',(1.88102292397987,1.,-3.24415531671311));
#50513=CARTESIAN_POINT('Ctrl Pts',(1.88117508446657,1.,-3.24428080352952));
#50514=CARTESIAN_POINT('Ctrl Pts',(1.88156537699118,1.,-3.24480754675942));
#50515=CARTESIAN_POINT('Ctrl Pts',(1.88242596600422,1.,-3.24625654410705));
#50516=CARTESIAN_POINT('Ctrl Pts',(1.88407708646435,1.,-3.24935200512055));
#50517=CARTESIAN_POINT('Ctrl Pts',(1.88646802523372,1.,-3.25408686339298));
#50518=CARTESIAN_POINT('Ctrl Pts',(1.88934996203508,1.,-3.2599988519361));
#50519=CARTESIAN_POINT('Ctrl Pts',(1.89255393500769,1.,-3.2667765388833));
#50520=CARTESIAN_POINT('Ctrl Pts',(1.89589172903662,1.,-3.27407108932908));
#50521=CARTESIAN_POINT('Ctrl Pts',(1.89918429230424,1.,-3.28154737912287));
#50522=CARTESIAN_POINT('Ctrl Pts',(1.9022897124757,1.,-3.28893448600364));
#50523=CARTESIAN_POINT('Ctrl Pts',(1.9051389186417,1.,-3.29608978722258));
#50524=CARTESIAN_POINT('Ctrl Pts',(1.90773912171424,1.,-3.30300595568341));
#50525=CARTESIAN_POINT('Ctrl Pts',(1.91014297830502,1.,-3.30975721158694));
#50526=CARTESIAN_POINT('Ctrl Pts',(1.91242616234459,1.,-3.31646052426395));
#50527=CARTESIAN_POINT('Ctrl Pts',(1.91466343916612,1.,-3.32323403454507));
#50528=CARTESIAN_POINT('Ctrl Pts',(1.91690081930297,1.,-3.33014884257812));
#50529=CARTESIAN_POINT('Ctrl Pts',(1.91914609610173,1.,-3.33721230709948));
#50530=CARTESIAN_POINT('Ctrl Pts',(1.92138450828378,1.,-3.34439448941915));
#50531=CARTESIAN_POINT('Ctrl Pts',(1.92358838440518,1.,-3.35164424847207));
#50532=CARTESIAN_POINT('Ctrl Pts',(1.92572846125763,1.,-3.35890824422976));
#50533=CARTESIAN_POINT('Ctrl Pts',(1.92778626543803,1.,-3.36615168657597));
#50534=CARTESIAN_POINT('Ctrl Pts',(1.92975993109897,1.,-3.37336807068078));
#50535=CARTESIAN_POINT('Ctrl Pts',(1.93165739093292,1.,-3.38056768525577));
#50536=CARTESIAN_POINT('Ctrl Pts',(1.93349233176794,1.,-3.38777076883267));
#50537=CARTESIAN_POINT('Ctrl Pts',(1.93527929945982,1.,-3.39499923640789));
#50538=CARTESIAN_POINT('Ctrl Pts',(1.93702857723089,1.,-3.40226802104093));
#50539=CARTESIAN_POINT('Ctrl Pts',(1.93874306008132,1.,-3.40957978266623));
#50540=CARTESIAN_POINT('Ctrl Pts',(1.94042111965237,1.,-3.41692971994082));
#50541=CARTESIAN_POINT('Ctrl Pts',(1.94205835913692,1.,-3.42430850941497));
#50542=CARTESIAN_POINT('Ctrl Pts',(1.94364973660285,1.,-3.43170586602436));
#50543=CARTESIAN_POINT('Ctrl Pts',(1.94519168842883,1.,-3.43911410197693));
#50544=CARTESIAN_POINT('Ctrl Pts',(1.94668377715332,1.,-3.44653088665685));
#50545=CARTESIAN_POINT('Ctrl Pts',(1.94812754766524,1.,-3.45395731584051));
#50546=CARTESIAN_POINT('Ctrl Pts',(1.94952575850196,1.,-3.46139661060959));
#50547=CARTESIAN_POINT('Ctrl Pts',(1.95088147859876,1.,-3.4688525897419));
#50548=CARTESIAN_POINT('Ctrl Pts',(1.95219722189878,1.,-3.47632820495926));
#50549=CARTESIAN_POINT('Ctrl Pts',(1.95347412486316,1.,-3.48382414832649));
#50550=CARTESIAN_POINT('Ctrl Pts',(1.95471236969653,1.,-3.49133956289154));
#50551=CARTESIAN_POINT('Ctrl Pts',(1.9559115382367,1.,-3.49887263575602));
#50552=CARTESIAN_POINT('Ctrl Pts',(1.95707099606513,1.,-3.50642124159913));
#50553=CARTESIAN_POINT('Ctrl Pts',(1.95819025316768,1.,-3.51398354617773));
#50554=CARTESIAN_POINT('Ctrl Pts',(1.95926936324436,1.,-3.52155867431438));
#50555=CARTESIAN_POINT('Ctrl Pts',(1.96030879411534,1.,-3.52914648844289));
#50556=CARTESIAN_POINT('Ctrl Pts',(1.96130926212661,1.,-3.53674730625759));
#50557=CARTESIAN_POINT('Ctrl Pts',(1.96227157573058,1.,-3.54436163300425));
#50558=CARTESIAN_POINT('Ctrl Pts',(1.96319648628667,1.,-3.55198990600929));
#50559=CARTESIAN_POINT('Ctrl Pts',(1.96408450906868,1.,-3.55963218706201));
#50560=CARTESIAN_POINT('Ctrl Pts',(1.96493594634643,1.,-3.56728820357933));
#50561=CARTESIAN_POINT('Ctrl Pts',(1.96575096652857,1.,-3.57495748601088));
#50562=CARTESIAN_POINT('Ctrl Pts',(1.9665296668894,1.,-3.58263947663884));
#50563=CARTESIAN_POINT('Ctrl Pts',(1.96727213799507,1.,-3.5903336402273));
#50564=CARTESIAN_POINT('Ctrl Pts',(1.96797854118257,1.,-3.59803959819725));
#50565=CARTESIAN_POINT('Ctrl Pts',(1.96864911885775,1.,-3.60575714017676));
#50566=CARTESIAN_POINT('Ctrl Pts',(1.96928416040712,1.,-3.61348615496393));
#50567=CARTESIAN_POINT('Ctrl Pts',(1.96988398129888,1.,-3.62122658401722));
#50568=CARTESIAN_POINT('Ctrl Pts',(1.97044889850518,1.,-3.62897836973397));
#50569=CARTESIAN_POINT('Ctrl Pts',(1.97097920454698,1.,-3.63674139590853));
#50570=CARTESIAN_POINT('Ctrl Pts',(1.97147515441539,1.,-3.64451546724222));
#50571=CARTESIAN_POINT('Ctrl Pts',(1.97193697240645,1.,-3.65230034717364));
#50572=CARTESIAN_POINT('Ctrl Pts',(1.97236485439317,1.,-3.66009578166865));
#50573=CARTESIAN_POINT('Ctrl Pts',(1.9727589719863,1.,-3.66790152751984));
#50574=CARTESIAN_POINT('Ctrl Pts',(1.97311947678035,1.,-3.67571738106175));
#50575=CARTESIAN_POINT('Ctrl Pts',(1.9734465030363,1.,-3.68354319913416));
#50576=CARTESIAN_POINT('Ctrl Pts',(1.97374016224397,1.,-3.69137888597855));
#50577=CARTESIAN_POINT('Ctrl Pts',(1.97394846382288,1.,-3.69765528558292));
#50578=CARTESIAN_POINT('Ctrl Pts',(1.97408973726149,1.,-3.70236698911837));
#50579=CARTESIAN_POINT('Ctrl Pts',(1.974177276451,1.,-3.7055100813194));
#50580=CARTESIAN_POINT('Ctrl Pts',(1.97421938526992,1.,-3.70708211654725));
#50581=CARTESIAN_POINT('Origin',(1.97421938526992,0.,-3.70708211654725));
#50582=CARTESIAN_POINT('',(1.83867539237861,1.,-3.77614523045147));
#50583=CARTESIAN_POINT('Origin',(0.,0.,0.));
#50584=CARTESIAN_POINT('',(2.03660101169564,1.,-3.14877060440425));
#50585=CARTESIAN_POINT('Origin',(0.,1.,0.));
#50586=CARTESIAN_POINT('Ctrl Pts',(2.03660101169564,1.,-3.14877060440425));
#50587=CARTESIAN_POINT('Ctrl Pts',(2.03660101169564,0.666666666666667,-3.14877060440425));
#50588=CARTESIAN_POINT('Ctrl Pts',(2.03660101169564,0.333333333333333,-3.14877060440425));
#50589=CARTESIAN_POINT('Ctrl Pts',(2.03660101169564,-0.333333333333333,
-3.14877060440425));
#50590=CARTESIAN_POINT('Ctrl Pts',(2.03660101169564,-0.666666666666667,
-3.14877060440425));
#50591=CARTESIAN_POINT('Ctrl Pts',(2.03660101169564,-1.,-3.14877060440425));
#50592=CARTESIAN_POINT('Ctrl Pts',(2.40675750623143,-1.,-3.44202241512147));
#50593=CARTESIAN_POINT('Ctrl Pts',(2.40675750623143,1.,-3.44202241512147));
#50594=CARTESIAN_POINT('Ctrl Pts',(2.40537592959345,-1.,-3.44127120683402));
#50595=CARTESIAN_POINT('Ctrl Pts',(2.40537592959345,1.,-3.44127120683402));
#50596=CARTESIAN_POINT('Ctrl Pts',(2.40261515590099,-1.,-3.43976627485223));
#50597=CARTESIAN_POINT('Ctrl Pts',(2.40261515590099,1.,-3.43976627485223));
#50598=CARTESIAN_POINT('Ctrl Pts',(2.39848113411428,-1.,-3.43750133066037));
#50599=CARTESIAN_POINT('Ctrl Pts',(2.39848113411428,1.,-3.43750133066037));
#50600=CARTESIAN_POINT('Ctrl Pts',(2.39298338805823,-1.,-3.43446630680436));
#50601=CARTESIAN_POINT('Ctrl Pts',(2.39298338805823,1.,-3.43446630680436));
#50602=CARTESIAN_POINT('Ctrl Pts',(2.38613505844641,-1.,-3.43064732714472));
#50603=CARTESIAN_POINT('Ctrl Pts',(2.38613505844641,1.,-3.43064732714472));
#50604=CARTESIAN_POINT('Ctrl Pts',(2.37931067029517,-1.,-3.42680309755241));
#50605=CARTESIAN_POINT('Ctrl Pts',(2.37931067029517,1.,-3.42680309755241));
#50606=CARTESIAN_POINT('Ctrl Pts',(2.37251035954351,-1.,-3.42293356216595));
#50607=CARTESIAN_POINT('Ctrl Pts',(2.37251035954351,1.,-3.42293356216595));
#50608=CARTESIAN_POINT('Ctrl Pts',(2.36573431470313,-1.,-3.41903866635384));
#50609=CARTESIAN_POINT('Ctrl Pts',(2.36573431470313,1.,-3.41903866635384));
#50610=CARTESIAN_POINT('Ctrl Pts',(2.35898278606449,-1.,-3.4151183675076));
#50611=CARTESIAN_POINT('Ctrl Pts',(2.35898278606449,1.,-3.4151183675076));
#50612=CARTESIAN_POINT('Ctrl Pts',(2.35225606823649,-1.,-3.41117262313464));
#50613=CARTESIAN_POINT('Ctrl Pts',(2.35225606823649,1.,-3.41117262313464));
#50614=CARTESIAN_POINT('Ctrl Pts',(2.34555447648901,-1.,-3.40720137403888));
#50615=CARTESIAN_POINT('Ctrl Pts',(2.34555447648901,1.,-3.40720137403888));
#50616=CARTESIAN_POINT('Ctrl Pts',(2.33887832342715,-1.,-3.40320452776646));
#50617=CARTESIAN_POINT('Ctrl Pts',(2.33887832342715,1.,-3.40320452776646));
#50618=CARTESIAN_POINT('Ctrl Pts',(2.33222789882601,-1.,-3.39918194578115));
#50619=CARTESIAN_POINT('Ctrl Pts',(2.33222789882601,1.,-3.39918194578115));
#50620=CARTESIAN_POINT('Ctrl Pts',(2.32560343902683,-1.,-3.39513342020045));
#50621=CARTESIAN_POINT('Ctrl Pts',(2.32560343902683,1.,-3.39513342020045));
#50622=CARTESIAN_POINT('Ctrl Pts',(2.31900513925627,-1.,-3.39105869475112));
#50623=CARTESIAN_POINT('Ctrl Pts',(2.31900513925627,1.,-3.39105869475112));
#50624=CARTESIAN_POINT('Ctrl Pts',(2.31243319489505,-1.,-3.38695751492659));
#50625=CARTESIAN_POINT('Ctrl Pts',(2.31243319489505,1.,-3.38695751492659));
#50626=CARTESIAN_POINT('Ctrl Pts',(2.30588783640389,-1.,-3.38282967336676));
#50627=CARTESIAN_POINT('Ctrl Pts',(2.30588783640389,1.,-3.38282967336676));
#50628=CARTESIAN_POINT('Ctrl Pts',(2.29936936127588,-1.,-3.37867504959382));
#50629=CARTESIAN_POINT('Ctrl Pts',(2.29936936127588,1.,-3.37867504959382));
#50630=CARTESIAN_POINT('Ctrl Pts',(2.2928781800731,-1.,-3.37449367172707));
#50631=CARTESIAN_POINT('Ctrl Pts',(2.2928781800731,1.,-3.37449367172707));
#50632=CARTESIAN_POINT('Ctrl Pts',(2.28641481081045,-1.,-3.37028570206357));
#50633=CARTESIAN_POINT('Ctrl Pts',(2.28641481081045,1.,-3.37028570206357));
#50634=CARTESIAN_POINT('Ctrl Pts',(2.27997979457968,-1.,-3.36605130712978));
#50635=CARTESIAN_POINT('Ctrl Pts',(2.27997979457968,1.,-3.36605130712978));
#50636=CARTESIAN_POINT('Ctrl Pts',(2.27357362620902,-1.,-3.36179055004369));
#50637=CARTESIAN_POINT('Ctrl Pts',(2.27357362620902,1.,-3.36179055004369));
#50638=CARTESIAN_POINT('Ctrl Pts',(2.26719668579921,-1.,-3.35750328523077));
#50639=CARTESIAN_POINT('Ctrl Pts',(2.26719668579921,1.,-3.35750328523077));
#50640=CARTESIAN_POINT('Ctrl Pts',(2.26084915222484,-1.,-3.35318902552676));
#50641=CARTESIAN_POINT('Ctrl Pts',(2.26084915222484,1.,-3.35318902552676));
#50642=CARTESIAN_POINT('Ctrl Pts',(2.25453097693524,-1.,-3.34884690292342));
#50643=CARTESIAN_POINT('Ctrl Pts',(2.25453097693524,1.,-3.34884690292342));
#50644=CARTESIAN_POINT('Ctrl Pts',(2.24824207678287,-1.,-3.34447596770768));
#50645=CARTESIAN_POINT('Ctrl Pts',(2.24824207678287,1.,-3.34447596770768));
#50646=CARTESIAN_POINT('Ctrl Pts',(2.24198249391437,-1.,-3.34007543738044));
#50647=CARTESIAN_POINT('Ctrl Pts',(2.24198249391437,1.,-3.34007543738044));
#50648=CARTESIAN_POINT('Ctrl Pts',(2.23575256328809,-1.,-3.33564495756478));
#50649=CARTESIAN_POINT('Ctrl Pts',(2.23575256328809,1.,-3.33564495756478));
#50650=CARTESIAN_POINT('Ctrl Pts',(2.22955308907221,-1.,-3.33118487773593));
#50651=CARTESIAN_POINT('Ctrl Pts',(2.22955308907221,1.,-3.33118487773593));
#50652=CARTESIAN_POINT('Ctrl Pts',(2.22338548312758,-1.,-3.32669646722871));
#50653=CARTESIAN_POINT('Ctrl Pts',(2.22338548312758,1.,-3.32669646722871));
#50654=CARTESIAN_POINT('Ctrl Pts',(2.21725135110889,-1.,-3.32218125618955));
#50655=CARTESIAN_POINT('Ctrl Pts',(2.21725135110889,1.,-3.32218125618955));
#50656=CARTESIAN_POINT('Ctrl Pts',(2.21115211847872,-1.,-3.31764044024231));
#50657=CARTESIAN_POINT('Ctrl Pts',(2.21115211847872,1.,-3.31764044024231));
#50658=CARTESIAN_POINT('Ctrl Pts',(2.20508863150608,-1.,-3.3130742460895));
#50659=CARTESIAN_POINT('Ctrl Pts',(2.20508863150608,1.,-3.3130742460895));
#50660=CARTESIAN_POINT('Ctrl Pts',(2.19906078949924,-1.,-3.30848134694597));
#50661=CARTESIAN_POINT('Ctrl Pts',(2.19906078949924,1.,-3.30848134694597));
#50662=CARTESIAN_POINT('Ctrl Pts',(2.19306710376112,-1.,-3.30385816281831));
#50663=CARTESIAN_POINT('Ctrl Pts',(2.19306710376112,1.,-3.30385816281831));
#50664=CARTESIAN_POINT('Ctrl Pts',(2.18710556500325,-1.,-3.29920022557635));
#50665=CARTESIAN_POINT('Ctrl Pts',(2.18710556500325,1.,-3.29920022557635));
#50666=CARTESIAN_POINT('Ctrl Pts',(2.18117455557062,-1.,-3.29450361500484));
#50667=CARTESIAN_POINT('Ctrl Pts',(2.18117455557062,1.,-3.29450361500484));
#50668=CARTESIAN_POINT('Ctrl Pts',(2.17527380048422,-1.,-3.28976645712566));
#50669=CARTESIAN_POINT('Ctrl Pts',(2.17527380048422,1.,-3.28976645712566));
#50670=CARTESIAN_POINT('Ctrl Pts',(2.16940517773459,-1.,-3.2849901997973));
#50671=CARTESIAN_POINT('Ctrl Pts',(2.16940517773459,1.,-3.2849901997973));
#50672=CARTESIAN_POINT('Ctrl Pts',(2.16357391934434,-1.,-3.28018150841414));
#50673=CARTESIAN_POINT('Ctrl Pts',(2.16357391934434,1.,-3.28018150841414));
#50674=CARTESIAN_POINT('Ctrl Pts',(2.15778690038359,-1.,-3.27534954469206));
#50675=CARTESIAN_POINT('Ctrl Pts',(2.15778690038359,1.,-3.27534954469206));
#50676=CARTESIAN_POINT('Ctrl Pts',(2.15205043199818,-1.,-3.27050245897244));
#50677=CARTESIAN_POINT('Ctrl Pts',(2.15205043199818,1.,-3.27050245897244));
#50678=CARTESIAN_POINT('Ctrl Pts',(2.14636805295663,-1.,-3.26564388189764));
#50679=CARTESIAN_POINT('Ctrl Pts',(2.14636805295663,1.,-3.26564388189764));
#50680=CARTESIAN_POINT('Ctrl Pts',(2.14073870754257,-1.,-3.26077002641868));
#50681=CARTESIAN_POINT('Ctrl Pts',(2.14073870754257,1.,-3.26077002641868));
#50682=CARTESIAN_POINT('Ctrl Pts',(2.13515375878786,-1.,-3.25586495065027));
#50683=CARTESIAN_POINT('Ctrl Pts',(2.13515375878786,1.,-3.25586495065027));
#50684=CARTESIAN_POINT('Ctrl Pts',(2.1296002839681,-1.,-3.25090574493994));
#50685=CARTESIAN_POINT('Ctrl Pts',(2.1296002839681,1.,-3.25090574493994));
#50686=CARTESIAN_POINT('Ctrl Pts',(2.12406646410943,-1.,-3.24587102613347));
#50687=CARTESIAN_POINT('Ctrl Pts',(2.12406646410943,1.,-3.24587102613347));
#50688=CARTESIAN_POINT('Ctrl Pts',(2.11854673326972,-1.,-3.24074905517282));
#50689=CARTESIAN_POINT('Ctrl Pts',(2.11854673326972,1.,-3.24074905517282));
#50690=CARTESIAN_POINT('Ctrl Pts',(2.11304604021784,-1.,-3.23554444767115));
#50691=CARTESIAN_POINT('Ctrl Pts',(2.11304604021784,1.,-3.23554444767115));
#50692=CARTESIAN_POINT('Ctrl Pts',(2.1075869964248,-1.,-3.23028945793334));
#50693=CARTESIAN_POINT('Ctrl Pts',(2.1075869964248,1.,-3.23028945793334));
#50694=CARTESIAN_POINT('Ctrl Pts',(2.10220384298533,-1.,-3.22503437553496));
#50695=CARTESIAN_POINT('Ctrl Pts',(2.10220384298533,1.,-3.22503437553496));
#50696=CARTESIAN_POINT('Ctrl Pts',(2.09692958434933,-1.,-3.21982707347067));
#50697=CARTESIAN_POINT('Ctrl Pts',(2.09692958434933,1.,-3.21982707347067));
#50698=CARTESIAN_POINT('Ctrl Pts',(2.0917841946046,-1.,-3.2146942960168));
#50699=CARTESIAN_POINT('Ctrl Pts',(2.0917841946046,1.,-3.2146942960168));
#50700=CARTESIAN_POINT('Ctrl Pts',(2.08676465517435,-1.,-3.20962575845433));
#50701=CARTESIAN_POINT('Ctrl Pts',(2.08676465517435,1.,-3.20962575845433));
#50702=CARTESIAN_POINT('Ctrl Pts',(2.08182850370816,-1.,-3.20454818630635));
#50703=CARTESIAN_POINT('Ctrl Pts',(2.08182850370816,1.,-3.20454818630635));
#50704=CARTESIAN_POINT('Ctrl Pts',(2.0769044187063,-1.,-3.19934132835879));
#50705=CARTESIAN_POINT('Ctrl Pts',(2.0769044187063,1.,-3.19934132835879));
#50706=CARTESIAN_POINT('Ctrl Pts',(2.07192253497765,-1.,-3.19388465568113));
#50707=CARTESIAN_POINT('Ctrl Pts',(2.07192253497765,1.,-3.19388465568113));
#50708=CARTESIAN_POINT('Ctrl Pts',(2.06684062744065,-1.,-3.18809755562297));
#50709=CARTESIAN_POINT('Ctrl Pts',(2.06684062744065,1.,-3.18809755562297));
#50710=CARTESIAN_POINT('Ctrl Pts',(2.06166849827143,-1.,-3.18197692964677));
#50711=CARTESIAN_POINT('Ctrl Pts',(2.06166849827143,1.,-3.18197692964677));
#50712=CARTESIAN_POINT('Ctrl Pts',(2.05650186773279,-1.,-3.17564906975592));
#50713=CARTESIAN_POINT('Ctrl Pts',(2.05650186773279,1.,-3.17564906975592));
#50714=CARTESIAN_POINT('Ctrl Pts',(2.05151770247452,-1.,-3.16936341689859));
#50715=CARTESIAN_POINT('Ctrl Pts',(2.05151770247452,1.,-3.16936341689859));
#50716=CARTESIAN_POINT('Ctrl Pts',(2.0469333124766,-1.,-3.16343165059235));
#50717=CARTESIAN_POINT('Ctrl Pts',(2.0469333124766,1.,-3.16343165059235));
#50718=CARTESIAN_POINT('Ctrl Pts',(2.04297406404132,-1.,-3.15817983946525));
#50719=CARTESIAN_POINT('Ctrl Pts',(2.04297406404132,1.,-3.15817983946525));
#50720=CARTESIAN_POINT('Ctrl Pts',(2.03984073791432,-1.,-3.1538999167466));
#50721=CARTESIAN_POINT('Ctrl Pts',(2.03984073791432,1.,-3.1538999167466));
#50722=CARTESIAN_POINT('Ctrl Pts',(2.03766932526171,-1.,-3.15079010635326));
#50723=CARTESIAN_POINT('Ctrl Pts',(2.03766932526171,1.,-3.15079010635326));
#50724=CARTESIAN_POINT('Ctrl Pts',(2.03675273048882,-1.,-3.14931281967585));
#50725=CARTESIAN_POINT('Ctrl Pts',(2.03675273048882,1.,-3.14931281967585));
#50726=CARTESIAN_POINT('Ctrl Pts',(2.03653654935384,-1.,-3.14878756590499));
#50727=CARTESIAN_POINT('Ctrl Pts',(2.03653654935384,1.,-3.14878756590499));
#50728=CARTESIAN_POINT('Ctrl Pts',(2.036601737578,-1.,-3.14869618937139));
#50729=CARTESIAN_POINT('Ctrl Pts',(2.036601737578,1.,-3.14869618937139));
#50730=CARTESIAN_POINT('Ctrl Pts',(2.03668666247593,-1.,-3.1487152044751));
#50731=CARTESIAN_POINT('Ctrl Pts',(2.03668666247593,1.,-3.1487152044751));
#50732=CARTESIAN_POINT('',(2.40675750623143,1.,-3.44202241512147));
#50733=CARTESIAN_POINT('Ctrl Pts',(2.40675750623143,1.,-3.44202241512147));
#50734=CARTESIAN_POINT('Ctrl Pts',(2.40537592959345,1.,-3.44127120683402));
#50735=CARTESIAN_POINT('Ctrl Pts',(2.40261515590099,1.,-3.43976627485223));
#50736=CARTESIAN_POINT('Ctrl Pts',(2.39848113411428,1.,-3.43750133066037));
#50737=CARTESIAN_POINT('Ctrl Pts',(2.39298338805823,1.,-3.43446630680436));
#50738=CARTESIAN_POINT('Ctrl Pts',(2.38613505844641,1.,-3.43064732714472));
#50739=CARTESIAN_POINT('Ctrl Pts',(2.37931067029517,1.,-3.42680309755241));
#50740=CARTESIAN_POINT('Ctrl Pts',(2.37251035954351,1.,-3.42293356216595));
#50741=CARTESIAN_POINT('Ctrl Pts',(2.36573431470313,1.,-3.41903866635384));
#50742=CARTESIAN_POINT('Ctrl Pts',(2.35898278606449,1.,-3.4151183675076));
#50743=CARTESIAN_POINT('Ctrl Pts',(2.35225606823649,1.,-3.41117262313464));
#50744=CARTESIAN_POINT('Ctrl Pts',(2.34555447648901,1.,-3.40720137403888));
#50745=CARTESIAN_POINT('Ctrl Pts',(2.33887832342715,1.,-3.40320452776646));
#50746=CARTESIAN_POINT('Ctrl Pts',(2.33222789882601,1.,-3.39918194578115));
#50747=CARTESIAN_POINT('Ctrl Pts',(2.32560343902683,1.,-3.39513342020045));
#50748=CARTESIAN_POINT('Ctrl Pts',(2.31900513925627,1.,-3.39105869475112));
#50749=CARTESIAN_POINT('Ctrl Pts',(2.31243319489505,1.,-3.38695751492659));
#50750=CARTESIAN_POINT('Ctrl Pts',(2.30588783640389,1.,-3.38282967336676));
#50751=CARTESIAN_POINT('Ctrl Pts',(2.29936936127588,1.,-3.37867504959382));
#50752=CARTESIAN_POINT('Ctrl Pts',(2.2928781800731,1.,-3.37449367172707));
#50753=CARTESIAN_POINT('Ctrl Pts',(2.28641481081045,1.,-3.37028570206357));
#50754=CARTESIAN_POINT('Ctrl Pts',(2.27997979457968,1.,-3.36605130712978));
#50755=CARTESIAN_POINT('Ctrl Pts',(2.27357362620902,1.,-3.36179055004369));
#50756=CARTESIAN_POINT('Ctrl Pts',(2.26719668579921,1.,-3.35750328523077));
#50757=CARTESIAN_POINT('Ctrl Pts',(2.26084915222484,1.,-3.35318902552676));
#50758=CARTESIAN_POINT('Ctrl Pts',(2.25453097693524,1.,-3.34884690292342));
#50759=CARTESIAN_POINT('Ctrl Pts',(2.24824207678287,1.,-3.34447596770768));
#50760=CARTESIAN_POINT('Ctrl Pts',(2.24198249391437,1.,-3.34007543738044));
#50761=CARTESIAN_POINT('Ctrl Pts',(2.23575256328809,1.,-3.33564495756478));
#50762=CARTESIAN_POINT('Ctrl Pts',(2.22955308907221,1.,-3.33118487773593));
#50763=CARTESIAN_POINT('Ctrl Pts',(2.22338548312758,1.,-3.32669646722871));
#50764=CARTESIAN_POINT('Ctrl Pts',(2.21725135110889,1.,-3.32218125618955));
#50765=CARTESIAN_POINT('Ctrl Pts',(2.21115211847872,1.,-3.31764044024231));
#50766=CARTESIAN_POINT('Ctrl Pts',(2.20508863150608,1.,-3.3130742460895));
#50767=CARTESIAN_POINT('Ctrl Pts',(2.19906078949924,1.,-3.30848134694597));
#50768=CARTESIAN_POINT('Ctrl Pts',(2.19306710376112,1.,-3.30385816281831));
#50769=CARTESIAN_POINT('Ctrl Pts',(2.18710556500325,1.,-3.29920022557635));
#50770=CARTESIAN_POINT('Ctrl Pts',(2.18117455557062,1.,-3.29450361500484));
#50771=CARTESIAN_POINT('Ctrl Pts',(2.17527380048422,1.,-3.28976645712566));
#50772=CARTESIAN_POINT('Ctrl Pts',(2.16940517773459,1.,-3.2849901997973));
#50773=CARTESIAN_POINT('Ctrl Pts',(2.16357391934434,1.,-3.28018150841414));
#50774=CARTESIAN_POINT('Ctrl Pts',(2.15778690038359,1.,-3.27534954469206));
#50775=CARTESIAN_POINT('Ctrl Pts',(2.15205043199818,1.,-3.27050245897244));
#50776=CARTESIAN_POINT('Ctrl Pts',(2.14636805295663,1.,-3.26564388189764));
#50777=CARTESIAN_POINT('Ctrl Pts',(2.14073870754257,1.,-3.26077002641868));
#50778=CARTESIAN_POINT('Ctrl Pts',(2.13515375878786,1.,-3.25586495065027));
#50779=CARTESIAN_POINT('Ctrl Pts',(2.1296002839681,1.,-3.25090574493994));
#50780=CARTESIAN_POINT('Ctrl Pts',(2.12406646410943,1.,-3.24587102613347));
#50781=CARTESIAN_POINT('Ctrl Pts',(2.11854673326972,1.,-3.24074905517282));
#50782=CARTESIAN_POINT('Ctrl Pts',(2.11304604021784,1.,-3.23554444767115));
#50783=CARTESIAN_POINT('Ctrl Pts',(2.1075869964248,1.,-3.23028945793334));
#50784=CARTESIAN_POINT('Ctrl Pts',(2.10220384298533,1.,-3.22503437553496));
#50785=CARTESIAN_POINT('Ctrl Pts',(2.09692958434933,1.,-3.21982707347067));
#50786=CARTESIAN_POINT('Ctrl Pts',(2.0917841946046,1.,-3.2146942960168));
#50787=CARTESIAN_POINT('Ctrl Pts',(2.08676465517435,1.,-3.20962575845433));
#50788=CARTESIAN_POINT('Ctrl Pts',(2.08182850370816,1.,-3.20454818630635));
#50789=CARTESIAN_POINT('Ctrl Pts',(2.0769044187063,1.,-3.19934132835879));
#50790=CARTESIAN_POINT('Ctrl Pts',(2.07192253497765,1.,-3.19388465568113));
#50791=CARTESIAN_POINT('Ctrl Pts',(2.06684062744065,1.,-3.18809755562297));
#50792=CARTESIAN_POINT('Ctrl Pts',(2.06166849827143,1.,-3.18197692964677));
#50793=CARTESIAN_POINT('Ctrl Pts',(2.05650186773279,1.,-3.17564906975592));
#50794=CARTESIAN_POINT('Ctrl Pts',(2.05151770247452,1.,-3.16936341689859));
#50795=CARTESIAN_POINT('Ctrl Pts',(2.0469333124766,1.,-3.16343165059235));
#50796=CARTESIAN_POINT('Ctrl Pts',(2.04297406404132,1.,-3.15817983946525));
#50797=CARTESIAN_POINT('Ctrl Pts',(2.03984073791432,1.,-3.1538999167466));
#50798=CARTESIAN_POINT('Ctrl Pts',(2.03783225496023,1.,-3.15102344775396));
#50799=CARTESIAN_POINT('Ctrl Pts',(2.03693188810614,1.,-3.14959882629936));
#50800=CARTESIAN_POINT('Ctrl Pts',(2.03663974554941,1.,-3.14901193669147));
#50801=CARTESIAN_POINT('Ctrl Pts',(2.03659701539175,1.,-3.1488193908823));
#50802=CARTESIAN_POINT('Ctrl Pts',(2.03660101169564,1.,-3.14877060440425));
#50803=CARTESIAN_POINT('',(2.40675750623143,0.,-3.44202241512147));
#50804=CARTESIAN_POINT('Ctrl Pts',(2.36523532225181,-1.,-2.91001063062876));
#50805=CARTESIAN_POINT('Ctrl Pts',(2.36523532225181,1.,-2.91001063062876));
#50806=CARTESIAN_POINT('Ctrl Pts',(2.36524348105112,-1.,-2.90992398626211));
#50807=CARTESIAN_POINT('Ctrl Pts',(2.36524348105112,1.,-2.90992398626211));
#50808=CARTESIAN_POINT('Ctrl Pts',(2.36535052956938,-1.,-2.90989022548032));
#50809=CARTESIAN_POINT('Ctrl Pts',(2.36535052956938,1.,-2.90989022548032));
#50810=CARTESIAN_POINT('Ctrl Pts',(2.36578327194741,-1.,-2.91025813830041));
#50811=CARTESIAN_POINT('Ctrl Pts',(2.36578327194741,1.,-2.91025813830041));
#50812=CARTESIAN_POINT('Ctrl Pts',(2.36690501170627,-1.,-2.9115863784204));
#50813=CARTESIAN_POINT('Ctrl Pts',(2.36690501170627,1.,-2.9115863784204));
#50814=CARTESIAN_POINT('Ctrl Pts',(2.36919161373173,-1.,-2.9146124988314));
#50815=CARTESIAN_POINT('Ctrl Pts',(2.36919161373173,1.,-2.9146124988314));
#50816=CARTESIAN_POINT('Ctrl Pts',(2.37229381109821,-1.,-2.91891503791411));
#50817=CARTESIAN_POINT('Ctrl Pts',(2.37229381109821,1.,-2.91891503791411));
#50818=CARTESIAN_POINT('Ctrl Pts',(2.3760651052403,-1.,-2.92430340582608));
#50819=CARTESIAN_POINT('Ctrl Pts',(2.3760651052403,1.,-2.92430340582608));
#50820=CARTESIAN_POINT('Ctrl Pts',(2.38028989582073,-1.,-2.93049643640206));
#50821=CARTESIAN_POINT('Ctrl Pts',(2.38028989582073,1.,-2.93049643640206));
#50822=CARTESIAN_POINT('Ctrl Pts',(2.38472771516311,-1.,-2.93717903280391));
#50823=CARTESIAN_POINT('Ctrl Pts',(2.38472771516311,1.,-2.93717903280391));
#50824=CARTESIAN_POINT('Ctrl Pts',(2.38914929090759,-1.,-2.94404820669076));
#50825=CARTESIAN_POINT('Ctrl Pts',(2.38914929090759,1.,-2.94404820669076));
#50826=CARTESIAN_POINT('Ctrl Pts',(2.39337207631667,-1.,-2.95085857128439));
#50827=CARTESIAN_POINT('Ctrl Pts',(2.39337207631667,1.,-2.95085857128439));
#50828=CARTESIAN_POINT('Ctrl Pts',(2.39730553974516,-1.,-2.95748006482942));
#50829=CARTESIAN_POINT('Ctrl Pts',(2.39730553974516,1.,-2.95748006482942));
#50830=CARTESIAN_POINT('Ctrl Pts',(2.4009556571164,-1.,-2.96390432240312));
#50831=CARTESIAN_POINT('Ctrl Pts',(2.4009556571164,1.,-2.96390432240312));
#50832=CARTESIAN_POINT('Ctrl Pts',(2.40438604734919,-1.,-2.9701964131236));
#50833=CARTESIAN_POINT('Ctrl Pts',(2.40438604734919,1.,-2.9701964131236));
#50834=CARTESIAN_POINT('Ctrl Pts',(2.40768975073713,-1.,-2.97646002822422));
#50835=CARTESIAN_POINT('Ctrl Pts',(2.40768975073713,1.,-2.97646002822422));
#50836=CARTESIAN_POINT('Ctrl Pts',(2.41095909342571,-1.,-2.98280015815107));
#50837=CARTESIAN_POINT('Ctrl Pts',(2.41095909342571,1.,-2.98280015815107));
#50838=CARTESIAN_POINT('Ctrl Pts',(2.41425064199586,-1.,-2.98927983005796));
#50839=CARTESIAN_POINT('Ctrl Pts',(2.41425064199586,1.,-2.98927983005796));
#50840=CARTESIAN_POINT('Ctrl Pts',(2.41757324500514,-1.,-2.99590509293503));
#50841=CARTESIAN_POINT('Ctrl Pts',(2.41757324500514,1.,-2.99590509293503));
#50842=CARTESIAN_POINT('Ctrl Pts',(2.42090763946779,-1.,-3.00264868585996));
#50843=CARTESIAN_POINT('Ctrl Pts',(2.42090763946779,1.,-3.00264868585996));
#50844=CARTESIAN_POINT('Ctrl Pts',(2.42421849439613,-1.,-3.00946442616659));
#50845=CARTESIAN_POINT('Ctrl Pts',(2.42421849439613,1.,-3.00946442616659));
#50846=CARTESIAN_POINT('Ctrl Pts',(2.42746856264168,-1.,-3.01630420830504));
#50847=CARTESIAN_POINT('Ctrl Pts',(2.42746856264168,1.,-3.01630420830504));
#50848=CARTESIAN_POINT('Ctrl Pts',(2.43063415586637,-1.,-3.02313656036004));
#50849=CARTESIAN_POINT('Ctrl Pts',(2.43063415586637,1.,-3.02313656036004));
#50850=CARTESIAN_POINT('Ctrl Pts',(2.43371241361488,-1.,-3.02995534946978));
#50851=CARTESIAN_POINT('Ctrl Pts',(2.43371241361488,1.,-3.02995534946978));
#50852=CARTESIAN_POINT('Ctrl Pts',(2.43671278042414,-1.,-3.03676949672822));
#50853=CARTESIAN_POINT('Ctrl Pts',(2.43671278042414,1.,-3.03676949672822));
#50854=CARTESIAN_POINT('Ctrl Pts',(2.43965194061857,-1.,-3.04359685040555));
#50855=CARTESIAN_POINT('Ctrl Pts',(2.43965194061857,1.,-3.04359685040555));
#50856=CARTESIAN_POINT('Ctrl Pts',(2.44254768923105,-1.,-3.05045678021504));
#50857=CARTESIAN_POINT('Ctrl Pts',(2.44254768923105,1.,-3.05045678021504));
#50858=CARTESIAN_POINT('Ctrl Pts',(2.44541251892556,-1.,-3.05736242671506));
#50859=CARTESIAN_POINT('Ctrl Pts',(2.44541251892556,1.,-3.05736242671506));
#50860=CARTESIAN_POINT('Ctrl Pts',(2.44824970516543,-1.,-3.06431596421405));
#50861=CARTESIAN_POINT('Ctrl Pts',(2.44824970516543,1.,-3.06431596421405));
#50862=CARTESIAN_POINT('Ctrl Pts',(2.45105688854422,-1.,-3.07131290521297));
#50863=CARTESIAN_POINT('Ctrl Pts',(2.45105688854422,1.,-3.07131290521297));
#50864=CARTESIAN_POINT('Ctrl Pts',(2.4538282678779,-1.,-3.07834472886139));
#50865=CARTESIAN_POINT('Ctrl Pts',(2.4538282678779,1.,-3.07834472886139));
#50866=CARTESIAN_POINT('Ctrl Pts',(2.45655725437039,-1.,-3.08540206545315));
#50867=CARTESIAN_POINT('Ctrl Pts',(2.45655725437039,1.,-3.08540206545315));
#50868=CARTESIAN_POINT('Ctrl Pts',(2.4592391256388,-1.,-3.09247787931887));
#50869=CARTESIAN_POINT('Ctrl Pts',(2.4592391256388,1.,-3.09247787931887));
#50870=CARTESIAN_POINT('Ctrl Pts',(2.46187308501884,-1.,-3.09956993697052));
#50871=CARTESIAN_POINT('Ctrl Pts',(2.46187308501884,1.,-3.09956993697052));
#50872=CARTESIAN_POINT('Ctrl Pts',(2.46446082979646,-1.,-3.1066790790198));
#50873=CARTESIAN_POINT('Ctrl Pts',(2.46446082979646,1.,-3.1066790790198));
#50874=CARTESIAN_POINT('Ctrl Pts',(2.46700558843506,-1.,-3.11380805536122));
#50875=CARTESIAN_POINT('Ctrl Pts',(2.46700558843506,1.,-3.11380805536122));
#50876=CARTESIAN_POINT('Ctrl Pts',(2.46951098947469,-1.,-3.12096015766983));
#50877=CARTESIAN_POINT('Ctrl Pts',(2.46951098947469,1.,-3.12096015766983));
#50878=CARTESIAN_POINT('Ctrl Pts',(2.47197997765871,-1.,-3.12813790805952));
#50879=CARTESIAN_POINT('Ctrl Pts',(2.47197997765871,1.,-3.12813790805952));
#50880=CARTESIAN_POINT('Ctrl Pts',(2.47441378371932,-1.,-3.13534181229295));
#50881=CARTESIAN_POINT('Ctrl Pts',(2.47441378371932,1.,-3.13534181229295));
#50882=CARTESIAN_POINT('Ctrl Pts',(2.47681245356109,-1.,-3.1425709954655));
#50883=CARTESIAN_POINT('Ctrl Pts',(2.47681245356109,1.,-3.1425709954655));
#50884=CARTESIAN_POINT('Ctrl Pts',(2.47917529057029,-1.,-3.14982373241352));
#50885=CARTESIAN_POINT('Ctrl Pts',(2.47917529057029,1.,-3.14982373241352));
#50886=CARTESIAN_POINT('Ctrl Pts',(2.48150133566571,-1.,-3.15709802322739));
#50887=CARTESIAN_POINT('Ctrl Pts',(2.48150133566571,1.,-3.15709802322739));
#50888=CARTESIAN_POINT('Ctrl Pts',(2.48378981792725,-1.,-3.16439213290161));
#50889=CARTESIAN_POINT('Ctrl Pts',(2.48378981792725,1.,-3.16439213290161));
#50890=CARTESIAN_POINT('Ctrl Pts',(2.48604065348587,-1.,-3.17170518863313));
#50891=CARTESIAN_POINT('Ctrl Pts',(2.48604065348587,1.,-3.17170518863313));
#50892=CARTESIAN_POINT('Ctrl Pts',(2.48825428288201,-1.,-3.17903698136622));
#50893=CARTESIAN_POINT('Ctrl Pts',(2.48825428288201,1.,-3.17903698136622));
#50894=CARTESIAN_POINT('Ctrl Pts',(2.49043146334059,-1.,-3.18638771282266));
#50895=CARTESIAN_POINT('Ctrl Pts',(2.49043146334059,1.,-3.18638771282266));
#50896=CARTESIAN_POINT('Ctrl Pts',(2.49257307239848,-1.,-3.19375775555798));
#50897=CARTESIAN_POINT('Ctrl Pts',(2.49257307239848,1.,-3.19375775555798));
#50898=CARTESIAN_POINT('Ctrl Pts',(2.49467992057755,-1.,-3.20114742397588));
#50899=CARTESIAN_POINT('Ctrl Pts',(2.49467992057755,1.,-3.20114742397588));
#50900=CARTESIAN_POINT('Ctrl Pts',(2.4967525264737,-1.,-3.20855669849836));
#50901=CARTESIAN_POINT('Ctrl Pts',(2.4967525264737,1.,-3.20855669849836));
#50902=CARTESIAN_POINT('Ctrl Pts',(2.4987911459939,-1.,-3.21598526261286));
#50903=CARTESIAN_POINT('Ctrl Pts',(2.4987911459939,1.,-3.21598526261286));
#50904=CARTESIAN_POINT('Ctrl Pts',(2.50079587201957,-1.,-3.22343262620503));
#50905=CARTESIAN_POINT('Ctrl Pts',(2.50079587201957,1.,-3.22343262620503));
#50906=CARTESIAN_POINT('Ctrl Pts',(2.50276671338111,-1.,-3.23089822320646));
#50907=CARTESIAN_POINT('Ctrl Pts',(2.50276671338111,1.,-3.23089822320646));
#50908=CARTESIAN_POINT('Ctrl Pts',(2.5047036758003,-1.,-3.23838151080319));
#50909=CARTESIAN_POINT('Ctrl Pts',(2.5047036758003,1.,-3.23838151080319));
#50910=CARTESIAN_POINT('Ctrl Pts',(2.506606859405,-1.,-3.24588208983849));
#50911=CARTESIAN_POINT('Ctrl Pts',(2.506606859405,1.,-3.24588208983849));
#50912=CARTESIAN_POINT('Ctrl Pts',(2.50847647070723,-1.,-3.25339971460982));
#50913=CARTESIAN_POINT('Ctrl Pts',(2.50847647070723,1.,-3.25339971460982));
#50914=CARTESIAN_POINT('Ctrl Pts',(2.51031277813486,-1.,-3.26093423001434));
#50915=CARTESIAN_POINT('Ctrl Pts',(2.51031277813486,1.,-3.26093423001434));
#50916=CARTESIAN_POINT('Ctrl Pts',(2.51211608411423,-1.,-3.26848552888116));
#50917=CARTESIAN_POINT('Ctrl Pts',(2.51211608411423,1.,-3.26848552888116));
#50918=CARTESIAN_POINT('Ctrl Pts',(2.513886692704,-1.,-3.27605350473142));
#50919=CARTESIAN_POINT('Ctrl Pts',(2.513886692704,1.,-3.27605350473142));
#50920=CARTESIAN_POINT('Ctrl Pts',(2.51562487464514,-1.,-3.28363799702982));
#50921=CARTESIAN_POINT('Ctrl Pts',(2.51562487464514,1.,-3.28363799702982));
#50922=CARTESIAN_POINT('Ctrl Pts',(2.51733085123797,-1.,-3.2912387729927));
#50923=CARTESIAN_POINT('Ctrl Pts',(2.51733085123797,1.,-3.2912387729927));
#50924=CARTESIAN_POINT('Ctrl Pts',(2.51900480701068,-1.,-3.29885556388353));
#50925=CARTESIAN_POINT('Ctrl Pts',(2.51900480701068,1.,-3.29885556388353));
#50926=CARTESIAN_POINT('Ctrl Pts',(2.52064689568511,-1.,-3.30648808815443));
#50927=CARTESIAN_POINT('Ctrl Pts',(2.52064689568511,1.,-3.30648808815443));
#50928=CARTESIAN_POINT('Ctrl Pts',(2.52225724871313,-1.,-3.31413607874645));
#50929=CARTESIAN_POINT('Ctrl Pts',(2.52225724871313,1.,-3.31413607874645));
#50930=CARTESIAN_POINT('Ctrl Pts',(2.5238359839626,-1.,-3.32179931078699));
#50931=CARTESIAN_POINT('Ctrl Pts',(2.5238359839626,1.,-3.32179931078699));
#50932=CARTESIAN_POINT('Ctrl Pts',(2.52538321164634,-1.,-3.32947762187533));
#50933=CARTESIAN_POINT('Ctrl Pts',(2.52538321164634,1.,-3.32947762187533));
#50934=CARTESIAN_POINT('Ctrl Pts',(2.52689902690158,-1.,-3.33717089999103));
#50935=CARTESIAN_POINT('Ctrl Pts',(2.52689902690158,1.,-3.33717089999103));
#50936=CARTESIAN_POINT('Ctrl Pts',(2.52808660915689,-1.,-3.34333744115511));
#50937=CARTESIAN_POINT('Ctrl Pts',(2.52808660915689,1.,-3.34333744115511));
#50938=CARTESIAN_POINT('Ctrl Pts',(2.52896321610703,-1.,-3.34796903576663));
#50939=CARTESIAN_POINT('Ctrl Pts',(2.52896321610703,1.,-3.34796903576663));
#50940=CARTESIAN_POINT('Ctrl Pts',(2.5295413654909,-1.,-3.35105973714072));
#50941=CARTESIAN_POINT('Ctrl Pts',(2.5295413654909,1.,-3.35105973714072));
#50942=CARTESIAN_POINT('Ctrl Pts',(2.52982887637028,-1.,-3.35260583073571));
#50943=CARTESIAN_POINT('Ctrl Pts',(2.52982887637028,1.,-3.35260583073571));
#50944=CARTESIAN_POINT('',(2.36531447826073,1.,-2.90994629141676));
#50945=CARTESIAN_POINT('Ctrl Pts',(2.36531447826073,-1.,-2.90994629141676));
#50946=CARTESIAN_POINT('Ctrl Pts',(2.36531447826073,-0.666666666666667,
-2.90994629141676));
#50947=CARTESIAN_POINT('Ctrl Pts',(2.36531447826073,-0.333333333333333,
-2.90994629141676));
#50948=CARTESIAN_POINT('Ctrl Pts',(2.36531447826073,0.333333333333333,-2.90994629141676));
#50949=CARTESIAN_POINT('Ctrl Pts',(2.36531447826074,0.666666666666667,-2.90994629141676));
#50950=CARTESIAN_POINT('Ctrl Pts',(2.36531447826074,1.,-2.90994629141676));
#50951=CARTESIAN_POINT('',(2.52982887637028,1.,-3.35260583073571));
#50952=CARTESIAN_POINT('',(2.52982887637028,0.,-3.35260583073571));
#50953=CARTESIAN_POINT('Ctrl Pts',(2.36531447826073,1.,-2.90994629141676));
#50954=CARTESIAN_POINT('Ctrl Pts',(2.36536211188453,1.,-2.90995756655606));
#50955=CARTESIAN_POINT('Ctrl Pts',(2.36553202948613,1.,-2.91005770527719));
#50956=CARTESIAN_POINT('Ctrl Pts',(2.36599991765749,1.,-2.91051690822156));
#50957=CARTESIAN_POINT('Ctrl Pts',(2.36707658451664,1.,-2.91181344022548));
#50958=CARTESIAN_POINT('Ctrl Pts',(2.36919161373173,1.,-2.9146124988314));
#50959=CARTESIAN_POINT('Ctrl Pts',(2.37229381109821,1.,-2.91891503791411));
#50960=CARTESIAN_POINT('Ctrl Pts',(2.3760651052403,1.,-2.92430340582608));
#50961=CARTESIAN_POINT('Ctrl Pts',(2.38028989582073,1.,-2.93049643640206));
#50962=CARTESIAN_POINT('Ctrl Pts',(2.38472771516311,1.,-2.93717903280391));
#50963=CARTESIAN_POINT('Ctrl Pts',(2.38914929090759,1.,-2.94404820669076));
#50964=CARTESIAN_POINT('Ctrl Pts',(2.39337207631667,1.,-2.95085857128439));
#50965=CARTESIAN_POINT('Ctrl Pts',(2.39730553974516,1.,-2.95748006482942));
#50966=CARTESIAN_POINT('Ctrl Pts',(2.4009556571164,1.,-2.96390432240312));
#50967=CARTESIAN_POINT('Ctrl Pts',(2.40438604734919,1.,-2.9701964131236));
#50968=CARTESIAN_POINT('Ctrl Pts',(2.40768975073713,1.,-2.97646002822422));
#50969=CARTESIAN_POINT('Ctrl Pts',(2.41095909342571,1.,-2.98280015815107));
#50970=CARTESIAN_POINT('Ctrl Pts',(2.41425064199586,1.,-2.98927983005796));
#50971=CARTESIAN_POINT('Ctrl Pts',(2.41757324500514,1.,-2.99590509293503));
#50972=CARTESIAN_POINT('Ctrl Pts',(2.42090763946779,1.,-3.00264868585996));
#50973=CARTESIAN_POINT('Ctrl Pts',(2.42421849439613,1.,-3.00946442616659));
#50974=CARTESIAN_POINT('Ctrl Pts',(2.42746856264168,1.,-3.01630420830504));
#50975=CARTESIAN_POINT('Ctrl Pts',(2.43063415586637,1.,-3.02313656036004));
#50976=CARTESIAN_POINT('Ctrl Pts',(2.43371241361488,1.,-3.02995534946978));
#50977=CARTESIAN_POINT('Ctrl Pts',(2.43671278042414,1.,-3.03676949672822));
#50978=CARTESIAN_POINT('Ctrl Pts',(2.43965194061857,1.,-3.04359685040555));
#50979=CARTESIAN_POINT('Ctrl Pts',(2.44254768923105,1.,-3.05045678021504));
#50980=CARTESIAN_POINT('Ctrl Pts',(2.44541251892556,1.,-3.05736242671506));
#50981=CARTESIAN_POINT('Ctrl Pts',(2.44824970516543,1.,-3.06431596421405));
#50982=CARTESIAN_POINT('Ctrl Pts',(2.45105688854422,1.,-3.07131290521297));
#50983=CARTESIAN_POINT('Ctrl Pts',(2.4538282678779,1.,-3.07834472886139));
#50984=CARTESIAN_POINT('Ctrl Pts',(2.45655725437039,1.,-3.08540206545315));
#50985=CARTESIAN_POINT('Ctrl Pts',(2.4592391256388,1.,-3.09247787931887));
#50986=CARTESIAN_POINT('Ctrl Pts',(2.46187308501884,1.,-3.09956993697052));
#50987=CARTESIAN_POINT('Ctrl Pts',(2.46446082979646,1.,-3.1066790790198));
#50988=CARTESIAN_POINT('Ctrl Pts',(2.46700558843506,1.,-3.11380805536122));
#50989=CARTESIAN_POINT('Ctrl Pts',(2.46951098947469,1.,-3.12096015766983));
#50990=CARTESIAN_POINT('Ctrl Pts',(2.47197997765871,1.,-3.12813790805952));
#50991=CARTESIAN_POINT('Ctrl Pts',(2.47441378371932,1.,-3.13534181229295));
#50992=CARTESIAN_POINT('Ctrl Pts',(2.47681245356109,1.,-3.1425709954655));
#50993=CARTESIAN_POINT('Ctrl Pts',(2.47917529057029,1.,-3.14982373241352));
#50994=CARTESIAN_POINT('Ctrl Pts',(2.48150133566571,1.,-3.15709802322739));
#50995=CARTESIAN_POINT('Ctrl Pts',(2.48378981792725,1.,-3.16439213290161));
#50996=CARTESIAN_POINT('Ctrl Pts',(2.48604065348587,1.,-3.17170518863313));
#50997=CARTESIAN_POINT('Ctrl Pts',(2.48825428288201,1.,-3.17903698136622));
#50998=CARTESIAN_POINT('Ctrl Pts',(2.49043146334059,1.,-3.18638771282266));
#50999=CARTESIAN_POINT('Ctrl Pts',(2.49257307239848,1.,-3.19375775555798));
#51000=CARTESIAN_POINT('Ctrl Pts',(2.49467992057755,1.,-3.20114742397588));
#51001=CARTESIAN_POINT('Ctrl Pts',(2.4967525264737,1.,-3.20855669849836));
#51002=CARTESIAN_POINT('Ctrl Pts',(2.4987911459939,1.,-3.21598526261286));
#51003=CARTESIAN_POINT('Ctrl Pts',(2.50079587201957,1.,-3.22343262620503));
#51004=CARTESIAN_POINT('Ctrl Pts',(2.50276671338111,1.,-3.23089822320646));
#51005=CARTESIAN_POINT('Ctrl Pts',(2.5047036758003,1.,-3.23838151080319));
#51006=CARTESIAN_POINT('Ctrl Pts',(2.506606859405,1.,-3.24588208983849));
#51007=CARTESIAN_POINT('Ctrl Pts',(2.50847647070723,1.,-3.25339971460982));
#51008=CARTESIAN_POINT('Ctrl Pts',(2.51031277813486,1.,-3.26093423001434));
#51009=CARTESIAN_POINT('Ctrl Pts',(2.51211608411423,1.,-3.26848552888116));
#51010=CARTESIAN_POINT('Ctrl Pts',(2.513886692704,1.,-3.27605350473142));
#51011=CARTESIAN_POINT('Ctrl Pts',(2.51562487464514,1.,-3.28363799702982));
#51012=CARTESIAN_POINT('Ctrl Pts',(2.51733085123797,1.,-3.2912387729927));
#51013=CARTESIAN_POINT('Ctrl Pts',(2.51900480701068,1.,-3.29885556388353));
#51014=CARTESIAN_POINT('Ctrl Pts',(2.52064689568511,1.,-3.30648808815443));
#51015=CARTESIAN_POINT('Ctrl Pts',(2.52225724871313,1.,-3.31413607874645));
#51016=CARTESIAN_POINT('Ctrl Pts',(2.5238359839626,1.,-3.32179931078699));
#51017=CARTESIAN_POINT('Ctrl Pts',(2.52538321164634,1.,-3.32947762187533));
#51018=CARTESIAN_POINT('Ctrl Pts',(2.52689902690158,1.,-3.33717089999103));
#51019=CARTESIAN_POINT('Ctrl Pts',(2.52808660915689,1.,-3.34333744115511));
#51020=CARTESIAN_POINT('Ctrl Pts',(2.52896321610703,1.,-3.34796903576663));
#51021=CARTESIAN_POINT('Ctrl Pts',(2.5295413654909,1.,-3.35105973714072));
#51022=CARTESIAN_POINT('Ctrl Pts',(2.52982887637028,1.,-3.35260583073571));
#51023=CARTESIAN_POINT('Origin',(2.52982887637028,0.,-3.35260583073571));
#51024=CARTESIAN_POINT('',(2.40675750623143,1.,-3.44202241512147));
#51025=CARTESIAN_POINT('Origin',(0.,0.,0.));
#51026=CARTESIAN_POINT('',(2.50410331873042,1.,-2.79140942341378));
#51027=CARTESIAN_POINT('Origin',(0.,1.,0.));
#51028=CARTESIAN_POINT('Ctrl Pts',(2.50410331873042,1.,-2.79140942341378));
#51029=CARTESIAN_POINT('Ctrl Pts',(2.50410331873042,0.666666666666667,-2.79140942341378));
#51030=CARTESIAN_POINT('Ctrl Pts',(2.50410331873042,0.333333333333333,-2.79140942341378));
#51031=CARTESIAN_POINT('Ctrl Pts',(2.50410331873042,-0.333333333333333,
-2.79140942341378));
#51032=CARTESIAN_POINT('Ctrl Pts',(2.50410331873042,-0.666666666666667,
-2.79140942341378));
#51033=CARTESIAN_POINT('Ctrl Pts',(2.50410331873042,-1.,-2.79140942341378));
#51034=CARTESIAN_POINT('Ctrl Pts',(2.91557726271063,-1.,-3.02314558451372));
#51035=CARTESIAN_POINT('Ctrl Pts',(2.91557726271063,1.,-3.02314558451372));
#51036=CARTESIAN_POINT('Ctrl Pts',(2.91409518070707,-1.,-3.02261975104912));
#51037=CARTESIAN_POINT('Ctrl Pts',(2.91409518070707,1.,-3.02261975104912));
#51038=CARTESIAN_POINT('Ctrl Pts',(2.91113297349052,-1.,-3.02156522743299));
#51039=CARTESIAN_POINT('Ctrl Pts',(2.91113297349052,1.,-3.02156522743299));
#51040=CARTESIAN_POINT('Ctrl Pts',(2.90669553303902,-1.,-3.01997487194926));
#51041=CARTESIAN_POINT('Ctrl Pts',(2.90669553303902,1.,-3.01997487194926));
#51042=CARTESIAN_POINT('Ctrl Pts',(2.90079069102661,-1.,-3.01783725123646));
#51043=CARTESIAN_POINT('Ctrl Pts',(2.90079069102661,1.,-3.01783725123646));
#51044=CARTESIAN_POINT('Ctrl Pts',(2.8934292556764,-1.,-3.01513660433291));
#51045=CARTESIAN_POINT('Ctrl Pts',(2.8934292556764,1.,-3.01513660433291));
#51046=CARTESIAN_POINT('Ctrl Pts',(2.88608751706796,-1.,-3.01240727309568));
#51047=CARTESIAN_POINT('Ctrl Pts',(2.88608751706796,1.,-3.01240727309568));
#51048=CARTESIAN_POINT('Ctrl Pts',(2.87876560072799,-1.,-3.0096491810855));
#51049=CARTESIAN_POINT('Ctrl Pts',(2.87876560072799,1.,-3.0096491810855));
#51050=CARTESIAN_POINT('Ctrl Pts',(2.87146368430104,-1.,-3.00686224485374));
#51051=CARTESIAN_POINT('Ctrl Pts',(2.87146368430104,1.,-3.00686224485374));
#51052=CARTESIAN_POINT('Ctrl Pts',(2.86418200833065,-1.,-3.00404638316245));
#51053=CARTESIAN_POINT('Ctrl Pts',(2.86418200833065,1.,-3.00404638316245));
#51054=CARTESIAN_POINT('Ctrl Pts',(2.85692085715129,-1.,-3.0012015079552));
#51055=CARTESIAN_POINT('Ctrl Pts',(2.85692085715129,1.,-3.0012015079552));
#51056=CARTESIAN_POINT('Ctrl Pts',(2.84968053289104,-1.,-2.99832751144566));
#51057=CARTESIAN_POINT('Ctrl Pts',(2.84968053289104,1.,-2.99832751144566));
#51058=CARTESIAN_POINT('Ctrl Pts',(2.84246132984334,-1.,-2.995424253416));
#51059=CARTESIAN_POINT('Ctrl Pts',(2.84246132984334,1.,-2.995424253416));
#51060=CARTESIAN_POINT('Ctrl Pts',(2.83526351254383,-1.,-2.99249155170479));
#51061=CARTESIAN_POINT('Ctrl Pts',(2.83526351254383,1.,-2.99249155170479));
#51062=CARTESIAN_POINT('Ctrl Pts',(2.82808728190402,-1.,-2.98952916401699));
#51063=CARTESIAN_POINT('Ctrl Pts',(2.82808728190402,1.,-2.98952916401699));
#51064=CARTESIAN_POINT('Ctrl Pts',(2.82093279065704,-1.,-2.98653680669434));
#51065=CARTESIAN_POINT('Ctrl Pts',(2.82093279065704,1.,-2.98653680669434));
#51066=CARTESIAN_POINT('Ctrl Pts',(2.81380019196454,-1.,-2.9835141977994));
#51067=CARTESIAN_POINT('Ctrl Pts',(2.81380019196454,1.,-2.9835141977994));
#51068=CARTESIAN_POINT('Ctrl Pts',(2.80668968101162,-1.,-2.98046109647299));
#51069=CARTESIAN_POINT('Ctrl Pts',(2.80668968101162,1.,-2.98046109647299));
#51070=CARTESIAN_POINT('Ctrl Pts',(2.79960153278186,-1.,-2.97737733718242));
#51071=CARTESIAN_POINT('Ctrl Pts',(2.79960153278186,1.,-2.97737733718242));
#51072=CARTESIAN_POINT('Ctrl Pts',(2.79253615718147,-1.,-2.97426288347475));
#51073=CARTESIAN_POINT('Ctrl Pts',(2.79253615718147,1.,-2.97426288347475));
#51074=CARTESIAN_POINT('Ctrl Pts',(2.78549409123657,-1.,-2.97111781461349));
#51075=CARTESIAN_POINT('Ctrl Pts',(2.78549409123657,1.,-2.97111781461349));
#51076=CARTESIAN_POINT('Ctrl Pts',(2.77847589542767,-1.,-2.9679422104295));
#51077=CARTESIAN_POINT('Ctrl Pts',(2.77847589542767,1.,-2.9679422104295));
#51078=CARTESIAN_POINT('Ctrl Pts',(2.77148206836464,-1.,-2.96473605585548));
#51079=CARTESIAN_POINT('Ctrl Pts',(2.77148206836464,1.,-2.96473605585548));
#51080=CARTESIAN_POINT('Ctrl Pts',(2.76451296269571,-1.,-2.96149914764832));
#51081=CARTESIAN_POINT('Ctrl Pts',(2.76451296269571,1.,-2.96149914764832));
#51082=CARTESIAN_POINT('Ctrl Pts',(2.75756867888393,-1.,-2.9582309766594));
#51083=CARTESIAN_POINT('Ctrl Pts',(2.75756867888393,1.,-2.9582309766594));
#51084=CARTESIAN_POINT('Ctrl Pts',(2.75064903318996,-1.,-2.95493069316211));
#51085=CARTESIAN_POINT('Ctrl Pts',(2.75064903318996,1.,-2.95493069316211));
#51086=CARTESIAN_POINT('Ctrl Pts',(2.7437537949221,-1.,-2.95159737214305));
#51087=CARTESIAN_POINT('Ctrl Pts',(2.7437537949221,1.,-2.95159737214305));
#51088=CARTESIAN_POINT('Ctrl Pts',(2.73688288329825,-1.,-2.94823023414381));
#51089=CARTESIAN_POINT('Ctrl Pts',(2.73688288329825,1.,-2.94823023414381));
#51090=CARTESIAN_POINT('Ctrl Pts',(2.73003657371613,-1.,-2.94482887675139));
#51091=CARTESIAN_POINT('Ctrl Pts',(2.73003657371613,1.,-2.94482887675139));
#51092=CARTESIAN_POINT('Ctrl Pts',(2.72321571511322,-1.,-2.94139351933882));
#51093=CARTESIAN_POINT('Ctrl Pts',(2.72321571511322,1.,-2.94139351933882));
#51094=CARTESIAN_POINT('Ctrl Pts',(2.71642190053575,-1.,-2.93792519474955));
#51095=CARTESIAN_POINT('Ctrl Pts',(2.71642190053575,1.,-2.93792519474955));
#51096=CARTESIAN_POINT('Ctrl Pts',(2.70965695523776,-1.,-2.93442516311168));
#51097=CARTESIAN_POINT('Ctrl Pts',(2.70965695523776,1.,-2.93442516311168));
#51098=CARTESIAN_POINT('Ctrl Pts',(2.70292247416881,-1.,-2.93089438233746));
#51099=CARTESIAN_POINT('Ctrl Pts',(2.70292247416881,1.,-2.93089438233746));
#51100=CARTESIAN_POINT('Ctrl Pts',(2.69621932864302,-1.,-2.92733294395268));
#51101=CARTESIAN_POINT('Ctrl Pts',(2.69621932864302,1.,-2.92733294395268));
#51102=CARTESIAN_POINT('Ctrl Pts',(2.68954721165342,-1.,-2.92373955325876));
#51103=CARTESIAN_POINT('Ctrl Pts',(2.68954721165342,1.,-2.92373955325876));
#51104=CARTESIAN_POINT('Ctrl Pts',(2.68290409279689,-1.,-2.92011090722152));
#51105=CARTESIAN_POINT('Ctrl Pts',(2.68290409279689,1.,-2.92011090722152));
#51106=CARTESIAN_POINT('Ctrl Pts',(2.67628728855309,-1.,-2.91644290704281));
#51107=CARTESIAN_POINT('Ctrl Pts',(2.67628728855309,1.,-2.91644290704281));
#51108=CARTESIAN_POINT('Ctrl Pts',(2.66969458792627,-1.,-2.91273193382876));
#51109=CARTESIAN_POINT('Ctrl Pts',(2.66969458792627,1.,-2.91273193382876));
#51110=CARTESIAN_POINT('Ctrl Pts',(2.66312542616808,-1.,-2.90897617968921));
#51111=CARTESIAN_POINT('Ctrl Pts',(2.66312542616808,1.,-2.90897617968921));
#51112=CARTESIAN_POINT('Ctrl Pts',(2.65658188464287,-1.,-2.90517678087467));
#51113=CARTESIAN_POINT('Ctrl Pts',(2.65658188464287,1.,-2.90517678087467));
#51114=CARTESIAN_POINT('Ctrl Pts',(2.65007017365576,-1.,-2.90133950224879));
#51115=CARTESIAN_POINT('Ctrl Pts',(2.65007017365576,1.,-2.90133950224879));
#51116=CARTESIAN_POINT('Ctrl Pts',(2.64359851684146,-1.,-2.89747231723361));
#51117=CARTESIAN_POINT('Ctrl Pts',(2.64359851684146,1.,-2.89747231723361));
#51118=CARTESIAN_POINT('Ctrl Pts',(2.63717442263944,-1.,-2.89358228854557));
#51119=CARTESIAN_POINT('Ctrl Pts',(2.63717442263944,1.,-2.89358228854557));
#51120=CARTESIAN_POINT('Ctrl Pts',(2.63080195420771,-1.,-2.88967244854243));
#51121=CARTESIAN_POINT('Ctrl Pts',(2.63080195420771,1.,-2.88967244854243));
#51122=CARTESIAN_POINT('Ctrl Pts',(2.62447947640253,-1.,-2.88573922195049));
#51123=CARTESIAN_POINT('Ctrl Pts',(2.62447947640253,1.,-2.88573922195049));
#51124=CARTESIAN_POINT('Ctrl Pts',(2.61819596473087,-1.,-2.88176821427502));
#51125=CARTESIAN_POINT('Ctrl Pts',(2.61819596473087,1.,-2.88176821427502));
#51126=CARTESIAN_POINT('Ctrl Pts',(2.61193507170928,-1.,-2.87773881947885));
#51127=CARTESIAN_POINT('Ctrl Pts',(2.61193507170928,1.,-2.87773881947885));
#51128=CARTESIAN_POINT('Ctrl Pts',(2.6056817788128,-1.,-2.87363176656475));
#51129=CARTESIAN_POINT('Ctrl Pts',(2.6056817788128,1.,-2.87363176656475));
#51130=CARTESIAN_POINT('Ctrl Pts',(2.59942875223202,-1.,-2.86943633170712));
#51131=CARTESIAN_POINT('Ctrl Pts',(2.59942875223202,1.,-2.86943633170712));
#51132=CARTESIAN_POINT('Ctrl Pts',(2.59318160184921,-1.,-2.86515629953528));
#51133=CARTESIAN_POINT('Ctrl Pts',(2.59318160184921,1.,-2.86515629953528));
#51134=CARTESIAN_POINT('Ctrl Pts',(2.5869677064356,-1.,-2.86081999003668));
#51135=CARTESIAN_POINT('Ctrl Pts',(2.5869677064356,1.,-2.86081999003668));
#51136=CARTESIAN_POINT('Ctrl Pts',(2.58082875254407,-1.,-2.85647171715147));
#51137=CARTESIAN_POINT('Ctrl Pts',(2.58082875254407,1.,-2.85647171715147));
#51138=CARTESIAN_POINT('Ctrl Pts',(2.57480482727128,-1.,-2.85215360144483));
#51139=CARTESIAN_POINT('Ctrl Pts',(2.57480482727128,1.,-2.85215360144483));
#51140=CARTESIAN_POINT('Ctrl Pts',(2.56891984251743,-1.,-2.84788893329091));
#51141=CARTESIAN_POINT('Ctrl Pts',(2.56891984251743,1.,-2.84788893329091));
#51142=CARTESIAN_POINT('Ctrl Pts',(2.56316920798489,-1.,-2.84366802680211));
#51143=CARTESIAN_POINT('Ctrl Pts',(2.56316920798489,1.,-2.84366802680211));
#51144=CARTESIAN_POINT('Ctrl Pts',(2.55749952145165,-1.,-2.83942515220699));
#51145=CARTESIAN_POINT('Ctrl Pts',(2.55749952145165,1.,-2.83942515220699));
#51146=CARTESIAN_POINT('Ctrl Pts',(2.55182152806964,-1.,-2.83505269592412));
#51147=CARTESIAN_POINT('Ctrl Pts',(2.55182152806964,1.,-2.83505269592412));
#51148=CARTESIAN_POINT('Ctrl Pts',(2.54604736792542,-1.,-2.83044254225794));
#51149=CARTESIAN_POINT('Ctrl Pts',(2.54604736792542,1.,-2.83044254225794));
#51150=CARTESIAN_POINT('Ctrl Pts',(2.54012272520141,-1.,-2.82552167649157));
#51151=CARTESIAN_POINT('Ctrl Pts',(2.54012272520141,1.,-2.82552167649157));
#51152=CARTESIAN_POINT('Ctrl Pts',(2.53405679667463,-1.,-2.82028550483744));
#51153=CARTESIAN_POINT('Ctrl Pts',(2.53405679667463,1.,-2.82028550483744));
#51154=CARTESIAN_POINT('Ctrl Pts',(2.52796388055457,-1.,-2.8148437904867));
#51155=CARTESIAN_POINT('Ctrl Pts',(2.52796388055457,1.,-2.8148437904867));
#51156=CARTESIAN_POINT('Ctrl Pts',(2.52205778589922,-1.,-2.80941521967234));
#51157=CARTESIAN_POINT('Ctrl Pts',(2.52205778589922,1.,-2.80941521967234));
#51158=CARTESIAN_POINT('Ctrl Pts',(2.51660190466067,-1.,-2.80427363984939));
#51159=CARTESIAN_POINT('Ctrl Pts',(2.51660190466067,1.,-2.80427363984939));
#51160=CARTESIAN_POINT('Ctrl Pts',(2.51186983687947,-1.,-2.79970585014308));
#51161=CARTESIAN_POINT('Ctrl Pts',(2.51186983687947,1.,-2.79970585014308));
#51162=CARTESIAN_POINT('Ctrl Pts',(2.50810555977564,-1.,-2.7959687805717));
#51163=CARTESIAN_POINT('Ctrl Pts',(2.50810555977564,1.,-2.7959687805717));
#51164=CARTESIAN_POINT('Ctrl Pts',(2.50547439929077,-1.,-2.79323694088143));
#51165=CARTESIAN_POINT('Ctrl Pts',(2.50547439929077,1.,-2.79323694088143));
#51166=CARTESIAN_POINT('Ctrl Pts',(2.50433799076945,-1.,-2.79192122906739));
#51167=CARTESIAN_POINT('Ctrl Pts',(2.50433799076945,1.,-2.79192122906739));
#51168=CARTESIAN_POINT('Ctrl Pts',(2.50404230339032,-1.,-2.79143626022225));
#51169=CARTESIAN_POINT('Ctrl Pts',(2.50404230339032,1.,-2.79143626022225));
#51170=CARTESIAN_POINT('Ctrl Pts',(2.50409239460011,-1.,-2.79133581100044));
#51171=CARTESIAN_POINT('Ctrl Pts',(2.50409239460011,1.,-2.79133581100044));
#51172=CARTESIAN_POINT('Ctrl Pts',(2.50417924854921,-1.,-2.79134130681569));
#51173=CARTESIAN_POINT('Ctrl Pts',(2.50417924854921,1.,-2.79134130681569));
#51174=CARTESIAN_POINT('',(2.91557726271063,1.,-3.02314558451372));
#51175=CARTESIAN_POINT('Ctrl Pts',(2.91557726271063,1.,-3.02314558451372));
#51176=CARTESIAN_POINT('Ctrl Pts',(2.91409518070707,1.,-3.02261975104912));
#51177=CARTESIAN_POINT('Ctrl Pts',(2.91113297349052,1.,-3.02156522743299));
#51178=CARTESIAN_POINT('Ctrl Pts',(2.90669553303902,1.,-3.01997487194926));
#51179=CARTESIAN_POINT('Ctrl Pts',(2.90079069102661,1.,-3.01783725123646));
#51180=CARTESIAN_POINT('Ctrl Pts',(2.8934292556764,1.,-3.01513660433291));
#51181=CARTESIAN_POINT('Ctrl Pts',(2.88608751706796,1.,-3.01240727309568));
#51182=CARTESIAN_POINT('Ctrl Pts',(2.87876560072799,1.,-3.0096491810855));
#51183=CARTESIAN_POINT('Ctrl Pts',(2.87146368430104,1.,-3.00686224485374));
#51184=CARTESIAN_POINT('Ctrl Pts',(2.86418200833065,1.,-3.00404638316245));
#51185=CARTESIAN_POINT('Ctrl Pts',(2.85692085715129,1.,-3.0012015079552));
#51186=CARTESIAN_POINT('Ctrl Pts',(2.84968053289104,1.,-2.99832751144566));
#51187=CARTESIAN_POINT('Ctrl Pts',(2.84246132984334,1.,-2.995424253416));
#51188=CARTESIAN_POINT('Ctrl Pts',(2.83526351254383,1.,-2.99249155170479));
#51189=CARTESIAN_POINT('Ctrl Pts',(2.82808728190402,1.,-2.98952916401699));
#51190=CARTESIAN_POINT('Ctrl Pts',(2.82093279065704,1.,-2.98653680669434));
#51191=CARTESIAN_POINT('Ctrl Pts',(2.81380019196454,1.,-2.9835141977994));
#51192=CARTESIAN_POINT('Ctrl Pts',(2.80668968101162,1.,-2.98046109647299));
#51193=CARTESIAN_POINT('Ctrl Pts',(2.79960153278186,1.,-2.97737733718242));
#51194=CARTESIAN_POINT('Ctrl Pts',(2.79253615718147,1.,-2.97426288347475));
#51195=CARTESIAN_POINT('Ctrl Pts',(2.78549409123657,1.,-2.97111781461349));
#51196=CARTESIAN_POINT('Ctrl Pts',(2.77847589542767,1.,-2.9679422104295));
#51197=CARTESIAN_POINT('Ctrl Pts',(2.77148206836464,1.,-2.96473605585548));
#51198=CARTESIAN_POINT('Ctrl Pts',(2.76451296269571,1.,-2.96149914764832));
#51199=CARTESIAN_POINT('Ctrl Pts',(2.75756867888393,1.,-2.9582309766594));
#51200=CARTESIAN_POINT('Ctrl Pts',(2.75064903318996,1.,-2.95493069316211));
#51201=CARTESIAN_POINT('Ctrl Pts',(2.7437537949221,1.,-2.95159737214305));
#51202=CARTESIAN_POINT('Ctrl Pts',(2.73688288329825,1.,-2.94823023414381));
#51203=CARTESIAN_POINT('Ctrl Pts',(2.73003657371613,1.,-2.94482887675139));
#51204=CARTESIAN_POINT('Ctrl Pts',(2.72321571511322,1.,-2.94139351933882));
#51205=CARTESIAN_POINT('Ctrl Pts',(2.71642190053575,1.,-2.93792519474955));
#51206=CARTESIAN_POINT('Ctrl Pts',(2.70965695523776,1.,-2.93442516311168));
#51207=CARTESIAN_POINT('Ctrl Pts',(2.70292247416881,1.,-2.93089438233746));
#51208=CARTESIAN_POINT('Ctrl Pts',(2.69621932864302,1.,-2.92733294395268));
#51209=CARTESIAN_POINT('Ctrl Pts',(2.68954721165342,1.,-2.92373955325876));
#51210=CARTESIAN_POINT('Ctrl Pts',(2.68290409279689,1.,-2.92011090722152));
#51211=CARTESIAN_POINT('Ctrl Pts',(2.67628728855309,1.,-2.91644290704281));
#51212=CARTESIAN_POINT('Ctrl Pts',(2.66969458792627,1.,-2.91273193382876));
#51213=CARTESIAN_POINT('Ctrl Pts',(2.66312542616808,1.,-2.90897617968921));
#51214=CARTESIAN_POINT('Ctrl Pts',(2.65658188464287,1.,-2.90517678087467));
#51215=CARTESIAN_POINT('Ctrl Pts',(2.65007017365576,1.,-2.90133950224879));
#51216=CARTESIAN_POINT('Ctrl Pts',(2.64359851684146,1.,-2.89747231723361));
#51217=CARTESIAN_POINT('Ctrl Pts',(2.63717442263944,1.,-2.89358228854557));
#51218=CARTESIAN_POINT('Ctrl Pts',(2.63080195420771,1.,-2.88967244854243));
#51219=CARTESIAN_POINT('Ctrl Pts',(2.62447947640253,1.,-2.88573922195049));
#51220=CARTESIAN_POINT('Ctrl Pts',(2.61819596473087,1.,-2.88176821427502));
#51221=CARTESIAN_POINT('Ctrl Pts',(2.61193507170928,1.,-2.87773881947885));
#51222=CARTESIAN_POINT('Ctrl Pts',(2.6056817788128,1.,-2.87363176656475));
#51223=CARTESIAN_POINT('Ctrl Pts',(2.59942875223202,1.,-2.86943633170712));
#51224=CARTESIAN_POINT('Ctrl Pts',(2.59318160184921,1.,-2.86515629953528));
#51225=CARTESIAN_POINT('Ctrl Pts',(2.5869677064356,1.,-2.86081999003668));
#51226=CARTESIAN_POINT('Ctrl Pts',(2.58082875254407,1.,-2.85647171715147));
#51227=CARTESIAN_POINT('Ctrl Pts',(2.57480482727128,1.,-2.85215360144483));
#51228=CARTESIAN_POINT('Ctrl Pts',(2.56891984251743,1.,-2.84788893329091));
#51229=CARTESIAN_POINT('Ctrl Pts',(2.56316920798489,1.,-2.84366802680211));
#51230=CARTESIAN_POINT('Ctrl Pts',(2.55749952145165,1.,-2.83942515220699));
#51231=CARTESIAN_POINT('Ctrl Pts',(2.55182152806964,1.,-2.83505269592412));
#51232=CARTESIAN_POINT('Ctrl Pts',(2.54604736792542,1.,-2.83044254225794));
#51233=CARTESIAN_POINT('Ctrl Pts',(2.54012272520141,1.,-2.82552167649157));
#51234=CARTESIAN_POINT('Ctrl Pts',(2.53405679667463,1.,-2.82028550483744));
#51235=CARTESIAN_POINT('Ctrl Pts',(2.52796388055457,1.,-2.8148437904867));
#51236=CARTESIAN_POINT('Ctrl Pts',(2.52205778589922,1.,-2.80941521967234));
#51237=CARTESIAN_POINT('Ctrl Pts',(2.51660190466067,1.,-2.80427363984939));
#51238=CARTESIAN_POINT('Ctrl Pts',(2.51186983687947,1.,-2.79970585014308));
#51239=CARTESIAN_POINT('Ctrl Pts',(2.50810555977564,1.,-2.7959687805717));
#51240=CARTESIAN_POINT('Ctrl Pts',(2.50567182569153,1.,-2.79344192164204));
#51241=CARTESIAN_POINT('Ctrl Pts',(2.50455968395235,1.,-2.79217568804874));
#51242=CARTESIAN_POINT('Ctrl Pts',(2.50417932839344,1.,-2.79164172519039));
#51243=CARTESIAN_POINT('Ctrl Pts',(2.50410700351427,1.,-2.79145823440899));
#51244=CARTESIAN_POINT('Ctrl Pts',(2.50410331873043,1.,-2.79140942341378));
#51245=CARTESIAN_POINT('',(2.91557726271063,0.,-3.02314558451372));
#51246=CARTESIAN_POINT('Ctrl Pts',(2.79134130681569,-1.,-2.50417924854921));
#51247=CARTESIAN_POINT('Ctrl Pts',(2.79134130681569,1.,-2.50417924854921));
#51248=CARTESIAN_POINT('Ctrl Pts',(2.7913358110015,-1.,-2.50409239460108));
#51249=CARTESIAN_POINT('Ctrl Pts',(2.7913358110015,1.,-2.50409239460108));
#51250=CARTESIAN_POINT('Ctrl Pts',(2.79143626022503,-1.,-2.50404230339286));
#51251=CARTESIAN_POINT('Ctrl Pts',(2.79143626022503,1.,-2.50404230339286));
#51252=CARTESIAN_POINT('Ctrl Pts',(2.79192122907148,-1.,-2.5043379907732));
#51253=CARTESIAN_POINT('Ctrl Pts',(2.79192122907148,1.,-2.5043379907732));
#51254=CARTESIAN_POINT('Ctrl Pts',(2.7932369408851,-1.,-2.50547439929414));
#51255=CARTESIAN_POINT('Ctrl Pts',(2.7932369408851,1.,-2.50547439929414));
#51256=CARTESIAN_POINT('Ctrl Pts',(2.79596878057287,-1.,-2.50810555977671));
#51257=CARTESIAN_POINT('Ctrl Pts',(2.79596878057287,1.,-2.50810555977671));
#51258=CARTESIAN_POINT('Ctrl Pts',(2.79970585014168,-1.,-2.51186983687818));
#51259=CARTESIAN_POINT('Ctrl Pts',(2.79970585014168,1.,-2.51186983687818));
#51260=CARTESIAN_POINT('Ctrl Pts',(2.80427363984653,-1.,-2.51660190465805));
#51261=CARTESIAN_POINT('Ctrl Pts',(2.80427363984653,1.,-2.51660190465805));
#51262=CARTESIAN_POINT('Ctrl Pts',(2.80941521966941,-1.,-2.52205778589653));
#51263=CARTESIAN_POINT('Ctrl Pts',(2.80941521966941,1.,-2.52205778589653));
#51264=CARTESIAN_POINT('Ctrl Pts',(2.81484379048475,-1.,-2.52796388055278));
#51265=CARTESIAN_POINT('Ctrl Pts',(2.81484379048475,1.,-2.52796388055278));
#51266=CARTESIAN_POINT('Ctrl Pts',(2.82028550483689,-1.,-2.53405679667412));
#51267=CARTESIAN_POINT('Ctrl Pts',(2.82028550483689,1.,-2.53405679667412));
#51268=CARTESIAN_POINT('Ctrl Pts',(2.8255216764922,-1.,-2.54012272520199));
#51269=CARTESIAN_POINT('Ctrl Pts',(2.8255216764922,1.,-2.54012272520199));
#51270=CARTESIAN_POINT('Ctrl Pts',(2.83044254225917,-1.,-2.54604736792655));
#51271=CARTESIAN_POINT('Ctrl Pts',(2.83044254225917,1.,-2.54604736792655));
#51272=CARTESIAN_POINT('Ctrl Pts',(2.83505269592536,-1.,-2.55182152807077));
#51273=CARTESIAN_POINT('Ctrl Pts',(2.83505269592536,1.,-2.55182152807077));
#51274=CARTESIAN_POINT('Ctrl Pts',(2.83942515220782,-1.,-2.55749952145241));
#51275=CARTESIAN_POINT('Ctrl Pts',(2.83942515220782,1.,-2.55749952145241));
#51276=CARTESIAN_POINT('Ctrl Pts',(2.84366802680237,-1.,-2.56316920798513));
#51277=CARTESIAN_POINT('Ctrl Pts',(2.84366802680237,1.,-2.56316920798513));
#51278=CARTESIAN_POINT('Ctrl Pts',(2.84788893329067,-1.,-2.56891984251721));
#51279=CARTESIAN_POINT('Ctrl Pts',(2.84788893329067,1.,-2.56891984251721));
#51280=CARTESIAN_POINT('Ctrl Pts',(2.85215360144431,-1.,-2.57480482727081));
#51281=CARTESIAN_POINT('Ctrl Pts',(2.85215360144431,1.,-2.57480482727081));
#51282=CARTESIAN_POINT('Ctrl Pts',(2.85647171715092,-1.,-2.58082875254357));
#51283=CARTESIAN_POINT('Ctrl Pts',(2.85647171715092,1.,-2.58082875254357));
#51284=CARTESIAN_POINT('Ctrl Pts',(2.86081999003629,-1.,-2.58696770643524));
#51285=CARTESIAN_POINT('Ctrl Pts',(2.86081999003629,1.,-2.58696770643524));
#51286=CARTESIAN_POINT('Ctrl Pts',(2.86515629953513,-1.,-2.59318160184908));
#51287=CARTESIAN_POINT('Ctrl Pts',(2.86515629953513,1.,-2.59318160184908));
#51288=CARTESIAN_POINT('Ctrl Pts',(2.86943633170722,-1.,-2.5994287522321));
#51289=CARTESIAN_POINT('Ctrl Pts',(2.86943633170722,1.,-2.5994287522321));
#51290=CARTESIAN_POINT('Ctrl Pts',(2.87363176656501,-1.,-2.60568177881303));
#51291=CARTESIAN_POINT('Ctrl Pts',(2.87363176656501,1.,-2.60568177881303));
#51292=CARTESIAN_POINT('Ctrl Pts',(2.87773881947915,-1.,-2.61193507170955));
#51293=CARTESIAN_POINT('Ctrl Pts',(2.87773881947915,1.,-2.61193507170955));
#51294=CARTESIAN_POINT('Ctrl Pts',(2.88176821427525,-1.,-2.61819596473108));
#51295=CARTESIAN_POINT('Ctrl Pts',(2.88176821427525,1.,-2.61819596473108));
#51296=CARTESIAN_POINT('Ctrl Pts',(2.88573922195059,-1.,-2.62447947640262));
#51297=CARTESIAN_POINT('Ctrl Pts',(2.88573922195059,1.,-2.62447947640262));
#51298=CARTESIAN_POINT('Ctrl Pts',(2.88967244854239,-1.,-2.63080195420767));
#51299=CARTESIAN_POINT('Ctrl Pts',(2.88967244854239,1.,-2.63080195420767));
#51300=CARTESIAN_POINT('Ctrl Pts',(2.89358228854544,-1.,-2.63717442263932));
#51301=CARTESIAN_POINT('Ctrl Pts',(2.89358228854544,1.,-2.63717442263932));
#51302=CARTESIAN_POINT('Ctrl Pts',(2.89747231723345,-1.,-2.64359851684131));
#51303=CARTESIAN_POINT('Ctrl Pts',(2.89747231723345,1.,-2.64359851684131));
#51304=CARTESIAN_POINT('Ctrl Pts',(2.90133950224867,-1.,-2.65007017365564));
#51305=CARTESIAN_POINT('Ctrl Pts',(2.90133950224867,1.,-2.65007017365564));
#51306=CARTESIAN_POINT('Ctrl Pts',(2.90517678087461,-1.,-2.65658188464282));
#51307=CARTESIAN_POINT('Ctrl Pts',(2.90517678087461,1.,-2.65658188464282));
#51308=CARTESIAN_POINT('Ctrl Pts',(2.90897617968923,-1.,-2.6631254261681));
#51309=CARTESIAN_POINT('Ctrl Pts',(2.90897617968923,1.,-2.6631254261681));
#51310=CARTESIAN_POINT('Ctrl Pts',(2.91273193382882,-1.,-2.66969458792631));
#51311=CARTESIAN_POINT('Ctrl Pts',(2.91273193382882,1.,-2.66969458792631));
#51312=CARTESIAN_POINT('Ctrl Pts',(2.91644290704285,-1.,-2.67628728855312));
#51313=CARTESIAN_POINT('Ctrl Pts',(2.91644290704285,1.,-2.67628728855312));
#51314=CARTESIAN_POINT('Ctrl Pts',(2.92011090722152,-1.,-2.68290409279688));
#51315=CARTESIAN_POINT('Ctrl Pts',(2.92011090722152,1.,-2.68290409279688));
#51316=CARTESIAN_POINT('Ctrl Pts',(2.92373955325875,-1.,-2.68954721165339));
#51317=CARTESIAN_POINT('Ctrl Pts',(2.92373955325875,1.,-2.68954721165339));
#51318=CARTESIAN_POINT('Ctrl Pts',(2.92733294395267,-1.,-2.69621932864301));
#51319=CARTESIAN_POINT('Ctrl Pts',(2.92733294395267,1.,-2.69621932864301));
#51320=CARTESIAN_POINT('Ctrl Pts',(2.93089438233749,-1.,-2.70292247416885));
#51321=CARTESIAN_POINT('Ctrl Pts',(2.93089438233749,1.,-2.70292247416885));
#51322=CARTESIAN_POINT('Ctrl Pts',(2.93442516311179,-1.,-2.70965695523787));
#51323=CARTESIAN_POINT('Ctrl Pts',(2.93442516311179,1.,-2.70965695523787));
#51324=CARTESIAN_POINT('Ctrl Pts',(2.93792519474972,-1.,-2.71642190053592));
#51325=CARTESIAN_POINT('Ctrl Pts',(2.93792519474972,1.,-2.71642190053592));
#51326=CARTESIAN_POINT('Ctrl Pts',(2.94139351933897,-1.,-2.72321571511337));
#51327=CARTESIAN_POINT('Ctrl Pts',(2.94139351933897,1.,-2.72321571511337));
#51328=CARTESIAN_POINT('Ctrl Pts',(2.94482887675143,-1.,-2.73003657371617));
#51329=CARTESIAN_POINT('Ctrl Pts',(2.94482887675143,1.,-2.73003657371617));
#51330=CARTESIAN_POINT('Ctrl Pts',(2.94823023414364,-1.,-2.73688288329808));
#51331=CARTESIAN_POINT('Ctrl Pts',(2.94823023414364,1.,-2.73688288329808));
#51332=CARTESIAN_POINT('Ctrl Pts',(2.95159737214266,-1.,-2.74375379492172));
#51333=CARTESIAN_POINT('Ctrl Pts',(2.95159737214266,1.,-2.74375379492172));
#51334=CARTESIAN_POINT('Ctrl Pts',(2.95493069316161,-1.,-2.75064903318947));
#51335=CARTESIAN_POINT('Ctrl Pts',(2.95493069316161,1.,-2.75064903318947));
#51336=CARTESIAN_POINT('Ctrl Pts',(2.95823097665896,-1.,-2.7575686788835));
#51337=CARTESIAN_POINT('Ctrl Pts',(2.95823097665896,1.,-2.7575686788835));
#51338=CARTESIAN_POINT('Ctrl Pts',(2.96149914764818,-1.,-2.76451296269557));
#51339=CARTESIAN_POINT('Ctrl Pts',(2.96149914764818,1.,-2.76451296269557));
#51340=CARTESIAN_POINT('Ctrl Pts',(2.96473605585583,-1.,-2.77148206836498));
#51341=CARTESIAN_POINT('Ctrl Pts',(2.96473605585583,1.,-2.77148206836498));
#51342=CARTESIAN_POINT('Ctrl Pts',(2.96794221043036,-1.,-2.7784758954285));
#51343=CARTESIAN_POINT('Ctrl Pts',(2.96794221043036,1.,-2.7784758954285));
#51344=CARTESIAN_POINT('Ctrl Pts',(2.97111781461465,-1.,-2.78549409123769));
#51345=CARTESIAN_POINT('Ctrl Pts',(2.97111781461465,1.,-2.78549409123769));
#51346=CARTESIAN_POINT('Ctrl Pts',(2.9742628834758,-1.,-2.79253615718248));
#51347=CARTESIAN_POINT('Ctrl Pts',(2.9742628834758,1.,-2.79253615718248));
#51348=CARTESIAN_POINT('Ctrl Pts',(2.97737733718287,-1.,-2.7996015327823));
#51349=CARTESIAN_POINT('Ctrl Pts',(2.97737733718287,1.,-2.7996015327823));
#51350=CARTESIAN_POINT('Ctrl Pts',(2.98046109647241,-1.,-2.80668968101106));
#51351=CARTESIAN_POINT('Ctrl Pts',(2.98046109647241,1.,-2.80668968101106));
#51352=CARTESIAN_POINT('Ctrl Pts',(2.98351419779767,-1.,-2.81380019196286));
#51353=CARTESIAN_POINT('Ctrl Pts',(2.98351419779767,1.,-2.81380019196286));
#51354=CARTESIAN_POINT('Ctrl Pts',(2.9865368066918,-1.,-2.82093279065457));
#51355=CARTESIAN_POINT('Ctrl Pts',(2.9865368066918,1.,-2.82093279065457));
#51356=CARTESIAN_POINT('Ctrl Pts',(2.98952916401446,-1.,-2.82808728190157));
#51357=CARTESIAN_POINT('Ctrl Pts',(2.98952916401446,1.,-2.82808728190157));
#51358=CARTESIAN_POINT('Ctrl Pts',(2.99249155170339,-1.,-2.83526351254248));
#51359=CARTESIAN_POINT('Ctrl Pts',(2.99249155170339,1.,-2.83526351254248));
#51360=CARTESIAN_POINT('Ctrl Pts',(2.99542425341685,-1.,-2.84246132984415));
#51361=CARTESIAN_POINT('Ctrl Pts',(2.99542425341685,1.,-2.84246132984415));
#51362=CARTESIAN_POINT('Ctrl Pts',(2.99832751144925,-1.,-2.84968053289451));
#51363=CARTESIAN_POINT('Ctrl Pts',(2.99832751144925,1.,-2.84968053289451));
#51364=CARTESIAN_POINT('Ctrl Pts',(3.00120150796095,-1.,-2.85692085715686));
#51365=CARTESIAN_POINT('Ctrl Pts',(3.00120150796095,1.,-2.85692085715686));
#51366=CARTESIAN_POINT('Ctrl Pts',(3.00404638316867,-1.,-2.86418200833667));
#51367=CARTESIAN_POINT('Ctrl Pts',(3.00404638316867,1.,-2.86418200833667));
#51368=CARTESIAN_POINT('Ctrl Pts',(3.00686224485784,-1.,-2.87146368430502));
#51369=CARTESIAN_POINT('Ctrl Pts',(3.00686224485784,1.,-2.87146368430502));
#51370=CARTESIAN_POINT('Ctrl Pts',(3.00964918108476,-1.,-2.87876560072727));
#51371=CARTESIAN_POINT('Ctrl Pts',(3.00964918108476,1.,-2.87876560072727));
#51372=CARTESIAN_POINT('Ctrl Pts',(3.01240727308829,-1.,-2.8860875170608));
#51373=CARTESIAN_POINT('Ctrl Pts',(3.01240727308829,1.,-2.8860875170608));
#51374=CARTESIAN_POINT('Ctrl Pts',(3.01513660431928,-1.,-2.89342925566321));
#51375=CARTESIAN_POINT('Ctrl Pts',(3.01513660431928,1.,-2.89342925566321));
#51376=CARTESIAN_POINT('Ctrl Pts',(3.01783725121981,-1.,-2.9007906910105));
#51377=CARTESIAN_POINT('Ctrl Pts',(3.01783725121981,1.,-2.9007906910105));
#51378=CARTESIAN_POINT('Ctrl Pts',(3.01997487193503,-1.,-2.90669553302526));
#51379=CARTESIAN_POINT('Ctrl Pts',(3.01997487193503,1.,-2.90669553302526));
#51380=CARTESIAN_POINT('Ctrl Pts',(3.02156522742431,-1.,-2.91113297348212));
#51381=CARTESIAN_POINT('Ctrl Pts',(3.02156522742431,1.,-2.91113297348212));
#51382=CARTESIAN_POINT('Ctrl Pts',(3.02261975104593,-1.,-2.91409518070399));
#51383=CARTESIAN_POINT('Ctrl Pts',(3.02261975104593,1.,-2.91409518070399));
#51384=CARTESIAN_POINT('Ctrl Pts',(3.02314558451372,-1.,-2.91557726271063));
#51385=CARTESIAN_POINT('Ctrl Pts',(3.02314558451372,1.,-2.91557726271063));
#51386=CARTESIAN_POINT('',(2.79140942341258,1.,-2.50410331873176));
#51387=CARTESIAN_POINT('Ctrl Pts',(2.79140942341258,-1.,-2.50410331873176));
#51388=CARTESIAN_POINT('Ctrl Pts',(2.79140942341258,-0.666666666666667,
-2.50410331873176));
#51389=CARTESIAN_POINT('Ctrl Pts',(2.79140942341258,-0.333333333333333,
-2.50410331873176));
#51390=CARTESIAN_POINT('Ctrl Pts',(2.79140942341258,0.333333333333333,-2.50410331873176));
#51391=CARTESIAN_POINT('Ctrl Pts',(2.79140942341258,0.666666666666667,-2.50410331873176));
#51392=CARTESIAN_POINT('Ctrl Pts',(2.79140942341258,1.,-2.50410331873176));
#51393=CARTESIAN_POINT('',(3.02314558451372,1.,-2.91557726271063));
#51394=CARTESIAN_POINT('',(3.02314558451372,0.,-2.91557726271063));
#51395=CARTESIAN_POINT('Ctrl Pts',(2.79140942341258,1.,-2.50410331873176));
#51396=CARTESIAN_POINT('Ctrl Pts',(2.79145823440781,1.,-2.50410700351493));
#51397=CARTESIAN_POINT('Ctrl Pts',(2.79164172518905,1.,-2.50417932839313));
#51398=CARTESIAN_POINT('Ctrl Pts',(2.79217568804755,1.,-2.50455968395146));
#51399=CARTESIAN_POINT('Ctrl Pts',(2.79344192164147,1.,-2.50567182569081));
#51400=CARTESIAN_POINT('Ctrl Pts',(2.79596878057287,1.,-2.50810555977671));
#51401=CARTESIAN_POINT('Ctrl Pts',(2.79970585014168,1.,-2.51186983687818));
#51402=CARTESIAN_POINT('Ctrl Pts',(2.80427363984653,1.,-2.51660190465805));
#51403=CARTESIAN_POINT('Ctrl Pts',(2.80941521966941,1.,-2.52205778589653));
#51404=CARTESIAN_POINT('Ctrl Pts',(2.81484379048475,1.,-2.52796388055278));
#51405=CARTESIAN_POINT('Ctrl Pts',(2.82028550483689,1.,-2.53405679667412));
#51406=CARTESIAN_POINT('Ctrl Pts',(2.8255216764922,1.,-2.54012272520199));
#51407=CARTESIAN_POINT('Ctrl Pts',(2.83044254225917,1.,-2.54604736792655));
#51408=CARTESIAN_POINT('Ctrl Pts',(2.83505269592536,1.,-2.55182152807077));
#51409=CARTESIAN_POINT('Ctrl Pts',(2.83942515220782,1.,-2.55749952145241));
#51410=CARTESIAN_POINT('Ctrl Pts',(2.84366802680237,1.,-2.56316920798513));
#51411=CARTESIAN_POINT('Ctrl Pts',(2.84788893329067,1.,-2.56891984251721));
#51412=CARTESIAN_POINT('Ctrl Pts',(2.85215360144431,1.,-2.57480482727081));
#51413=CARTESIAN_POINT('Ctrl Pts',(2.85647171715092,1.,-2.58082875254357));
#51414=CARTESIAN_POINT('Ctrl Pts',(2.86081999003629,1.,-2.58696770643524));
#51415=CARTESIAN_POINT('Ctrl Pts',(2.86515629953513,1.,-2.59318160184908));
#51416=CARTESIAN_POINT('Ctrl Pts',(2.86943633170722,1.,-2.5994287522321));
#51417=CARTESIAN_POINT('Ctrl Pts',(2.87363176656501,1.,-2.60568177881303));
#51418=CARTESIAN_POINT('Ctrl Pts',(2.87773881947915,1.,-2.61193507170955));
#51419=CARTESIAN_POINT('Ctrl Pts',(2.88176821427525,1.,-2.61819596473108));
#51420=CARTESIAN_POINT('Ctrl Pts',(2.88573922195059,1.,-2.62447947640262));
#51421=CARTESIAN_POINT('Ctrl Pts',(2.88967244854239,1.,-2.63080195420767));
#51422=CARTESIAN_POINT('Ctrl Pts',(2.89358228854544,1.,-2.63717442263932));
#51423=CARTESIAN_POINT('Ctrl Pts',(2.89747231723345,1.,-2.64359851684131));
#51424=CARTESIAN_POINT('Ctrl Pts',(2.90133950224867,1.,-2.65007017365564));
#51425=CARTESIAN_POINT('Ctrl Pts',(2.90517678087461,1.,-2.65658188464282));
#51426=CARTESIAN_POINT('Ctrl Pts',(2.90897617968923,1.,-2.6631254261681));
#51427=CARTESIAN_POINT('Ctrl Pts',(2.91273193382882,1.,-2.66969458792631));
#51428=CARTESIAN_POINT('Ctrl Pts',(2.91644290704285,1.,-2.67628728855312));
#51429=CARTESIAN_POINT('Ctrl Pts',(2.92011090722152,1.,-2.68290409279688));
#51430=CARTESIAN_POINT('Ctrl Pts',(2.92373955325875,1.,-2.68954721165339));
#51431=CARTESIAN_POINT('Ctrl Pts',(2.92733294395267,1.,-2.69621932864301));
#51432=CARTESIAN_POINT('Ctrl Pts',(2.93089438233749,1.,-2.70292247416885));
#51433=CARTESIAN_POINT('Ctrl Pts',(2.93442516311179,1.,-2.70965695523787));
#51434=CARTESIAN_POINT('Ctrl Pts',(2.93792519474972,1.,-2.71642190053592));
#51435=CARTESIAN_POINT('Ctrl Pts',(2.94139351933897,1.,-2.72321571511337));
#51436=CARTESIAN_POINT('Ctrl Pts',(2.94482887675143,1.,-2.73003657371617));
#51437=CARTESIAN_POINT('Ctrl Pts',(2.94823023414364,1.,-2.73688288329808));
#51438=CARTESIAN_POINT('Ctrl Pts',(2.95159737214266,1.,-2.74375379492172));
#51439=CARTESIAN_POINT('Ctrl Pts',(2.95493069316161,1.,-2.75064903318947));
#51440=CARTESIAN_POINT('Ctrl Pts',(2.95823097665896,1.,-2.7575686788835));
#51441=CARTESIAN_POINT('Ctrl Pts',(2.96149914764818,1.,-2.76451296269557));
#51442=CARTESIAN_POINT('Ctrl Pts',(2.96473605585583,1.,-2.77148206836498));
#51443=CARTESIAN_POINT('Ctrl Pts',(2.96794221043036,1.,-2.7784758954285));
#51444=CARTESIAN_POINT('Ctrl Pts',(2.97111781461465,1.,-2.78549409123769));
#51445=CARTESIAN_POINT('Ctrl Pts',(2.9742628834758,1.,-2.79253615718248));
#51446=CARTESIAN_POINT('Ctrl Pts',(2.97737733718287,1.,-2.7996015327823));
#51447=CARTESIAN_POINT('Ctrl Pts',(2.98046109647241,1.,-2.80668968101106));
#51448=CARTESIAN_POINT('Ctrl Pts',(2.98351419779767,1.,-2.81380019196286));
#51449=CARTESIAN_POINT('Ctrl Pts',(2.9865368066918,1.,-2.82093279065457));
#51450=CARTESIAN_POINT('Ctrl Pts',(2.98952916401446,1.,-2.82808728190157));
#51451=CARTESIAN_POINT('Ctrl Pts',(2.99249155170339,1.,-2.83526351254248));
#51452=CARTESIAN_POINT('Ctrl Pts',(2.99542425341685,1.,-2.84246132984415));
#51453=CARTESIAN_POINT('Ctrl Pts',(2.99832751144925,1.,-2.84968053289451));
#51454=CARTESIAN_POINT('Ctrl Pts',(3.00120150796095,1.,-2.85692085715686));
#51455=CARTESIAN_POINT('Ctrl Pts',(3.00404638316867,1.,-2.86418200833667));
#51456=CARTESIAN_POINT('Ctrl Pts',(3.00686224485784,1.,-2.87146368430502));
#51457=CARTESIAN_POINT('Ctrl Pts',(3.00964918108476,1.,-2.87876560072727));
#51458=CARTESIAN_POINT('Ctrl Pts',(3.01240727308829,1.,-2.8860875170608));
#51459=CARTESIAN_POINT('Ctrl Pts',(3.01513660431928,1.,-2.89342925566321));
#51460=CARTESIAN_POINT('Ctrl Pts',(3.01783725121981,1.,-2.9007906910105));
#51461=CARTESIAN_POINT('Ctrl Pts',(3.01997487193503,1.,-2.90669553302526));
#51462=CARTESIAN_POINT('Ctrl Pts',(3.02156522742431,1.,-2.91113297348212));
#51463=CARTESIAN_POINT('Ctrl Pts',(3.02261975104593,1.,-2.91409518070399));
#51464=CARTESIAN_POINT('Ctrl Pts',(3.02314558451372,1.,-2.91557726271063));
#51465=CARTESIAN_POINT('Origin',(3.02314558451372,0.,-2.91557726271063));
#51466=CARTESIAN_POINT('',(2.91557726271063,1.,-3.02314558451372));
#51467=CARTESIAN_POINT('Origin',(0.,0.,0.));
#51468=CARTESIAN_POINT('',(2.90994629141562,1.,-2.36531447826213));
#51469=CARTESIAN_POINT('Origin',(0.,1.,0.));
#51470=CARTESIAN_POINT('Ctrl Pts',(2.90994629141562,1.,-2.36531447826213));
#51471=CARTESIAN_POINT('Ctrl Pts',(2.90994629141562,0.666666666666667,-2.36531447826213));
#51472=CARTESIAN_POINT('Ctrl Pts',(2.90994629141562,0.333333333333333,-2.36531447826213));
#51473=CARTESIAN_POINT('Ctrl Pts',(2.90994629141562,-0.333333333333333,
-2.36531447826213));
#51474=CARTESIAN_POINT('Ctrl Pts',(2.90994629141562,-0.666666666666667,
-2.36531447826213));
#51475=CARTESIAN_POINT('Ctrl Pts',(2.90994629141562,-1.,-2.36531447826213));
#51476=CARTESIAN_POINT('Ctrl Pts',(3.35260583073571,-1.,-2.52982887637028));
#51477=CARTESIAN_POINT('Ctrl Pts',(3.35260583073571,1.,-2.52982887637028));
#51478=CARTESIAN_POINT('Ctrl Pts',(3.35105973714426,-1.,-2.52954136549357));
#51479=CARTESIAN_POINT('Ctrl Pts',(3.35105973714426,1.,-2.52954136549357));
#51480=CARTESIAN_POINT('Ctrl Pts',(3.34796903577628,-1.,-2.5289632161143));
#51481=CARTESIAN_POINT('Ctrl Pts',(3.34796903577628,1.,-2.5289632161143));
#51482=CARTESIAN_POINT('Ctrl Pts',(3.34333744117093,-1.,-2.52808660916879));
#51483=CARTESIAN_POINT('Ctrl Pts',(3.34333744117093,1.,-2.52808660916879));
#51484=CARTESIAN_POINT('Ctrl Pts',(3.33717090000955,-1.,-2.52689902691551));
#51485=CARTESIAN_POINT('Ctrl Pts',(3.33717090000955,1.,-2.52689902691551));
#51486=CARTESIAN_POINT('Ctrl Pts',(3.32947762189049,-1.,-2.52538321165774));
#51487=CARTESIAN_POINT('Ctrl Pts',(3.32947762189049,1.,-2.52538321165774));
#51488=CARTESIAN_POINT('Ctrl Pts',(3.32179931079521,-1.,-2.52383598396878));
#51489=CARTESIAN_POINT('Ctrl Pts',(3.32179931079521,1.,-2.52383598396878));
#51490=CARTESIAN_POINT('Ctrl Pts',(3.31413607874727,-1.,-2.52225724871375));
#51491=CARTESIAN_POINT('Ctrl Pts',(3.31413607874727,1.,-2.52225724871375));
#51492=CARTESIAN_POINT('Ctrl Pts',(3.30648808814986,-1.,-2.52064689568167));
#51493=CARTESIAN_POINT('Ctrl Pts',(3.30648808814986,1.,-2.52064689568167));
#51494=CARTESIAN_POINT('Ctrl Pts',(3.29885556387661,-1.,-2.51900480700548));
#51495=CARTESIAN_POINT('Ctrl Pts',(3.29885556387661,1.,-2.51900480700548));
#51496=CARTESIAN_POINT('Ctrl Pts',(3.2912387729863,-1.,-2.51733085123316));
#51497=CARTESIAN_POINT('Ctrl Pts',(3.2912387729863,1.,-2.51733085123316));
#51498=CARTESIAN_POINT('Ctrl Pts',(3.28363799702583,-1.,-2.51562487464215));
#51499=CARTESIAN_POINT('Ctrl Pts',(3.28363799702583,1.,-2.51562487464215));
#51500=CARTESIAN_POINT('Ctrl Pts',(3.27605350473048,-1.,-2.51388669270329));
#51501=CARTESIAN_POINT('Ctrl Pts',(3.27605350473048,1.,-2.51388669270329));
#51502=CARTESIAN_POINT('Ctrl Pts',(3.26848552888271,-1.,-2.51211608411539));
#51503=CARTESIAN_POINT('Ctrl Pts',(3.26848552888271,1.,-2.51211608411539));
#51504=CARTESIAN_POINT('Ctrl Pts',(3.26093423001716,-1.,-2.51031277813697));
#51505=CARTESIAN_POINT('Ctrl Pts',(3.26093423001716,1.,-2.51031277813697));
#51506=CARTESIAN_POINT('Ctrl Pts',(3.25339971461265,-1.,-2.50847647070936));
#51507=CARTESIAN_POINT('Ctrl Pts',(3.25339971461265,1.,-2.50847647070936));
#51508=CARTESIAN_POINT('Ctrl Pts',(3.24588208984042,-1.,-2.50660685940645));
#51509=CARTESIAN_POINT('Ctrl Pts',(3.24588208984042,1.,-2.50660685940645));
#51510=CARTESIAN_POINT('Ctrl Pts',(3.23838151080383,-1.,-2.50470367580078));
#51511=CARTESIAN_POINT('Ctrl Pts',(3.23838151080383,1.,-2.50470367580078));
#51512=CARTESIAN_POINT('Ctrl Pts',(3.23089822320596,-1.,-2.50276671338074));
#51513=CARTESIAN_POINT('Ctrl Pts',(3.23089822320596,1.,-2.50276671338074));
#51514=CARTESIAN_POINT('Ctrl Pts',(3.22343262620387,-1.,-2.5007958720187));
#51515=CARTESIAN_POINT('Ctrl Pts',(3.22343262620387,1.,-2.5007958720187));
#51516=CARTESIAN_POINT('Ctrl Pts',(3.21598526261157,-1.,-2.49879114599293));
#51517=CARTESIAN_POINT('Ctrl Pts',(3.21598526261157,1.,-2.49879114599293));
#51518=CARTESIAN_POINT('Ctrl Pts',(3.2085566984974,-1.,-2.49675252647298));
#51519=CARTESIAN_POINT('Ctrl Pts',(3.2085566984974,1.,-2.49675252647298));
#51520=CARTESIAN_POINT('Ctrl Pts',(3.20114742397549,-1.,-2.49467992057726));
#51521=CARTESIAN_POINT('Ctrl Pts',(3.20114742397549,1.,-2.49467992057726));
#51522=CARTESIAN_POINT('Ctrl Pts',(3.19375775555814,-1.,-2.4925730723986));
#51523=CARTESIAN_POINT('Ctrl Pts',(3.19375775555814,1.,-2.4925730723986));
#51524=CARTESIAN_POINT('Ctrl Pts',(3.18638771282315,-1.,-2.49043146334095));
#51525=CARTESIAN_POINT('Ctrl Pts',(3.18638771282315,1.,-2.49043146334095));
#51526=CARTESIAN_POINT('Ctrl Pts',(3.17903698136678,-1.,-2.48825428288243));
#51527=CARTESIAN_POINT('Ctrl Pts',(3.17903698136678,1.,-2.48825428288243));
#51528=CARTESIAN_POINT('Ctrl Pts',(3.17170518863357,-1.,-2.48604065348619));
#51529=CARTESIAN_POINT('Ctrl Pts',(3.17170518863357,1.,-2.48604065348619));
#51530=CARTESIAN_POINT('Ctrl Pts',(3.16439213290181,-1.,-2.48378981792739));
#51531=CARTESIAN_POINT('Ctrl Pts',(3.16439213290181,1.,-2.48378981792739));
#51532=CARTESIAN_POINT('Ctrl Pts',(3.15709802322735,-1.,-2.48150133566568));
#51533=CARTESIAN_POINT('Ctrl Pts',(3.15709802322735,1.,-2.48150133566568));
#51534=CARTESIAN_POINT('Ctrl Pts',(3.14982373241335,-1.,-2.47917529057016));
#51535=CARTESIAN_POINT('Ctrl Pts',(3.14982373241335,1.,-2.47917529057016));
#51536=CARTESIAN_POINT('Ctrl Pts',(3.14257099546531,-1.,-2.47681245356095));
#51537=CARTESIAN_POINT('Ctrl Pts',(3.14257099546531,1.,-2.47681245356095));
#51538=CARTESIAN_POINT('Ctrl Pts',(3.13534181229282,-1.,-2.47441378371923));
#51539=CARTESIAN_POINT('Ctrl Pts',(3.13534181229282,1.,-2.47441378371923));
#51540=CARTESIAN_POINT('Ctrl Pts',(3.12813790805948,-1.,-2.47197997765868));
#51541=CARTESIAN_POINT('Ctrl Pts',(3.12813790805948,1.,-2.47197997765868));
#51542=CARTESIAN_POINT('Ctrl Pts',(3.12096015766984,-1.,-2.4695109894747));
#51543=CARTESIAN_POINT('Ctrl Pts',(3.12096015766984,1.,-2.4695109894747));
#51544=CARTESIAN_POINT('Ctrl Pts',(3.11380805536124,-1.,-2.46700558843507));
#51545=CARTESIAN_POINT('Ctrl Pts',(3.11380805536124,1.,-2.46700558843507));
#51546=CARTESIAN_POINT('Ctrl Pts',(3.10667907901981,-1.,-2.46446082979645));
#51547=CARTESIAN_POINT('Ctrl Pts',(3.10667907901981,1.,-2.46446082979645));
#51548=CARTESIAN_POINT('Ctrl Pts',(3.09956993697048,-1.,-2.4618730850188));
#51549=CARTESIAN_POINT('Ctrl Pts',(3.09956993697048,1.,-2.4618730850188));
#51550=CARTESIAN_POINT('Ctrl Pts',(3.09247787931881,-1.,-2.45923912563875));
#51551=CARTESIAN_POINT('Ctrl Pts',(3.09247787931881,1.,-2.45923912563875));
#51552=CARTESIAN_POINT('Ctrl Pts',(3.08540206545313,-1.,-2.45655725437037));
#51553=CARTESIAN_POINT('Ctrl Pts',(3.08540206545313,1.,-2.45655725437037));
#51554=CARTESIAN_POINT('Ctrl Pts',(3.07834472886145,-1.,-2.45382826787795));
#51555=CARTESIAN_POINT('Ctrl Pts',(3.07834472886145,1.,-2.45382826787795));
#51556=CARTESIAN_POINT('Ctrl Pts',(3.0713129052131,-1.,-2.45105688854432));
#51557=CARTESIAN_POINT('Ctrl Pts',(3.0713129052131,1.,-2.45105688854432));
#51558=CARTESIAN_POINT('Ctrl Pts',(3.06431596421422,-1.,-2.44824970516558));
#51559=CARTESIAN_POINT('Ctrl Pts',(3.06431596421422,1.,-2.44824970516558));
#51560=CARTESIAN_POINT('Ctrl Pts',(3.05736242671521,-1.,-2.44541251892568));
#51561=CARTESIAN_POINT('Ctrl Pts',(3.05736242671521,1.,-2.44541251892568));
#51562=CARTESIAN_POINT('Ctrl Pts',(3.05045678021509,-1.,-2.44254768923109));
#51563=CARTESIAN_POINT('Ctrl Pts',(3.05045678021509,1.,-2.44254768923109));
#51564=CARTESIAN_POINT('Ctrl Pts',(3.04359685040545,-1.,-2.43965194061849));
#51565=CARTESIAN_POINT('Ctrl Pts',(3.04359685040545,1.,-2.43965194061849));
#51566=CARTESIAN_POINT('Ctrl Pts',(3.03676949672797,-1.,-2.43671278042394));
#51567=CARTESIAN_POINT('Ctrl Pts',(3.03676949672797,1.,-2.43671278042394));
#51568=CARTESIAN_POINT('Ctrl Pts',(3.02995534946946,-1.,-2.43371241361462));
#51569=CARTESIAN_POINT('Ctrl Pts',(3.02995534946946,1.,-2.43371241361462));
#51570=CARTESIAN_POINT('Ctrl Pts',(3.02313656035977,-1.,-2.43063415586615));
#51571=CARTESIAN_POINT('Ctrl Pts',(3.02313656035977,1.,-2.43063415586615));
#51572=CARTESIAN_POINT('Ctrl Pts',(3.01630420830493,-1.,-2.4274685626416));
#51573=CARTESIAN_POINT('Ctrl Pts',(3.01630420830493,1.,-2.4274685626416));
#51574=CARTESIAN_POINT('Ctrl Pts',(3.00946442616674,-1.,-2.42421849439625));
#51575=CARTESIAN_POINT('Ctrl Pts',(3.00946442616674,1.,-2.42421849439625));
#51576=CARTESIAN_POINT('Ctrl Pts',(3.00264868586038,-1.,-2.42090763946812));
#51577=CARTESIAN_POINT('Ctrl Pts',(3.00264868586038,1.,-2.42090763946812));
#51578=CARTESIAN_POINT('Ctrl Pts',(2.99590509293561,-1.,-2.4175732450056));
#51579=CARTESIAN_POINT('Ctrl Pts',(2.99590509293561,1.,-2.4175732450056));
#51580=CARTESIAN_POINT('Ctrl Pts',(2.98927983005851,-1.,-2.4142506419963));
#51581=CARTESIAN_POINT('Ctrl Pts',(2.98927983005851,1.,-2.4142506419963));
#51582=CARTESIAN_POINT('Ctrl Pts',(2.98280015815132,-1.,-2.41095909342591));
#51583=CARTESIAN_POINT('Ctrl Pts',(2.98280015815132,1.,-2.41095909342591));
#51584=CARTESIAN_POINT('Ctrl Pts',(2.97646002822395,-1.,-2.40768975073691));
#51585=CARTESIAN_POINT('Ctrl Pts',(2.97646002822395,1.,-2.40768975073691));
#51586=CARTESIAN_POINT('Ctrl Pts',(2.97019641312272,-1.,-2.40438604734848));
#51587=CARTESIAN_POINT('Ctrl Pts',(2.97019641312272,1.,-2.40438604734848));
#51588=CARTESIAN_POINT('Ctrl Pts',(2.9639043224018,-1.,-2.40095565711535));
#51589=CARTESIAN_POINT('Ctrl Pts',(2.9639043224018,1.,-2.40095565711535));
#51590=CARTESIAN_POINT('Ctrl Pts',(2.95748006482811,-1.,-2.39730553974412));
#51591=CARTESIAN_POINT('Ctrl Pts',(2.95748006482811,1.,-2.39730553974412));
#51592=CARTESIAN_POINT('Ctrl Pts',(2.95085857128372,-1.,-2.39337207631613));
#51593=CARTESIAN_POINT('Ctrl Pts',(2.95085857128372,1.,-2.39337207631613));
#51594=CARTESIAN_POINT('Ctrl Pts',(2.94404820669135,-1.,-2.38914929090806));
#51595=CARTESIAN_POINT('Ctrl Pts',(2.94404820669135,1.,-2.38914929090806));
#51596=CARTESIAN_POINT('Ctrl Pts',(2.93717903280599,-1.,-2.38472771516476));
#51597=CARTESIAN_POINT('Ctrl Pts',(2.93717903280599,1.,-2.38472771516476));
#51598=CARTESIAN_POINT('Ctrl Pts',(2.93049643640517,-1.,-2.3802898958232));
#51599=CARTESIAN_POINT('Ctrl Pts',(2.93049643640517,1.,-2.3802898958232));
#51600=CARTESIAN_POINT('Ctrl Pts',(2.92430340582912,-1.,-2.37606510524271));
#51601=CARTESIAN_POINT('Ctrl Pts',(2.92430340582912,1.,-2.37606510524271));
#51602=CARTESIAN_POINT('Ctrl Pts',(2.9189150379156,-1.,-2.37229381109939));
#51603=CARTESIAN_POINT('Ctrl Pts',(2.9189150379156,1.,-2.37229381109939));
#51604=CARTESIAN_POINT('Ctrl Pts',(2.91461249883016,-1.,-2.36919161373074));
#51605=CARTESIAN_POINT('Ctrl Pts',(2.91461249883016,1.,-2.36919161373074));
#51606=CARTESIAN_POINT('Ctrl Pts',(2.9115863784165,-1.,-2.36690501170317));
#51607=CARTESIAN_POINT('Ctrl Pts',(2.9115863784165,1.,-2.36690501170317));
#51608=CARTESIAN_POINT('Ctrl Pts',(2.91025813829606,-1.,-2.36578327194396));
#51609=CARTESIAN_POINT('Ctrl Pts',(2.91025813829606,1.,-2.36578327194396));
#51610=CARTESIAN_POINT('Ctrl Pts',(2.90989022547738,-1.,-2.36535052956704));
#51611=CARTESIAN_POINT('Ctrl Pts',(2.90989022547738,1.,-2.36535052956704));
#51612=CARTESIAN_POINT('Ctrl Pts',(2.90992398626098,-1.,-2.36524348105023));
#51613=CARTESIAN_POINT('Ctrl Pts',(2.90992398626098,1.,-2.36524348105023));
#51614=CARTESIAN_POINT('Ctrl Pts',(2.91001063062876,-1.,-2.36523532225181));
#51615=CARTESIAN_POINT('Ctrl Pts',(2.91001063062876,1.,-2.36523532225181));
#51616=CARTESIAN_POINT('',(3.35260583073571,1.,-2.52982887637028));
#51617=CARTESIAN_POINT('Ctrl Pts',(3.35260583073571,1.,-2.52982887637028));
#51618=CARTESIAN_POINT('Ctrl Pts',(3.35105973714426,1.,-2.52954136549357));
#51619=CARTESIAN_POINT('Ctrl Pts',(3.34796903577628,1.,-2.5289632161143));
#51620=CARTESIAN_POINT('Ctrl Pts',(3.34333744117093,1.,-2.52808660916879));
#51621=CARTESIAN_POINT('Ctrl Pts',(3.33717090000955,1.,-2.52689902691551));
#51622=CARTESIAN_POINT('Ctrl Pts',(3.32947762189049,1.,-2.52538321165774));
#51623=CARTESIAN_POINT('Ctrl Pts',(3.32179931079521,1.,-2.52383598396878));
#51624=CARTESIAN_POINT('Ctrl Pts',(3.31413607874727,1.,-2.52225724871375));
#51625=CARTESIAN_POINT('Ctrl Pts',(3.30648808814986,1.,-2.52064689568167));
#51626=CARTESIAN_POINT('Ctrl Pts',(3.29885556387661,1.,-2.51900480700548));
#51627=CARTESIAN_POINT('Ctrl Pts',(3.2912387729863,1.,-2.51733085123316));
#51628=CARTESIAN_POINT('Ctrl Pts',(3.28363799702583,1.,-2.51562487464215));
#51629=CARTESIAN_POINT('Ctrl Pts',(3.27605350473048,1.,-2.51388669270329));
#51630=CARTESIAN_POINT('Ctrl Pts',(3.26848552888271,1.,-2.51211608411539));
#51631=CARTESIAN_POINT('Ctrl Pts',(3.26093423001716,1.,-2.51031277813697));
#51632=CARTESIAN_POINT('Ctrl Pts',(3.25339971461265,1.,-2.50847647070936));
#51633=CARTESIAN_POINT('Ctrl Pts',(3.24588208984042,1.,-2.50660685940645));
#51634=CARTESIAN_POINT('Ctrl Pts',(3.23838151080383,1.,-2.50470367580078));
#51635=CARTESIAN_POINT('Ctrl Pts',(3.23089822320596,1.,-2.50276671338074));
#51636=CARTESIAN_POINT('Ctrl Pts',(3.22343262620387,1.,-2.5007958720187));
#51637=CARTESIAN_POINT('Ctrl Pts',(3.21598526261157,1.,-2.49879114599293));
#51638=CARTESIAN_POINT('Ctrl Pts',(3.2085566984974,1.,-2.49675252647298));
#51639=CARTESIAN_POINT('Ctrl Pts',(3.20114742397549,1.,-2.49467992057726));
#51640=CARTESIAN_POINT('Ctrl Pts',(3.19375775555814,1.,-2.4925730723986));
#51641=CARTESIAN_POINT('Ctrl Pts',(3.18638771282315,1.,-2.49043146334095));
#51642=CARTESIAN_POINT('Ctrl Pts',(3.17903698136678,1.,-2.48825428288243));
#51643=CARTESIAN_POINT('Ctrl Pts',(3.17170518863357,1.,-2.48604065348619));
#51644=CARTESIAN_POINT('Ctrl Pts',(3.16439213290181,1.,-2.48378981792739));
#51645=CARTESIAN_POINT('Ctrl Pts',(3.15709802322735,1.,-2.48150133566568));
#51646=CARTESIAN_POINT('Ctrl Pts',(3.14982373241335,1.,-2.47917529057016));
#51647=CARTESIAN_POINT('Ctrl Pts',(3.14257099546531,1.,-2.47681245356095));
#51648=CARTESIAN_POINT('Ctrl Pts',(3.13534181229282,1.,-2.47441378371923));
#51649=CARTESIAN_POINT('Ctrl Pts',(3.12813790805948,1.,-2.47197997765868));
#51650=CARTESIAN_POINT('Ctrl Pts',(3.12096015766984,1.,-2.4695109894747));
#51651=CARTESIAN_POINT('Ctrl Pts',(3.11380805536124,1.,-2.46700558843507));
#51652=CARTESIAN_POINT('Ctrl Pts',(3.10667907901981,1.,-2.46446082979645));
#51653=CARTESIAN_POINT('Ctrl Pts',(3.09956993697048,1.,-2.4618730850188));
#51654=CARTESIAN_POINT('Ctrl Pts',(3.09247787931881,1.,-2.45923912563875));
#51655=CARTESIAN_POINT('Ctrl Pts',(3.08540206545313,1.,-2.45655725437037));
#51656=CARTESIAN_POINT('Ctrl Pts',(3.07834472886145,1.,-2.45382826787795));
#51657=CARTESIAN_POINT('Ctrl Pts',(3.0713129052131,1.,-2.45105688854432));
#51658=CARTESIAN_POINT('Ctrl Pts',(3.06431596421422,1.,-2.44824970516558));
#51659=CARTESIAN_POINT('Ctrl Pts',(3.05736242671521,1.,-2.44541251892568));
#51660=CARTESIAN_POINT('Ctrl Pts',(3.05045678021509,1.,-2.44254768923109));
#51661=CARTESIAN_POINT('Ctrl Pts',(3.04359685040545,1.,-2.43965194061849));
#51662=CARTESIAN_POINT('Ctrl Pts',(3.03676949672797,1.,-2.43671278042394));
#51663=CARTESIAN_POINT('Ctrl Pts',(3.02995534946946,1.,-2.43371241361462));
#51664=CARTESIAN_POINT('Ctrl Pts',(3.02313656035977,1.,-2.43063415586615));
#51665=CARTESIAN_POINT('Ctrl Pts',(3.01630420830493,1.,-2.4274685626416));
#51666=CARTESIAN_POINT('Ctrl Pts',(3.00946442616674,1.,-2.42421849439625));
#51667=CARTESIAN_POINT('Ctrl Pts',(3.00264868586038,1.,-2.42090763946812));
#51668=CARTESIAN_POINT('Ctrl Pts',(2.99590509293561,1.,-2.4175732450056));
#51669=CARTESIAN_POINT('Ctrl Pts',(2.98927983005851,1.,-2.4142506419963));
#51670=CARTESIAN_POINT('Ctrl Pts',(2.98280015815132,1.,-2.41095909342591));
#51671=CARTESIAN_POINT('Ctrl Pts',(2.97646002822395,1.,-2.40768975073691));
#51672=CARTESIAN_POINT('Ctrl Pts',(2.97019641312272,1.,-2.40438604734848));
#51673=CARTESIAN_POINT('Ctrl Pts',(2.9639043224018,1.,-2.40095565711535));
#51674=CARTESIAN_POINT('Ctrl Pts',(2.95748006482811,1.,-2.39730553974412));
#51675=CARTESIAN_POINT('Ctrl Pts',(2.95085857128372,1.,-2.39337207631613));
#51676=CARTESIAN_POINT('Ctrl Pts',(2.94404820669135,1.,-2.38914929090806));
#51677=CARTESIAN_POINT('Ctrl Pts',(2.93717903280599,1.,-2.38472771516476));
#51678=CARTESIAN_POINT('Ctrl Pts',(2.93049643640517,1.,-2.3802898958232));
#51679=CARTESIAN_POINT('Ctrl Pts',(2.92430340582912,1.,-2.37606510524271));
#51680=CARTESIAN_POINT('Ctrl Pts',(2.9189150379156,1.,-2.37229381109939));
#51681=CARTESIAN_POINT('Ctrl Pts',(2.91461249883016,1.,-2.36919161373074));
#51682=CARTESIAN_POINT('Ctrl Pts',(2.91181344022628,1.,-2.36707658451709));
#51683=CARTESIAN_POINT('Ctrl Pts',(2.91051690822262,1.,-2.36599991765853));
#51684=CARTESIAN_POINT('Ctrl Pts',(2.9100577052777,1.,-2.36553202948741));
#51685=CARTESIAN_POINT('Ctrl Pts',(2.90995756655558,1.,-2.3653621118858));
#51686=CARTESIAN_POINT('Ctrl Pts',(2.90994629141562,1.,-2.36531447826213));
#51687=CARTESIAN_POINT('',(3.35260583073571,0.,-2.52982887637028));
#51688=CARTESIAN_POINT('Ctrl Pts',(3.1487152044751,-1.,-2.03668666247593));
#51689=CARTESIAN_POINT('Ctrl Pts',(3.1487152044751,1.,-2.03668666247593));
#51690=CARTESIAN_POINT('Ctrl Pts',(3.14869618937258,-1.,-2.03660173757879));
#51691=CARTESIAN_POINT('Ctrl Pts',(3.14869618937258,1.,-2.03660173757879));
#51692=CARTESIAN_POINT('Ctrl Pts',(3.14878756590812,-1.,-2.03653654935592));
#51693=CARTESIAN_POINT('Ctrl Pts',(3.14878756590812,1.,-2.03653654935592));
#51694=CARTESIAN_POINT('Ctrl Pts',(3.14931281968048,-1.,-2.03675273049189));
#51695=CARTESIAN_POINT('Ctrl Pts',(3.14931281968048,1.,-2.03675273049189));
#51696=CARTESIAN_POINT('Ctrl Pts',(3.15079010635742,-1.,-2.03766932526445));
#51697=CARTESIAN_POINT('Ctrl Pts',(3.15079010635742,1.,-2.03766932526445));
#51698=CARTESIAN_POINT('Ctrl Pts',(3.15389991674792,-1.,-2.03984073791519));
#51699=CARTESIAN_POINT('Ctrl Pts',(3.15389991674792,1.,-2.03984073791519));
#51700=CARTESIAN_POINT('Ctrl Pts',(3.15817983946367,-1.,-2.04297406404027));
#51701=CARTESIAN_POINT('Ctrl Pts',(3.15817983946367,1.,-2.04297406404027));
#51702=CARTESIAN_POINT('Ctrl Pts',(3.16343165058912,-1.,-2.04693331247446));
#51703=CARTESIAN_POINT('Ctrl Pts',(3.16343165058912,1.,-2.04693331247446));
#51704=CARTESIAN_POINT('Ctrl Pts',(3.16936341689527,-1.,-2.05151770247233));
#51705=CARTESIAN_POINT('Ctrl Pts',(3.16936341689527,1.,-2.05151770247233));
#51706=CARTESIAN_POINT('Ctrl Pts',(3.17564906975371,-1.,-2.05650186773132));
#51707=CARTESIAN_POINT('Ctrl Pts',(3.17564906975371,1.,-2.05650186773132));
#51708=CARTESIAN_POINT('Ctrl Pts',(3.18197692964614,-1.,-2.06166849827101));
#51709=CARTESIAN_POINT('Ctrl Pts',(3.18197692964614,1.,-2.06166849827101));
#51710=CARTESIAN_POINT('Ctrl Pts',(3.18809755562368,-1.,-2.06684062744112));
#51711=CARTESIAN_POINT('Ctrl Pts',(3.18809755562368,1.,-2.06684062744112));
#51712=CARTESIAN_POINT('Ctrl Pts',(3.19388465568252,-1.,-2.07192253497857));
#51713=CARTESIAN_POINT('Ctrl Pts',(3.19388465568252,1.,-2.07192253497857));
#51714=CARTESIAN_POINT('Ctrl Pts',(3.19934132836019,-1.,-2.07690441870722));
#51715=CARTESIAN_POINT('Ctrl Pts',(3.19934132836019,1.,-2.07690441870722));
#51716=CARTESIAN_POINT('Ctrl Pts',(3.2045481863073,-1.,-2.08182850370878));
#51717=CARTESIAN_POINT('Ctrl Pts',(3.2045481863073,1.,-2.08182850370878));
#51718=CARTESIAN_POINT('Ctrl Pts',(3.20962575845463,-1.,-2.08676465517455));
#51719=CARTESIAN_POINT('Ctrl Pts',(3.20962575845463,1.,-2.08676465517455));
#51720=CARTESIAN_POINT('Ctrl Pts',(3.21469429601654,-1.,-2.09178419460443));
#51721=CARTESIAN_POINT('Ctrl Pts',(3.21469429601654,1.,-2.09178419460443));
#51722=CARTESIAN_POINT('Ctrl Pts',(3.21982707347009,-1.,-2.09692958434895));
#51723=CARTESIAN_POINT('Ctrl Pts',(3.21982707347009,1.,-2.09692958434895));
#51724=CARTESIAN_POINT('Ctrl Pts',(3.22503437553434,-1.,-2.10220384298492));
#51725=CARTESIAN_POINT('Ctrl Pts',(3.22503437553434,1.,-2.10220384298492));
#51726=CARTESIAN_POINT('Ctrl Pts',(3.23028945793289,-1.,-2.10758699642451));
#51727=CARTESIAN_POINT('Ctrl Pts',(3.23028945793289,1.,-2.10758699642451));
#51728=CARTESIAN_POINT('Ctrl Pts',(3.23554444767099,-1.,-2.11304604021773));
#51729=CARTESIAN_POINT('Ctrl Pts',(3.23554444767099,1.,-2.11304604021773));
#51730=CARTESIAN_POINT('Ctrl Pts',(3.24074905517293,-1.,-2.11854673326979));
#51731=CARTESIAN_POINT('Ctrl Pts',(3.24074905517293,1.,-2.11854673326979));
#51732=CARTESIAN_POINT('Ctrl Pts',(3.24587102613376,-1.,-2.12406646410962));
#51733=CARTESIAN_POINT('Ctrl Pts',(3.24587102613376,1.,-2.12406646410962));
#51734=CARTESIAN_POINT('Ctrl Pts',(3.25090574494028,-1.,-2.12960028396832));
#51735=CARTESIAN_POINT('Ctrl Pts',(3.25090574494028,1.,-2.12960028396832));
#51736=CARTESIAN_POINT('Ctrl Pts',(3.25586495065054,-1.,-2.13515375878803));
#51737=CARTESIAN_POINT('Ctrl Pts',(3.25586495065054,1.,-2.13515375878803));
#51738=CARTESIAN_POINT('Ctrl Pts',(3.26077002641879,-1.,-2.14073870754264));
#51739=CARTESIAN_POINT('Ctrl Pts',(3.26077002641879,1.,-2.14073870754264));
#51740=CARTESIAN_POINT('Ctrl Pts',(3.26564388189759,-1.,-2.1463680529566));
#51741=CARTESIAN_POINT('Ctrl Pts',(3.26564388189759,1.,-2.1463680529566));
#51742=CARTESIAN_POINT('Ctrl Pts',(3.27050245897228,-1.,-2.15205043199808));
#51743=CARTESIAN_POINT('Ctrl Pts',(3.27050245897228,1.,-2.15205043199808));
#51744=CARTESIAN_POINT('Ctrl Pts',(3.27534954469187,-1.,-2.15778690038347));
#51745=CARTESIAN_POINT('Ctrl Pts',(3.27534954469187,1.,-2.15778690038347));
#51746=CARTESIAN_POINT('Ctrl Pts',(3.280181508414,-1.,-2.16357391934425));
#51747=CARTESIAN_POINT('Ctrl Pts',(3.280181508414,1.,-2.16357391934425));
#51748=CARTESIAN_POINT('Ctrl Pts',(3.28499019979724,-1.,-2.16940517773455));
#51749=CARTESIAN_POINT('Ctrl Pts',(3.28499019979724,1.,-2.16940517773455));
#51750=CARTESIAN_POINT('Ctrl Pts',(3.28976645712568,-1.,-2.17527380048423));
#51751=CARTESIAN_POINT('Ctrl Pts',(3.28976645712568,1.,-2.17527380048423));
#51752=CARTESIAN_POINT('Ctrl Pts',(3.2945036150049,-1.,-2.18117455557065));
#51753=CARTESIAN_POINT('Ctrl Pts',(3.2945036150049,1.,-2.18117455557065));
#51754=CARTESIAN_POINT('Ctrl Pts',(3.29920022557639,-1.,-2.18710556500327));
#51755=CARTESIAN_POINT('Ctrl Pts',(3.29920022557639,1.,-2.18710556500327));
#51756=CARTESIAN_POINT('Ctrl Pts',(3.30385816281831,-1.,-2.19306710376111));
#51757=CARTESIAN_POINT('Ctrl Pts',(3.30385816281831,1.,-2.19306710376111));
#51758=CARTESIAN_POINT('Ctrl Pts',(3.30848134694595,-1.,-2.19906078949923));
#51759=CARTESIAN_POINT('Ctrl Pts',(3.30848134694595,1.,-2.19906078949923));
#51760=CARTESIAN_POINT('Ctrl Pts',(3.31307424608949,-1.,-2.20508863150607));
#51761=CARTESIAN_POINT('Ctrl Pts',(3.31307424608949,1.,-2.20508863150607));
#51762=CARTESIAN_POINT('Ctrl Pts',(3.31764044024235,-1.,-2.21115211847875));
#51763=CARTESIAN_POINT('Ctrl Pts',(3.31764044024235,1.,-2.21115211847875));
#51764=CARTESIAN_POINT('Ctrl Pts',(3.32218125618968,-1.,-2.21725135110898));
#51765=CARTESIAN_POINT('Ctrl Pts',(3.32218125618968,1.,-2.21725135110898));
#51766=CARTESIAN_POINT('Ctrl Pts',(3.3266964672289,-1.,-2.22338548312772));
#51767=CARTESIAN_POINT('Ctrl Pts',(3.3266964672289,1.,-2.22338548312772));
#51768=CARTESIAN_POINT('Ctrl Pts',(3.33118487773611,-1.,-2.22955308907233));
#51769=CARTESIAN_POINT('Ctrl Pts',(3.33118487773611,1.,-2.22955308907233));
#51770=CARTESIAN_POINT('Ctrl Pts',(3.33564495756481,-1.,-2.23575256328812));
#51771=CARTESIAN_POINT('Ctrl Pts',(3.33564495756481,1.,-2.23575256328812));
#51772=CARTESIAN_POINT('Ctrl Pts',(3.34007543738025,-1.,-2.24198249391422));
#51773=CARTESIAN_POINT('Ctrl Pts',(3.34007543738025,1.,-2.24198249391422));
#51774=CARTESIAN_POINT('Ctrl Pts',(3.34447596770723,-1.,-2.24824207678256));
#51775=CARTESIAN_POINT('Ctrl Pts',(3.34447596770723,1.,-2.24824207678256));
#51776=CARTESIAN_POINT('Ctrl Pts',(3.34884690292285,-1.,-2.25453097693483));
#51777=CARTESIAN_POINT('Ctrl Pts',(3.34884690292285,1.,-2.25453097693483));
#51778=CARTESIAN_POINT('Ctrl Pts',(3.35318902552626,-1.,-2.26084915222449));
#51779=CARTESIAN_POINT('Ctrl Pts',(3.35318902552626,1.,-2.26084915222449));
#51780=CARTESIAN_POINT('Ctrl Pts',(3.35750328523061,-1.,-2.2671966857991));
#51781=CARTESIAN_POINT('Ctrl Pts',(3.35750328523061,1.,-2.2671966857991));
#51782=CARTESIAN_POINT('Ctrl Pts',(3.36179055004409,-1.,-2.2735736262093));
#51783=CARTESIAN_POINT('Ctrl Pts',(3.36179055004409,1.,-2.2735736262093));
#51784=CARTESIAN_POINT('Ctrl Pts',(3.36605130713076,-1.,-2.27997979458037));
#51785=CARTESIAN_POINT('Ctrl Pts',(3.36605130713076,1.,-2.27997979458037));
#51786=CARTESIAN_POINT('Ctrl Pts',(3.37028570206488,-1.,-2.28641481081137));
#51787=CARTESIAN_POINT('Ctrl Pts',(3.37028570206488,1.,-2.28641481081137));
#51788=CARTESIAN_POINT('Ctrl Pts',(3.37449367172826,-1.,-2.29287818007393));
#51789=CARTESIAN_POINT('Ctrl Pts',(3.37449367172826,1.,-2.29287818007393));
#51790=CARTESIAN_POINT('Ctrl Pts',(3.37867504959433,-1.,-2.29936936127624));
#51791=CARTESIAN_POINT('Ctrl Pts',(3.37867504959433,1.,-2.29936936127624));
#51792=CARTESIAN_POINT('Ctrl Pts',(3.3828296733661,-1.,-2.30588783640343));
#51793=CARTESIAN_POINT('Ctrl Pts',(3.3828296733661,1.,-2.30588783640343));
#51794=CARTESIAN_POINT('Ctrl Pts',(3.38695751492462,-1.,-2.31243319489367));
#51795=CARTESIAN_POINT('Ctrl Pts',(3.38695751492462,1.,-2.31243319489367));
#51796=CARTESIAN_POINT('Ctrl Pts',(3.39105869474822,-1.,-2.31900513925424));
#51797=CARTESIAN_POINT('Ctrl Pts',(3.39105869474822,1.,-2.31900513925424));
#51798=CARTESIAN_POINT('Ctrl Pts',(3.39513342019756,-1.,-2.3256034390248));
#51799=CARTESIAN_POINT('Ctrl Pts',(3.39513342019756,1.,-2.3256034390248));
#51800=CARTESIAN_POINT('Ctrl Pts',(3.39918194577956,-1.,-2.33222789882489));
#51801=CARTESIAN_POINT('Ctrl Pts',(3.39918194577956,1.,-2.33222789882489));
#51802=CARTESIAN_POINT('Ctrl Pts',(3.40320452776743,-1.,-2.33887832342782));
#51803=CARTESIAN_POINT('Ctrl Pts',(3.40320452776743,1.,-2.33887832342782));
#51804=CARTESIAN_POINT('Ctrl Pts',(3.40720137404297,-1.,-2.34555447649188));
#51805=CARTESIAN_POINT('Ctrl Pts',(3.40720137404297,1.,-2.34555447649188));
#51806=CARTESIAN_POINT('Ctrl Pts',(3.41117262314119,-1.,-2.35225606824109));
#51807=CARTESIAN_POINT('Ctrl Pts',(3.41117262314119,1.,-2.35225606824109));
#51808=CARTESIAN_POINT('Ctrl Pts',(3.41511836751469,-1.,-2.35898278606946));
#51809=CARTESIAN_POINT('Ctrl Pts',(3.41511836751469,1.,-2.35898278606946));
#51810=CARTESIAN_POINT('Ctrl Pts',(3.41903866635852,-1.,-2.36573431470642));
#51811=CARTESIAN_POINT('Ctrl Pts',(3.41903866635852,1.,-2.36573431470642));
#51812=CARTESIAN_POINT('Ctrl Pts',(3.42293356216511,-1.,-2.37251035954292));
#51813=CARTESIAN_POINT('Ctrl Pts',(3.42293356216511,1.,-2.37251035954292));
#51814=CARTESIAN_POINT('Ctrl Pts',(3.42680309754399,-1.,-2.37931067028926));
#51815=CARTESIAN_POINT('Ctrl Pts',(3.42680309754399,1.,-2.37931067028926));
#51816=CARTESIAN_POINT('Ctrl Pts',(3.43064732712919,-1.,-2.38613505843552));
#51817=CARTESIAN_POINT('Ctrl Pts',(3.43064732712919,1.,-2.38613505843552));
#51818=CARTESIAN_POINT('Ctrl Pts',(3.4344663067854,-1.,-2.39298338804493));
#51819=CARTESIAN_POINT('Ctrl Pts',(3.4344663067854,1.,-2.39298338804493));
#51820=CARTESIAN_POINT('Ctrl Pts',(3.43750133064416,-1.,-2.39848113410292));
#51821=CARTESIAN_POINT('Ctrl Pts',(3.43750133064416,1.,-2.39848113410292));
#51822=CARTESIAN_POINT('Ctrl Pts',(3.43976627484234,-1.,-2.40261515589405));
#51823=CARTESIAN_POINT('Ctrl Pts',(3.43976627484234,1.,-2.40261515589405));
#51824=CARTESIAN_POINT('Ctrl Pts',(3.44127120683039,-1.,-2.4053759295909));
#51825=CARTESIAN_POINT('Ctrl Pts',(3.44127120683039,1.,-2.4053759295909));
#51826=CARTESIAN_POINT('Ctrl Pts',(3.44202241512147,-1.,-2.40675750623143));
#51827=CARTESIAN_POINT('Ctrl Pts',(3.44202241512147,1.,-2.40675750623143));
#51828=CARTESIAN_POINT('',(3.14877060440327,1.,-2.03660101169715));
#51829=CARTESIAN_POINT('Ctrl Pts',(3.14877060440327,-1.,-2.03660101169715));
#51830=CARTESIAN_POINT('Ctrl Pts',(3.14877060440327,-0.666666666666667,
-2.03660101169715));
#51831=CARTESIAN_POINT('Ctrl Pts',(3.14877060440327,-0.333333333333333,
-2.03660101169715));
#51832=CARTESIAN_POINT('Ctrl Pts',(3.14877060440327,0.333333333333333,-2.03660101169715));
#51833=CARTESIAN_POINT('Ctrl Pts',(3.14877060440328,0.666666666666667,-2.03660101169714));
#51834=CARTESIAN_POINT('Ctrl Pts',(3.14877060440328,1.,-2.03660101169714));
#51835=CARTESIAN_POINT('',(3.44202241512147,1.,-2.40675750623143));
#51836=CARTESIAN_POINT('',(3.44202241512147,0.,-2.40675750623143));
#51837=CARTESIAN_POINT('Ctrl Pts',(3.14877060440327,1.,-2.03660101169715));
#51838=CARTESIAN_POINT('Ctrl Pts',(3.14881939088124,1.,-2.03659701539259));
#51839=CARTESIAN_POINT('Ctrl Pts',(3.1490119366901,1.,-2.03663974554932));
#51840=CARTESIAN_POINT('Ctrl Pts',(3.14959882629804,1.,-2.03693188810544));
#51841=CARTESIAN_POINT('Ctrl Pts',(3.15102344775328,1.,-2.03783225495961));
#51842=CARTESIAN_POINT('Ctrl Pts',(3.15389991674792,1.,-2.03984073791519));
#51843=CARTESIAN_POINT('Ctrl Pts',(3.15817983946367,1.,-2.04297406404027));
#51844=CARTESIAN_POINT('Ctrl Pts',(3.16343165058912,1.,-2.04693331247446));
#51845=CARTESIAN_POINT('Ctrl Pts',(3.16936341689527,1.,-2.05151770247233));
#51846=CARTESIAN_POINT('Ctrl Pts',(3.17564906975371,1.,-2.05650186773132));
#51847=CARTESIAN_POINT('Ctrl Pts',(3.18197692964614,1.,-2.06166849827101));
#51848=CARTESIAN_POINT('Ctrl Pts',(3.18809755562368,1.,-2.06684062744112));
#51849=CARTESIAN_POINT('Ctrl Pts',(3.19388465568252,1.,-2.07192253497857));
#51850=CARTESIAN_POINT('Ctrl Pts',(3.19934132836019,1.,-2.07690441870722));
#51851=CARTESIAN_POINT('Ctrl Pts',(3.2045481863073,1.,-2.08182850370878));
#51852=CARTESIAN_POINT('Ctrl Pts',(3.20962575845463,1.,-2.08676465517455));
#51853=CARTESIAN_POINT('Ctrl Pts',(3.21469429601654,1.,-2.09178419460443));
#51854=CARTESIAN_POINT('Ctrl Pts',(3.21982707347009,1.,-2.09692958434895));
#51855=CARTESIAN_POINT('Ctrl Pts',(3.22503437553434,1.,-2.10220384298492));
#51856=CARTESIAN_POINT('Ctrl Pts',(3.23028945793289,1.,-2.10758699642451));
#51857=CARTESIAN_POINT('Ctrl Pts',(3.23554444767099,1.,-2.11304604021773));
#51858=CARTESIAN_POINT('Ctrl Pts',(3.24074905517293,1.,-2.11854673326979));
#51859=CARTESIAN_POINT('Ctrl Pts',(3.24587102613376,1.,-2.12406646410962));
#51860=CARTESIAN_POINT('Ctrl Pts',(3.25090574494028,1.,-2.12960028396832));
#51861=CARTESIAN_POINT('Ctrl Pts',(3.25586495065054,1.,-2.13515375878803));
#51862=CARTESIAN_POINT('Ctrl Pts',(3.26077002641879,1.,-2.14073870754264));
#51863=CARTESIAN_POINT('Ctrl Pts',(3.26564388189759,1.,-2.1463680529566));
#51864=CARTESIAN_POINT('Ctrl Pts',(3.27050245897228,1.,-2.15205043199808));
#51865=CARTESIAN_POINT('Ctrl Pts',(3.27534954469187,1.,-2.15778690038347));
#51866=CARTESIAN_POINT('Ctrl Pts',(3.280181508414,1.,-2.16357391934425));
#51867=CARTESIAN_POINT('Ctrl Pts',(3.28499019979724,1.,-2.16940517773455));
#51868=CARTESIAN_POINT('Ctrl Pts',(3.28976645712568,1.,-2.17527380048423));
#51869=CARTESIAN_POINT('Ctrl Pts',(3.2945036150049,1.,-2.18117455557065));
#51870=CARTESIAN_POINT('Ctrl Pts',(3.29920022557639,1.,-2.18710556500327));
#51871=CARTESIAN_POINT('Ctrl Pts',(3.30385816281831,1.,-2.19306710376111));
#51872=CARTESIAN_POINT('Ctrl Pts',(3.30848134694595,1.,-2.19906078949923));
#51873=CARTESIAN_POINT('Ctrl Pts',(3.31307424608949,1.,-2.20508863150607));
#51874=CARTESIAN_POINT('Ctrl Pts',(3.31764044024235,1.,-2.21115211847875));
#51875=CARTESIAN_POINT('Ctrl Pts',(3.32218125618968,1.,-2.21725135110898));
#51876=CARTESIAN_POINT('Ctrl Pts',(3.3266964672289,1.,-2.22338548312772));
#51877=CARTESIAN_POINT('Ctrl Pts',(3.33118487773611,1.,-2.22955308907233));
#51878=CARTESIAN_POINT('Ctrl Pts',(3.33564495756481,1.,-2.23575256328812));
#51879=CARTESIAN_POINT('Ctrl Pts',(3.34007543738025,1.,-2.24198249391422));
#51880=CARTESIAN_POINT('Ctrl Pts',(3.34447596770723,1.,-2.24824207678256));
#51881=CARTESIAN_POINT('Ctrl Pts',(3.34884690292285,1.,-2.25453097693483));
#51882=CARTESIAN_POINT('Ctrl Pts',(3.35318902552626,1.,-2.26084915222449));
#51883=CARTESIAN_POINT('Ctrl Pts',(3.35750328523061,1.,-2.2671966857991));
#51884=CARTESIAN_POINT('Ctrl Pts',(3.36179055004409,1.,-2.2735736262093));
#51885=CARTESIAN_POINT('Ctrl Pts',(3.36605130713076,1.,-2.27997979458037));
#51886=CARTESIAN_POINT('Ctrl Pts',(3.37028570206488,1.,-2.28641481081137));
#51887=CARTESIAN_POINT('Ctrl Pts',(3.37449367172826,1.,-2.29287818007393));
#51888=CARTESIAN_POINT('Ctrl Pts',(3.37867504959433,1.,-2.29936936127624));
#51889=CARTESIAN_POINT('Ctrl Pts',(3.3828296733661,1.,-2.30588783640343));
#51890=CARTESIAN_POINT('Ctrl Pts',(3.38695751492462,1.,-2.31243319489367));
#51891=CARTESIAN_POINT('Ctrl Pts',(3.39105869474822,1.,-2.31900513925424));
#51892=CARTESIAN_POINT('Ctrl Pts',(3.39513342019756,1.,-2.3256034390248));
#51893=CARTESIAN_POINT('Ctrl Pts',(3.39918194577956,1.,-2.33222789882489));
#51894=CARTESIAN_POINT('Ctrl Pts',(3.40320452776743,1.,-2.33887832342782));
#51895=CARTESIAN_POINT('Ctrl Pts',(3.40720137404297,1.,-2.34555447649188));
#51896=CARTESIAN_POINT('Ctrl Pts',(3.41117262314119,1.,-2.35225606824109));
#51897=CARTESIAN_POINT('Ctrl Pts',(3.41511836751469,1.,-2.35898278606946));
#51898=CARTESIAN_POINT('Ctrl Pts',(3.41903866635852,1.,-2.36573431470642));
#51899=CARTESIAN_POINT('Ctrl Pts',(3.42293356216511,1.,-2.37251035954292));
#51900=CARTESIAN_POINT('Ctrl Pts',(3.42680309754399,1.,-2.37931067028926));
#51901=CARTESIAN_POINT('Ctrl Pts',(3.43064732712919,1.,-2.38613505843552));
#51902=CARTESIAN_POINT('Ctrl Pts',(3.4344663067854,1.,-2.39298338804493));
#51903=CARTESIAN_POINT('Ctrl Pts',(3.43750133064416,1.,-2.39848113410292));
#51904=CARTESIAN_POINT('Ctrl Pts',(3.43976627484234,1.,-2.40261515589405));
#51905=CARTESIAN_POINT('Ctrl Pts',(3.44127120683039,1.,-2.4053759295909));
#51906=CARTESIAN_POINT('Ctrl Pts',(3.44202241512147,1.,-2.40675750623143));
#51907=CARTESIAN_POINT('Origin',(3.44202241512147,0.,-2.40675750623143));
#51908=CARTESIAN_POINT('',(3.35260583073571,1.,-2.52982887637028));
#51909=CARTESIAN_POINT('Origin',(0.,0.,0.));
#51910=CARTESIAN_POINT('',(3.24413672884812,1.,-1.88097764062697));
#51911=CARTESIAN_POINT('Origin',(0.,1.,0.));
#51912=CARTESIAN_POINT('Ctrl Pts',(3.24413672884812,1.,-1.88097764062697));
#51913=CARTESIAN_POINT('Ctrl Pts',(3.24413672884812,0.666666666666667,-1.88097764062697));
#51914=CARTESIAN_POINT('Ctrl Pts',(3.24413672884812,0.333333333333333,-1.88097764062697));
#51915=CARTESIAN_POINT('Ctrl Pts',(3.24413672884812,-0.333333333333333,
-1.88097764062697));
#51916=CARTESIAN_POINT('Ctrl Pts',(3.24413672884812,-0.666666666666667,
-1.88097764062697));
#51917=CARTESIAN_POINT('Ctrl Pts',(3.24413672884812,-1.,-1.88097764062697));
#51918=CARTESIAN_POINT('Ctrl Pts',(3.70708211654725,-1.,-1.97421938526992));
#51919=CARTESIAN_POINT('Ctrl Pts',(3.70708211654725,1.,-1.97421938526992));
#51920=CARTESIAN_POINT('Ctrl Pts',(3.70551008132332,-1.,-1.97417727645308));
#51921=CARTESIAN_POINT('Ctrl Pts',(3.70551008132332,1.,-1.97417727645308));
#51922=CARTESIAN_POINT('Ctrl Pts',(3.70236698912904,-1.,-1.97408973726715));
#51923=CARTESIAN_POINT('Ctrl Pts',(3.70236698912904,1.,-1.97408973726715));
#51924=CARTESIAN_POINT('Ctrl Pts',(3.6976552856004,-1.,-1.97394846383216));
#51925=CARTESIAN_POINT('Ctrl Pts',(3.6976552856004,1.,-1.97394846383216));
#51926=CARTESIAN_POINT('Ctrl Pts',(3.69137888599902,-1.,-1.97374016225483));
#51927=CARTESIAN_POINT('Ctrl Pts',(3.69137888599902,1.,-1.97374016225483));
#51928=CARTESIAN_POINT('Ctrl Pts',(3.68354319915092,-1.,-1.97344650304519));
#51929=CARTESIAN_POINT('Ctrl Pts',(3.68354319915092,1.,-1.97344650304519));
#51930=CARTESIAN_POINT('Ctrl Pts',(3.67571738107084,-1.,-1.97311947678517));
#51931=CARTESIAN_POINT('Ctrl Pts',(3.67571738107084,1.,-1.97311947678517));
#51932=CARTESIAN_POINT('Ctrl Pts',(3.66790152752075,-1.,-1.97275897198678));
#51933=CARTESIAN_POINT('Ctrl Pts',(3.66790152752075,1.,-1.97275897198678));
#51934=CARTESIAN_POINT('Ctrl Pts',(3.6600957816636,-1.,-1.9723648543905));
#51935=CARTESIAN_POINT('Ctrl Pts',(3.6600957816636,1.,-1.9723648543905));
#51936=CARTESIAN_POINT('Ctrl Pts',(3.652300347166,-1.,-1.9719369724024));
#51937=CARTESIAN_POINT('Ctrl Pts',(3.652300347166,1.,-1.9719369724024));
#51938=CARTESIAN_POINT('Ctrl Pts',(3.64451546723514,-1.,-1.97147515441164));
#51939=CARTESIAN_POINT('Ctrl Pts',(3.64451546723514,1.,-1.97147515441164));
#51940=CARTESIAN_POINT('Ctrl Pts',(3.63674139590412,-1.,-1.97097920454464));
#51941=CARTESIAN_POINT('Ctrl Pts',(3.63674139590412,1.,-1.97097920454464));
#51942=CARTESIAN_POINT('Ctrl Pts',(3.62897836973293,-1.,-1.97044889850463));
#51943=CARTESIAN_POINT('Ctrl Pts',(3.62897836973293,1.,-1.97044889850463));
#51944=CARTESIAN_POINT('Ctrl Pts',(3.62122658401893,-1.,-1.96988398129978));
#51945=CARTESIAN_POINT('Ctrl Pts',(3.62122658401893,1.,-1.96988398129978));
#51946=CARTESIAN_POINT('Ctrl Pts',(3.61348615496704,-1.,-1.96928416040877));
#51947=CARTESIAN_POINT('Ctrl Pts',(3.61348615496704,1.,-1.96928416040877));
#51948=CARTESIAN_POINT('Ctrl Pts',(3.60575714017989,-1.,-1.9686491188594));
#51949=CARTESIAN_POINT('Ctrl Pts',(3.60575714017989,1.,-1.9686491188594));
#51950=CARTESIAN_POINT('Ctrl Pts',(3.59803959819938,-1.,-1.96797854118369));
#51951=CARTESIAN_POINT('Ctrl Pts',(3.59803959819938,1.,-1.96797854118369));
#51952=CARTESIAN_POINT('Ctrl Pts',(3.59033364022801,-1.,-1.96727213799544));
#51953=CARTESIAN_POINT('Ctrl Pts',(3.59033364022801,1.,-1.96727213799544));
#51954=CARTESIAN_POINT('Ctrl Pts',(3.58263947663829,-1.,-1.96652966688911));
#51955=CARTESIAN_POINT('Ctrl Pts',(3.58263947663829,1.,-1.96652966688911));
#51956=CARTESIAN_POINT('Ctrl Pts',(3.57495748600959,-1.,-1.96575096652789));
#51957=CARTESIAN_POINT('Ctrl Pts',(3.57495748600959,1.,-1.96575096652789));
#51958=CARTESIAN_POINT('Ctrl Pts',(3.56728820357791,-1.,-1.96493594634567));
#51959=CARTESIAN_POINT('Ctrl Pts',(3.56728820357791,1.,-1.96493594634567));
#51960=CARTESIAN_POINT('Ctrl Pts',(3.55963218706096,-1.,-1.96408450906812));
#51961=CARTESIAN_POINT('Ctrl Pts',(3.55963218706096,1.,-1.96408450906812));
#51962=CARTESIAN_POINT('Ctrl Pts',(3.55198990600886,-1.,-1.96319648628644));
#51963=CARTESIAN_POINT('Ctrl Pts',(3.55198990600886,1.,-1.96319648628644));
#51964=CARTESIAN_POINT('Ctrl Pts',(3.54436163300443,-1.,-1.96227157573067));
#51965=CARTESIAN_POINT('Ctrl Pts',(3.54436163300443,1.,-1.96227157573067));
#51966=CARTESIAN_POINT('Ctrl Pts',(3.53674730625813,-1.,-1.96130926212689));
#51967=CARTESIAN_POINT('Ctrl Pts',(3.53674730625813,1.,-1.96130926212689));
#51968=CARTESIAN_POINT('Ctrl Pts',(3.52914648844351,-1.,-1.96030879411566));
#51969=CARTESIAN_POINT('Ctrl Pts',(3.52914648844351,1.,-1.96030879411566));
#51970=CARTESIAN_POINT('Ctrl Pts',(3.52155867431486,-1.,-1.95926936324461));
#51971=CARTESIAN_POINT('Ctrl Pts',(3.52155867431486,1.,-1.95926936324461));
#51972=CARTESIAN_POINT('Ctrl Pts',(3.51398354617794,-1.,-1.95819025316779));
#51973=CARTESIAN_POINT('Ctrl Pts',(3.51398354617794,1.,-1.95819025316779));
#51974=CARTESIAN_POINT('Ctrl Pts',(3.50642124159909,-1.,-1.95707099606511));
#51975=CARTESIAN_POINT('Ctrl Pts',(3.50642124159909,1.,-1.95707099606511));
#51976=CARTESIAN_POINT('Ctrl Pts',(3.49887263575583,-1.,-1.95591153823661));
#51977=CARTESIAN_POINT('Ctrl Pts',(3.49887263575583,1.,-1.95591153823661));
#51978=CARTESIAN_POINT('Ctrl Pts',(3.49133956289133,-1.,-1.95471236969643));
#51979=CARTESIAN_POINT('Ctrl Pts',(3.49133956289133,1.,-1.95471236969643));
#51980=CARTESIAN_POINT('Ctrl Pts',(3.48382414832634,-1.,-1.95347412486309));
#51981=CARTESIAN_POINT('Ctrl Pts',(3.48382414832634,1.,-1.95347412486309));
#51982=CARTESIAN_POINT('Ctrl Pts',(3.47632820495921,-1.,-1.95219722189876));
#51983=CARTESIAN_POINT('Ctrl Pts',(3.47632820495921,1.,-1.95219722189876));
#51984=CARTESIAN_POINT('Ctrl Pts',(3.46885258974191,-1.,-1.95088147859877));
#51985=CARTESIAN_POINT('Ctrl Pts',(3.46885258974191,1.,-1.95088147859877));
#51986=CARTESIAN_POINT('Ctrl Pts',(3.46139661060962,-1.,-1.94952575850197));
#51987=CARTESIAN_POINT('Ctrl Pts',(3.46139661060962,1.,-1.94952575850197));
#51988=CARTESIAN_POINT('Ctrl Pts',(3.45395731584051,-1.,-1.94812754766524));
#51989=CARTESIAN_POINT('Ctrl Pts',(3.45395731584051,1.,-1.94812754766524));
#51990=CARTESIAN_POINT('Ctrl Pts',(3.44653088665681,-1.,-1.94668377715329));
#51991=CARTESIAN_POINT('Ctrl Pts',(3.44653088665681,1.,-1.94668377715329));
#51992=CARTESIAN_POINT('Ctrl Pts',(3.43911410197687,-1.,-1.94519168842879));
#51993=CARTESIAN_POINT('Ctrl Pts',(3.43911410197687,1.,-1.94519168842879));
#51994=CARTESIAN_POINT('Ctrl Pts',(3.43170586602434,-1.,-1.94364973660284));
#51995=CARTESIAN_POINT('Ctrl Pts',(3.43170586602434,1.,-1.94364973660284));
#51996=CARTESIAN_POINT('Ctrl Pts',(3.42430850941503,-1.,-1.94205835913696));
#51997=CARTESIAN_POINT('Ctrl Pts',(3.42430850941503,1.,-1.94205835913696));
#51998=CARTESIAN_POINT('Ctrl Pts',(3.41692971994096,-1.,-1.94042111965246));
#51999=CARTESIAN_POINT('Ctrl Pts',(3.41692971994096,1.,-1.94042111965246));
#52000=CARTESIAN_POINT('Ctrl Pts',(3.40957978266642,-1.,-1.93874306008143));
#52001=CARTESIAN_POINT('Ctrl Pts',(3.40957978266642,1.,-1.93874306008143));
#52002=CARTESIAN_POINT('Ctrl Pts',(3.40226802104109,-1.,-1.93702857723098));
#52003=CARTESIAN_POINT('Ctrl Pts',(3.40226802104109,1.,-1.93702857723098));
#52004=CARTESIAN_POINT('Ctrl Pts',(3.39499923640795,-1.,-1.93527929945985));
#52005=CARTESIAN_POINT('Ctrl Pts',(3.39499923640795,1.,-1.93527929945985));
#52006=CARTESIAN_POINT('Ctrl Pts',(3.38777076883256,-1.,-1.93349233176788));
#52007=CARTESIAN_POINT('Ctrl Pts',(3.38777076883256,1.,-1.93349233176788));
#52008=CARTESIAN_POINT('Ctrl Pts',(3.3805676852555,-1.,-1.93165739093276));
#52009=CARTESIAN_POINT('Ctrl Pts',(3.3805676852555,1.,-1.93165739093276));
#52010=CARTESIAN_POINT('Ctrl Pts',(3.37336807068043,-1.,-1.92975993109877));
#52011=CARTESIAN_POINT('Ctrl Pts',(3.37336807068043,1.,-1.92975993109877));
#52012=CARTESIAN_POINT('Ctrl Pts',(3.36615168657567,-1.,-1.92778626543786));
#52013=CARTESIAN_POINT('Ctrl Pts',(3.36615168657567,1.,-1.92778626543786));
#52014=CARTESIAN_POINT('Ctrl Pts',(3.35890824422965,-1.,-1.92572846125756));
#52015=CARTESIAN_POINT('Ctrl Pts',(3.35890824422965,1.,-1.92572846125756));
#52016=CARTESIAN_POINT('Ctrl Pts',(3.35164424847223,-1.,-1.92358838440528));
#52017=CARTESIAN_POINT('Ctrl Pts',(3.35164424847223,1.,-1.92358838440528));
#52018=CARTESIAN_POINT('Ctrl Pts',(3.34439448941961,-1.,-1.92138450828404));
#52019=CARTESIAN_POINT('Ctrl Pts',(3.34439448941961,1.,-1.92138450828404));
#52020=CARTESIAN_POINT('Ctrl Pts',(3.33721230710012,-1.,-1.9191460961021));
#52021=CARTESIAN_POINT('Ctrl Pts',(3.33721230710012,1.,-1.9191460961021));
#52022=CARTESIAN_POINT('Ctrl Pts',(3.33014884257873,-1.,-1.91690081930332));
#52023=CARTESIAN_POINT('Ctrl Pts',(3.33014884257873,1.,-1.91690081930332));
#52024=CARTESIAN_POINT('Ctrl Pts',(3.32323403454535,-1.,-1.91466343916628));
#52025=CARTESIAN_POINT('Ctrl Pts',(3.32323403454535,1.,-1.91466343916628));
#52026=CARTESIAN_POINT('Ctrl Pts',(3.31646052426364,-1.,-1.91242616234442));
#52027=CARTESIAN_POINT('Ctrl Pts',(3.31646052426364,1.,-1.91242616234442));
#52028=CARTESIAN_POINT('Ctrl Pts',(3.30975721158596,-1.,-1.91014297830446));
#52029=CARTESIAN_POINT('Ctrl Pts',(3.30975721158596,1.,-1.91014297830446));
#52030=CARTESIAN_POINT('Ctrl Pts',(3.30300595568195,-1.,-1.90773912171341));
#52031=CARTESIAN_POINT('Ctrl Pts',(3.30300595568195,1.,-1.90773912171341));
#52032=CARTESIAN_POINT('Ctrl Pts',(3.29608978722113,-1.,-1.90513891864087));
#52033=CARTESIAN_POINT('Ctrl Pts',(3.29608978722113,1.,-1.90513891864087));
#52034=CARTESIAN_POINT('Ctrl Pts',(3.2889344860029,-1.,-1.90228971247527));
#52035=CARTESIAN_POINT('Ctrl Pts',(3.2889344860029,1.,-1.90228971247527));
#52036=CARTESIAN_POINT('Ctrl Pts',(3.28154737912352,-1.,-1.89918429230462));
#52037=CARTESIAN_POINT('Ctrl Pts',(3.28154737912352,1.,-1.89918429230462));
#52038=CARTESIAN_POINT('Ctrl Pts',(3.27407108933139,-1.,-1.89589172903793));
#52039=CARTESIAN_POINT('Ctrl Pts',(3.27407108933139,1.,-1.89589172903793));
#52040=CARTESIAN_POINT('Ctrl Pts',(3.26677653888676,-1.,-1.89255393500965));
#52041=CARTESIAN_POINT('Ctrl Pts',(3.26677653888676,1.,-1.89255393500965));
#52042=CARTESIAN_POINT('Ctrl Pts',(3.25999885193947,-1.,-1.88934996203698));
#52043=CARTESIAN_POINT('Ctrl Pts',(3.25999885193947,1.,-1.88934996203698));
#52044=CARTESIAN_POINT('Ctrl Pts',(3.25408686339463,-1.,-1.88646802523466));
#52045=CARTESIAN_POINT('Ctrl Pts',(3.25408686339463,1.,-1.88646802523466));
#52046=CARTESIAN_POINT('Ctrl Pts',(3.24935200511918,-1.,-1.88407708646357));
#52047=CARTESIAN_POINT('Ctrl Pts',(3.24935200511918,1.,-1.88407708646357));
#52048=CARTESIAN_POINT('Ctrl Pts',(3.24600543790443,-1.,-1.88229202582941));
#52049=CARTESIAN_POINT('Ctrl Pts',(3.24600543790443,1.,-1.88229202582941));
#52050=CARTESIAN_POINT('Ctrl Pts',(3.24451807186481,-1.,-1.88139187908074));
#52051=CARTESIAN_POINT('Ctrl Pts',(3.24451807186481,1.,-1.88139187908074));
#52052=CARTESIAN_POINT('Ctrl Pts',(3.24408699284121,-1.,-1.88102201872555));
#52053=CARTESIAN_POINT('Ctrl Pts',(3.24408699284121,1.,-1.88102201872555));
#52054=CARTESIAN_POINT('Ctrl Pts',(3.24410359189609,-1.,-1.88091100680349));
#52055=CARTESIAN_POINT('Ctrl Pts',(3.24410359189609,1.,-1.88091100680349));
#52056=CARTESIAN_POINT('Ctrl Pts',(3.24418789321065,-1.,-1.8808893942881));
#52057=CARTESIAN_POINT('Ctrl Pts',(3.24418789321065,1.,-1.8808893942881));
#52058=CARTESIAN_POINT('',(3.70708211654725,1.,-1.97421938526992));
#52059=CARTESIAN_POINT('Ctrl Pts',(3.70708211654725,1.,-1.97421938526992));
#52060=CARTESIAN_POINT('Ctrl Pts',(3.70551008132332,1.,-1.97417727645308));
#52061=CARTESIAN_POINT('Ctrl Pts',(3.70236698912904,1.,-1.97408973726715));
#52062=CARTESIAN_POINT('Ctrl Pts',(3.6976552856004,1.,-1.97394846383216));
#52063=CARTESIAN_POINT('Ctrl Pts',(3.69137888599902,1.,-1.97374016225483));
#52064=CARTESIAN_POINT('Ctrl Pts',(3.68354319915092,1.,-1.97344650304519));
#52065=CARTESIAN_POINT('Ctrl Pts',(3.67571738107084,1.,-1.97311947678517));
#52066=CARTESIAN_POINT('Ctrl Pts',(3.66790152752075,1.,-1.97275897198678));
#52067=CARTESIAN_POINT('Ctrl Pts',(3.6600957816636,1.,-1.9723648543905));
#52068=CARTESIAN_POINT('Ctrl Pts',(3.652300347166,1.,-1.9719369724024));
#52069=CARTESIAN_POINT('Ctrl Pts',(3.64451546723514,1.,-1.97147515441164));
#52070=CARTESIAN_POINT('Ctrl Pts',(3.63674139590412,1.,-1.97097920454464));
#52071=CARTESIAN_POINT('Ctrl Pts',(3.62897836973293,1.,-1.97044889850463));
#52072=CARTESIAN_POINT('Ctrl Pts',(3.62122658401893,1.,-1.96988398129978));
#52073=CARTESIAN_POINT('Ctrl Pts',(3.61348615496704,1.,-1.96928416040877));
#52074=CARTESIAN_POINT('Ctrl Pts',(3.60575714017989,1.,-1.9686491188594));
#52075=CARTESIAN_POINT('Ctrl Pts',(3.59803959819938,1.,-1.96797854118369));
#52076=CARTESIAN_POINT('Ctrl Pts',(3.59033364022801,1.,-1.96727213799544));
#52077=CARTESIAN_POINT('Ctrl Pts',(3.58263947663829,1.,-1.96652966688911));
#52078=CARTESIAN_POINT('Ctrl Pts',(3.57495748600959,1.,-1.96575096652789));
#52079=CARTESIAN_POINT('Ctrl Pts',(3.56728820357791,1.,-1.96493594634567));
#52080=CARTESIAN_POINT('Ctrl Pts',(3.55963218706096,1.,-1.96408450906812));
#52081=CARTESIAN_POINT('Ctrl Pts',(3.55198990600886,1.,-1.96319648628644));
#52082=CARTESIAN_POINT('Ctrl Pts',(3.54436163300443,1.,-1.96227157573067));
#52083=CARTESIAN_POINT('Ctrl Pts',(3.53674730625813,1.,-1.96130926212689));
#52084=CARTESIAN_POINT('Ctrl Pts',(3.52914648844351,1.,-1.96030879411566));
#52085=CARTESIAN_POINT('Ctrl Pts',(3.52155867431486,1.,-1.95926936324461));
#52086=CARTESIAN_POINT('Ctrl Pts',(3.51398354617794,1.,-1.95819025316779));
#52087=CARTESIAN_POINT('Ctrl Pts',(3.50642124159909,1.,-1.95707099606511));
#52088=CARTESIAN_POINT('Ctrl Pts',(3.49887263575583,1.,-1.95591153823661));
#52089=CARTESIAN_POINT('Ctrl Pts',(3.49133956289133,1.,-1.95471236969643));
#52090=CARTESIAN_POINT('Ctrl Pts',(3.48382414832634,1.,-1.95347412486309));
#52091=CARTESIAN_POINT('Ctrl Pts',(3.47632820495921,1.,-1.95219722189876));
#52092=CARTESIAN_POINT('Ctrl Pts',(3.46885258974191,1.,-1.95088147859877));
#52093=CARTESIAN_POINT('Ctrl Pts',(3.46139661060962,1.,-1.94952575850197));
#52094=CARTESIAN_POINT('Ctrl Pts',(3.45395731584051,1.,-1.94812754766524));
#52095=CARTESIAN_POINT('Ctrl Pts',(3.44653088665681,1.,-1.94668377715329));
#52096=CARTESIAN_POINT('Ctrl Pts',(3.43911410197687,1.,-1.94519168842879));
#52097=CARTESIAN_POINT('Ctrl Pts',(3.43170586602434,1.,-1.94364973660284));
#52098=CARTESIAN_POINT('Ctrl Pts',(3.42430850941503,1.,-1.94205835913696));
#52099=CARTESIAN_POINT('Ctrl Pts',(3.41692971994096,1.,-1.94042111965246));
#52100=CARTESIAN_POINT('Ctrl Pts',(3.40957978266642,1.,-1.93874306008143));
#52101=CARTESIAN_POINT('Ctrl Pts',(3.40226802104109,1.,-1.93702857723098));
#52102=CARTESIAN_POINT('Ctrl Pts',(3.39499923640795,1.,-1.93527929945985));
#52103=CARTESIAN_POINT('Ctrl Pts',(3.38777076883256,1.,-1.93349233176788));
#52104=CARTESIAN_POINT('Ctrl Pts',(3.3805676852555,1.,-1.93165739093276));
#52105=CARTESIAN_POINT('Ctrl Pts',(3.37336807068043,1.,-1.92975993109877));
#52106=CARTESIAN_POINT('Ctrl Pts',(3.36615168657567,1.,-1.92778626543786));
#52107=CARTESIAN_POINT('Ctrl Pts',(3.35890824422965,1.,-1.92572846125756));
#52108=CARTESIAN_POINT('Ctrl Pts',(3.35164424847223,1.,-1.92358838440528));
#52109=CARTESIAN_POINT('Ctrl Pts',(3.34439448941961,1.,-1.92138450828404));
#52110=CARTESIAN_POINT('Ctrl Pts',(3.33721230710012,1.,-1.9191460961021));
#52111=CARTESIAN_POINT('Ctrl Pts',(3.33014884257873,1.,-1.91690081930332));
#52112=CARTESIAN_POINT('Ctrl Pts',(3.32323403454535,1.,-1.91466343916628));
#52113=CARTESIAN_POINT('Ctrl Pts',(3.31646052426364,1.,-1.91242616234442));
#52114=CARTESIAN_POINT('Ctrl Pts',(3.30975721158596,1.,-1.91014297830446));
#52115=CARTESIAN_POINT('Ctrl Pts',(3.30300595568195,1.,-1.90773912171341));
#52116=CARTESIAN_POINT('Ctrl Pts',(3.29608978722113,1.,-1.90513891864087));
#52117=CARTESIAN_POINT('Ctrl Pts',(3.2889344860029,1.,-1.90228971247527));
#52118=CARTESIAN_POINT('Ctrl Pts',(3.28154737912352,1.,-1.89918429230462));
#52119=CARTESIAN_POINT('Ctrl Pts',(3.27407108933139,1.,-1.89589172903793));
#52120=CARTESIAN_POINT('Ctrl Pts',(3.26677653888676,1.,-1.89255393500965));
#52121=CARTESIAN_POINT('Ctrl Pts',(3.25999885193947,1.,-1.88934996203698));
#52122=CARTESIAN_POINT('Ctrl Pts',(3.25408686339463,1.,-1.88646802523466));
#52123=CARTESIAN_POINT('Ctrl Pts',(3.24935200511918,1.,-1.88407708646357));
#52124=CARTESIAN_POINT('Ctrl Pts',(3.2462565441079,1.,-1.88242596600454));
#52125=CARTESIAN_POINT('Ctrl Pts',(3.24480754676064,1.,-1.88156537699203));
#52126=CARTESIAN_POINT('Ctrl Pts',(3.24428080353022,1.,-1.88117508446775));
#52127=CARTESIAN_POINT('Ctrl Pts',(3.24415531671284,1.,-1.8810229239812));
#52128=CARTESIAN_POINT('Ctrl Pts',(3.24413672884812,1.,-1.88097764062697));
#52129=CARTESIAN_POINT('',(3.70708211654725,0.,-1.97421938526992));
#52130=CARTESIAN_POINT('Ctrl Pts',(3.42855728381368,-1.,-1.519044091397));
#52131=CARTESIAN_POINT('Ctrl Pts',(3.42855728381368,1.,-1.519044091397));
#52132=CARTESIAN_POINT('Ctrl Pts',(3.42852521763778,-1.,-1.51896318668366));
#52133=CARTESIAN_POINT('Ctrl Pts',(3.42852521763778,1.,-1.51896318668366));
#52134=CARTESIAN_POINT('Ctrl Pts',(3.42860527149177,-1.,-1.51888450659652));
#52135=CARTESIAN_POINT('Ctrl Pts',(3.42860527149177,1.,-1.51888450659652));
#52136=CARTESIAN_POINT('Ctrl Pts',(3.42915787669893,-1.,-1.51901585839109));
#52137=CARTESIAN_POINT('Ctrl Pts',(3.42915787669893,1.,-1.51901585839109));
#52138=CARTESIAN_POINT('Ctrl Pts',(3.43076036253837,-1.,-1.51969006980999));
#52139=CARTESIAN_POINT('Ctrl Pts',(3.43076036253837,1.,-1.51969006980999));
#52140=CARTESIAN_POINT('Ctrl Pts',(3.43417156977893,-1.,-1.52134826724293));
#52141=CARTESIAN_POINT('Ctrl Pts',(3.43417156977893,1.,-1.52134826724293));
#52142=CARTESIAN_POINT('Ctrl Pts',(3.4388889597401,-1.,-1.5237734895035));
#52143=CARTESIAN_POINT('Ctrl Pts',(3.4388889597401,1.,-1.5237734895035));
#52144=CARTESIAN_POINT('Ctrl Pts',(3.44469547526647,-1.,-1.52686242875556));
#52145=CARTESIAN_POINT('Ctrl Pts',(3.44469547526647,1.,-1.52686242875556));
#52146=CARTESIAN_POINT('Ctrl Pts',(3.45127136828305,-1.,-1.53046244461635));
#52147=CARTESIAN_POINT('Ctrl Pts',(3.45127136828305,1.,-1.53046244461635));
#52148=CARTESIAN_POINT('Ctrl Pts',(3.45825932955032,-1.,-1.53440195378792));
#52149=CARTESIAN_POINT('Ctrl Pts',(3.45825932955032,1.,-1.53440195378792));
#52150=CARTESIAN_POINT('Ctrl Pts',(3.46531752207153,-1.,-1.53851507915502));
#52151=CARTESIAN_POINT('Ctrl Pts',(3.46531752207153,1.,-1.53851507915502));
#52152=CARTESIAN_POINT('Ctrl Pts',(3.47217189224653,-1.,-1.54266605398188));
#52153=CARTESIAN_POINT('Ctrl Pts',(3.47217189224653,1.,-1.54266605398188));
#52154=CARTESIAN_POINT('Ctrl Pts',(3.47868272898751,-1.,-1.54678009290276));
#52155=CARTESIAN_POINT('Ctrl Pts',(3.47868272898751,1.,-1.54678009290276));
#52156=CARTESIAN_POINT('Ctrl Pts',(3.48485155928567,-1.,-1.55084702970452));
#52157=CARTESIAN_POINT('Ctrl Pts',(3.48485155928567,1.,-1.55084702970452));
#52158=CARTESIAN_POINT('Ctrl Pts',(3.4907646087742,-1.,-1.55489595901116));
#52159=CARTESIAN_POINT('Ctrl Pts',(3.4907646087742,1.,-1.55489595901116));
#52160=CARTESIAN_POINT('Ctrl Pts',(3.49655185179655,-1.,-1.55897703097874));
#52161=CARTESIAN_POINT('Ctrl Pts',(3.49655185179655,1.,-1.55897703097874));
#52162=CARTESIAN_POINT('Ctrl Pts',(3.50234321621578,-1.,-1.56314187758675));
#52163=CARTESIAN_POINT('Ctrl Pts',(3.50234321621578,1.,-1.56314187758675));
#52164=CARTESIAN_POINT('Ctrl Pts',(3.50821771695363,-1.,-1.56742097575012));
#52165=CARTESIAN_POINT('Ctrl Pts',(3.50821771695363,1.,-1.56742097575012));
#52166=CARTESIAN_POINT('Ctrl Pts',(3.51418598431665,-1.,-1.57181569799743));
#52167=CARTESIAN_POINT('Ctrl Pts',(3.51418598431665,1.,-1.57181569799743));
#52168=CARTESIAN_POINT('Ctrl Pts',(3.52021847865912,-1.,-1.57631049988158));
#52169=CARTESIAN_POINT('Ctrl Pts',(3.52021847865912,1.,-1.57631049988158));
#52170=CARTESIAN_POINT('Ctrl Pts',(3.52626275334881,-1.,-1.58088027227848));
#52171=CARTESIAN_POINT('Ctrl Pts',(3.52626275334881,1.,-1.58088027227848));
#52172=CARTESIAN_POINT('Ctrl Pts',(3.5322637814708,-1.,-1.58549906268088));
#52173=CARTESIAN_POINT('Ctrl Pts',(3.5322637814708,1.,-1.58549906268088));
#52174=CARTESIAN_POINT('Ctrl Pts',(3.53818616861077,-1.,-1.59014958368739));
#52175=CARTESIAN_POINT('Ctrl Pts',(3.53818616861077,1.,-1.59014958368739));
#52176=CARTESIAN_POINT('Ctrl Pts',(3.54402458182337,-1.,-1.59482766949766));
#52177=CARTESIAN_POINT('Ctrl Pts',(3.54402458182337,1.,-1.59482766949766));
#52178=CARTESIAN_POINT('Ctrl Pts',(3.54979148634454,-1.,-1.59953698113457));
#52179=CARTESIAN_POINT('Ctrl Pts',(3.54979148634454,1.,-1.59953698113457));
#52180=CARTESIAN_POINT('Ctrl Pts',(3.55550985096129,-1.,-1.60428584699853));
#52181=CARTESIAN_POINT('Ctrl Pts',(3.55550985096129,1.,-1.60428584699853));
#52182=CARTESIAN_POINT('Ctrl Pts',(3.5612043248298,-1.,-1.60908344685457));
#52183=CARTESIAN_POINT('Ctrl Pts',(3.5612043248298,1.,-1.60908344685457));
#52184=CARTESIAN_POINT('Ctrl Pts',(3.56689200468387,-1.,-1.61393581747514));
#52185=CARTESIAN_POINT('Ctrl Pts',(3.56689200468387,1.,-1.61393581747514));
#52186=CARTESIAN_POINT('Ctrl Pts',(3.57257679609806,-1.,-1.61884340915404));
#52187=CARTESIAN_POINT('Ctrl Pts',(3.57257679609806,1.,-1.61884340915404));
#52188=CARTESIAN_POINT('Ctrl Pts',(3.5782545595439,-1.,-1.62380329464844));
#52189=CARTESIAN_POINT('Ctrl Pts',(3.5782545595439,1.,-1.62380329464844));
#52190=CARTESIAN_POINT('Ctrl Pts',(3.58391625774343,-1.,-1.62881051550745));
#52191=CARTESIAN_POINT('Ctrl Pts',(3.58391625774343,1.,-1.62881051550745));
#52192=CARTESIAN_POINT('Ctrl Pts',(3.58955176627879,-1.,-1.6338597145126));
#52193=CARTESIAN_POINT('Ctrl Pts',(3.58955176627879,1.,-1.6338597145126));
#52194=CARTESIAN_POINT('Ctrl Pts',(3.59515368334893,-1.,-1.63894676675352));
#52195=CARTESIAN_POINT('Ctrl Pts',(3.59515368334893,1.,-1.63894676675352));
#52196=CARTESIAN_POINT('Ctrl Pts',(3.60072028513845,-1.,-1.64407004385582));
#52197=CARTESIAN_POINT('Ctrl Pts',(3.60072028513845,1.,-1.64407004385582));
#52198=CARTESIAN_POINT('Ctrl Pts',(3.60625346556992,-1.,-1.64922952425832));
#52199=CARTESIAN_POINT('Ctrl Pts',(3.60625346556992,1.,-1.64922952425832));
#52200=CARTESIAN_POINT('Ctrl Pts',(3.61175734965127,-1.,-1.65442619244325));
#52201=CARTESIAN_POINT('Ctrl Pts',(3.61175734965127,1.,-1.65442619244325));
#52202=CARTESIAN_POINT('Ctrl Pts',(3.61723666482456,-1.,-1.65966133399186));
#52203=CARTESIAN_POINT('Ctrl Pts',(3.61723666482456,1.,-1.65966133399186));
#52204=CARTESIAN_POINT('Ctrl Pts',(3.62269517989109,-1.,-1.66493585923855));
#52205=CARTESIAN_POINT('Ctrl Pts',(3.62269517989109,1.,-1.66493585923855));
#52206=CARTESIAN_POINT('Ctrl Pts',(3.62813422105271,-1.,-1.67024966008045));
#52207=CARTESIAN_POINT('Ctrl Pts',(3.62813422105271,1.,-1.67024966008045));
#52208=CARTESIAN_POINT('Ctrl Pts',(3.63355343201232,-1.,-1.67560193613156));
#52209=CARTESIAN_POINT('Ctrl Pts',(3.63355343201232,1.,-1.67560193613156));
#52210=CARTESIAN_POINT('Ctrl Pts',(3.63895140887462,-1.,-1.68099146651586));
#52211=CARTESIAN_POINT('Ctrl Pts',(3.63895140887462,1.,-1.68099146651586));
#52212=CARTESIAN_POINT('Ctrl Pts',(3.64432638915203,-1.,-1.68641690471457));
#52213=CARTESIAN_POINT('Ctrl Pts',(3.64432638915203,1.,-1.68641690471457));
#52214=CARTESIAN_POINT('Ctrl Pts',(3.64967689827371,-1.,-1.69187705481689));
#52215=CARTESIAN_POINT('Ctrl Pts',(3.64967689827371,1.,-1.69187705481689));
#52216=CARTESIAN_POINT('Ctrl Pts',(3.65500246526749,-1.,-1.69737117722534));
#52217=CARTESIAN_POINT('Ctrl Pts',(3.65500246526749,1.,-1.69737117722534));
#52218=CARTESIAN_POINT('Ctrl Pts',(3.66030338774847,-1.,-1.70289888566873));
#52219=CARTESIAN_POINT('Ctrl Pts',(3.66030338774847,1.,-1.70289888566873));
#52220=CARTESIAN_POINT('Ctrl Pts',(3.66558043198876,-1.,-1.70846001610956));
#52221=CARTESIAN_POINT('Ctrl Pts',(3.66558043198876,1.,-1.70846001610956));
#52222=CARTESIAN_POINT('Ctrl Pts',(3.67083454901611,-1.,-1.71405450210384));
#52223=CARTESIAN_POINT('Ctrl Pts',(3.67083454901611,1.,-1.71405450210384));
#52224=CARTESIAN_POINT('Ctrl Pts',(3.67606660374709,-1.,-1.71968225581808));
#52225=CARTESIAN_POINT('Ctrl Pts',(3.67606660374709,1.,-1.71968225581808));
#52226=CARTESIAN_POINT('Ctrl Pts',(3.68127704936579,-1.,-1.72534302437056));
#52227=CARTESIAN_POINT('Ctrl Pts',(3.68127704936579,1.,-1.72534302437056));
#52228=CARTESIAN_POINT('Ctrl Pts',(3.68646597019332,-1.,-1.73103640956717));
#52229=CARTESIAN_POINT('Ctrl Pts',(3.68646597019332,1.,-1.73103640956717));
#52230=CARTESIAN_POINT('Ctrl Pts',(3.69163322648036,-1.,-1.73676193254557));
#52231=CARTESIAN_POINT('Ctrl Pts',(3.69163322648036,1.,-1.73676193254557));
#52232=CARTESIAN_POINT('Ctrl Pts',(3.69677856910517,-1.,-1.74251908492617));
#52233=CARTESIAN_POINT('Ctrl Pts',(3.69677856910517,1.,-1.74251908492617));
#52234=CARTESIAN_POINT('Ctrl Pts',(3.7019017567335,-1.,-1.74830738046057));
#52235=CARTESIAN_POINT('Ctrl Pts',(3.7019017567335,1.,-1.74830738046057));
#52236=CARTESIAN_POINT('Ctrl Pts',(3.70700269736659,-1.,-1.75412641804042));
#52237=CARTESIAN_POINT('Ctrl Pts',(3.70700269736659,1.,-1.75412641804042));
#52238=CARTESIAN_POINT('Ctrl Pts',(3.71208146346136,-1.,-1.75997588498865));
#52239=CARTESIAN_POINT('Ctrl Pts',(3.71208146346136,1.,-1.75997588498865));
#52240=CARTESIAN_POINT('Ctrl Pts',(3.71713822377359,-1.,-1.76585552124394));
#52241=CARTESIAN_POINT('Ctrl Pts',(3.71713822377359,1.,-1.76585552124394));
#52242=CARTESIAN_POINT('Ctrl Pts',(3.72217319911254,-1.,-1.77176509401761));
#52243=CARTESIAN_POINT('Ctrl Pts',(3.72217319911254,1.,-1.77176509401761));
#52244=CARTESIAN_POINT('Ctrl Pts',(3.72718661205609,-1.,-1.77770437039658));
#52245=CARTESIAN_POINT('Ctrl Pts',(3.72718661205609,1.,-1.77770437039658));
#52246=CARTESIAN_POINT('Ctrl Pts',(3.7321786309547,-1.,-1.78367308442901));
#52247=CARTESIAN_POINT('Ctrl Pts',(3.7321786309547,1.,-1.78367308442901));
#52248=CARTESIAN_POINT('Ctrl Pts',(3.73714934730681,-1.,-1.78967092823491));
#52249=CARTESIAN_POINT('Ctrl Pts',(3.73714934730681,1.,-1.78967092823491));
#52250=CARTESIAN_POINT('Ctrl Pts',(3.74209880352445,-1.,-1.79569757859422));
#52251=CARTESIAN_POINT('Ctrl Pts',(3.74209880352445,1.,-1.79569757859422));
#52252=CARTESIAN_POINT('Ctrl Pts',(3.74702700875467,-1.,-1.8017527148577));
#52253=CARTESIAN_POINT('Ctrl Pts',(3.74702700875467,1.,-1.8017527148577));
#52254=CARTESIAN_POINT('Ctrl Pts',(3.75193395887977,-1.,-1.80783603939617));
#52255=CARTESIAN_POINT('Ctrl Pts',(3.75193395887977,1.,-1.80783603939617));
#52256=CARTESIAN_POINT('Ctrl Pts',(3.75681965683071,-1.,-1.8139472983358));
#52257=CARTESIAN_POINT('Ctrl Pts',(3.75681965683071,1.,-1.8139472983358));
#52258=CARTESIAN_POINT('Ctrl Pts',(3.76168412707948,-1.,-1.82008629694091));
#52259=CARTESIAN_POINT('Ctrl Pts',(3.76168412707948,1.,-1.82008629694091));
#52260=CARTESIAN_POINT('Ctrl Pts',(3.76652740353775,-1.,-1.82625289220915));
#52261=CARTESIAN_POINT('Ctrl Pts',(3.76652740353775,1.,-1.82625289220915));
#52262=CARTESIAN_POINT('Ctrl Pts',(3.77038509817999,-1.,-1.83120816955646));
#52263=CARTESIAN_POINT('Ctrl Pts',(3.77038509817999,1.,-1.83120816955646));
#52264=CARTESIAN_POINT('Ctrl Pts',(3.77326886064398,-1.,-1.83493697934534));
#52265=CARTESIAN_POINT('Ctrl Pts',(3.77326886064398,1.,-1.83493697934534));
#52266=CARTESIAN_POINT('Ctrl Pts',(3.77518714457833,-1.,-1.83742834010626));
#52267=CARTESIAN_POINT('Ctrl Pts',(3.77518714457833,1.,-1.83742834010626));
#52268=CARTESIAN_POINT('Ctrl Pts',(3.77614523045147,-1.,-1.83867539237861));
#52269=CARTESIAN_POINT('Ctrl Pts',(3.77614523045147,1.,-1.83867539237861));
#52270=CARTESIAN_POINT('',(3.42859860294306,1.,-1.5189508286633));
#52271=CARTESIAN_POINT('Ctrl Pts',(3.42859860294306,-1.,-1.5189508286633));
#52272=CARTESIAN_POINT('Ctrl Pts',(3.42859860294306,-0.666666666666667,
-1.5189508286633));
#52273=CARTESIAN_POINT('Ctrl Pts',(3.42859860294306,-0.333333333333333,
-1.5189508286633));
#52274=CARTESIAN_POINT('Ctrl Pts',(3.42859860294306,0.333333333333333,-1.5189508286633));
#52275=CARTESIAN_POINT('Ctrl Pts',(3.42859860294306,0.666666666666667,-1.5189508286633));
#52276=CARTESIAN_POINT('Ctrl Pts',(3.42859860294306,1.,-1.5189508286633));
#52277=CARTESIAN_POINT('',(3.77614523045147,1.,-1.83867539237861));
#52278=CARTESIAN_POINT('',(3.77614523045147,0.,-1.83867539237861));
#52279=CARTESIAN_POINT('Ctrl Pts',(3.42859860294306,1.,-1.5189508286633));
#52280=CARTESIAN_POINT('Ctrl Pts',(3.42864616361875,1.,-1.51893924967331));
#52281=CARTESIAN_POINT('Ctrl Pts',(3.42884302333841,1.,-1.5189513329503));
#52282=CARTESIAN_POINT('Ctrl Pts',(3.42946838852588,1.,-1.51914806898491));
#52283=CARTESIAN_POINT('Ctrl Pts',(3.43101631893414,1.,-1.5198144909338));
#52284=CARTESIAN_POINT('Ctrl Pts',(3.43417156977893,1.,-1.52134826724293));
#52285=CARTESIAN_POINT('Ctrl Pts',(3.4388889597401,1.,-1.5237734895035));
#52286=CARTESIAN_POINT('Ctrl Pts',(3.44469547526647,1.,-1.52686242875556));
#52287=CARTESIAN_POINT('Ctrl Pts',(3.45127136828305,1.,-1.53046244461635));
#52288=CARTESIAN_POINT('Ctrl Pts',(3.45825932955032,1.,-1.53440195378792));
#52289=CARTESIAN_POINT('Ctrl Pts',(3.46531752207153,1.,-1.53851507915502));
#52290=CARTESIAN_POINT('Ctrl Pts',(3.47217189224653,1.,-1.54266605398188));
#52291=CARTESIAN_POINT('Ctrl Pts',(3.47868272898751,1.,-1.54678009290276));
#52292=CARTESIAN_POINT('Ctrl Pts',(3.48485155928567,1.,-1.55084702970452));
#52293=CARTESIAN_POINT('Ctrl Pts',(3.4907646087742,1.,-1.55489595901116));
#52294=CARTESIAN_POINT('Ctrl Pts',(3.49655185179655,1.,-1.55897703097874));
#52295=CARTESIAN_POINT('Ctrl Pts',(3.50234321621578,1.,-1.56314187758675));
#52296=CARTESIAN_POINT('Ctrl Pts',(3.50821771695363,1.,-1.56742097575012));
#52297=CARTESIAN_POINT('Ctrl Pts',(3.51418598431665,1.,-1.57181569799743));
#52298=CARTESIAN_POINT('Ctrl Pts',(3.52021847865912,1.,-1.57631049988158));
#52299=CARTESIAN_POINT('Ctrl Pts',(3.52626275334881,1.,-1.58088027227848));
#52300=CARTESIAN_POINT('Ctrl Pts',(3.5322637814708,1.,-1.58549906268088));
#52301=CARTESIAN_POINT('Ctrl Pts',(3.53818616861077,1.,-1.59014958368739));
#52302=CARTESIAN_POINT('Ctrl Pts',(3.54402458182337,1.,-1.59482766949766));
#52303=CARTESIAN_POINT('Ctrl Pts',(3.54979148634454,1.,-1.59953698113457));
#52304=CARTESIAN_POINT('Ctrl Pts',(3.55550985096129,1.,-1.60428584699853));
#52305=CARTESIAN_POINT('Ctrl Pts',(3.5612043248298,1.,-1.60908344685457));
#52306=CARTESIAN_POINT('Ctrl Pts',(3.56689200468387,1.,-1.61393581747514));
#52307=CARTESIAN_POINT('Ctrl Pts',(3.57257679609806,1.,-1.61884340915404));
#52308=CARTESIAN_POINT('Ctrl Pts',(3.5782545595439,1.,-1.62380329464844));
#52309=CARTESIAN_POINT('Ctrl Pts',(3.58391625774343,1.,-1.62881051550745));
#52310=CARTESIAN_POINT('Ctrl Pts',(3.58955176627879,1.,-1.6338597145126));
#52311=CARTESIAN_POINT('Ctrl Pts',(3.59515368334893,1.,-1.63894676675352));
#52312=CARTESIAN_POINT('Ctrl Pts',(3.60072028513845,1.,-1.64407004385582));
#52313=CARTESIAN_POINT('Ctrl Pts',(3.60625346556992,1.,-1.64922952425832));
#52314=CARTESIAN_POINT('Ctrl Pts',(3.61175734965127,1.,-1.65442619244325));
#52315=CARTESIAN_POINT('Ctrl Pts',(3.61723666482456,1.,-1.65966133399186));
#52316=CARTESIAN_POINT('Ctrl Pts',(3.62269517989109,1.,-1.66493585923855));
#52317=CARTESIAN_POINT('Ctrl Pts',(3.62813422105271,1.,-1.67024966008045));
#52318=CARTESIAN_POINT('Ctrl Pts',(3.63355343201232,1.,-1.67560193613156));
#52319=CARTESIAN_POINT('Ctrl Pts',(3.63895140887462,1.,-1.68099146651586));
#52320=CARTESIAN_POINT('Ctrl Pts',(3.64432638915203,1.,-1.68641690471457));
#52321=CARTESIAN_POINT('Ctrl Pts',(3.64967689827371,1.,-1.69187705481689));
#52322=CARTESIAN_POINT('Ctrl Pts',(3.65500246526749,1.,-1.69737117722534));
#52323=CARTESIAN_POINT('Ctrl Pts',(3.66030338774847,1.,-1.70289888566873));
#52324=CARTESIAN_POINT('Ctrl Pts',(3.66558043198876,1.,-1.70846001610956));
#52325=CARTESIAN_POINT('Ctrl Pts',(3.67083454901611,1.,-1.71405450210384));
#52326=CARTESIAN_POINT('Ctrl Pts',(3.67606660374709,1.,-1.71968225581808));
#52327=CARTESIAN_POINT('Ctrl Pts',(3.68127704936579,1.,-1.72534302437056));
#52328=CARTESIAN_POINT('Ctrl Pts',(3.68646597019332,1.,-1.73103640956717));
#52329=CARTESIAN_POINT('Ctrl Pts',(3.69163322648036,1.,-1.73676193254557));
#52330=CARTESIAN_POINT('Ctrl Pts',(3.69677856910517,1.,-1.74251908492617));
#52331=CARTESIAN_POINT('Ctrl Pts',(3.7019017567335,1.,-1.74830738046057));
#52332=CARTESIAN_POINT('Ctrl Pts',(3.70700269736659,1.,-1.75412641804042));
#52333=CARTESIAN_POINT('Ctrl Pts',(3.71208146346136,1.,-1.75997588498865));
#52334=CARTESIAN_POINT('Ctrl Pts',(3.71713822377359,1.,-1.76585552124394));
#52335=CARTESIAN_POINT('Ctrl Pts',(3.72217319911254,1.,-1.77176509401761));
#52336=CARTESIAN_POINT('Ctrl Pts',(3.72718661205609,1.,-1.77770437039658));
#52337=CARTESIAN_POINT('Ctrl Pts',(3.7321786309547,1.,-1.78367308442901));
#52338=CARTESIAN_POINT('Ctrl Pts',(3.73714934730681,1.,-1.78967092823491));
#52339=CARTESIAN_POINT('Ctrl Pts',(3.74209880352445,1.,-1.79569757859422));
#52340=CARTESIAN_POINT('Ctrl Pts',(3.74702700875467,1.,-1.8017527148577));
#52341=CARTESIAN_POINT('Ctrl Pts',(3.75193395887977,1.,-1.80783603939617));
#52342=CARTESIAN_POINT('Ctrl Pts',(3.75681965683071,1.,-1.8139472983358));
#52343=CARTESIAN_POINT('Ctrl Pts',(3.76168412707948,1.,-1.82008629694091));
#52344=CARTESIAN_POINT('Ctrl Pts',(3.76652740353775,1.,-1.82625289220915));
#52345=CARTESIAN_POINT('Ctrl Pts',(3.77038509817999,1.,-1.83120816955646));
#52346=CARTESIAN_POINT('Ctrl Pts',(3.77326886064398,1.,-1.83493697934534));
#52347=CARTESIAN_POINT('Ctrl Pts',(3.77518714457833,1.,-1.83742834010626));
#52348=CARTESIAN_POINT('Ctrl Pts',(3.77614523045147,1.,-1.83867539237861));
#52349=CARTESIAN_POINT('Origin',(3.77614523045147,0.,-1.83867539237861));
#52350=CARTESIAN_POINT('',(3.70708211654725,1.,-1.97421938526992));
#52351=CARTESIAN_POINT('Origin',(0.,0.,0.));
#52352=CARTESIAN_POINT('',(3.49844575334386,1.,-1.35032489087269));
#52353=CARTESIAN_POINT('Origin',(0.,1.,0.));
#52354=CARTESIAN_POINT('Ctrl Pts',(3.49844575334386,1.,-1.35032489087269));
#52355=CARTESIAN_POINT('Ctrl Pts',(3.49844575334386,0.666666666666667,-1.35032489087269));
#52356=CARTESIAN_POINT('Ctrl Pts',(3.49844575334386,0.333333333333333,-1.35032489087269));
#52357=CARTESIAN_POINT('Ctrl Pts',(3.49844575334386,-0.333333333333333,
-1.35032489087269));
#52358=CARTESIAN_POINT('Ctrl Pts',(3.49844575334386,-0.666666666666667,
-1.35032489087269));
#52359=CARTESIAN_POINT('Ctrl Pts',(3.49844575334386,-1.,-1.35032489087269));
#52360=CARTESIAN_POINT('Ctrl Pts',(3.97027773754922,-1.,-1.36999806084572));
#52361=CARTESIAN_POINT('Ctrl Pts',(3.97027773754922,1.,-1.36999806084572));
#52362=CARTESIAN_POINT('Ctrl Pts',(3.9687184694173,-1.,-1.37020239094758));
#52363=CARTESIAN_POINT('Ctrl Pts',(3.9687184694173,1.,-1.37020239094758));
#52364=CARTESIAN_POINT('Ctrl Pts',(3.96560037975788,-1.,-1.37060761746027));
#52365=CARTESIAN_POINT('Ctrl Pts',(3.96560037975788,1.,-1.37060761746027));
#52366=CARTESIAN_POINT('Ctrl Pts',(3.96092458508407,-1.,-1.37120515615663));
#52367=CARTESIAN_POINT('Ctrl Pts',(3.96092458508407,1.,-1.37120515615663));
#52368=CARTESIAN_POINT('Ctrl Pts',(3.95469287283105,-1.,-1.37198126433139));
#52369=CARTESIAN_POINT('Ctrl Pts',(3.95469287283105,1.,-1.37198126433139));
#52370=CARTESIAN_POINT('Ctrl Pts',(3.94690771786926,-1.,-1.37291699203423));
#52371=CARTESIAN_POINT('Ctrl Pts',(3.94690771786926,1.,-1.37291699203423));
#52372=CARTESIAN_POINT('Ctrl Pts',(3.93912709041791,-1.,-1.37381821967499));
#52373=CARTESIAN_POINT('Ctrl Pts',(3.93912709041791,1.,-1.37381821967499));
#52374=CARTESIAN_POINT('Ctrl Pts',(3.93135106761941,-1.,-1.37468482215784));
#52375=CARTESIAN_POINT('Ctrl Pts',(3.93135106761941,1.,-1.37468482215784));
#52376=CARTESIAN_POINT('Ctrl Pts',(3.92357976987132,-1.,-1.37551664448057));
#52377=CARTESIAN_POINT('Ctrl Pts',(3.92357976987132,1.,-1.37551664448057));
#52378=CARTESIAN_POINT('Ctrl Pts',(3.91581337461825,-1.,-1.37631350505516));
#52379=CARTESIAN_POINT('Ctrl Pts',(3.91581337461825,1.,-1.37631350505516));
#52380=CARTESIAN_POINT('Ctrl Pts',(3.90805209522729,-1.,-1.3770751963376));
#52381=CARTESIAN_POINT('Ctrl Pts',(3.90805209522729,1.,-1.3770751963376));
#52382=CARTESIAN_POINT('Ctrl Pts',(3.90029615196255,-1.,-1.3778014851263));
#52383=CARTESIAN_POINT('Ctrl Pts',(3.90029615196255,1.,-1.3778014851263));
#52384=CARTESIAN_POINT('Ctrl Pts',(3.89254574338385,-1.,-1.37849211287981));
#52385=CARTESIAN_POINT('Ctrl Pts',(3.89254574338385,1.,-1.37849211287981));
#52386=CARTESIAN_POINT('Ctrl Pts',(3.88480102249461,-1.,-1.37914679719446));
#52387=CARTESIAN_POINT('Ctrl Pts',(3.88480102249461,1.,-1.37914679719446));
#52388=CARTESIAN_POINT('Ctrl Pts',(3.87706205830865,-1.,-1.37976523097187));
#52389=CARTESIAN_POINT('Ctrl Pts',(3.87706205830865,1.,-1.37976523097187));
#52390=CARTESIAN_POINT('Ctrl Pts',(3.86932885813403,-1.,-1.38034709213129));
#52391=CARTESIAN_POINT('Ctrl Pts',(3.86932885813403,1.,-1.38034709213129));
#52392=CARTESIAN_POINT('Ctrl Pts',(3.86160143044187,-1.,-1.38089205993068));
#52393=CARTESIAN_POINT('Ctrl Pts',(3.86160143044187,1.,-1.38089205993068));
#52394=CARTESIAN_POINT('Ctrl Pts',(3.85387983979557,-1.,-1.38139983115075));
#52395=CARTESIAN_POINT('Ctrl Pts',(3.85387983979557,1.,-1.38139983115075));
#52396=CARTESIAN_POINT('Ctrl Pts',(3.84616425605705,-1.,-1.38187013346089));
#52397=CARTESIAN_POINT('Ctrl Pts',(3.84616425605705,1.,-1.38187013346089));
#52398=CARTESIAN_POINT('Ctrl Pts',(3.83845502790609,-1.,-1.38230274828774));
#52399=CARTESIAN_POINT('Ctrl Pts',(3.83845502790609,1.,-1.38230274828774));
#52400=CARTESIAN_POINT('Ctrl Pts',(3.83075266982138,-1.,-1.38269750245086));
#52401=CARTESIAN_POINT('Ctrl Pts',(3.83075266982138,1.,-1.38269750245086));
#52402=CARTESIAN_POINT('Ctrl Pts',(3.82305771743715,-1.,-1.38305421262724));
#52403=CARTESIAN_POINT('Ctrl Pts',(3.82305771743715,1.,-1.38305421262724));
#52404=CARTESIAN_POINT('Ctrl Pts',(3.81537060817765,-1.,-1.38337263902766));
#52405=CARTESIAN_POINT('Ctrl Pts',(3.81537060817765,1.,-1.38337263902766));
#52406=CARTESIAN_POINT('Ctrl Pts',(3.80769156398429,-1.,-1.38365244046226));
#52407=CARTESIAN_POINT('Ctrl Pts',(3.80769156398429,1.,-1.38365244046226));
#52408=CARTESIAN_POINT('Ctrl Pts',(3.80002044322169,-1.,-1.38389311766701));
#52409=CARTESIAN_POINT('Ctrl Pts',(3.80002044322169,1.,-1.38389311766701));
#52410=CARTESIAN_POINT('Ctrl Pts',(3.79235669640907,-1.,-1.38409399694589));
#52411=CARTESIAN_POINT('Ctrl Pts',(3.79235669640907,1.,-1.38409399694589));
#52412=CARTESIAN_POINT('Ctrl Pts',(3.78469969805134,-1.,-1.38425435883773));
#52413=CARTESIAN_POINT('Ctrl Pts',(3.78469969805134,1.,-1.38425435883773));
#52414=CARTESIAN_POINT('Ctrl Pts',(3.77704902230441,-1.,-1.38437354551435));
#52415=CARTESIAN_POINT('Ctrl Pts',(3.77704902230441,1.,-1.38437354551435));
#52416=CARTESIAN_POINT('Ctrl Pts',(3.76940473185775,-1.,-1.38445107339517));
#52417=CARTESIAN_POINT('Ctrl Pts',(3.76940473185775,1.,-1.38445107339517));
#52418=CARTESIAN_POINT('Ctrl Pts',(3.76176768271347,-1.,-1.38448675253343));
#52419=CARTESIAN_POINT('Ctrl Pts',(3.76176768271347,1.,-1.38448675253343));
#52420=CARTESIAN_POINT('Ctrl Pts',(3.75413976318727,-1.,-1.38448077997155));
#52421=CARTESIAN_POINT('Ctrl Pts',(3.75413976318727,1.,-1.38448077997155));
#52422=CARTESIAN_POINT('Ctrl Pts',(3.7465231716786,-1.,-1.38443344984389));
#52423=CARTESIAN_POINT('Ctrl Pts',(3.7465231716786,1.,-1.38443344984389));
#52424=CARTESIAN_POINT('Ctrl Pts',(3.73891976418099,-1.,-1.38434489156456));
#52425=CARTESIAN_POINT('Ctrl Pts',(3.73891976418099,1.,-1.38434489156456));
#52426=CARTESIAN_POINT('Ctrl Pts',(3.73133035859283,-1.,-1.38421479111531));
#52427=CARTESIAN_POINT('Ctrl Pts',(3.73133035859283,1.,-1.38421479111531));
#52428=CARTESIAN_POINT('Ctrl Pts',(3.72375409358805,-1.,-1.3840421342895));
#52429=CARTESIAN_POINT('Ctrl Pts',(3.72375409358805,1.,-1.3840421342895));
#52430=CARTESIAN_POINT('Ctrl Pts',(3.7161876605181,-1.,-1.38382489984585));
#52431=CARTESIAN_POINT('Ctrl Pts',(3.7161876605181,1.,-1.38382489984585));
#52432=CARTESIAN_POINT('Ctrl Pts',(3.70862680753343,-1.,-1.38356065402122));
#52433=CARTESIAN_POINT('Ctrl Pts',(3.70862680753343,1.,-1.38356065402122));
#52434=CARTESIAN_POINT('Ctrl Pts',(3.70106792167894,-1.,-1.38324717612862));
#52435=CARTESIAN_POINT('Ctrl Pts',(3.70106792167894,1.,-1.38324717612862));
#52436=CARTESIAN_POINT('Ctrl Pts',(3.69350967899523,-1.,-1.38288311171649));
#52437=CARTESIAN_POINT('Ctrl Pts',(3.69350967899523,1.,-1.38288311171649));
#52438=CARTESIAN_POINT('Ctrl Pts',(3.68595444983844,-1.,-1.38246852827185));
#52439=CARTESIAN_POINT('Ctrl Pts',(3.68595444983844,1.,-1.38246852827185));
#52440=CARTESIAN_POINT('Ctrl Pts',(3.6784103848243,-1.,-1.38200574290626));
#52441=CARTESIAN_POINT('Ctrl Pts',(3.6784103848243,1.,-1.38200574290626));
#52442=CARTESIAN_POINT('Ctrl Pts',(3.67088843112282,-1.,-1.38149812653876));
#52443=CARTESIAN_POINT('Ctrl Pts',(3.67088843112282,1.,-1.38149812653876));
#52444=CARTESIAN_POINT('Ctrl Pts',(3.66339848520874,-1.,-1.38094856333558));
#52445=CARTESIAN_POINT('Ctrl Pts',(3.66339848520874,1.,-1.38094856333558));
#52446=CARTESIAN_POINT('Ctrl Pts',(3.65594554404396,-1.,-1.38035791051215));
#52447=CARTESIAN_POINT('Ctrl Pts',(3.65594554404396,1.,-1.38035791051215));
#52448=CARTESIAN_POINT('Ctrl Pts',(3.64852652756444,-1.,-1.37972372481598));
#52449=CARTESIAN_POINT('Ctrl Pts',(3.64852652756444,1.,-1.37972372481598));
#52450=CARTESIAN_POINT('Ctrl Pts',(3.64112507791112,-1.,-1.37903818567347));
#52451=CARTESIAN_POINT('Ctrl Pts',(3.64112507791112,1.,-1.37903818567347));
#52452=CARTESIAN_POINT('Ctrl Pts',(3.63371727442448,-1.,-1.37829035457325));
#52453=CARTESIAN_POINT('Ctrl Pts',(3.63371727442448,1.,-1.37829035457325));
#52454=CARTESIAN_POINT('Ctrl Pts',(3.62628098665112,-1.,-1.37746987919868));
#52455=CARTESIAN_POINT('Ctrl Pts',(3.62628098665112,1.,-1.37746987919868));
#52456=CARTESIAN_POINT('Ctrl Pts',(3.61880481160408,-1.,-1.37657053403102));
#52457=CARTESIAN_POINT('Ctrl Pts',(3.61880481160408,1.,-1.37657053403102));
#52458=CARTESIAN_POINT('Ctrl Pts',(3.61129546591082,-1.,-1.37559314436641));
#52459=CARTESIAN_POINT('Ctrl Pts',(3.61129546591082,1.,-1.37559314436641));
#52460=CARTESIAN_POINT('Ctrl Pts',(3.60379020124038,-1.,-1.37455051379642));
#52461=CARTESIAN_POINT('Ctrl Pts',(3.60379020124038,1.,-1.37455051379642));
#52462=CARTESIAN_POINT('Ctrl Pts',(3.59634627869117,-1.,-1.37346320103184));
#52463=CARTESIAN_POINT('Ctrl Pts',(3.59634627869117,1.,-1.37346320103184));
#52464=CARTESIAN_POINT('Ctrl Pts',(3.5890185384643,-1.,-1.37235053661));
#52465=CARTESIAN_POINT('Ctrl Pts',(3.5890185384643,1.,-1.37235053661));
#52466=CARTESIAN_POINT('Ctrl Pts',(3.58183885982745,-1.,-1.37122241663073));
#52467=CARTESIAN_POINT('Ctrl Pts',(3.58183885982745,1.,-1.37122241663073));
#52468=CARTESIAN_POINT('Ctrl Pts',(3.57479875549453,-1.,-1.37007229485646));
#52469=CARTESIAN_POINT('Ctrl Pts',(3.57479875549453,1.,-1.37007229485646));
#52470=CARTESIAN_POINT('Ctrl Pts',(3.56782080304554,-1.,-1.36886584973349));
#52471=CARTESIAN_POINT('Ctrl Pts',(3.56782080304554,1.,-1.36886584973349));
#52472=CARTESIAN_POINT('Ctrl Pts',(3.56077662028492,-1.,-1.36754771771174));
#52473=CARTESIAN_POINT('Ctrl Pts',(3.56077662028492,1.,-1.36754771771174));
#52474=CARTESIAN_POINT('Ctrl Pts',(3.55353883995793,-1.,-1.36606145456711));
#52475=CARTESIAN_POINT('Ctrl Pts',(3.55353883995793,1.,-1.36606145456711));
#52476=CARTESIAN_POINT('Ctrl Pts',(3.54602591832893,-1.,-1.36436666257568));
#52477=CARTESIAN_POINT('Ctrl Pts',(3.54602591832893,1.,-1.36436666257568));
#52478=CARTESIAN_POINT('Ctrl Pts',(3.53824396425032,-1.,-1.36245507339334));
#52479=CARTESIAN_POINT('Ctrl Pts',(3.53824396425032,1.,-1.36245507339334));
#52480=CARTESIAN_POINT('Ctrl Pts',(3.53034464961849,-1.,-1.36037259643827));
#52481=CARTESIAN_POINT('Ctrl Pts',(3.53034464961849,1.,-1.36037259643827));
#52482=CARTESIAN_POINT('Ctrl Pts',(3.52261776117121,-1.,-1.35821701528975));
#52483=CARTESIAN_POINT('Ctrl Pts',(3.52261776117121,1.,-1.35821701528975));
#52484=CARTESIAN_POINT('Ctrl Pts',(3.51542230699919,-1.,-1.35611275237288));
#52485=CARTESIAN_POINT('Ctrl Pts',(3.51542230699919,1.,-1.35611275237288));
#52486=CARTESIAN_POINT('Ctrl Pts',(3.50913227060177,-1.,-1.35419113576022));
#52487=CARTESIAN_POINT('Ctrl Pts',(3.50913227060177,1.,-1.35419113576022));
#52488=CARTESIAN_POINT('Ctrl Pts',(3.50408168106113,-1.,-1.3525703284343));
#52489=CARTESIAN_POINT('Ctrl Pts',(3.50408168106113,1.,-1.3525703284343));
#52490=CARTESIAN_POINT('Ctrl Pts',(3.50049707063673,-1.,-1.35133076331065));
#52491=CARTESIAN_POINT('Ctrl Pts',(3.50049707063673,1.,-1.35133076331065));
#52492=CARTESIAN_POINT('Ctrl Pts',(3.49888720256612,-1.,-1.35067437417289));
#52493=CARTESIAN_POINT('Ctrl Pts',(3.49888720256612,1.,-1.35067437417289));
#52494=CARTESIAN_POINT('Ctrl Pts',(3.49840357193384,-1.,-1.35037650302887));
#52495=CARTESIAN_POINT('Ctrl Pts',(3.49840357193384,1.,-1.35037650302887));
#52496=CARTESIAN_POINT('Ctrl Pts',(3.49840260053616,-1.,-1.35026426118352));
#52497=CARTESIAN_POINT('Ctrl Pts',(3.49840260053616,1.,-1.35026426118352));
#52498=CARTESIAN_POINT('Ctrl Pts',(3.49848248301936,-1.,-1.35022972712301));
#52499=CARTESIAN_POINT('Ctrl Pts',(3.49848248301936,1.,-1.35022972712301));
#52500=CARTESIAN_POINT('',(3.97027773754922,1.,-1.36999806084572));
#52501=CARTESIAN_POINT('Ctrl Pts',(3.97027773754922,1.,-1.36999806084572));
#52502=CARTESIAN_POINT('Ctrl Pts',(3.9687184694173,1.,-1.37020239094758));
#52503=CARTESIAN_POINT('Ctrl Pts',(3.96560037975788,1.,-1.37060761746027));
#52504=CARTESIAN_POINT('Ctrl Pts',(3.96092458508407,1.,-1.37120515615663));
#52505=CARTESIAN_POINT('Ctrl Pts',(3.95469287283105,1.,-1.37198126433139));
#52506=CARTESIAN_POINT('Ctrl Pts',(3.94690771786926,1.,-1.37291699203423));
#52507=CARTESIAN_POINT('Ctrl Pts',(3.93912709041791,1.,-1.37381821967499));
#52508=CARTESIAN_POINT('Ctrl Pts',(3.93135106761941,1.,-1.37468482215784));
#52509=CARTESIAN_POINT('Ctrl Pts',(3.92357976987132,1.,-1.37551664448057));
#52510=CARTESIAN_POINT('Ctrl Pts',(3.91581337461825,1.,-1.37631350505516));
#52511=CARTESIAN_POINT('Ctrl Pts',(3.90805209522729,1.,-1.3770751963376));
#52512=CARTESIAN_POINT('Ctrl Pts',(3.90029615196255,1.,-1.3778014851263));
#52513=CARTESIAN_POINT('Ctrl Pts',(3.89254574338385,1.,-1.37849211287981));
#52514=CARTESIAN_POINT('Ctrl Pts',(3.88480102249461,1.,-1.37914679719446));
#52515=CARTESIAN_POINT('Ctrl Pts',(3.87706205830865,1.,-1.37976523097187));
#52516=CARTESIAN_POINT('Ctrl Pts',(3.86932885813403,1.,-1.38034709213129));
#52517=CARTESIAN_POINT('Ctrl Pts',(3.86160143044187,1.,-1.38089205993068));
#52518=CARTESIAN_POINT('Ctrl Pts',(3.85387983979557,1.,-1.38139983115075));
#52519=CARTESIAN_POINT('Ctrl Pts',(3.84616425605705,1.,-1.38187013346089));
#52520=CARTESIAN_POINT('Ctrl Pts',(3.83845502790609,1.,-1.38230274828774));
#52521=CARTESIAN_POINT('Ctrl Pts',(3.83075266982138,1.,-1.38269750245086));
#52522=CARTESIAN_POINT('Ctrl Pts',(3.82305771743715,1.,-1.38305421262724));
#52523=CARTESIAN_POINT('Ctrl Pts',(3.81537060817765,1.,-1.38337263902766));
#52524=CARTESIAN_POINT('Ctrl Pts',(3.80769156398429,1.,-1.38365244046226));
#52525=CARTESIAN_POINT('Ctrl Pts',(3.80002044322169,1.,-1.38389311766701));
#52526=CARTESIAN_POINT('Ctrl Pts',(3.79235669640907,1.,-1.38409399694589));
#52527=CARTESIAN_POINT('Ctrl Pts',(3.78469969805134,1.,-1.38425435883773));
#52528=CARTESIAN_POINT('Ctrl Pts',(3.77704902230441,1.,-1.38437354551435));
#52529=CARTESIAN_POINT('Ctrl Pts',(3.76940473185775,1.,-1.38445107339517));
#52530=CARTESIAN_POINT('Ctrl Pts',(3.76176768271347,1.,-1.38448675253343));
#52531=CARTESIAN_POINT('Ctrl Pts',(3.75413976318727,1.,-1.38448077997155));
#52532=CARTESIAN_POINT('Ctrl Pts',(3.7465231716786,1.,-1.38443344984389));
#52533=CARTESIAN_POINT('Ctrl Pts',(3.73891976418099,1.,-1.38434489156456));
#52534=CARTESIAN_POINT('Ctrl Pts',(3.73133035859283,1.,-1.38421479111531));
#52535=CARTESIAN_POINT('Ctrl Pts',(3.72375409358805,1.,-1.3840421342895));
#52536=CARTESIAN_POINT('Ctrl Pts',(3.7161876605181,1.,-1.38382489984585));
#52537=CARTESIAN_POINT('Ctrl Pts',(3.70862680753343,1.,-1.38356065402122));
#52538=CARTESIAN_POINT('Ctrl Pts',(3.70106792167894,1.,-1.38324717612862));
#52539=CARTESIAN_POINT('Ctrl Pts',(3.69350967899523,1.,-1.38288311171649));
#52540=CARTESIAN_POINT('Ctrl Pts',(3.68595444983844,1.,-1.38246852827185));
#52541=CARTESIAN_POINT('Ctrl Pts',(3.6784103848243,1.,-1.38200574290626));
#52542=CARTESIAN_POINT('Ctrl Pts',(3.67088843112282,1.,-1.38149812653876));
#52543=CARTESIAN_POINT('Ctrl Pts',(3.66339848520874,1.,-1.38094856333558));
#52544=CARTESIAN_POINT('Ctrl Pts',(3.65594554404396,1.,-1.38035791051215));
#52545=CARTESIAN_POINT('Ctrl Pts',(3.64852652756444,1.,-1.37972372481598));
#52546=CARTESIAN_POINT('Ctrl Pts',(3.64112507791112,1.,-1.37903818567347));
#52547=CARTESIAN_POINT('Ctrl Pts',(3.63371727442448,1.,-1.37829035457325));
#52548=CARTESIAN_POINT('Ctrl Pts',(3.62628098665112,1.,-1.37746987919868));
#52549=CARTESIAN_POINT('Ctrl Pts',(3.61880481160408,1.,-1.37657053403102));
#52550=CARTESIAN_POINT('Ctrl Pts',(3.61129546591082,1.,-1.37559314436641));
#52551=CARTESIAN_POINT('Ctrl Pts',(3.60379020124038,1.,-1.37455051379642));
#52552=CARTESIAN_POINT('Ctrl Pts',(3.59634627869117,1.,-1.37346320103184));
#52553=CARTESIAN_POINT('Ctrl Pts',(3.5890185384643,1.,-1.37235053661));
#52554=CARTESIAN_POINT('Ctrl Pts',(3.58183885982745,1.,-1.37122241663073));
#52555=CARTESIAN_POINT('Ctrl Pts',(3.57479875549453,1.,-1.37007229485646));
#52556=CARTESIAN_POINT('Ctrl Pts',(3.56782080304554,1.,-1.36886584973349));
#52557=CARTESIAN_POINT('Ctrl Pts',(3.56077662028492,1.,-1.36754771771174));
#52558=CARTESIAN_POINT('Ctrl Pts',(3.55353883995793,1.,-1.36606145456711));
#52559=CARTESIAN_POINT('Ctrl Pts',(3.54602591832893,1.,-1.36436666257568));
#52560=CARTESIAN_POINT('Ctrl Pts',(3.53824396425032,1.,-1.36245507339334));
#52561=CARTESIAN_POINT('Ctrl Pts',(3.53034464961849,1.,-1.36037259643827));
#52562=CARTESIAN_POINT('Ctrl Pts',(3.52261776117121,1.,-1.35821701528975));
#52563=CARTESIAN_POINT('Ctrl Pts',(3.51542230699919,1.,-1.35611275237288));
#52564=CARTESIAN_POINT('Ctrl Pts',(3.50913227060177,1.,-1.35419113576022));
#52565=CARTESIAN_POINT('Ctrl Pts',(3.50408168106113,1.,-1.3525703284343));
#52566=CARTESIAN_POINT('Ctrl Pts',(3.5007660381658,1.,-1.35142377279535));
#52567=CARTESIAN_POINT('Ctrl Pts',(3.49920025459856,1.,-1.35080045218652));
#52568=CARTESIAN_POINT('Ctrl Pts',(3.49861894124915,1.,-1.35049736560633));
#52569=CARTESIAN_POINT('Ctrl Pts',(3.49847119623841,1.,-1.35036670893102));
#52570=CARTESIAN_POINT('Ctrl Pts',(3.49844575334386,1.,-1.35032489087269));
#52571=CARTESIAN_POINT('',(3.97027773754922,0.,-1.36999806084572));
#52572=CARTESIAN_POINT('Ctrl Pts',(3.62397690409552,-1.,-0.963997613369571));
#52573=CARTESIAN_POINT('Ctrl Pts',(3.62397690409552,1.,-0.963997613369571));
#52574=CARTESIAN_POINT('Ctrl Pts',(3.62393257642191,-1.,-0.963922720982576));
#52575=CARTESIAN_POINT('Ctrl Pts',(3.62393257642191,1.,-0.963922720982576));
#52576=CARTESIAN_POINT('Ctrl Pts',(3.62399933640277,-1.,-0.963832486396056));
#52577=CARTESIAN_POINT('Ctrl Pts',(3.62399933640277,1.,-0.963832486396056));
#52578=CARTESIAN_POINT('Ctrl Pts',(3.62456568607055,-1.,-0.963875774532103));
#52579=CARTESIAN_POINT('Ctrl Pts',(3.62456568607055,1.,-0.963875774532103));
#52580=CARTESIAN_POINT('Ctrl Pts',(3.62625391255277,-1.,-0.964291001274619));
#52581=CARTESIAN_POINT('Ctrl Pts',(3.62625391255277,1.,-0.964291001274619));
#52582=CARTESIAN_POINT('Ctrl Pts',(3.62988252139998,-1.,-0.965395153165716));
#52583=CARTESIAN_POINT('Ctrl Pts',(3.62988252139998,1.,-0.965395153165716));
#52584=CARTESIAN_POINT('Ctrl Pts',(3.6349212208096,-1.,-0.967052554540878));
#52585=CARTESIAN_POINT('Ctrl Pts',(3.6349212208096,1.,-0.967052554540878));
#52586=CARTESIAN_POINT('Ctrl Pts',(3.64113946505393,-1.,-0.969195124674829));
#52587=CARTESIAN_POINT('Ctrl Pts',(3.64113946505393,1.,-0.969195124674829));
#52588=CARTESIAN_POINT('Ctrl Pts',(3.64819756447072,-1.,-0.971722122060278));
#52589=CARTESIAN_POINT('Ctrl Pts',(3.64819756447072,1.,-0.971722122060278));
#52590=CARTESIAN_POINT('Ctrl Pts',(3.6557157673487,-1.,-0.974519971354139));
#52591=CARTESIAN_POINT('Ctrl Pts',(3.6557157673487,1.,-0.974519971354139));
#52592=CARTESIAN_POINT('Ctrl Pts',(3.66333049637403,-1.,-0.977478312751416));
#52593=CARTESIAN_POINT('Ctrl Pts',(3.66333049637403,1.,-0.977478312751416));
#52594=CARTESIAN_POINT('Ctrl Pts',(3.67074983340444,-1.,-0.980505922458495));
#52595=CARTESIAN_POINT('Ctrl Pts',(3.67074983340444,1.,-0.980505922458495));
#52596=CARTESIAN_POINT('Ctrl Pts',(3.67782408841876,-1.,-0.983550791470865));
#52597=CARTESIAN_POINT('Ctrl Pts',(3.67782408841876,1.,-0.983550791470865));
#52598=CARTESIAN_POINT('Ctrl Pts',(3.6845531792623,-1.,-0.986602639864286));
#52599=CARTESIAN_POINT('Ctrl Pts',(3.6845531792623,1.,-0.986602639864286));
#52600=CARTESIAN_POINT('Ctrl Pts',(3.69102682138955,-1.,-0.989676715398859));
#52601=CARTESIAN_POINT('Ctrl Pts',(3.69102682138955,1.,-0.989676715398859));
#52602=CARTESIAN_POINT('Ctrl Pts',(3.69738123415696,-1.,-0.992802218332104));
#52603=CARTESIAN_POINT('Ctrl Pts',(3.69738123415696,1.,-0.992802218332104));
#52604=CARTESIAN_POINT('Ctrl Pts',(3.70375282282107,-1.,-0.996009819772432));
#52605=CARTESIAN_POINT('Ctrl Pts',(3.70375282282107,1.,-0.996009819772432));
#52606=CARTESIAN_POINT('Ctrl Pts',(3.7102243971387,-1.,-0.999317260756345));
#52607=CARTESIAN_POINT('Ctrl Pts',(3.7102243971387,1.,-0.999317260756345));
#52608=CARTESIAN_POINT('Ctrl Pts',(3.71680667125047,-1.,-1.00272423396802));
#52609=CARTESIAN_POINT('Ctrl Pts',(3.71680667125047,1.,-1.00272423396802));
#52610=CARTESIAN_POINT('Ctrl Pts',(3.72346803750544,-1.,-1.00622000735696));
#52611=CARTESIAN_POINT('Ctrl Pts',(3.72346803750544,1.,-1.00622000735696));
#52612=CARTESIAN_POINT('Ctrl Pts',(3.73015276704407,-1.,-1.00978798539491));
#52613=CARTESIAN_POINT('Ctrl Pts',(3.73015276704407,1.,-1.00978798539491));
#52614=CARTESIAN_POINT('Ctrl Pts',(3.73680245055747,-1.,-1.01341114319906));
#52615=CARTESIAN_POINT('Ctrl Pts',(3.73680245055747,1.,-1.01341114319906));
#52616=CARTESIAN_POINT('Ctrl Pts',(3.74337942504993,-1.,-1.01707794311088));
#52617=CARTESIAN_POINT('Ctrl Pts',(3.74337942504993,1.,-1.01707794311088));
#52618=CARTESIAN_POINT('Ctrl Pts',(3.74987777155873,-1.,-1.02078510487439));
#52619=CARTESIAN_POINT('Ctrl Pts',(3.74987777155873,1.,-1.02078510487439));
#52620=CARTESIAN_POINT('Ctrl Pts',(3.75631037456224,-1.,-1.02453429444668));
#52621=CARTESIAN_POINT('Ctrl Pts',(3.75631037456224,1.,-1.02453429444668));
#52622=CARTESIAN_POINT('Ctrl Pts',(3.76270122291245,-1.,-1.02833014458184));
#52623=CARTESIAN_POINT('Ctrl Pts',(3.76270122291245,1.,-1.02833014458184));
#52624=CARTESIAN_POINT('Ctrl Pts',(3.76907609832516,-1.,-1.03217786604919));
#52625=CARTESIAN_POINT('Ctrl Pts',(3.76907609832516,1.,-1.03217786604919));
#52626=CARTESIAN_POINT('Ctrl Pts',(3.77545283140427,-1.,-1.03608074678008));
#52627=CARTESIAN_POINT('Ctrl Pts',(3.77545283140427,1.,-1.03608074678008));
#52628=CARTESIAN_POINT('Ctrl Pts',(3.7818353500817,-1.,-1.04003862055798));
#52629=CARTESIAN_POINT('Ctrl Pts',(3.7818353500817,1.,-1.04003862055798));
#52630=CARTESIAN_POINT('Ctrl Pts',(3.78821910787179,-1.,-1.04404924374422));
#52631=CARTESIAN_POINT('Ctrl Pts',(3.78821910787179,1.,-1.04404924374422));
#52632=CARTESIAN_POINT('Ctrl Pts',(3.79459440308786,-1.,-1.04810913267639));
#52633=CARTESIAN_POINT('Ctrl Pts',(3.79459440308786,1.,-1.04810913267639));
#52634=CARTESIAN_POINT('Ctrl Pts',(3.80095039790681,-1.,-1.05221457990016));
#52635=CARTESIAN_POINT('Ctrl Pts',(3.80095039790681,1.,-1.05221457990016));
#52636=CARTESIAN_POINT('Ctrl Pts',(3.80727913637791,-1.,-1.05636266918644));
#52637=CARTESIAN_POINT('Ctrl Pts',(3.80727913637791,1.,-1.05636266918644));
#52638=CARTESIAN_POINT('Ctrl Pts',(3.8135786611749,-1.,-1.06055206187299));
#52639=CARTESIAN_POINT('Ctrl Pts',(3.8135786611749,1.,-1.06055206187299));
#52640=CARTESIAN_POINT('Ctrl Pts',(3.81985083953012,-1.,-1.0647824403893));
#52641=CARTESIAN_POINT('Ctrl Pts',(3.81985083953012,1.,-1.0647824403893));
#52642=CARTESIAN_POINT('Ctrl Pts',(3.82609989967276,-1.,-1.06905413180359));
#52643=CARTESIAN_POINT('Ctrl Pts',(3.82609989967276,1.,-1.06905413180359));
#52644=CARTESIAN_POINT('Ctrl Pts',(3.83233071195144,-1.,-1.07336766633459));
#52645=CARTESIAN_POINT('Ctrl Pts',(3.83233071195144,1.,-1.07336766633459));
#52646=CARTESIAN_POINT('Ctrl Pts',(3.83854714117491,-1.,-1.07772335353858));
#52647=CARTESIAN_POINT('Ctrl Pts',(3.83854714117491,1.,-1.07772335353858));
#52648=CARTESIAN_POINT('Ctrl Pts',(3.8447504803063,-1.,-1.08212087917991));
#52649=CARTESIAN_POINT('Ctrl Pts',(3.8447504803063,1.,-1.08212087917991));
#52650=CARTESIAN_POINT('Ctrl Pts',(3.85094025222713,-1.,-1.08655950846384));
#52651=CARTESIAN_POINT('Ctrl Pts',(3.85094025222713,1.,-1.08655950846384));
#52652=CARTESIAN_POINT('Ctrl Pts',(3.85711487933931,-1.,-1.09103825516294));
#52653=CARTESIAN_POINT('Ctrl Pts',(3.85711487933931,1.,-1.09103825516294));
#52654=CARTESIAN_POINT('Ctrl Pts',(3.86327241021247,-1.,-1.09555606505013));
#52655=CARTESIAN_POINT('Ctrl Pts',(3.86327241021247,1.,-1.09555606505013));
#52656=CARTESIAN_POINT('Ctrl Pts',(3.86941120134849,-1.,-1.10011198761195));
#52657=CARTESIAN_POINT('Ctrl Pts',(3.86941120134849,1.,-1.10011198761195));
#52658=CARTESIAN_POINT('Ctrl Pts',(3.87553067187514,-1.,-1.10470536603287));
#52659=CARTESIAN_POINT('Ctrl Pts',(3.87553067187514,1.,-1.10470536603287));
#52660=CARTESIAN_POINT('Ctrl Pts',(3.88163105531724,-1.,-1.10933577224008));
#52661=CARTESIAN_POINT('Ctrl Pts',(3.88163105531724,1.,-1.10933577224008));
#52662=CARTESIAN_POINT('Ctrl Pts',(3.88771308285171,-1.,-1.11400292434429));
#52663=CARTESIAN_POINT('Ctrl Pts',(3.88771308285171,1.,-1.11400292434429));
#52664=CARTESIAN_POINT('Ctrl Pts',(3.89377768340344,-1.,-1.11870660794603));
#52665=CARTESIAN_POINT('Ctrl Pts',(3.89377768340344,1.,-1.11870660794603));
#52666=CARTESIAN_POINT('Ctrl Pts',(3.89982569750025,-1.,-1.12344660099043));
#52667=CARTESIAN_POINT('Ctrl Pts',(3.89982569750025,1.,-1.12344660099043));
#52668=CARTESIAN_POINT('Ctrl Pts',(3.90585753318737,-1.,-1.12822258281553));
#52669=CARTESIAN_POINT('Ctrl Pts',(3.90585753318737,1.,-1.12822258281553));
#52670=CARTESIAN_POINT('Ctrl Pts',(3.91187321145649,-1.,-1.13303414693896));
#52671=CARTESIAN_POINT('Ctrl Pts',(3.91187321145649,1.,-1.13303414693896));
#52672=CARTESIAN_POINT('Ctrl Pts',(3.91787251936827,-1.,-1.13788084225554));
#52673=CARTESIAN_POINT('Ctrl Pts',(3.91787251936827,1.,-1.13788084225554));
#52674=CARTESIAN_POINT('Ctrl Pts',(3.92385513133997,-1.,-1.14276220561593));
#52675=CARTESIAN_POINT('Ctrl Pts',(3.92385513133997,1.,-1.14276220561593));
#52676=CARTESIAN_POINT('Ctrl Pts',(3.92982073294257,-1.,-1.14767779451124));
#52677=CARTESIAN_POINT('Ctrl Pts',(3.92982073294257,1.,-1.14767779451124));
#52678=CARTESIAN_POINT('Ctrl Pts',(3.9357691705628,-1.,-1.1526272271632));
#52679=CARTESIAN_POINT('Ctrl Pts',(3.9357691705628,1.,-1.1526272271632));
#52680=CARTESIAN_POINT('Ctrl Pts',(3.94170046685203,-1.,-1.15761018340956));
#52681=CARTESIAN_POINT('Ctrl Pts',(3.94170046685203,1.,-1.15761018340956));
#52682=CARTESIAN_POINT('Ctrl Pts',(3.94761474780583,-1.,-1.16262637999157));
#52683=CARTESIAN_POINT('Ctrl Pts',(3.94761474780583,1.,-1.16262637999157));
#52684=CARTESIAN_POINT('Ctrl Pts',(3.95351219509876,-1.,-1.16767555244438));
#52685=CARTESIAN_POINT('Ctrl Pts',(3.95351219509876,1.,-1.16767555244438));
#52686=CARTESIAN_POINT('Ctrl Pts',(3.95939299213276,-1.,-1.17275743590361));
#52687=CARTESIAN_POINT('Ctrl Pts',(3.95939299213276,1.,-1.17275743590361));
#52688=CARTESIAN_POINT('Ctrl Pts',(3.96525726358159,-1.,-1.17787174135592));
#52689=CARTESIAN_POINT('Ctrl Pts',(3.96525726358159,1.,-1.17787174135592));
#52690=CARTESIAN_POINT('Ctrl Pts',(3.97110505165415,-1.,-1.18301815039831));
#52691=CARTESIAN_POINT('Ctrl Pts',(3.97110505165415,1.,-1.18301815039831));
#52692=CARTESIAN_POINT('Ctrl Pts',(3.97693634767754,-1.,-1.18819633715539));
#52693=CARTESIAN_POINT('Ctrl Pts',(3.97693634767754,1.,-1.18819633715539));
#52694=CARTESIAN_POINT('Ctrl Pts',(3.98275111052561,-1.,-1.19340598349475));
#52695=CARTESIAN_POINT('Ctrl Pts',(3.98275111052561,1.,-1.19340598349475));
#52696=CARTESIAN_POINT('Ctrl Pts',(3.98854928957189,-1.,-1.19864679609566));
#52697=CARTESIAN_POINT('Ctrl Pts',(3.98854928957189,1.,-1.19864679609566));
#52698=CARTESIAN_POINT('Ctrl Pts',(3.99433084799666,-1.,-1.20391852375139));
#52699=CARTESIAN_POINT('Ctrl Pts',(3.99433084799666,1.,-1.20391852375139));
#52700=CARTESIAN_POINT('Ctrl Pts',(4.00009577950721,-1.,-1.20922097029551));
#52701=CARTESIAN_POINT('Ctrl Pts',(4.00009577950721,1.,-1.20922097029551));
#52702=CARTESIAN_POINT('Ctrl Pts',(4.00584409522722,-1.,-1.21455398918133));
#52703=CARTESIAN_POINT('Ctrl Pts',(4.00584409522722,1.,-1.21455398918133));
#52704=CARTESIAN_POINT('Ctrl Pts',(4.01042947140789,-1.,-1.21884478244403));
#52705=CARTESIAN_POINT('Ctrl Pts',(4.01042947140789,1.,-1.21884478244403));
#52706=CARTESIAN_POINT('Ctrl Pts',(4.01386104433519,-1.,-1.22207656455845));
#52707=CARTESIAN_POINT('Ctrl Pts',(4.01386104433519,1.,-1.22207656455845));
#52708=CARTESIAN_POINT('Ctrl Pts',(4.01614544569895,-1.,-1.22423716681317));
#52709=CARTESIAN_POINT('Ctrl Pts',(4.01614544569895,1.,-1.22423716681317));
#52710=CARTESIAN_POINT('Ctrl Pts',(4.01728681790024,-1.,-1.22531898815164));
#52711=CARTESIAN_POINT('Ctrl Pts',(4.01728681790024,1.,-1.22531898815164));
#52712=CARTESIAN_POINT('',(3.62400312501199,1.,-0.963899035118984));
#52713=CARTESIAN_POINT('Ctrl Pts',(3.62400312501199,-1.,-0.963899035118986));
#52714=CARTESIAN_POINT('Ctrl Pts',(3.62400312501199,-0.666666666666667,
-0.963899035118986));
#52715=CARTESIAN_POINT('Ctrl Pts',(3.62400312501199,-0.333333333333333,
-0.963899035118986));
#52716=CARTESIAN_POINT('Ctrl Pts',(3.62400312501199,0.333333333333333,-0.963899035118986));
#52717=CARTESIAN_POINT('Ctrl Pts',(3.62400312501199,0.666666666666667,-0.963899035118986));
#52718=CARTESIAN_POINT('Ctrl Pts',(3.62400312501199,1.,-0.963899035118986));
#52719=CARTESIAN_POINT('',(4.01728681790024,1.,-1.22531898815164));
#52720=CARTESIAN_POINT('',(4.01728681790024,0.,-1.22531898815164));
#52721=CARTESIAN_POINT('Ctrl Pts',(3.62400312501199,1.,-0.963899035118985));
#52722=CARTESIAN_POINT('Ctrl Pts',(3.62404828878374,1.,-0.963880158556713));
#52723=CARTESIAN_POINT('Ctrl Pts',(3.62424461507455,1.,-0.963861297423579));
#52724=CARTESIAN_POINT('Ctrl Pts',(3.62489305727516,1.,-0.96395778264259));
#52725=CARTESIAN_POINT('Ctrl Pts',(3.62652618145252,1.,-0.964373850166082));
#52726=CARTESIAN_POINT('Ctrl Pts',(3.62988252139998,1.,-0.965395153165716));
#52727=CARTESIAN_POINT('Ctrl Pts',(3.6349212208096,1.,-0.967052554540878));
#52728=CARTESIAN_POINT('Ctrl Pts',(3.64113946505393,1.,-0.969195124674829));
#52729=CARTESIAN_POINT('Ctrl Pts',(3.64819756447072,1.,-0.971722122060278));
#52730=CARTESIAN_POINT('Ctrl Pts',(3.6557157673487,1.,-0.974519971354139));
#52731=CARTESIAN_POINT('Ctrl Pts',(3.66333049637403,1.,-0.977478312751416));
#52732=CARTESIAN_POINT('Ctrl Pts',(3.67074983340444,1.,-0.980505922458495));
#52733=CARTESIAN_POINT('Ctrl Pts',(3.67782408841876,1.,-0.983550791470865));
#52734=CARTESIAN_POINT('Ctrl Pts',(3.6845531792623,1.,-0.986602639864286));
#52735=CARTESIAN_POINT('Ctrl Pts',(3.69102682138955,1.,-0.989676715398859));
#52736=CARTESIAN_POINT('Ctrl Pts',(3.69738123415696,1.,-0.992802218332104));
#52737=CARTESIAN_POINT('Ctrl Pts',(3.70375282282107,1.,-0.996009819772432));
#52738=CARTESIAN_POINT('Ctrl Pts',(3.7102243971387,1.,-0.999317260756345));
#52739=CARTESIAN_POINT('Ctrl Pts',(3.71680667125047,1.,-1.00272423396802));
#52740=CARTESIAN_POINT('Ctrl Pts',(3.72346803750544,1.,-1.00622000735696));
#52741=CARTESIAN_POINT('Ctrl Pts',(3.73015276704407,1.,-1.00978798539491));
#52742=CARTESIAN_POINT('Ctrl Pts',(3.73680245055747,1.,-1.01341114319906));
#52743=CARTESIAN_POINT('Ctrl Pts',(3.74337942504993,1.,-1.01707794311088));
#52744=CARTESIAN_POINT('Ctrl Pts',(3.74987777155873,1.,-1.02078510487439));
#52745=CARTESIAN_POINT('Ctrl Pts',(3.75631037456224,1.,-1.02453429444668));
#52746=CARTESIAN_POINT('Ctrl Pts',(3.76270122291245,1.,-1.02833014458184));
#52747=CARTESIAN_POINT('Ctrl Pts',(3.76907609832516,1.,-1.03217786604919));
#52748=CARTESIAN_POINT('Ctrl Pts',(3.77545283140427,1.,-1.03608074678008));
#52749=CARTESIAN_POINT('Ctrl Pts',(3.7818353500817,1.,-1.04003862055798));
#52750=CARTESIAN_POINT('Ctrl Pts',(3.78821910787179,1.,-1.04404924374422));
#52751=CARTESIAN_POINT('Ctrl Pts',(3.79459440308786,1.,-1.04810913267639));
#52752=CARTESIAN_POINT('Ctrl Pts',(3.80095039790681,1.,-1.05221457990016));
#52753=CARTESIAN_POINT('Ctrl Pts',(3.80727913637791,1.,-1.05636266918644));
#52754=CARTESIAN_POINT('Ctrl Pts',(3.8135786611749,1.,-1.06055206187299));
#52755=CARTESIAN_POINT('Ctrl Pts',(3.81985083953012,1.,-1.0647824403893));
#52756=CARTESIAN_POINT('Ctrl Pts',(3.82609989967276,1.,-1.06905413180359));
#52757=CARTESIAN_POINT('Ctrl Pts',(3.83233071195144,1.,-1.07336766633459));
#52758=CARTESIAN_POINT('Ctrl Pts',(3.83854714117491,1.,-1.07772335353858));
#52759=CARTESIAN_POINT('Ctrl Pts',(3.8447504803063,1.,-1.08212087917991));
#52760=CARTESIAN_POINT('Ctrl Pts',(3.85094025222713,1.,-1.08655950846384));
#52761=CARTESIAN_POINT('Ctrl Pts',(3.85711487933931,1.,-1.09103825516294));
#52762=CARTESIAN_POINT('Ctrl Pts',(3.86327241021247,1.,-1.09555606505013));
#52763=CARTESIAN_POINT('Ctrl Pts',(3.86941120134849,1.,-1.10011198761195));
#52764=CARTESIAN_POINT('Ctrl Pts',(3.87553067187514,1.,-1.10470536603287));
#52765=CARTESIAN_POINT('Ctrl Pts',(3.88163105531724,1.,-1.10933577224008));
#52766=CARTESIAN_POINT('Ctrl Pts',(3.88771308285171,1.,-1.11400292434429));
#52767=CARTESIAN_POINT('Ctrl Pts',(3.89377768340344,1.,-1.11870660794603));
#52768=CARTESIAN_POINT('Ctrl Pts',(3.89982569750025,1.,-1.12344660099043));
#52769=CARTESIAN_POINT('Ctrl Pts',(3.90585753318737,1.,-1.12822258281553));
#52770=CARTESIAN_POINT('Ctrl Pts',(3.91187321145649,1.,-1.13303414693896));
#52771=CARTESIAN_POINT('Ctrl Pts',(3.91787251936827,1.,-1.13788084225554));
#52772=CARTESIAN_POINT('Ctrl Pts',(3.92385513133997,1.,-1.14276220561593));
#52773=CARTESIAN_POINT('Ctrl Pts',(3.92982073294257,1.,-1.14767779451124));
#52774=CARTESIAN_POINT('Ctrl Pts',(3.9357691705628,1.,-1.1526272271632));
#52775=CARTESIAN_POINT('Ctrl Pts',(3.94170046685203,1.,-1.15761018340956));
#52776=CARTESIAN_POINT('Ctrl Pts',(3.94761474780583,1.,-1.16262637999157));
#52777=CARTESIAN_POINT('Ctrl Pts',(3.95351219509876,1.,-1.16767555244438));
#52778=CARTESIAN_POINT('Ctrl Pts',(3.95939299213276,1.,-1.17275743590361));
#52779=CARTESIAN_POINT('Ctrl Pts',(3.96525726358159,1.,-1.17787174135592));
#52780=CARTESIAN_POINT('Ctrl Pts',(3.97110505165415,1.,-1.18301815039831));
#52781=CARTESIAN_POINT('Ctrl Pts',(3.97693634767754,1.,-1.18819633715539));
#52782=CARTESIAN_POINT('Ctrl Pts',(3.98275111052561,1.,-1.19340598349475));
#52783=CARTESIAN_POINT('Ctrl Pts',(3.98854928957189,1.,-1.19864679609566));
#52784=CARTESIAN_POINT('Ctrl Pts',(3.99433084799666,1.,-1.20391852375139));
#52785=CARTESIAN_POINT('Ctrl Pts',(4.00009577950721,1.,-1.20922097029551));
#52786=CARTESIAN_POINT('Ctrl Pts',(4.00584409522722,1.,-1.21455398918133));
#52787=CARTESIAN_POINT('Ctrl Pts',(4.01042947140789,1.,-1.21884478244403));
#52788=CARTESIAN_POINT('Ctrl Pts',(4.01386104433519,1.,-1.22207656455845));
#52789=CARTESIAN_POINT('Ctrl Pts',(4.01614544569895,1.,-1.22423716681317));
#52790=CARTESIAN_POINT('Ctrl Pts',(4.01728681790024,1.,-1.22531898815164));
#52791=CARTESIAN_POINT('Origin',(4.01728681790024,0.,-1.22531898815164));
#52792=CARTESIAN_POINT('',(3.97027773754922,1.,-1.36999806084572));
#52793=CARTESIAN_POINT('Origin',(0.,0.,0.));
#52794=CARTESIAN_POINT('',(3.66661143271648,1.,-0.786422660833743));
#52795=CARTESIAN_POINT('Origin',(0.,1.,0.));
#52796=CARTESIAN_POINT('Ctrl Pts',(3.66661143271648,1.,-0.786422660833743));
#52797=CARTESIAN_POINT('Ctrl Pts',(3.66661143271648,0.666666666666667,-0.786422660833743));
#52798=CARTESIAN_POINT('Ctrl Pts',(3.66661143271648,0.333333333333333,-0.786422660833743));
#52799=CARTESIAN_POINT('Ctrl Pts',(3.66661143271648,-0.333333333333333,
-0.786422660833743));
#52800=CARTESIAN_POINT('Ctrl Pts',(3.66661143271648,-0.666666666666667,
-0.786422660833742));
#52801=CARTESIAN_POINT('Ctrl Pts',(3.66661143271648,-1.,-0.786422660833742));
#52802=CARTESIAN_POINT('Ctrl Pts',(4.13571194405636,-1.,-0.73204283740062));
#52803=CARTESIAN_POINT('Ctrl Pts',(4.13571194405636,1.,-0.73204283740062));
#52804=CARTESIAN_POINT('Ctrl Pts',(4.13420383737278,-1.,-0.732488575135926));
#52805=CARTESIAN_POINT('Ctrl Pts',(4.13420383737278,1.,-0.732488575135926));
#52806=CARTESIAN_POINT('Ctrl Pts',(4.13118752796397,-1.,-0.733376589325634));
#52807=CARTESIAN_POINT('Ctrl Pts',(4.13118752796397,1.,-0.733376589325634));
#52808=CARTESIAN_POINT('Ctrl Pts',(4.12666277572794,-1.,-0.734698226767513));
#52809=CARTESIAN_POINT('Ctrl Pts',(4.12666277572794,1.,-0.734698226767513));
#52810=CARTESIAN_POINT('Ctrl Pts',(4.12062919626082,-1.,-0.736439634335347));
#52811=CARTESIAN_POINT('Ctrl Pts',(4.12062919626082,1.,-0.736439634335347));
#52812=CARTESIAN_POINT('Ctrl Pts',(4.11308626953795,-1.,-0.738581708229119));
#52813=CARTESIAN_POINT('Ctrl Pts',(4.11308626953795,1.,-0.738581708229119));
#52814=CARTESIAN_POINT('Ctrl Pts',(4.1055424175856,-1.,-0.740688998555152));
#52815=CARTESIAN_POINT('Ctrl Pts',(4.1055424175856,1.,-0.740688998555152));
#52816=CARTESIAN_POINT('Ctrl Pts',(4.09799769702712,-1.,-0.742761369690018));
#52817=CARTESIAN_POINT('Ctrl Pts',(4.09799769702712,1.,-0.742761369690018));
#52818=CARTESIAN_POINT('Ctrl Pts',(4.09045220253011,-1.,-0.744798649705514));
#52819=CARTESIAN_POINT('Ctrl Pts',(4.09045220253011,1.,-0.744798649705514));
#52820=CARTESIAN_POINT('Ctrl Pts',(4.08290608094789,-1.,-0.746800631490822));
#52821=CARTESIAN_POINT('Ctrl Pts',(4.08290608094789,1.,-0.746800631490822));
#52822=CARTESIAN_POINT('Ctrl Pts',(4.07535951055363,-1.,-0.748767076679177));
#52823=CARTESIAN_POINT('Ctrl Pts',(4.07535951055363,1.,-0.748767076679177));
#52824=CARTESIAN_POINT('Ctrl Pts',(4.06781267241886,-1.,-0.750697720483176));
#52825=CARTESIAN_POINT('Ctrl Pts',(4.06781267241886,1.,-0.750697720483176));
#52826=CARTESIAN_POINT('Ctrl Pts',(4.06026572221399,-1.,-0.752592276482869));
#52827=CARTESIAN_POINT('Ctrl Pts',(4.06026572221399,1.,-0.752592276482869));
#52828=CARTESIAN_POINT('Ctrl Pts',(4.05271876688106,-1.,-0.754450441816412));
#52829=CARTESIAN_POINT('Ctrl Pts',(4.05271876688106,1.,-0.754450441816412));
#52830=CARTESIAN_POINT('Ctrl Pts',(4.04517182654344,-1.,-0.756271902370187));
#52831=CARTESIAN_POINT('Ctrl Pts',(4.04517182654344,1.,-0.756271902370187));
#52832=CARTESIAN_POINT('Ctrl Pts',(4.03762485803468,-1.,-0.758056338885554));
#52833=CARTESIAN_POINT('Ctrl Pts',(4.03762485803468,1.,-0.758056338885554));
#52834=CARTESIAN_POINT('Ctrl Pts',(4.0300778195465,-1.,-0.759803433244166));
#52835=CARTESIAN_POINT('Ctrl Pts',(4.0300778195465,1.,-0.759803433244166));
#52836=CARTESIAN_POINT('Ctrl Pts',(4.02253072741347,-1.,-0.761512875859942));
#52837=CARTESIAN_POINT('Ctrl Pts',(4.02253072741347,1.,-0.761512875859942));
#52838=CARTESIAN_POINT('Ctrl Pts',(4.01498370680434,-1.,-0.763184371182827));
#52839=CARTESIAN_POINT('Ctrl Pts',(4.01498370680434,1.,-0.763184371182827));
#52840=CARTESIAN_POINT('Ctrl Pts',(4.00743706791366,-1.,-0.764817648784947));
#52841=CARTESIAN_POINT('Ctrl Pts',(4.00743706791366,1.,-0.764817648784947));
#52842=CARTESIAN_POINT('Ctrl Pts',(3.99989129179464,-1.,-0.766412457135786));
#52843=CARTESIAN_POINT('Ctrl Pts',(3.99989129179464,1.,-0.766412457135786));
#52844=CARTESIAN_POINT('Ctrl Pts',(3.99234687880892,-1.,-0.767968531377708));
#52845=CARTESIAN_POINT('Ctrl Pts',(3.99234687880892,1.,-0.767968531377708));
#52846=CARTESIAN_POINT('Ctrl Pts',(3.98480422348403,-1.,-0.76948556624546));
#52847=CARTESIAN_POINT('Ctrl Pts',(3.98480422348403,1.,-0.76948556624546));
#52848=CARTESIAN_POINT('Ctrl Pts',(3.97726349165507,-1.,-0.770963190030504));
#52849=CARTESIAN_POINT('Ctrl Pts',(3.97726349165507,1.,-0.770963190030504));
#52850=CARTESIAN_POINT('Ctrl Pts',(3.96972446532832,-1.,-0.772400931772239));
#52851=CARTESIAN_POINT('Ctrl Pts',(3.96972446532832,1.,-0.772400931772239));
#52852=CARTESIAN_POINT('Ctrl Pts',(3.96218649639876,-1.,-0.773798212026683));
#52853=CARTESIAN_POINT('Ctrl Pts',(3.96218649639876,1.,-0.773798212026683));
#52854=CARTESIAN_POINT('Ctrl Pts',(3.95464885452364,-1.,-0.775154418039442));
#52855=CARTESIAN_POINT('Ctrl Pts',(3.95464885452364,1.,-0.775154418039442));
#52856=CARTESIAN_POINT('Ctrl Pts',(3.94711101619471,-1.,-0.77646896669796));
#52857=CARTESIAN_POINT('Ctrl Pts',(3.94711101619471,1.,-0.77646896669796));
#52858=CARTESIAN_POINT('Ctrl Pts',(3.93957296768098,-1.,-0.77774137056855));
#52859=CARTESIAN_POINT('Ctrl Pts',(3.93957296768098,1.,-0.77774137056855));
#52860=CARTESIAN_POINT('Ctrl Pts',(3.93203552473153,-1.,-0.778971308134786));
#52861=CARTESIAN_POINT('Ctrl Pts',(3.93203552473153,1.,-0.778971308134786));
#52862=CARTESIAN_POINT('Ctrl Pts',(3.92450058323799,-1.,-0.780158678615507));
#52863=CARTESIAN_POINT('Ctrl Pts',(3.92450058323799,1.,-0.780158678615507));
#52864=CARTESIAN_POINT('Ctrl Pts',(3.9169703605466,-1.,-0.781303428618344));
#52865=CARTESIAN_POINT('Ctrl Pts',(3.9169703605466,1.,-0.781303428618344));
#52866=CARTESIAN_POINT('Ctrl Pts',(3.90944671004536,-1.,-0.782405395622759));
#52867=CARTESIAN_POINT('Ctrl Pts',(3.90944671004536,1.,-0.782405395622759));
#52868=CARTESIAN_POINT('Ctrl Pts',(3.90193039043971,-1.,-0.783464141529083));
#52869=CARTESIAN_POINT('Ctrl Pts',(3.90193039043971,1.,-0.783464141529083));
#52870=CARTESIAN_POINT('Ctrl Pts',(3.89442039235105,-1.,-0.784478799358336));
#52871=CARTESIAN_POINT('Ctrl Pts',(3.89442039235105,1.,-0.784478799358336));
#52872=CARTESIAN_POINT('Ctrl Pts',(3.88691313167399,-1.,-0.785447890340723));
#52873=CARTESIAN_POINT('Ctrl Pts',(3.88691313167399,1.,-0.785447890340723));
#52874=CARTESIAN_POINT('Ctrl Pts',(3.87940402818186,-1.,-0.786369675812592));
#52875=CARTESIAN_POINT('Ctrl Pts',(3.87940402818186,1.,-0.786369675812592));
#52876=CARTESIAN_POINT('Ctrl Pts',(3.87188916600905,-1.,-0.787242527617981));
#52877=CARTESIAN_POINT('Ctrl Pts',(3.87188916600905,1.,-0.787242527617981));
#52878=CARTESIAN_POINT('Ctrl Pts',(3.86436702561342,-1.,-0.788065315093771));
#52879=CARTESIAN_POINT('Ctrl Pts',(3.86436702561342,1.,-0.788065315093771));
#52880=CARTESIAN_POINT('Ctrl Pts',(3.85683995872536,-1.,-0.788837734090688));
#52881=CARTESIAN_POINT('Ctrl Pts',(3.85683995872536,1.,-0.788837734090688));
#52882=CARTESIAN_POINT('Ctrl Pts',(3.8493163780891,-1.,-0.789560798155619));
#52883=CARTESIAN_POINT('Ctrl Pts',(3.8493163780891,1.,-0.789560798155619));
#52884=CARTESIAN_POINT('Ctrl Pts',(3.84180762342476,-1.,-0.790236124191289));
#52885=CARTESIAN_POINT('Ctrl Pts',(3.84180762342476,1.,-0.790236124191289));
#52886=CARTESIAN_POINT('Ctrl Pts',(3.83432392054804,-1.,-0.79086501270534));
#52887=CARTESIAN_POINT('Ctrl Pts',(3.83432392054804,1.,-0.79086501270534));
#52888=CARTESIAN_POINT('Ctrl Pts',(3.82687033899799,-1.,-0.791447528662381));
#52889=CARTESIAN_POINT('Ctrl Pts',(3.82687033899799,1.,-0.791447528662381));
#52890=CARTESIAN_POINT('Ctrl Pts',(3.81944345442237,-1.,-0.791981740718607));
#52891=CARTESIAN_POINT('Ctrl Pts',(3.81944345442237,1.,-0.791981740718607));
#52892=CARTESIAN_POINT('Ctrl Pts',(3.81202588694726,-1.,-0.792462483517568));
#52893=CARTESIAN_POINT('Ctrl Pts',(3.81202588694726,1.,-0.792462483517568));
#52894=CARTESIAN_POINT('Ctrl Pts',(3.80459229925598,-1.,-0.792882695234693));
#52895=CARTESIAN_POINT('Ctrl Pts',(3.80459229925598,1.,-0.792882695234693));
#52896=CARTESIAN_POINT('Ctrl Pts',(3.79711921389862,-1.,-0.793235612973201));
#52897=CARTESIAN_POINT('Ctrl Pts',(3.79711921389862,1.,-0.793235612973201));
#52898=CARTESIAN_POINT('Ctrl Pts',(3.78959439439222,-1.,-0.793516871680966));
#52899=CARTESIAN_POINT('Ctrl Pts',(3.78959439439222,1.,-0.793516871680966));
#52900=CARTESIAN_POINT('Ctrl Pts',(3.78202460377617,-1.,-0.79372623578134));
#52901=CARTESIAN_POINT('Ctrl Pts',(3.78202460377617,1.,-0.79372623578134));
#52902=CARTESIAN_POINT('Ctrl Pts',(3.77444863801264,-1.,-0.793870523787515));
#52903=CARTESIAN_POINT('Ctrl Pts',(3.77444863801264,1.,-0.793870523787515));
#52904=CARTESIAN_POINT('Ctrl Pts',(3.76692626931184,-1.,-0.793961083689141));
#52905=CARTESIAN_POINT('Ctrl Pts',(3.76692626931184,1.,-0.793961083689141));
#52906=CARTESIAN_POINT('Ctrl Pts',(3.75951468666325,-1.,-0.794008429135047));
#52907=CARTESIAN_POINT('Ctrl Pts',(3.75951468666325,1.,-0.794008429135047));
#52908=CARTESIAN_POINT('Ctrl Pts',(3.75224692493895,-1.,-0.794017347371441));
#52909=CARTESIAN_POINT('Ctrl Pts',(3.75224692493895,1.,-0.794017347371441));
#52910=CARTESIAN_POINT('Ctrl Pts',(3.74511357728827,-1.,-0.79398270045988));
#52911=CARTESIAN_POINT('Ctrl Pts',(3.74511357728827,1.,-0.79398270045988));
#52912=CARTESIAN_POINT('Ctrl Pts',(3.73803280541576,-1.,-0.793882700936791));
#52913=CARTESIAN_POINT('Ctrl Pts',(3.73803280541576,1.,-0.793882700936791));
#52914=CARTESIAN_POINT('Ctrl Pts',(3.7308691469564,-1.,-0.793682750269348));
#52915=CARTESIAN_POINT('Ctrl Pts',(3.7308691469564,1.,-0.793682750269348));
#52916=CARTESIAN_POINT('Ctrl Pts',(3.7234879729357,-1.,-0.793347023783871));
#52917=CARTESIAN_POINT('Ctrl Pts',(3.7234879729357,1.,-0.793347023783871));
#52918=CARTESIAN_POINT('Ctrl Pts',(3.7158024239604,-1.,-0.792848377370116));
#52919=CARTESIAN_POINT('Ctrl Pts',(3.7158024239604,1.,-0.792848377370116));
#52920=CARTESIAN_POINT('Ctrl Pts',(3.70781724021879,-1.,-0.792177688845968));
#52921=CARTESIAN_POINT('Ctrl Pts',(3.70781724021879,1.,-0.792177688845968));
#52922=CARTESIAN_POINT('Ctrl Pts',(3.69968940808982,-1.,-0.791356575696509));
#52923=CARTESIAN_POINT('Ctrl Pts',(3.69968940808982,1.,-0.791356575696509));
#52924=CARTESIAN_POINT('Ctrl Pts',(3.69172044327754,-1.,-0.79043628498958));
#52925=CARTESIAN_POINT('Ctrl Pts',(3.69172044327754,1.,-0.79043628498958));
#52926=CARTESIAN_POINT('Ctrl Pts',(3.68428439784285,-1.,-0.789483546065159));
#52927=CARTESIAN_POINT('Ctrl Pts',(3.68428439784285,1.,-0.789483546065159));
#52928=CARTESIAN_POINT('Ctrl Pts',(3.67777119516438,-1.,-0.788569566220663));
#52929=CARTESIAN_POINT('Ctrl Pts',(3.67777119516438,1.,-0.788569566220663));
#52930=CARTESIAN_POINT('Ctrl Pts',(3.672529236635,-1.,-0.787758799995427));
#52931=CARTESIAN_POINT('Ctrl Pts',(3.672529236635,1.,-0.787758799995427));
#52932=CARTESIAN_POINT('Ctrl Pts',(3.66879484800625,-1.,-0.787095252589508));
#52933=CARTESIAN_POINT('Ctrl Pts',(3.66879484800625,1.,-0.787095252589508));
#52934=CARTESIAN_POINT('Ctrl Pts',(3.66710211819938,-1.,-0.786698783541658));
#52935=CARTESIAN_POINT('Ctrl Pts',(3.66710211819938,1.,-0.786698783541658));
#52936=CARTESIAN_POINT('Ctrl Pts',(3.66657784454965,-1.,-0.786480236184947));
#52937=CARTESIAN_POINT('Ctrl Pts',(3.66657784454965,1.,-0.786480236184947));
#52938=CARTESIAN_POINT('Ctrl Pts',(3.66655932661846,-1.,-0.78636952818304));
#52939=CARTESIAN_POINT('Ctrl Pts',(3.66655932661846,1.,-0.78636952818304));
#52940=CARTESIAN_POINT('Ctrl Pts',(3.66663282329846,-1.,-0.786322922920599));
#52941=CARTESIAN_POINT('Ctrl Pts',(3.66663282329846,1.,-0.786322922920599));
#52942=CARTESIAN_POINT('',(4.13571194405636,1.,-0.73204283740062));
#52943=CARTESIAN_POINT('Ctrl Pts',(4.13571194405636,1.,-0.73204283740062));
#52944=CARTESIAN_POINT('Ctrl Pts',(4.13420383737278,1.,-0.732488575135926));
#52945=CARTESIAN_POINT('Ctrl Pts',(4.13118752796397,1.,-0.733376589325634));
#52946=CARTESIAN_POINT('Ctrl Pts',(4.12666277572794,1.,-0.734698226767513));
#52947=CARTESIAN_POINT('Ctrl Pts',(4.12062919626082,1.,-0.736439634335347));
#52948=CARTESIAN_POINT('Ctrl Pts',(4.11308626953795,1.,-0.738581708229119));
#52949=CARTESIAN_POINT('Ctrl Pts',(4.1055424175856,1.,-0.740688998555152));
#52950=CARTESIAN_POINT('Ctrl Pts',(4.09799769702712,1.,-0.742761369690018));
#52951=CARTESIAN_POINT('Ctrl Pts',(4.09045220253011,1.,-0.744798649705514));
#52952=CARTESIAN_POINT('Ctrl Pts',(4.08290608094789,1.,-0.746800631490822));
#52953=CARTESIAN_POINT('Ctrl Pts',(4.07535951055363,1.,-0.748767076679177));
#52954=CARTESIAN_POINT('Ctrl Pts',(4.06781267241886,1.,-0.750697720483176));
#52955=CARTESIAN_POINT('Ctrl Pts',(4.06026572221399,1.,-0.752592276482869));
#52956=CARTESIAN_POINT('Ctrl Pts',(4.05271876688106,1.,-0.754450441816412));
#52957=CARTESIAN_POINT('Ctrl Pts',(4.04517182654344,1.,-0.756271902370187));
#52958=CARTESIAN_POINT('Ctrl Pts',(4.03762485803468,1.,-0.758056338885554));
#52959=CARTESIAN_POINT('Ctrl Pts',(4.0300778195465,1.,-0.759803433244166));
#52960=CARTESIAN_POINT('Ctrl Pts',(4.02253072741347,1.,-0.761512875859942));
#52961=CARTESIAN_POINT('Ctrl Pts',(4.01498370680434,1.,-0.763184371182827));
#52962=CARTESIAN_POINT('Ctrl Pts',(4.00743706791366,1.,-0.764817648784947));
#52963=CARTESIAN_POINT('Ctrl Pts',(3.99989129179464,1.,-0.766412457135786));
#52964=CARTESIAN_POINT('Ctrl Pts',(3.99234687880892,1.,-0.767968531377708));
#52965=CARTESIAN_POINT('Ctrl Pts',(3.98480422348403,1.,-0.76948556624546));
#52966=CARTESIAN_POINT('Ctrl Pts',(3.97726349165507,1.,-0.770963190030504));
#52967=CARTESIAN_POINT('Ctrl Pts',(3.96972446532832,1.,-0.772400931772239));
#52968=CARTESIAN_POINT('Ctrl Pts',(3.96218649639876,1.,-0.773798212026683));
#52969=CARTESIAN_POINT('Ctrl Pts',(3.95464885452364,1.,-0.775154418039442));
#52970=CARTESIAN_POINT('Ctrl Pts',(3.94711101619471,1.,-0.77646896669796));
#52971=CARTESIAN_POINT('Ctrl Pts',(3.93957296768098,1.,-0.77774137056855));
#52972=CARTESIAN_POINT('Ctrl Pts',(3.93203552473153,1.,-0.778971308134786));
#52973=CARTESIAN_POINT('Ctrl Pts',(3.92450058323799,1.,-0.780158678615507));
#52974=CARTESIAN_POINT('Ctrl Pts',(3.9169703605466,1.,-0.781303428618344));
#52975=CARTESIAN_POINT('Ctrl Pts',(3.90944671004536,1.,-0.782405395622759));
#52976=CARTESIAN_POINT('Ctrl Pts',(3.90193039043971,1.,-0.783464141529083));
#52977=CARTESIAN_POINT('Ctrl Pts',(3.89442039235105,1.,-0.784478799358336));
#52978=CARTESIAN_POINT('Ctrl Pts',(3.88691313167399,1.,-0.785447890340723));
#52979=CARTESIAN_POINT('Ctrl Pts',(3.87940402818186,1.,-0.786369675812592));
#52980=CARTESIAN_POINT('Ctrl Pts',(3.87188916600905,1.,-0.787242527617981));
#52981=CARTESIAN_POINT('Ctrl Pts',(3.86436702561342,1.,-0.788065315093771));
#52982=CARTESIAN_POINT('Ctrl Pts',(3.85683995872536,1.,-0.788837734090688));
#52983=CARTESIAN_POINT('Ctrl Pts',(3.8493163780891,1.,-0.789560798155619));
#52984=CARTESIAN_POINT('Ctrl Pts',(3.84180762342476,1.,-0.790236124191289));
#52985=CARTESIAN_POINT('Ctrl Pts',(3.83432392054804,1.,-0.79086501270534));
#52986=CARTESIAN_POINT('Ctrl Pts',(3.82687033899799,1.,-0.791447528662381));
#52987=CARTESIAN_POINT('Ctrl Pts',(3.81944345442237,1.,-0.791981740718607));
#52988=CARTESIAN_POINT('Ctrl Pts',(3.81202588694726,1.,-0.792462483517568));
#52989=CARTESIAN_POINT('Ctrl Pts',(3.80459229925598,1.,-0.792882695234693));
#52990=CARTESIAN_POINT('Ctrl Pts',(3.79711921389862,1.,-0.793235612973201));
#52991=CARTESIAN_POINT('Ctrl Pts',(3.78959439439222,1.,-0.793516871680966));
#52992=CARTESIAN_POINT('Ctrl Pts',(3.78202460377617,1.,-0.79372623578134));
#52993=CARTESIAN_POINT('Ctrl Pts',(3.77444863801264,1.,-0.793870523787515));
#52994=CARTESIAN_POINT('Ctrl Pts',(3.76692626931184,1.,-0.793961083689141));
#52995=CARTESIAN_POINT('Ctrl Pts',(3.75951468666325,1.,-0.794008429135047));
#52996=CARTESIAN_POINT('Ctrl Pts',(3.75224692493895,1.,-0.794017347371441));
#52997=CARTESIAN_POINT('Ctrl Pts',(3.74511357728827,1.,-0.79398270045988));
#52998=CARTESIAN_POINT('Ctrl Pts',(3.73803280541576,1.,-0.793882700936791));
#52999=CARTESIAN_POINT('Ctrl Pts',(3.7308691469564,1.,-0.793682750269348));
#53000=CARTESIAN_POINT('Ctrl Pts',(3.7234879729357,1.,-0.793347023783871));
#53001=CARTESIAN_POINT('Ctrl Pts',(3.7158024239604,1.,-0.792848377370116));
#53002=CARTESIAN_POINT('Ctrl Pts',(3.70781724021879,1.,-0.792177688845968));
#53003=CARTESIAN_POINT('Ctrl Pts',(3.69968940808982,1.,-0.791356575696509));
#53004=CARTESIAN_POINT('Ctrl Pts',(3.69172044327754,1.,-0.79043628498958));
#53005=CARTESIAN_POINT('Ctrl Pts',(3.68428439784285,1.,-0.789483546065159));
#53006=CARTESIAN_POINT('Ctrl Pts',(3.67777119516438,1.,-0.788569566220663));
#53007=CARTESIAN_POINT('Ctrl Pts',(3.672529236635,1.,-0.787758799995427));
#53008=CARTESIAN_POINT('Ctrl Pts',(3.66907505398769,1.,-0.787145041181589));
#53009=CARTESIAN_POINT('Ctrl Pts',(3.66743103898844,1.,-0.7867743371985));
#53010=CARTESIAN_POINT('Ctrl Pts',(3.66680946938396,1.,-0.78656591955989));
#53011=CARTESIAN_POINT('Ctrl Pts',(3.66664310415236,1.,-0.786459983896781));
#53012=CARTESIAN_POINT('Ctrl Pts',(3.66661143271648,1.,-0.786422660833743));
#53013=CARTESIAN_POINT('',(4.13571194405636,0.,-0.73204283740062));
#53014=CARTESIAN_POINT('Origin',(4.15950947128175,0.,-0.581791163835815));
#53015=CARTESIAN_POINT('',(4.15950947128175,1.,-0.581791163835815));
#53016=CARTESIAN_POINT('',(4.13571194405636,1.,-0.73204283740062));
#53017=CARTESIAN_POINT('',(4.15950947128175,0.,-0.581791163835815));
#53018=CARTESIAN_POINT('Ctrl Pts',(3.73016218570874,-1.,-0.385214314776329));
#53019=CARTESIAN_POINT('Ctrl Pts',(3.73016218570874,1.,-0.385214314776329));
#53020=CARTESIAN_POINT('Ctrl Pts',(3.73010668803185,-1.,-0.385147278814804));
#53021=CARTESIAN_POINT('Ctrl Pts',(3.73010668803185,1.,-0.385147278814804));
#53022=CARTESIAN_POINT('Ctrl Pts',(3.73015851028729,-1.,-0.385047711603887));
#53023=CARTESIAN_POINT('Ctrl Pts',(3.73015851028729,1.,-0.385047711603887));
#53024=CARTESIAN_POINT('Ctrl Pts',(3.73072465900727,-1.,-0.385001870183842));
#53025=CARTESIAN_POINT('Ctrl Pts',(3.73072465900727,1.,-0.385001870183842));
#53026=CARTESIAN_POINT('Ctrl Pts',(3.73245705639337,-1.,-0.385147887989515));
#53027=CARTESIAN_POINT('Ctrl Pts',(3.73245705639337,1.,-0.385147887989515));
#53028=CARTESIAN_POINT('Ctrl Pts',(3.73621371845475,-1.,-0.385670806454744));
#53029=CARTESIAN_POINT('Ctrl Pts',(3.73621371845475,1.,-0.385670806454744));
#53030=CARTESIAN_POINT('Ctrl Pts',(3.74144965781088,-1.,-0.386519576222036));
#53031=CARTESIAN_POINT('Ctrl Pts',(3.74144965781088,1.,-0.386519576222036));
#53032=CARTESIAN_POINT('Ctrl Pts',(3.74792651696269,-1.,-0.387663020050396));
#53033=CARTESIAN_POINT('Ctrl Pts',(3.74792651696269,1.,-0.387663020050396));
#53034=CARTESIAN_POINT('Ctrl Pts',(3.75529302894757,-1.,-0.389054775898251));
#53035=CARTESIAN_POINT('Ctrl Pts',(3.75529302894757,1.,-0.389054775898251));
#53036=CARTESIAN_POINT('Ctrl Pts',(3.76315635032993,-1.,-0.390642072979259));
#53037=CARTESIAN_POINT('Ctrl Pts',(3.76315635032993,1.,-0.390642072979259));
#53038=CARTESIAN_POINT('Ctrl Pts',(3.77114011595892,-1.,-0.392372786223347));
#53039=CARTESIAN_POINT('Ctrl Pts',(3.77114011595892,1.,-0.392372786223347));
#53040=CARTESIAN_POINT('Ctrl Pts',(3.77894173114368,-1.,-0.394202481011595));
#53041=CARTESIAN_POINT('Ctrl Pts',(3.77894173114368,1.,-0.394202481011595));
#53042=CARTESIAN_POINT('Ctrl Pts',(3.78640521279479,-1.,-0.396103205335029));
#53043=CARTESIAN_POINT('Ctrl Pts',(3.78640521279479,1.,-0.396103205335029));
#53044=CARTESIAN_POINT('Ctrl Pts',(3.79352887163457,-1.,-0.398064818684159));
#53045=CARTESIAN_POINT('Ctrl Pts',(3.79352887163457,1.,-0.398064818684159));
#53046=CARTESIAN_POINT('Ctrl Pts',(3.80040370384659,-1.,-0.400088346504727));
#53047=CARTESIAN_POINT('Ctrl Pts',(3.80040370384659,1.,-0.400088346504727));
#53048=CARTESIAN_POINT('Ctrl Pts',(3.80716881962763,-1.,-0.402181320148475));
#53049=CARTESIAN_POINT('Ctrl Pts',(3.80716881962763,1.,-0.402181320148475));
#53050=CARTESIAN_POINT('Ctrl Pts',(3.81396374287762,-1.,-0.404352694628237));
#53051=CARTESIAN_POINT('Ctrl Pts',(3.81396374287762,1.,-0.404352694628237));
#53052=CARTESIAN_POINT('Ctrl Pts',(3.82087303913741,-1.,-0.406607038258907));
#53053=CARTESIAN_POINT('Ctrl Pts',(3.82087303913741,1.,-0.406607038258907));
#53054=CARTESIAN_POINT('Ctrl Pts',(3.82790724256397,-1.,-0.408942371447377));
#53055=CARTESIAN_POINT('Ctrl Pts',(3.82790724256397,1.,-0.408942371447377));
#53056=CARTESIAN_POINT('Ctrl Pts',(3.83503345578645,-1.,-0.41135303879846));
#53057=CARTESIAN_POINT('Ctrl Pts',(3.83503345578645,1.,-0.41135303879846));
#53058=CARTESIAN_POINT('Ctrl Pts',(3.84219403994742,-1.,-0.413831367016727));
#53059=CARTESIAN_POINT('Ctrl Pts',(3.84219403994742,1.,-0.413831367016727));
#53060=CARTESIAN_POINT('Ctrl Pts',(3.8493286415751,-1.,-0.41636967805292));
#53061=CARTESIAN_POINT('Ctrl Pts',(3.8493286415751,1.,-0.41636967805292));
#53062=CARTESIAN_POINT('Ctrl Pts',(3.85639825648031,-1.,-0.41896246808681));
#53063=CARTESIAN_POINT('Ctrl Pts',(3.85639825648031,1.,-0.41896246808681));
#53064=CARTESIAN_POINT('Ctrl Pts',(3.86339652542749,-1.,-0.421607423177576));
#53065=CARTESIAN_POINT('Ctrl Pts',(3.86339652542749,1.,-0.421607423177576));
#53066=CARTESIAN_POINT('Ctrl Pts',(3.87033643487882,-1.,-0.424304173195143));
#53067=CARTESIAN_POINT('Ctrl Pts',(3.87033643487882,1.,-0.424304173195143));
#53068=CARTESIAN_POINT('Ctrl Pts',(3.87724240306609,-1.,-0.427053541173469));
#53069=CARTESIAN_POINT('Ctrl Pts',(3.87724240306609,1.,-0.427053541173469));
#53070=CARTESIAN_POINT('Ctrl Pts',(3.88414070943334,-1.,-0.429856640579734));
#53071=CARTESIAN_POINT('Ctrl Pts',(3.88414070943334,1.,-0.429856640579734));
#53072=CARTESIAN_POINT('Ctrl Pts',(3.89104947940592,-1.,-0.43271392954444));
#53073=CARTESIAN_POINT('Ctrl Pts',(3.89104947940592,1.,-0.43271392954444));
#53074=CARTESIAN_POINT('Ctrl Pts',(3.8979725665544,-1.,-0.435624629433506));
#53075=CARTESIAN_POINT('Ctrl Pts',(3.8979725665544,1.,-0.435624629433506));
#53076=CARTESIAN_POINT('Ctrl Pts',(3.90490512938546,-1.,-0.438587235458234));
#53077=CARTESIAN_POINT('Ctrl Pts',(3.90490512938546,1.,-0.438587235458234));
#53078=CARTESIAN_POINT('Ctrl Pts',(3.91183704069146,-1.,-0.441599824524048));
#53079=CARTESIAN_POINT('Ctrl Pts',(3.91183704069146,1.,-0.441599824524048));
#53080=CARTESIAN_POINT('Ctrl Pts',(3.91875701610721,-1.,-0.444660430230593));
#53081=CARTESIAN_POINT('Ctrl Pts',(3.91875701610721,1.,-0.444660430230593));
#53082=CARTESIAN_POINT('Ctrl Pts',(3.92565674143424,-1.,-0.447767416837297));
#53083=CARTESIAN_POINT('Ctrl Pts',(3.92565674143424,1.,-0.447767416837297));
#53084=CARTESIAN_POINT('Ctrl Pts',(3.93253407403128,-1.,-0.450919768356347));
#53085=CARTESIAN_POINT('Ctrl Pts',(3.93253407403128,1.,-0.450919768356347));
#53086=CARTESIAN_POINT('Ctrl Pts',(3.93939080846298,-1.,-0.454116879027576));
#53087=CARTESIAN_POINT('Ctrl Pts',(3.93939080846298,1.,-0.454116879027576));
#53088=CARTESIAN_POINT('Ctrl Pts',(3.94623117206675,-1.,-0.457358410451674));
#53089=CARTESIAN_POINT('Ctrl Pts',(3.94623117206675,1.,-0.457358410451674));
#53090=CARTESIAN_POINT('Ctrl Pts',(3.95306005817363,-1.,-0.460644124429119));
#53091=CARTESIAN_POINT('Ctrl Pts',(3.95306005817363,1.,-0.460644124429119));
#53092=CARTESIAN_POINT('Ctrl Pts',(3.95988133243543,-1.,-0.463973722115745));
#53093=CARTESIAN_POINT('Ctrl Pts',(3.95988133243543,1.,-0.463973722115745));
#53094=CARTESIAN_POINT('Ctrl Pts',(3.96669622273946,-1.,-0.467346690880672));
#53095=CARTESIAN_POINT('Ctrl Pts',(3.96669622273946,1.,-0.467346690880672));
#53096=CARTESIAN_POINT('Ctrl Pts',(3.97350414289415,-1.,-0.470762379613478));
#53097=CARTESIAN_POINT('Ctrl Pts',(3.97350414289415,1.,-0.470762379613478));
#53098=CARTESIAN_POINT('Ctrl Pts',(3.9803033804443,-1.,-0.474220061019542));
#53099=CARTESIAN_POINT('Ctrl Pts',(3.9803033804443,1.,-0.474220061019542));
#53100=CARTESIAN_POINT('Ctrl Pts',(3.98709184306743,-1.,-0.477718999122033));
#53101=CARTESIAN_POINT('Ctrl Pts',(3.98709184306743,1.,-0.477718999122033));
#53102=CARTESIAN_POINT('Ctrl Pts',(3.99386775880655,-1.,-0.481258512209638));
#53103=CARTESIAN_POINT('Ctrl Pts',(3.99386775880655,1.,-0.481258512209638));
#53104=CARTESIAN_POINT('Ctrl Pts',(4.00063045119234,-1.,-0.484838042421754));
#53105=CARTESIAN_POINT('Ctrl Pts',(4.00063045119234,1.,-0.484838042421754));
#53106=CARTESIAN_POINT('Ctrl Pts',(4.0073800839092,-1.,-0.488457130424531));
#53107=CARTESIAN_POINT('Ctrl Pts',(4.0073800839092,1.,-0.488457130424531));
#53108=CARTESIAN_POINT('Ctrl Pts',(4.01411733503486,-1.,-0.492115383417931));
#53109=CARTESIAN_POINT('Ctrl Pts',(4.01411733503486,1.,-0.492115383417931));
#53110=CARTESIAN_POINT('Ctrl Pts',(4.02084308851813,-1.,-0.495812444326223));
#53111=CARTESIAN_POINT('Ctrl Pts',(4.02084308851813,1.,-0.495812444326223));
#53112=CARTESIAN_POINT('Ctrl Pts',(4.0275581398015,-1.,-0.49954796234089));
#53113=CARTESIAN_POINT('Ctrl Pts',(4.0275581398015,1.,-0.49954796234089));
#53114=CARTESIAN_POINT('Ctrl Pts',(4.0342628417439,-1.,-0.503321556915514));
#53115=CARTESIAN_POINT('Ctrl Pts',(4.0342628417439,1.,-0.503321556915514));
#53116=CARTESIAN_POINT('Ctrl Pts',(4.04095715149074,-1.,-0.507132823288362));
#53117=CARTESIAN_POINT('Ctrl Pts',(4.04095715149074,1.,-0.507132823288362));
#53118=CARTESIAN_POINT('Ctrl Pts',(4.04764078815591,-1.,-0.510981349219174));
#53119=CARTESIAN_POINT('Ctrl Pts',(4.04764078815591,1.,-0.510981349219174));
#53120=CARTESIAN_POINT('Ctrl Pts',(4.05431335771261,-1.,-0.514866728193104));
#53121=CARTESIAN_POINT('Ctrl Pts',(4.05431335771261,1.,-0.514866728193104));
#53122=CARTESIAN_POINT('Ctrl Pts',(4.06097448037934,-1.,-0.51878857233681));
#53123=CARTESIAN_POINT('Ctrl Pts',(4.06097448037934,1.,-0.51878857233681));
#53124=CARTESIAN_POINT('Ctrl Pts',(4.06762394471075,-1.,-0.522746528602768));
#53125=CARTESIAN_POINT('Ctrl Pts',(4.06762394471075,1.,-0.522746528602768));
#53126=CARTESIAN_POINT('Ctrl Pts',(4.07426172299496,-1.,-0.526740277227));
#53127=CARTESIAN_POINT('Ctrl Pts',(4.07426172299496,1.,-0.526740277227));
#53128=CARTESIAN_POINT('Ctrl Pts',(4.08088789536488,-1.,-0.530769518728076));
#53129=CARTESIAN_POINT('Ctrl Pts',(4.08088789536488,1.,-0.530769518728076));
#53130=CARTESIAN_POINT('Ctrl Pts',(4.08750259988693,-1.,-0.534833963477));
#53131=CARTESIAN_POINT('Ctrl Pts',(4.08750259988693,1.,-0.534833963477));
#53132=CARTESIAN_POINT('Ctrl Pts',(4.09410597627116,-1.,-0.538933321179921));
#53133=CARTESIAN_POINT('Ctrl Pts',(4.09410597627116,1.,-0.538933321179921));
#53134=CARTESIAN_POINT('Ctrl Pts',(4.10069810244473,-1.,-0.543067286878457));
#53135=CARTESIAN_POINT('Ctrl Pts',(4.10069810244473,1.,-0.543067286878457));
#53136=CARTESIAN_POINT('Ctrl Pts',(4.1072789702877,-1.,-0.54723553948676));
#53137=CARTESIAN_POINT('Ctrl Pts',(4.1072789702877,1.,-0.54723553948676));
#53138=CARTESIAN_POINT('Ctrl Pts',(4.11384852025578,-1.,-0.551437758498247));
#53139=CARTESIAN_POINT('Ctrl Pts',(4.11384852025578,1.,-0.551437758498247));
#53140=CARTESIAN_POINT('Ctrl Pts',(4.1204066619623,-1.,-0.555673636130778));
#53141=CARTESIAN_POINT('Ctrl Pts',(4.1204066619623,1.,-0.555673636130778));
#53142=CARTESIAN_POINT('Ctrl Pts',(4.12695329951859,-1.,-0.559942890594628));
#53143=CARTESIAN_POINT('Ctrl Pts',(4.12695329951859,1.,-0.559942890594628));
#53144=CARTESIAN_POINT('Ctrl Pts',(4.13348835726086,-1.,-0.564245279535706));
#53145=CARTESIAN_POINT('Ctrl Pts',(4.13348835726086,1.,-0.564245279535706));
#53146=CARTESIAN_POINT('Ctrl Pts',(4.14001179828669,-1.,-0.568580610187116));
#53147=CARTESIAN_POINT('Ctrl Pts',(4.14001179828669,1.,-0.568580610187116));
#53148=CARTESIAN_POINT('Ctrl Pts',(4.14652361065787,-1.,-0.572948736066277));
#53149=CARTESIAN_POINT('Ctrl Pts',(4.14652361065787,1.,-0.572948736066277));
#53150=CARTESIAN_POINT('Ctrl Pts',(4.1517237611974,-1.,-0.576469391673917));
#53151=CARTESIAN_POINT('Ctrl Pts',(4.1517237611974,1.,-0.576469391673917));
#53152=CARTESIAN_POINT('Ctrl Pts',(4.15561864787379,-1.,-0.579124568912544));
#53153=CARTESIAN_POINT('Ctrl Pts',(4.15561864787379,1.,-0.579124568912544));
#53154=CARTESIAN_POINT('Ctrl Pts',(4.15821291712391,-1.,-0.580901211462913));
#53155=CARTESIAN_POINT('Ctrl Pts',(4.15821291712391,1.,-0.580901211462913));
#53156=CARTESIAN_POINT('Ctrl Pts',(4.15950947128175,-1.,-0.581791163835815));
#53157=CARTESIAN_POINT('Ctrl Pts',(4.15950947128175,1.,-0.581791163835815));
#53158=CARTESIAN_POINT('',(3.73017266276632,1.,-0.385112848332548));
#53159=CARTESIAN_POINT('Ctrl Pts',(3.73017266276632,-1.,-0.385112848332549));
#53160=CARTESIAN_POINT('Ctrl Pts',(3.73017266276632,-0.666666666666667,
-0.385112848332549));
#53161=CARTESIAN_POINT('Ctrl Pts',(3.73017266276632,-0.333333333333333,
-0.385112848332549));
#53162=CARTESIAN_POINT('Ctrl Pts',(3.73017266276632,0.333333333333333,-0.385112848332549));
#53163=CARTESIAN_POINT('Ctrl Pts',(3.73017266276632,0.666666666666667,-0.38511284833255));
#53164=CARTESIAN_POINT('Ctrl Pts',(3.73017266276632,1.,-0.38511284833255));
#53165=CARTESIAN_POINT('Ctrl Pts',(3.73017266276632,1.,-0.385112848332549));
#53166=CARTESIAN_POINT('Ctrl Pts',(3.73021431755218,1.,-0.385087139001609));
#53167=CARTESIAN_POINT('Ctrl Pts',(3.73040527620929,1.,-0.385037797882046));
#53168=CARTESIAN_POINT('Ctrl Pts',(3.731060828624,1.,-0.385031656499142));
#53169=CARTESIAN_POINT('Ctrl Pts',(3.73273893363318,1.,-0.385187124633965));
#53170=CARTESIAN_POINT('Ctrl Pts',(3.73621371845475,1.,-0.385670806454744));
#53171=CARTESIAN_POINT('Ctrl Pts',(3.74144965781088,1.,-0.386519576222036));
#53172=CARTESIAN_POINT('Ctrl Pts',(3.74792651696269,1.,-0.387663020050396));
#53173=CARTESIAN_POINT('Ctrl Pts',(3.75529302894757,1.,-0.389054775898251));
#53174=CARTESIAN_POINT('Ctrl Pts',(3.76315635032993,1.,-0.390642072979259));
#53175=CARTESIAN_POINT('Ctrl Pts',(3.77114011595892,1.,-0.392372786223347));
#53176=CARTESIAN_POINT('Ctrl Pts',(3.77894173114368,1.,-0.394202481011595));
#53177=CARTESIAN_POINT('Ctrl Pts',(3.78640521279479,1.,-0.396103205335029));
#53178=CARTESIAN_POINT('Ctrl Pts',(3.79352887163457,1.,-0.398064818684159));
#53179=CARTESIAN_POINT('Ctrl Pts',(3.80040370384659,1.,-0.400088346504727));
#53180=CARTESIAN_POINT('Ctrl Pts',(3.80716881962763,1.,-0.402181320148475));
#53181=CARTESIAN_POINT('Ctrl Pts',(3.81396374287762,1.,-0.404352694628237));
#53182=CARTESIAN_POINT('Ctrl Pts',(3.82087303913741,1.,-0.406607038258907));
#53183=CARTESIAN_POINT('Ctrl Pts',(3.82790724256397,1.,-0.408942371447377));
#53184=CARTESIAN_POINT('Ctrl Pts',(3.83503345578645,1.,-0.41135303879846));
#53185=CARTESIAN_POINT('Ctrl Pts',(3.84219403994742,1.,-0.413831367016727));
#53186=CARTESIAN_POINT('Ctrl Pts',(3.8493286415751,1.,-0.41636967805292));
#53187=CARTESIAN_POINT('Ctrl Pts',(3.85639825648031,1.,-0.41896246808681));
#53188=CARTESIAN_POINT('Ctrl Pts',(3.86339652542749,1.,-0.421607423177576));
#53189=CARTESIAN_POINT('Ctrl Pts',(3.87033643487882,1.,-0.424304173195143));
#53190=CARTESIAN_POINT('Ctrl Pts',(3.87724240306609,1.,-0.427053541173469));
#53191=CARTESIAN_POINT('Ctrl Pts',(3.88414070943334,1.,-0.429856640579734));
#53192=CARTESIAN_POINT('Ctrl Pts',(3.89104947940592,1.,-0.43271392954444));
#53193=CARTESIAN_POINT('Ctrl Pts',(3.8979725665544,1.,-0.435624629433506));
#53194=CARTESIAN_POINT('Ctrl Pts',(3.90490512938546,1.,-0.438587235458234));
#53195=CARTESIAN_POINT('Ctrl Pts',(3.91183704069146,1.,-0.441599824524048));
#53196=CARTESIAN_POINT('Ctrl Pts',(3.91875701610721,1.,-0.444660430230593));
#53197=CARTESIAN_POINT('Ctrl Pts',(3.92565674143424,1.,-0.447767416837297));
#53198=CARTESIAN_POINT('Ctrl Pts',(3.93253407403128,1.,-0.450919768356347));
#53199=CARTESIAN_POINT('Ctrl Pts',(3.93939080846298,1.,-0.454116879027576));
#53200=CARTESIAN_POINT('Ctrl Pts',(3.94623117206675,1.,-0.457358410451674));
#53201=CARTESIAN_POINT('Ctrl Pts',(3.95306005817363,1.,-0.460644124429119));
#53202=CARTESIAN_POINT('Ctrl Pts',(3.95988133243543,1.,-0.463973722115745));
#53203=CARTESIAN_POINT('Ctrl Pts',(3.96669622273946,1.,-0.467346690880672));
#53204=CARTESIAN_POINT('Ctrl Pts',(3.97350414289415,1.,-0.470762379613478));
#53205=CARTESIAN_POINT('Ctrl Pts',(3.9803033804443,1.,-0.474220061019542));
#53206=CARTESIAN_POINT('Ctrl Pts',(3.98709184306743,1.,-0.477718999122033));
#53207=CARTESIAN_POINT('Ctrl Pts',(3.99386775880655,1.,-0.481258512209638));
#53208=CARTESIAN_POINT('Ctrl Pts',(4.00063045119234,1.,-0.484838042421754));
#53209=CARTESIAN_POINT('Ctrl Pts',(4.0073800839092,1.,-0.488457130424531));
#53210=CARTESIAN_POINT('Ctrl Pts',(4.01411733503486,1.,-0.492115383417931));
#53211=CARTESIAN_POINT('Ctrl Pts',(4.02084308851813,1.,-0.495812444326223));
#53212=CARTESIAN_POINT('Ctrl Pts',(4.0275581398015,1.,-0.49954796234089));
#53213=CARTESIAN_POINT('Ctrl Pts',(4.0342628417439,1.,-0.503321556915514));
#53214=CARTESIAN_POINT('Ctrl Pts',(4.04095715149074,1.,-0.507132823288362));
#53215=CARTESIAN_POINT('Ctrl Pts',(4.04764078815591,1.,-0.510981349219174));
#53216=CARTESIAN_POINT('Ctrl Pts',(4.05431335771261,1.,-0.514866728193104));
#53217=CARTESIAN_POINT('Ctrl Pts',(4.06097448037934,1.,-0.51878857233681));
#53218=CARTESIAN_POINT('Ctrl Pts',(4.06762394471075,1.,-0.522746528602768));
#53219=CARTESIAN_POINT('Ctrl Pts',(4.07426172299496,1.,-0.526740277227));
#53220=CARTESIAN_POINT('Ctrl Pts',(4.08088789536488,1.,-0.530769518728076));
#53221=CARTESIAN_POINT('Ctrl Pts',(4.08750259988693,1.,-0.534833963477));
#53222=CARTESIAN_POINT('Ctrl Pts',(4.09410597627116,1.,-0.538933321179921));
#53223=CARTESIAN_POINT('Ctrl Pts',(4.10069810244473,1.,-0.543067286878457));
#53224=CARTESIAN_POINT('Ctrl Pts',(4.1072789702877,1.,-0.54723553948676));
#53225=CARTESIAN_POINT('Ctrl Pts',(4.11384852025578,1.,-0.551437758498247));
#53226=CARTESIAN_POINT('Ctrl Pts',(4.1204066619623,1.,-0.555673636130778));
#53227=CARTESIAN_POINT('Ctrl Pts',(4.12695329951859,1.,-0.559942890594628));
#53228=CARTESIAN_POINT('Ctrl Pts',(4.13348835726086,1.,-0.564245279535706));
#53229=CARTESIAN_POINT('Ctrl Pts',(4.14001179828669,1.,-0.568580610187116));
#53230=CARTESIAN_POINT('Ctrl Pts',(4.14652361065787,1.,-0.572948736066277));
#53231=CARTESIAN_POINT('Ctrl Pts',(4.1517237611974,1.,-0.576469391673917));
#53232=CARTESIAN_POINT('Ctrl Pts',(4.15561864787379,1.,-0.579124568912544));
#53233=CARTESIAN_POINT('Ctrl Pts',(4.15821291712391,1.,-0.580901211462913));
#53234=CARTESIAN_POINT('Ctrl Pts',(4.15950947128175,1.,-0.581791163835815));
#53235=CARTESIAN_POINT('Origin',(0.,0.,0.));
#53236=CARTESIAN_POINT('',(3.74449296982994,1.,-0.203156094897896));
#53237=CARTESIAN_POINT('Origin',(0.,1.,0.));
#53238=CARTESIAN_POINT('Ctrl Pts',(3.74449296982994,1.,-0.203156094897896));
#53239=CARTESIAN_POINT('Ctrl Pts',(3.74449296982994,0.666666666666667,-0.203156094897896));
#53240=CARTESIAN_POINT('Ctrl Pts',(3.74449296982994,0.333333333333333,-0.203156094897896));
#53241=CARTESIAN_POINT('Ctrl Pts',(3.74449296982994,-0.333333333333333,
-0.203156094897896));
#53242=CARTESIAN_POINT('Ctrl Pts',(3.74449296982994,-0.666666666666667,
-0.203156094897895));
#53243=CARTESIAN_POINT('Ctrl Pts',(3.74449296982994,-1.,-0.203156094897895));
#53244=CARTESIAN_POINT('Ctrl Pts',(3.74449849461127,-1.,0.20305423869972));
#53245=CARTESIAN_POINT('Ctrl Pts',(3.74449849461127,1.,0.20305423869972));
#53246=CARTESIAN_POINT('Ctrl Pts',(3.7444331934681,-1.,0.203111767587923));
#53247=CARTESIAN_POINT('Ctrl Pts',(3.7444331934681,1.,0.203111767587923));
#53248=CARTESIAN_POINT('Ctrl Pts',(3.7444688019622,-1.,0.203218215748058));
#53249=CARTESIAN_POINT('Ctrl Pts',(3.7444688019622,1.,0.203218215748058));
#53250=CARTESIAN_POINT('Ctrl Pts',(3.74502080927395,-1.,0.203352057956297));
#53251=CARTESIAN_POINT('Ctrl Pts',(3.74502080927395,1.,0.203352057956297));
#53252=CARTESIAN_POINT('Ctrl Pts',(3.7467547201908,-1.,0.203478844530446));
#53253=CARTESIAN_POINT('Ctrl Pts',(3.7467547201908,1.,0.203478844530446));
#53254=CARTESIAN_POINT('Ctrl Pts',(3.75054693397875,-1.,0.203550035479166));
#53255=CARTESIAN_POINT('Ctrl Pts',(3.75054693397875,1.,0.203550035479166));
#53256=CARTESIAN_POINT('Ctrl Pts',(3.75585118707734,-1.,0.203530796848321));
#53257=CARTESIAN_POINT('Ctrl Pts',(3.75585118707734,1.,0.203530796848321));
#53258=CARTESIAN_POINT('Ctrl Pts',(3.76242717936885,-1.,0.203414634707478));
#53259=CARTESIAN_POINT('Ctrl Pts',(3.76242717936885,1.,0.203414634707478));
#53260=CARTESIAN_POINT('Ctrl Pts',(3.7699207159487,-1.,0.203192390045164));
#53261=CARTESIAN_POINT('Ctrl Pts',(3.7699207159487,1.,0.203192390045164));
#53262=CARTESIAN_POINT('Ctrl Pts',(3.77793553476614,-1.,0.20285472969908));
#53263=CARTESIAN_POINT('Ctrl Pts',(3.77793553476614,1.,0.20285472969908));
#53264=CARTESIAN_POINT('Ctrl Pts',(3.78609175019242,-1.,0.20239426051216));
#53265=CARTESIAN_POINT('Ctrl Pts',(3.78609175019242,1.,0.20239426051216));
#53266=CARTESIAN_POINT('Ctrl Pts',(3.7940835418736,-1.,0.201807533800837));
#53267=CARTESIAN_POINT('Ctrl Pts',(3.7940835418736,1.,0.201807533800837));
#53268=CARTESIAN_POINT('Ctrl Pts',(3.80175247447337,-1.,0.201097756307325));
#53269=CARTESIAN_POINT('Ctrl Pts',(3.80175247447337,1.,0.201097756307325));
#53270=CARTESIAN_POINT('Ctrl Pts',(3.80909529318669,-1.,0.200274679433364));
#53271=CARTESIAN_POINT('Ctrl Pts',(3.80909529318669,1.,0.200274679433364));
#53272=CARTESIAN_POINT('Ctrl Pts',(3.81620203429815,-1.,0.199351525297447));
#53273=CARTESIAN_POINT('Ctrl Pts',(3.81620203429815,1.,0.199351525297447));
#53274=CARTESIAN_POINT('Ctrl Pts',(3.82321127349016,-1.,0.198342616900486));
#53275=CARTESIAN_POINT('Ctrl Pts',(3.82321127349016,1.,0.198342616900486));
#53276=CARTESIAN_POINT('Ctrl Pts',(3.83026221776456,-1.,0.197260935827361));
#53277=CARTESIAN_POINT('Ctrl Pts',(3.83026221776456,1.,0.197260935827361));
#53278=CARTESIAN_POINT('Ctrl Pts',(3.83743910616195,-1.,0.196115198971858));
#53279=CARTESIAN_POINT('Ctrl Pts',(3.83743910616195,1.,0.196115198971858));
#53280=CARTESIAN_POINT('Ctrl Pts',(3.84475203346977,-1.,0.19490900946022));
#53281=CARTESIAN_POINT('Ctrl Pts',(3.84475203346977,1.,0.19490900946022));
#53282=CARTESIAN_POINT('Ctrl Pts',(3.85216762263966,-1.,0.193642806777722));
#53283=CARTESIAN_POINT('Ctrl Pts',(3.85216762263966,1.,0.193642806777722));
#53284=CARTESIAN_POINT('Ctrl Pts',(3.85962774407633,-1.,0.19231515304497));
#53285=CARTESIAN_POINT('Ctrl Pts',(3.85962774407633,1.,0.19231515304497));
#53286=CARTESIAN_POINT('Ctrl Pts',(3.86707158624783,-1.,0.190924190418619));
#53287=CARTESIAN_POINT('Ctrl Pts',(3.86707158624783,1.,0.190924190418619));
#53288=CARTESIAN_POINT('Ctrl Pts',(3.87445976418412,-1.,0.189469253358272));
#53289=CARTESIAN_POINT('Ctrl Pts',(3.87445976418412,1.,0.189469253358272));
#53290=CARTESIAN_POINT('Ctrl Pts',(3.88178563496228,-1.,0.187951632512684));
#53291=CARTESIAN_POINT('Ctrl Pts',(3.88178563496228,1.,0.187951632512684));
#53292=CARTESIAN_POINT('Ctrl Pts',(3.88906196725848,-1.,0.18637372498528));
#53293=CARTESIAN_POINT('Ctrl Pts',(3.88906196725848,1.,0.18637372498528));
#53294=CARTESIAN_POINT('Ctrl Pts',(3.89631300742646,-1.,0.184738537728042));
#53295=CARTESIAN_POINT('Ctrl Pts',(3.89631300742646,1.,0.184738537728042));
#53296=CARTESIAN_POINT('Ctrl Pts',(3.90356488555132,-1.,0.18304908199319));
#53297=CARTESIAN_POINT('Ctrl Pts',(3.90356488555132,1.,0.18304908199319));
#53298=CARTESIAN_POINT('Ctrl Pts',(3.91083557557175,-1.,0.181307740731785));
#53299=CARTESIAN_POINT('Ctrl Pts',(3.91083557557175,1.,0.181307740731785));
#53300=CARTESIAN_POINT('Ctrl Pts',(3.91812876180926,-1.,0.179515885822881));
#53301=CARTESIAN_POINT('Ctrl Pts',(3.91812876180926,1.,0.179515885822881));
#53302=CARTESIAN_POINT('Ctrl Pts',(3.92543942697655,-1.,0.177674246152317));
#53303=CARTESIAN_POINT('Ctrl Pts',(3.92543942697655,1.,0.177674246152317));
#53304=CARTESIAN_POINT('Ctrl Pts',(3.93275726771042,-1.,0.175783136893867));
#53305=CARTESIAN_POINT('Ctrl Pts',(3.93275726771042,1.,0.175783136893867));
#53306=CARTESIAN_POINT('Ctrl Pts',(3.94007083096217,-1.,0.173842734974609));
#53307=CARTESIAN_POINT('Ctrl Pts',(3.94007083096217,1.,0.173842734974609));
#53308=CARTESIAN_POINT('Ctrl Pts',(3.94737164900868,-1.,0.17185335536924));
#53309=CARTESIAN_POINT('Ctrl Pts',(3.94737164900868,1.,0.17185335536924));
#53310=CARTESIAN_POINT('Ctrl Pts',(3.95465744665268,-1.,0.169815666374138));
#53311=CARTESIAN_POINT('Ctrl Pts',(3.95465744665268,1.,0.169815666374138));
#53312=CARTESIAN_POINT('Ctrl Pts',(3.96192990160296,-1.,0.167730547023319));
#53313=CARTESIAN_POINT('Ctrl Pts',(3.96192990160296,1.,0.167730547023319));
#53314=CARTESIAN_POINT('Ctrl Pts',(3.96919313621407,-1.,0.165598992851102));
#53315=CARTESIAN_POINT('Ctrl Pts',(3.96919313621407,1.,0.165598992851102));
#53316=CARTESIAN_POINT('Ctrl Pts',(3.97645194630943,-1.,0.163422004609999));
#53317=CARTESIAN_POINT('Ctrl Pts',(3.97645194630943,1.,0.163422004609999));
#53318=CARTESIAN_POINT('Ctrl Pts',(3.98371010319872,-1.,0.161200482186084));
#53319=CARTESIAN_POINT('Ctrl Pts',(3.98371010319872,1.,0.161200482186084));
#53320=CARTESIAN_POINT('Ctrl Pts',(3.99096873945878,-1.,0.158935123982793));
#53321=CARTESIAN_POINT('Ctrl Pts',(3.99096873945878,1.,0.158935123982793));
#53322=CARTESIAN_POINT('Ctrl Pts',(3.99822717425893,-1.,0.156626481393734));
#53323=CARTESIAN_POINT('Ctrl Pts',(3.99822717425893,1.,0.156626481393734));
#53324=CARTESIAN_POINT('Ctrl Pts',(4.00548360245319,-1.,0.15427500487231));
#53325=CARTESIAN_POINT('Ctrl Pts',(4.00548360245319,1.,0.15427500487231));
#53326=CARTESIAN_POINT('Ctrl Pts',(4.01273584234689,-1.,0.15188109402291));
#53327=CARTESIAN_POINT('Ctrl Pts',(4.01273584234689,1.,0.15188109402291));
#53328=CARTESIAN_POINT('Ctrl Pts',(4.01998203715564,-1.,0.149445144968706));
#53329=CARTESIAN_POINT('Ctrl Pts',(4.01998203715564,1.,0.149445144968706));
#53330=CARTESIAN_POINT('Ctrl Pts',(4.02722143146994,-1.,0.146967602878994));
#53331=CARTESIAN_POINT('Ctrl Pts',(4.02722143146994,1.,0.146967602878994));
#53332=CARTESIAN_POINT('Ctrl Pts',(4.03445411510333,-1.,0.144448947038344));
#53333=CARTESIAN_POINT('Ctrl Pts',(4.03445411510333,1.,0.144448947038344));
#53334=CARTESIAN_POINT('Ctrl Pts',(4.04168069633781,-1.,0.1418896714855));
#53335=CARTESIAN_POINT('Ctrl Pts',(4.04168069633781,1.,0.1418896714855));
#53336=CARTESIAN_POINT('Ctrl Pts',(4.04890199238036,-1.,0.139290267180057));
#53337=CARTESIAN_POINT('Ctrl Pts',(4.04890199238036,1.,0.139290267180057));
#53338=CARTESIAN_POINT('Ctrl Pts',(4.05611873400172,-1.,0.136651205046119));
#53339=CARTESIAN_POINT('Ctrl Pts',(4.05611873400172,1.,0.136651205046119));
#53340=CARTESIAN_POINT('Ctrl Pts',(4.06333121018596,-1.,0.133972916144244));
#53341=CARTESIAN_POINT('Ctrl Pts',(4.06333121018596,1.,0.133972916144244));
#53342=CARTESIAN_POINT('Ctrl Pts',(4.0705393152874,-1.,0.13125579354894));
#53343=CARTESIAN_POINT('Ctrl Pts',(4.0705393152874,1.,0.13125579354894));
#53344=CARTESIAN_POINT('Ctrl Pts',(4.07774270738954,-1.,0.128500200484837));
#53345=CARTESIAN_POINT('Ctrl Pts',(4.07774270738954,1.,0.128500200484837));
#53346=CARTESIAN_POINT('Ctrl Pts',(4.08494093372377,-1.,0.125706476822539));
#53347=CARTESIAN_POINT('Ctrl Pts',(4.08494093372377,1.,0.125706476822539));
#53348=CARTESIAN_POINT('Ctrl Pts',(4.09213355850756,-1.,0.122874946249106));
#53349=CARTESIAN_POINT('Ctrl Pts',(4.09213355850756,1.,0.122874946249106));
#53350=CARTESIAN_POINT('Ctrl Pts',(4.09932031767002,-1.,0.120005924388124));
#53351=CARTESIAN_POINT('Ctrl Pts',(4.09932031767002,1.,0.120005924388124));
#53352=CARTESIAN_POINT('Ctrl Pts',(4.10650113381833,-1.,0.117099722731648));
#53353=CARTESIAN_POINT('Ctrl Pts',(4.10650113381833,1.,0.117099722731648));
#53354=CARTESIAN_POINT('Ctrl Pts',(4.11367603924961,-1.,0.114156649609545));
#53355=CARTESIAN_POINT('Ctrl Pts',(4.11367603924961,1.,0.114156649609545));
#53356=CARTESIAN_POINT('Ctrl Pts',(4.1208451250225,-1.,0.111177012683346));
#53357=CARTESIAN_POINT('Ctrl Pts',(4.1208451250225,1.,0.111177012683346));
#53358=CARTESIAN_POINT('Ctrl Pts',(4.12800848371504,-1.,0.108161120528369));
#53359=CARTESIAN_POINT('Ctrl Pts',(4.12800848371504,1.,0.108161120528369));
#53360=CARTESIAN_POINT('Ctrl Pts',(4.13516614458895,-1.,0.105109286538945));
#53361=CARTESIAN_POINT('Ctrl Pts',(4.13516614458895,1.,0.105109286538945));
#53362=CARTESIAN_POINT('Ctrl Pts',(4.14231804939538,-1.,0.102021826577583));
#53363=CARTESIAN_POINT('Ctrl Pts',(4.14231804939538,1.,0.102021826577583));
#53364=CARTESIAN_POINT('Ctrl Pts',(4.14946408918485,-1.,0.0988990478901221));
#53365=CARTESIAN_POINT('Ctrl Pts',(4.14946408918485,1.,0.0988990478901221));
#53366=CARTESIAN_POINT('Ctrl Pts',(4.15660412653577,-1.,0.0957412403298002));
#53367=CARTESIAN_POINT('Ctrl Pts',(4.15660412653577,1.,0.0957412403298002));
#53368=CARTESIAN_POINT('Ctrl Pts',(4.16373802265839,-1.,0.0925486672167526));
#53369=CARTESIAN_POINT('Ctrl Pts',(4.16373802265839,1.,0.0925486672167526));
#53370=CARTESIAN_POINT('Ctrl Pts',(4.17086566490794,-1.,0.0893215560848644));
#53371=CARTESIAN_POINT('Ctrl Pts',(4.17086566490794,1.,0.0893215560848644));
#53372=CARTESIAN_POINT('Ctrl Pts',(4.17798698668094,-1.,0.0860600915549391));
#53373=CARTESIAN_POINT('Ctrl Pts',(4.17798698668094,1.,0.0860600915549391));
#53374=CARTESIAN_POINT('Ctrl Pts',(4.18510195327123,-1.,0.0827644164385674));
#53375=CARTESIAN_POINT('Ctrl Pts',(4.18510195327123,1.,0.0827644164385674));
#53376=CARTESIAN_POINT('Ctrl Pts',(4.19078883320504,-1.,0.0801005887114315));
#53377=CARTESIAN_POINT('Ctrl Pts',(4.19078883320504,1.,0.0801005887114315));
#53378=CARTESIAN_POINT('Ctrl Pts',(4.19505112859416,-1.,0.0780873956242392));
#53379=CARTESIAN_POINT('Ctrl Pts',(4.19505112859416,1.,0.0780873956242392));
#53380=CARTESIAN_POINT('Ctrl Pts',(4.1978913862118,-1.,0.0767384596141459));
#53381=CARTESIAN_POINT('Ctrl Pts',(4.1978913862118,1.,0.0767384596141459));
#53382=CARTESIAN_POINT('Ctrl Pts',(4.19931119685982,-1.,0.0760622897878241));
#53383=CARTESIAN_POINT('Ctrl Pts',(4.19931119685982,1.,0.0760622897878241));
#53384=CARTESIAN_POINT('',(3.74449296983004,1.,0.2031560948961));
#53385=CARTESIAN_POINT('Ctrl Pts',(3.74449296983004,-1.,0.2031560948961));
#53386=CARTESIAN_POINT('Ctrl Pts',(3.74449296983004,-0.666666666666667,
0.2031560948961));
#53387=CARTESIAN_POINT('Ctrl Pts',(3.74449296983004,-0.333333333333333,
0.2031560948961));
#53388=CARTESIAN_POINT('Ctrl Pts',(3.74449296983004,0.333333333333333,0.2031560948961));
#53389=CARTESIAN_POINT('Ctrl Pts',(3.74449296983004,0.666666666666667,0.2031560948961));
#53390=CARTESIAN_POINT('Ctrl Pts',(3.74449296983004,1.,0.2031560948961));
#53391=CARTESIAN_POINT('',(4.19931119685982,1.,0.0760622897878241));
#53392=CARTESIAN_POINT('',(4.19931119685982,0.,0.0760622897878241));
#53393=CARTESIAN_POINT('Ctrl Pts',(3.74449296983004,1.,0.2031560948961));
#53394=CARTESIAN_POINT('Ctrl Pts',(3.74453008995092,1.,0.203188003946656));
#53395=CARTESIAN_POINT('Ctrl Pts',(3.74471097893845,1.,0.20326661011053));
#53396=CARTESIAN_POINT('Ctrl Pts',(3.74535749969115,1.,0.203375226874121));
#53397=CARTESIAN_POINT('Ctrl Pts',(3.74703926501752,1.,0.203484186269415));
#53398=CARTESIAN_POINT('Ctrl Pts',(3.75054693397875,1.,0.203550035479166));
#53399=CARTESIAN_POINT('Ctrl Pts',(3.75585118707734,1.,0.203530796848321));
#53400=CARTESIAN_POINT('Ctrl Pts',(3.76242717936885,1.,0.203414634707478));
#53401=CARTESIAN_POINT('Ctrl Pts',(3.7699207159487,1.,0.203192390045164));
#53402=CARTESIAN_POINT('Ctrl Pts',(3.77793553476614,1.,0.20285472969908));
#53403=CARTESIAN_POINT('Ctrl Pts',(3.78609175019242,1.,0.20239426051216));
#53404=CARTESIAN_POINT('Ctrl Pts',(3.7940835418736,1.,0.201807533800837));
#53405=CARTESIAN_POINT('Ctrl Pts',(3.80175247447337,1.,0.201097756307325));
#53406=CARTESIAN_POINT('Ctrl Pts',(3.80909529318669,1.,0.200274679433364));
#53407=CARTESIAN_POINT('Ctrl Pts',(3.81620203429815,1.,0.199351525297447));
#53408=CARTESIAN_POINT('Ctrl Pts',(3.82321127349016,1.,0.198342616900486));
#53409=CARTESIAN_POINT('Ctrl Pts',(3.83026221776456,1.,0.197260935827361));
#53410=CARTESIAN_POINT('Ctrl Pts',(3.83743910616195,1.,0.196115198971858));
#53411=CARTESIAN_POINT('Ctrl Pts',(3.84475203346977,1.,0.19490900946022));
#53412=CARTESIAN_POINT('Ctrl Pts',(3.85216762263966,1.,0.193642806777722));
#53413=CARTESIAN_POINT('Ctrl Pts',(3.85962774407633,1.,0.19231515304497));
#53414=CARTESIAN_POINT('Ctrl Pts',(3.86707158624783,1.,0.190924190418619));
#53415=CARTESIAN_POINT('Ctrl Pts',(3.87445976418412,1.,0.189469253358272));
#53416=CARTESIAN_POINT('Ctrl Pts',(3.88178563496228,1.,0.187951632512684));
#53417=CARTESIAN_POINT('Ctrl Pts',(3.88906196725848,1.,0.18637372498528));
#53418=CARTESIAN_POINT('Ctrl Pts',(3.89631300742646,1.,0.184738537728042));
#53419=CARTESIAN_POINT('Ctrl Pts',(3.90356488555132,1.,0.18304908199319));
#53420=CARTESIAN_POINT('Ctrl Pts',(3.91083557557175,1.,0.181307740731785));
#53421=CARTESIAN_POINT('Ctrl Pts',(3.91812876180926,1.,0.179515885822881));
#53422=CARTESIAN_POINT('Ctrl Pts',(3.92543942697655,1.,0.177674246152317));
#53423=CARTESIAN_POINT('Ctrl Pts',(3.93275726771042,1.,0.175783136893867));
#53424=CARTESIAN_POINT('Ctrl Pts',(3.94007083096217,1.,0.173842734974609));
#53425=CARTESIAN_POINT('Ctrl Pts',(3.94737164900868,1.,0.17185335536924));
#53426=CARTESIAN_POINT('Ctrl Pts',(3.95465744665268,1.,0.169815666374138));
#53427=CARTESIAN_POINT('Ctrl Pts',(3.96192990160296,1.,0.167730547023319));
#53428=CARTESIAN_POINT('Ctrl Pts',(3.96919313621407,1.,0.165598992851102));
#53429=CARTESIAN_POINT('Ctrl Pts',(3.97645194630943,1.,0.163422004609999));
#53430=CARTESIAN_POINT('Ctrl Pts',(3.98371010319872,1.,0.161200482186084));
#53431=CARTESIAN_POINT('Ctrl Pts',(3.99096873945878,1.,0.158935123982793));
#53432=CARTESIAN_POINT('Ctrl Pts',(3.99822717425893,1.,0.156626481393734));
#53433=CARTESIAN_POINT('Ctrl Pts',(4.00548360245319,1.,0.15427500487231));
#53434=CARTESIAN_POINT('Ctrl Pts',(4.01273584234689,1.,0.15188109402291));
#53435=CARTESIAN_POINT('Ctrl Pts',(4.01998203715564,1.,0.149445144968706));
#53436=CARTESIAN_POINT('Ctrl Pts',(4.02722143146994,1.,0.146967602878994));
#53437=CARTESIAN_POINT('Ctrl Pts',(4.03445411510333,1.,0.144448947038344));
#53438=CARTESIAN_POINT('Ctrl Pts',(4.04168069633781,1.,0.1418896714855));
#53439=CARTESIAN_POINT('Ctrl Pts',(4.04890199238036,1.,0.139290267180057));
#53440=CARTESIAN_POINT('Ctrl Pts',(4.05611873400172,1.,0.136651205046119));
#53441=CARTESIAN_POINT('Ctrl Pts',(4.06333121018596,1.,0.133972916144244));
#53442=CARTESIAN_POINT('Ctrl Pts',(4.0705393152874,1.,0.13125579354894));
#53443=CARTESIAN_POINT('Ctrl Pts',(4.07774270738954,1.,0.128500200484837));
#53444=CARTESIAN_POINT('Ctrl Pts',(4.08494093372377,1.,0.125706476822539));
#53445=CARTESIAN_POINT('Ctrl Pts',(4.09213355850756,1.,0.122874946249106));
#53446=CARTESIAN_POINT('Ctrl Pts',(4.09932031767002,1.,0.120005924388124));
#53447=CARTESIAN_POINT('Ctrl Pts',(4.10650113381833,1.,0.117099722731648));
#53448=CARTESIAN_POINT('Ctrl Pts',(4.11367603924961,1.,0.114156649609545));
#53449=CARTESIAN_POINT('Ctrl Pts',(4.1208451250225,1.,0.111177012683346));
#53450=CARTESIAN_POINT('Ctrl Pts',(4.12800848371504,1.,0.108161120528369));
#53451=CARTESIAN_POINT('Ctrl Pts',(4.13516614458895,1.,0.105109286538945));
#53452=CARTESIAN_POINT('Ctrl Pts',(4.14231804939538,1.,0.102021826577583));
#53453=CARTESIAN_POINT('Ctrl Pts',(4.14946408918485,1.,0.0988990478901221));
#53454=CARTESIAN_POINT('Ctrl Pts',(4.15660412653577,1.,0.0957412403298002));
#53455=CARTESIAN_POINT('Ctrl Pts',(4.16373802265839,1.,0.0925486672167526));
#53456=CARTESIAN_POINT('Ctrl Pts',(4.17086566490794,1.,0.0893215560848644));
#53457=CARTESIAN_POINT('Ctrl Pts',(4.17798698668094,1.,0.0860600915549391));
#53458=CARTESIAN_POINT('Ctrl Pts',(4.18510195327123,1.,0.0827644164385674));
#53459=CARTESIAN_POINT('Ctrl Pts',(4.19078883320504,1.,0.0801005887114315));
#53460=CARTESIAN_POINT('Ctrl Pts',(4.19505112859416,1.,0.0780873956242392));
#53461=CARTESIAN_POINT('Ctrl Pts',(4.1978913862118,1.,0.0767384596141459));
#53462=CARTESIAN_POINT('Ctrl Pts',(4.19931119685982,1.,0.0760622897878241));
#53463=CARTESIAN_POINT('Ctrl Pts',(4.19931119685982,-1.,-0.0760622897878241));
#53464=CARTESIAN_POINT('Ctrl Pts',(4.19931119685982,1.,-0.0760622897878241));
#53465=CARTESIAN_POINT('Ctrl Pts',(4.19789138621624,-1.,-0.07673845961422));
#53466=CARTESIAN_POINT('Ctrl Pts',(4.19789138621624,1.,-0.07673845961422));
#53467=CARTESIAN_POINT('Ctrl Pts',(4.19505112860624,-1.,-0.0780873956244407));
#53468=CARTESIAN_POINT('Ctrl Pts',(4.19505112860624,1.,-0.0780873956244407));
#53469=CARTESIAN_POINT('Ctrl Pts',(4.19078883322483,-1.,-0.0801005887117608));
#53470=CARTESIAN_POINT('Ctrl Pts',(4.19078883322483,1.,-0.0801005887117608));
#53471=CARTESIAN_POINT('Ctrl Pts',(4.1851019532944,-1.,-0.0827644164389515));
#53472=CARTESIAN_POINT('Ctrl Pts',(4.1851019532944,1.,-0.0827644164389515));
#53473=CARTESIAN_POINT('Ctrl Pts',(4.17798698669991,-1.,-0.086060091555252));
#53474=CARTESIAN_POINT('Ctrl Pts',(4.17798698669991,1.,-0.086060091555252));
#53475=CARTESIAN_POINT('Ctrl Pts',(4.17086566491823,-1.,-0.0893215560850332));
#53476=CARTESIAN_POINT('Ctrl Pts',(4.17086566491823,1.,-0.0893215560850332));
#53477=CARTESIAN_POINT('Ctrl Pts',(4.16373802265942,-1.,-0.0925486672167695));
#53478=CARTESIAN_POINT('Ctrl Pts',(4.16373802265942,1.,-0.0925486672167695));
#53479=CARTESIAN_POINT('Ctrl Pts',(4.15660412653006,-1.,-0.0957412403297072));
#53480=CARTESIAN_POINT('Ctrl Pts',(4.15660412653006,1.,-0.0957412403297072));
#53481=CARTESIAN_POINT('Ctrl Pts',(4.1494640891762,-1.,-0.0988990478899816));
#53482=CARTESIAN_POINT('Ctrl Pts',(4.1494640891762,1.,-0.0988990478899816));
#53483=CARTESIAN_POINT('Ctrl Pts',(4.14231804938737,-1.,-0.102021826577454));
#53484=CARTESIAN_POINT('Ctrl Pts',(4.14231804938737,1.,-0.102021826577454));
#53485=CARTESIAN_POINT('Ctrl Pts',(4.13516614458396,-1.,-0.105109286538864));
#53486=CARTESIAN_POINT('Ctrl Pts',(4.13516614458396,1.,-0.105109286538864));
#53487=CARTESIAN_POINT('Ctrl Pts',(4.12800848371386,-1.,-0.10816112052835));
#53488=CARTESIAN_POINT('Ctrl Pts',(4.12800848371386,1.,-0.10816112052835));
#53489=CARTESIAN_POINT('Ctrl Pts',(4.12084512502444,-1.,-0.111177012683378));
#53490=CARTESIAN_POINT('Ctrl Pts',(4.12084512502444,1.,-0.111177012683378));
#53491=CARTESIAN_POINT('Ctrl Pts',(4.11367603925313,-1.,-0.114156649609602));
#53492=CARTESIAN_POINT('Ctrl Pts',(4.11367603925313,1.,-0.114156649609602));
#53493=CARTESIAN_POINT('Ctrl Pts',(4.10650113382187,-1.,-0.117099722731705));
#53494=CARTESIAN_POINT('Ctrl Pts',(4.10650113382187,1.,-0.117099722731705));
#53495=CARTESIAN_POINT('Ctrl Pts',(4.09932031767243,-1.,-0.120005924388162));
#53496=CARTESIAN_POINT('Ctrl Pts',(4.09932031767243,1.,-0.120005924388162));
#53497=CARTESIAN_POINT('Ctrl Pts',(4.09213355850836,-1.,-0.122874946249119));
#53498=CARTESIAN_POINT('Ctrl Pts',(4.09213355850836,1.,-0.122874946249119));
#53499=CARTESIAN_POINT('Ctrl Pts',(4.08494093372315,-1.,-0.12570647682253));
#53500=CARTESIAN_POINT('Ctrl Pts',(4.08494093372315,1.,-0.12570647682253));
#53501=CARTESIAN_POINT('Ctrl Pts',(4.07774270738809,-1.,-0.128500200484814));
#53502=CARTESIAN_POINT('Ctrl Pts',(4.07774270738809,1.,-0.128500200484814));
#53503=CARTESIAN_POINT('Ctrl Pts',(4.07053931528579,-1.,-0.131255793548914));
#53504=CARTESIAN_POINT('Ctrl Pts',(4.07053931528579,1.,-0.131255793548914));
#53505=CARTESIAN_POINT('Ctrl Pts',(4.06333121018476,-1.,-0.133972916144225));
#53506=CARTESIAN_POINT('Ctrl Pts',(4.06333121018476,1.,-0.133972916144225));
#53507=CARTESIAN_POINT('Ctrl Pts',(4.05611873400122,-1.,-0.136651205046111));
#53508=CARTESIAN_POINT('Ctrl Pts',(4.05611873400122,1.,-0.136651205046111));
#53509=CARTESIAN_POINT('Ctrl Pts',(4.04890199238056,-1.,-0.13929026718006));
#53510=CARTESIAN_POINT('Ctrl Pts',(4.04890199238056,1.,-0.13929026718006));
#53511=CARTESIAN_POINT('Ctrl Pts',(4.04168069633842,-1.,-0.141889671485508));
#53512=CARTESIAN_POINT('Ctrl Pts',(4.04168069633842,1.,-0.141889671485508));
#53513=CARTESIAN_POINT('Ctrl Pts',(4.03445411510403,-1.,-0.144448947038352));
#53514=CARTESIAN_POINT('Ctrl Pts',(4.03445411510403,1.,-0.144448947038352));
#53515=CARTESIAN_POINT('Ctrl Pts',(4.02722143147048,-1.,-0.146967602878999));
#53516=CARTESIAN_POINT('Ctrl Pts',(4.02722143147048,1.,-0.146967602878999));
#53517=CARTESIAN_POINT('Ctrl Pts',(4.01998203715588,-1.,-0.149445144968708));
#53518=CARTESIAN_POINT('Ctrl Pts',(4.01998203715588,1.,-0.149445144968708));
#53519=CARTESIAN_POINT('Ctrl Pts',(4.01273584234684,-1.,-0.151881094022909));
#53520=CARTESIAN_POINT('Ctrl Pts',(4.01273584234684,1.,-0.151881094022909));
#53521=CARTESIAN_POINT('Ctrl Pts',(4.00548360245297,-1.,-0.15427500487231));
#53522=CARTESIAN_POINT('Ctrl Pts',(4.00548360245297,1.,-0.15427500487231));
#53523=CARTESIAN_POINT('Ctrl Pts',(3.99822717425869,-1.,-0.156626481393736));
#53524=CARTESIAN_POINT('Ctrl Pts',(3.99822717425869,1.,-0.156626481393736));
#53525=CARTESIAN_POINT('Ctrl Pts',(3.99096873945862,-1.,-0.158935123982796));
#53526=CARTESIAN_POINT('Ctrl Pts',(3.99096873945862,1.,-0.158935123982796));
#53527=CARTESIAN_POINT('Ctrl Pts',(3.98371010319866,-1.,-0.161200482186088));
#53528=CARTESIAN_POINT('Ctrl Pts',(3.98371010319866,1.,-0.161200482186088));
#53529=CARTESIAN_POINT('Ctrl Pts',(3.97645194630944,-1.,-0.163422004609999));
#53530=CARTESIAN_POINT('Ctrl Pts',(3.97645194630944,1.,-0.163422004609999));
#53531=CARTESIAN_POINT('Ctrl Pts',(3.9691931362141,-1.,-0.165598992851098));
#53532=CARTESIAN_POINT('Ctrl Pts',(3.9691931362141,1.,-0.165598992851098));
#53533=CARTESIAN_POINT('Ctrl Pts',(3.96192990160296,-1.,-0.167730547023312));
#53534=CARTESIAN_POINT('Ctrl Pts',(3.96192990160296,1.,-0.167730547023312));
#53535=CARTESIAN_POINT('Ctrl Pts',(3.95465744665263,-1.,-0.16981566637413));
#53536=CARTESIAN_POINT('Ctrl Pts',(3.95465744665263,1.,-0.16981566637413));
#53537=CARTESIAN_POINT('Ctrl Pts',(3.94737164900861,-1.,-0.171853355369233));
#53538=CARTESIAN_POINT('Ctrl Pts',(3.94737164900861,1.,-0.171853355369233));
#53539=CARTESIAN_POINT('Ctrl Pts',(3.94007083096214,-1.,-0.173842734974608));
#53540=CARTESIAN_POINT('Ctrl Pts',(3.94007083096214,1.,-0.173842734974608));
#53541=CARTESIAN_POINT('Ctrl Pts',(3.93275726771049,-1.,-0.175783136893873));
#53542=CARTESIAN_POINT('Ctrl Pts',(3.93275726771049,1.,-0.175783136893873));
#53543=CARTESIAN_POINT('Ctrl Pts',(3.92543942697672,-1.,-0.177674246152328));
#53544=CARTESIAN_POINT('Ctrl Pts',(3.92543942697672,1.,-0.177674246152328));
#53545=CARTESIAN_POINT('Ctrl Pts',(3.91812876180948,-1.,-0.179515885822895));
#53546=CARTESIAN_POINT('Ctrl Pts',(3.91812876180948,1.,-0.179515885822895));
#53547=CARTESIAN_POINT('Ctrl Pts',(3.91083557557193,-1.,-0.181307740731796));
#53548=CARTESIAN_POINT('Ctrl Pts',(3.91083557557193,1.,-0.181307740731796));
#53549=CARTESIAN_POINT('Ctrl Pts',(3.90356488555138,-1.,-0.183049081993193));
#53550=CARTESIAN_POINT('Ctrl Pts',(3.90356488555138,1.,-0.183049081993193));
#53551=CARTESIAN_POINT('Ctrl Pts',(3.89631300742633,-1.,-0.184738537728035));
#53552=CARTESIAN_POINT('Ctrl Pts',(3.89631300742633,1.,-0.184738537728035));
#53553=CARTESIAN_POINT('Ctrl Pts',(3.88906196725817,-1.,-0.186373724985263));
#53554=CARTESIAN_POINT('Ctrl Pts',(3.88906196725817,1.,-0.186373724985263));
#53555=CARTESIAN_POINT('Ctrl Pts',(3.88178563496187,-1.,-0.187951632512664));
#53556=CARTESIAN_POINT('Ctrl Pts',(3.88178563496187,1.,-0.187951632512664));
#53557=CARTESIAN_POINT('Ctrl Pts',(3.87445976418377,-1.,-0.189469253358255));
#53558=CARTESIAN_POINT('Ctrl Pts',(3.87445976418377,1.,-0.189469253358255));
#53559=CARTESIAN_POINT('Ctrl Pts',(3.8670715862477,-1.,-0.190924190418613));
#53560=CARTESIAN_POINT('Ctrl Pts',(3.8670715862477,1.,-0.190924190418613));
#53561=CARTESIAN_POINT('Ctrl Pts',(3.85962774407652,-1.,-0.19231515304498));
#53562=CARTESIAN_POINT('Ctrl Pts',(3.85962774407652,1.,-0.19231515304498));
#53563=CARTESIAN_POINT('Ctrl Pts',(3.85216762264019,-1.,-0.193642806777748));
#53564=CARTESIAN_POINT('Ctrl Pts',(3.85216762264019,1.,-0.193642806777748));
#53565=CARTESIAN_POINT('Ctrl Pts',(3.84475203347052,-1.,-0.194909009460255));
#53566=CARTESIAN_POINT('Ctrl Pts',(3.84475203347052,1.,-0.194909009460255));
#53567=CARTESIAN_POINT('Ctrl Pts',(3.83743910616265,-1.,-0.19611519897189));
#53568=CARTESIAN_POINT('Ctrl Pts',(3.83743910616265,1.,-0.19611519897189));
#53569=CARTESIAN_POINT('Ctrl Pts',(3.83026221776488,-1.,-0.197260935827375));
#53570=CARTESIAN_POINT('Ctrl Pts',(3.83026221776488,1.,-0.197260935827375));
#53571=CARTESIAN_POINT('Ctrl Pts',(3.82321127348981,-1.,-0.19834261690047));
#53572=CARTESIAN_POINT('Ctrl Pts',(3.82321127348981,1.,-0.19834261690047));
#53573=CARTESIAN_POINT('Ctrl Pts',(3.81620203429702,-1.,-0.199351525297397));
#53574=CARTESIAN_POINT('Ctrl Pts',(3.81620203429702,1.,-0.199351525297397));
#53575=CARTESIAN_POINT('Ctrl Pts',(3.80909529318501,-1.,-0.20027467943329));
#53576=CARTESIAN_POINT('Ctrl Pts',(3.80909529318501,1.,-0.20027467943329));
#53577=CARTESIAN_POINT('Ctrl Pts',(3.80175247447171,-1.,-0.201097756307252));
#53578=CARTESIAN_POINT('Ctrl Pts',(3.80175247447171,1.,-0.201097756307252));
#53579=CARTESIAN_POINT('Ctrl Pts',(3.79408354187274,-1.,-0.201807533800799));
#53580=CARTESIAN_POINT('Ctrl Pts',(3.79408354187274,1.,-0.201807533800799));
#53581=CARTESIAN_POINT('Ctrl Pts',(3.78609175019317,-1.,-0.202394260512193));
#53582=CARTESIAN_POINT('Ctrl Pts',(3.78609175019317,1.,-0.202394260512193));
#53583=CARTESIAN_POINT('Ctrl Pts',(3.77793553476879,-1.,-0.202854729699197));
#53584=CARTESIAN_POINT('Ctrl Pts',(3.77793553476879,1.,-0.202854729699197));
#53585=CARTESIAN_POINT('Ctrl Pts',(3.76992071595267,-1.,-0.203192390045338));
#53586=CARTESIAN_POINT('Ctrl Pts',(3.76992071595267,1.,-0.203192390045338));
#53587=CARTESIAN_POINT('Ctrl Pts',(3.76242717937273,-1.,-0.203414634707647));
#53588=CARTESIAN_POINT('Ctrl Pts',(3.76242717937273,1.,-0.203414634707647));
#53589=CARTESIAN_POINT('Ctrl Pts',(3.75585118707924,-1.,-0.203530796848404));
#53590=CARTESIAN_POINT('Ctrl Pts',(3.75585118707924,1.,-0.203530796848404));
#53591=CARTESIAN_POINT('Ctrl Pts',(3.75054693397716,-1.,-0.203550035479097));
#53592=CARTESIAN_POINT('Ctrl Pts',(3.75054693397716,1.,-0.203550035479097));
#53593=CARTESIAN_POINT('Ctrl Pts',(3.74675472018582,-1.,-0.20347884453023));
#53594=CARTESIAN_POINT('Ctrl Pts',(3.74675472018582,1.,-0.20347884453023));
#53595=CARTESIAN_POINT('Ctrl Pts',(3.7450208092684,-1.,-0.203352057956056));
#53596=CARTESIAN_POINT('Ctrl Pts',(3.7450208092684,1.,-0.203352057956056));
#53597=CARTESIAN_POINT('Ctrl Pts',(3.74446880195845,-1.,-0.203218215747895));
#53598=CARTESIAN_POINT('Ctrl Pts',(3.74446880195845,1.,-0.203218215747895));
#53599=CARTESIAN_POINT('Ctrl Pts',(3.74443319346666,-1.,-0.20311176758786));
#53600=CARTESIAN_POINT('Ctrl Pts',(3.74443319346666,1.,-0.20311176758786));
#53601=CARTESIAN_POINT('Ctrl Pts',(3.74449849461127,-1.,-0.20305423869972));
#53602=CARTESIAN_POINT('Ctrl Pts',(3.74449849461127,1.,-0.20305423869972));
#53603=CARTESIAN_POINT('',(4.19931119685982,1.,-0.0760622897878241));
#53604=CARTESIAN_POINT('Ctrl Pts',(4.19931119685982,1.,-0.0760622897878241));
#53605=CARTESIAN_POINT('Ctrl Pts',(4.19789138621624,1.,-0.07673845961422));
#53606=CARTESIAN_POINT('Ctrl Pts',(4.19505112860624,1.,-0.0780873956244407));
#53607=CARTESIAN_POINT('Ctrl Pts',(4.19078883322483,1.,-0.0801005887117608));
#53608=CARTESIAN_POINT('Ctrl Pts',(4.1851019532944,1.,-0.0827644164389515));
#53609=CARTESIAN_POINT('Ctrl Pts',(4.17798698669991,1.,-0.086060091555252));
#53610=CARTESIAN_POINT('Ctrl Pts',(4.17086566491823,1.,-0.0893215560850332));
#53611=CARTESIAN_POINT('Ctrl Pts',(4.16373802265942,1.,-0.0925486672167695));
#53612=CARTESIAN_POINT('Ctrl Pts',(4.15660412653006,1.,-0.0957412403297072));
#53613=CARTESIAN_POINT('Ctrl Pts',(4.1494640891762,1.,-0.0988990478899816));
#53614=CARTESIAN_POINT('Ctrl Pts',(4.14231804938737,1.,-0.102021826577454));
#53615=CARTESIAN_POINT('Ctrl Pts',(4.13516614458396,1.,-0.105109286538864));
#53616=CARTESIAN_POINT('Ctrl Pts',(4.12800848371386,1.,-0.10816112052835));
#53617=CARTESIAN_POINT('Ctrl Pts',(4.12084512502444,1.,-0.111177012683378));
#53618=CARTESIAN_POINT('Ctrl Pts',(4.11367603925313,1.,-0.114156649609602));
#53619=CARTESIAN_POINT('Ctrl Pts',(4.10650113382187,1.,-0.117099722731705));
#53620=CARTESIAN_POINT('Ctrl Pts',(4.09932031767243,1.,-0.120005924388162));
#53621=CARTESIAN_POINT('Ctrl Pts',(4.09213355850836,1.,-0.122874946249119));
#53622=CARTESIAN_POINT('Ctrl Pts',(4.08494093372315,1.,-0.12570647682253));
#53623=CARTESIAN_POINT('Ctrl Pts',(4.07774270738809,1.,-0.128500200484814));
#53624=CARTESIAN_POINT('Ctrl Pts',(4.07053931528579,1.,-0.131255793548914));
#53625=CARTESIAN_POINT('Ctrl Pts',(4.06333121018476,1.,-0.133972916144225));
#53626=CARTESIAN_POINT('Ctrl Pts',(4.05611873400122,1.,-0.136651205046111));
#53627=CARTESIAN_POINT('Ctrl Pts',(4.04890199238056,1.,-0.13929026718006));
#53628=CARTESIAN_POINT('Ctrl Pts',(4.04168069633842,1.,-0.141889671485508));
#53629=CARTESIAN_POINT('Ctrl Pts',(4.03445411510403,1.,-0.144448947038352));
#53630=CARTESIAN_POINT('Ctrl Pts',(4.02722143147048,1.,-0.146967602878999));
#53631=CARTESIAN_POINT('Ctrl Pts',(4.01998203715588,1.,-0.149445144968708));
#53632=CARTESIAN_POINT('Ctrl Pts',(4.01273584234684,1.,-0.151881094022909));
#53633=CARTESIAN_POINT('Ctrl Pts',(4.00548360245297,1.,-0.15427500487231));
#53634=CARTESIAN_POINT('Ctrl Pts',(3.99822717425869,1.,-0.156626481393736));
#53635=CARTESIAN_POINT('Ctrl Pts',(3.99096873945862,1.,-0.158935123982796));
#53636=CARTESIAN_POINT('Ctrl Pts',(3.98371010319866,1.,-0.161200482186088));
#53637=CARTESIAN_POINT('Ctrl Pts',(3.97645194630944,1.,-0.163422004609999));
#53638=CARTESIAN_POINT('Ctrl Pts',(3.9691931362141,1.,-0.165598992851098));
#53639=CARTESIAN_POINT('Ctrl Pts',(3.96192990160296,1.,-0.167730547023312));
#53640=CARTESIAN_POINT('Ctrl Pts',(3.95465744665263,1.,-0.16981566637413));
#53641=CARTESIAN_POINT('Ctrl Pts',(3.94737164900861,1.,-0.171853355369233));
#53642=CARTESIAN_POINT('Ctrl Pts',(3.94007083096214,1.,-0.173842734974608));
#53643=CARTESIAN_POINT('Ctrl Pts',(3.93275726771049,1.,-0.175783136893873));
#53644=CARTESIAN_POINT('Ctrl Pts',(3.92543942697672,1.,-0.177674246152328));
#53645=CARTESIAN_POINT('Ctrl Pts',(3.91812876180948,1.,-0.179515885822895));
#53646=CARTESIAN_POINT('Ctrl Pts',(3.91083557557193,1.,-0.181307740731796));
#53647=CARTESIAN_POINT('Ctrl Pts',(3.90356488555138,1.,-0.183049081993193));
#53648=CARTESIAN_POINT('Ctrl Pts',(3.89631300742633,1.,-0.184738537728035));
#53649=CARTESIAN_POINT('Ctrl Pts',(3.88906196725817,1.,-0.186373724985263));
#53650=CARTESIAN_POINT('Ctrl Pts',(3.88178563496187,1.,-0.187951632512664));
#53651=CARTESIAN_POINT('Ctrl Pts',(3.87445976418377,1.,-0.189469253358255));
#53652=CARTESIAN_POINT('Ctrl Pts',(3.8670715862477,1.,-0.190924190418613));
#53653=CARTESIAN_POINT('Ctrl Pts',(3.85962774407652,1.,-0.19231515304498));
#53654=CARTESIAN_POINT('Ctrl Pts',(3.85216762264019,1.,-0.193642806777748));
#53655=CARTESIAN_POINT('Ctrl Pts',(3.84475203347052,1.,-0.194909009460255));
#53656=CARTESIAN_POINT('Ctrl Pts',(3.83743910616265,1.,-0.19611519897189));
#53657=CARTESIAN_POINT('Ctrl Pts',(3.83026221776488,1.,-0.197260935827375));
#53658=CARTESIAN_POINT('Ctrl Pts',(3.82321127348981,1.,-0.19834261690047));
#53659=CARTESIAN_POINT('Ctrl Pts',(3.81620203429702,1.,-0.199351525297397));
#53660=CARTESIAN_POINT('Ctrl Pts',(3.80909529318501,1.,-0.20027467943329));
#53661=CARTESIAN_POINT('Ctrl Pts',(3.80175247447171,1.,-0.201097756307252));
#53662=CARTESIAN_POINT('Ctrl Pts',(3.79408354187274,1.,-0.201807533800799));
#53663=CARTESIAN_POINT('Ctrl Pts',(3.78609175019317,1.,-0.202394260512193));
#53664=CARTESIAN_POINT('Ctrl Pts',(3.77793553476879,1.,-0.202854729699197));
#53665=CARTESIAN_POINT('Ctrl Pts',(3.76992071595267,1.,-0.203192390045338));
#53666=CARTESIAN_POINT('Ctrl Pts',(3.76242717937273,1.,-0.203414634707647));
#53667=CARTESIAN_POINT('Ctrl Pts',(3.75585118707924,1.,-0.203530796848404));
#53668=CARTESIAN_POINT('Ctrl Pts',(3.75054693397716,1.,-0.203550035479097));
#53669=CARTESIAN_POINT('Ctrl Pts',(3.74703926501843,1.,-0.203484186269315));
#53670=CARTESIAN_POINT('Ctrl Pts',(3.74535749969262,1.,-0.203375226874332));
#53671=CARTESIAN_POINT('Ctrl Pts',(3.74471097893961,1.,-0.203266610111264));
#53672=CARTESIAN_POINT('Ctrl Pts',(3.74453008995129,1.,-0.203188003947965));
#53673=CARTESIAN_POINT('Ctrl Pts',(3.74449296982994,1.,-0.203156094897896));
#53674=CARTESIAN_POINT('',(4.19931119685982,0.,-0.0760622897878241));
#53675=CARTESIAN_POINT('Origin',(4.19931119685982,0.,0.0760622897878241));
#53676=CARTESIAN_POINT('',(4.19931119685982,1.,-0.0760622897878241));
#53677=CARTESIAN_POINT('Origin',(0.,1.,0.));
#53678=CARTESIAN_POINT('Origin',(0.,1.,0.));
#53679=CARTESIAN_POINT('Origin',(0.,0.,0.));
#53856=UNCERTAINTY_MEASURE_WITH_UNIT(LENGTH_MEASURE(0.001),#53910,
'DISTANCE_ACCURACY_VALUE',
'Maximum model space distance between geometric entities at asserted c
onnectivities');
#53859=UNCERTAINTY_MEASURE_WITH_UNIT(LENGTH_MEASURE(0.001),#53910,
'DISTANCE_ACCURACY_VALUE',
'Maximum model space distance between geometric entities at asserted c
onnectivities');
#53906=(
GEOMETRIC_REPRESENTATION_CONTEXT(3)
GLOBAL_UNCERTAINTY_ASSIGNED_CONTEXT((#53856))
GLOBAL_UNIT_ASSIGNED_CONTEXT((#53910,#53912,#53913))
REPRESENTATION_CONTEXT('','3D')
);
#53909=(
GEOMETRIC_REPRESENTATION_CONTEXT(3)
GLOBAL_UNCERTAINTY_ASSIGNED_CONTEXT((#53859))
GLOBAL_UNIT_ASSIGNED_CONTEXT((#53910,#53912,#53913))
REPRESENTATION_CONTEXT('','3D')
);
#53910=(
LENGTH_UNIT()
NAMED_UNIT(*)
SI_UNIT(.CENTI.,.METRE.)
);
#53912=(
NAMED_UNIT(*)
PLANE_ANGLE_UNIT()
SI_UNIT($,.RADIAN.)
);
#53913=(
NAMED_UNIT(*)
SI_UNIT($,.STERADIAN.)
SOLID_ANGLE_UNIT()
);
#53960=SHAPE_DEFINITION_REPRESENTATION(#54058,#54132);
#54058=PRODUCT_DEFINITION_SHAPE('',$,#54182);
#54132=SHAPE_REPRESENTATION('',(#12756),#53906);
#54135=PRODUCT_DEFINITION_CONTEXT('part definition',#54284,'design');
#54182=PRODUCT_DEFINITION('Spur Gear - Module 2, 40 Teeth, 20 mm Bore',
'Spur Gear - Module 2, 40 Teeth, 20 mm Bore',#54231,#54135);
#54231=PRODUCT_DEFINITION_FORMATION('',$,#54332);
#54284=APPLICATION_CONTEXT(
'Core Data for Automotive Mechanical Design Process');
#54285=PRODUCT_CONTEXT('part definition',#54284,'mechanical');
#54332=PRODUCT('Spur Gear - Module 2, 40 Teeth, 20 mm Bore',
'Spur Gear - Module 2, 40 Teeth, 20 mm Bore',
'Spur Gear - Module 2, 40 Teeth, 20 mm Bore',(#54285));
#54384=COLOUR_RGB('Sky Blue',0.24,0.69,0.87);
#54385=FILL_AREA_STYLE_COLOUR('',#54384);
#54386=FILL_AREA_STYLE('',(#54385));
#54387=SURFACE_STYLE_FILL_AREA(#54386);
#54388=SURFACE_SIDE_STYLE('',(#54387));
#54389=SURFACE_STYLE_USAGE(.BOTH.,#54388);
#54390=PRESENTATION_STYLE_ASSIGNMENT((#54389));
ENDSEC;
END-ISO-10303-21;
